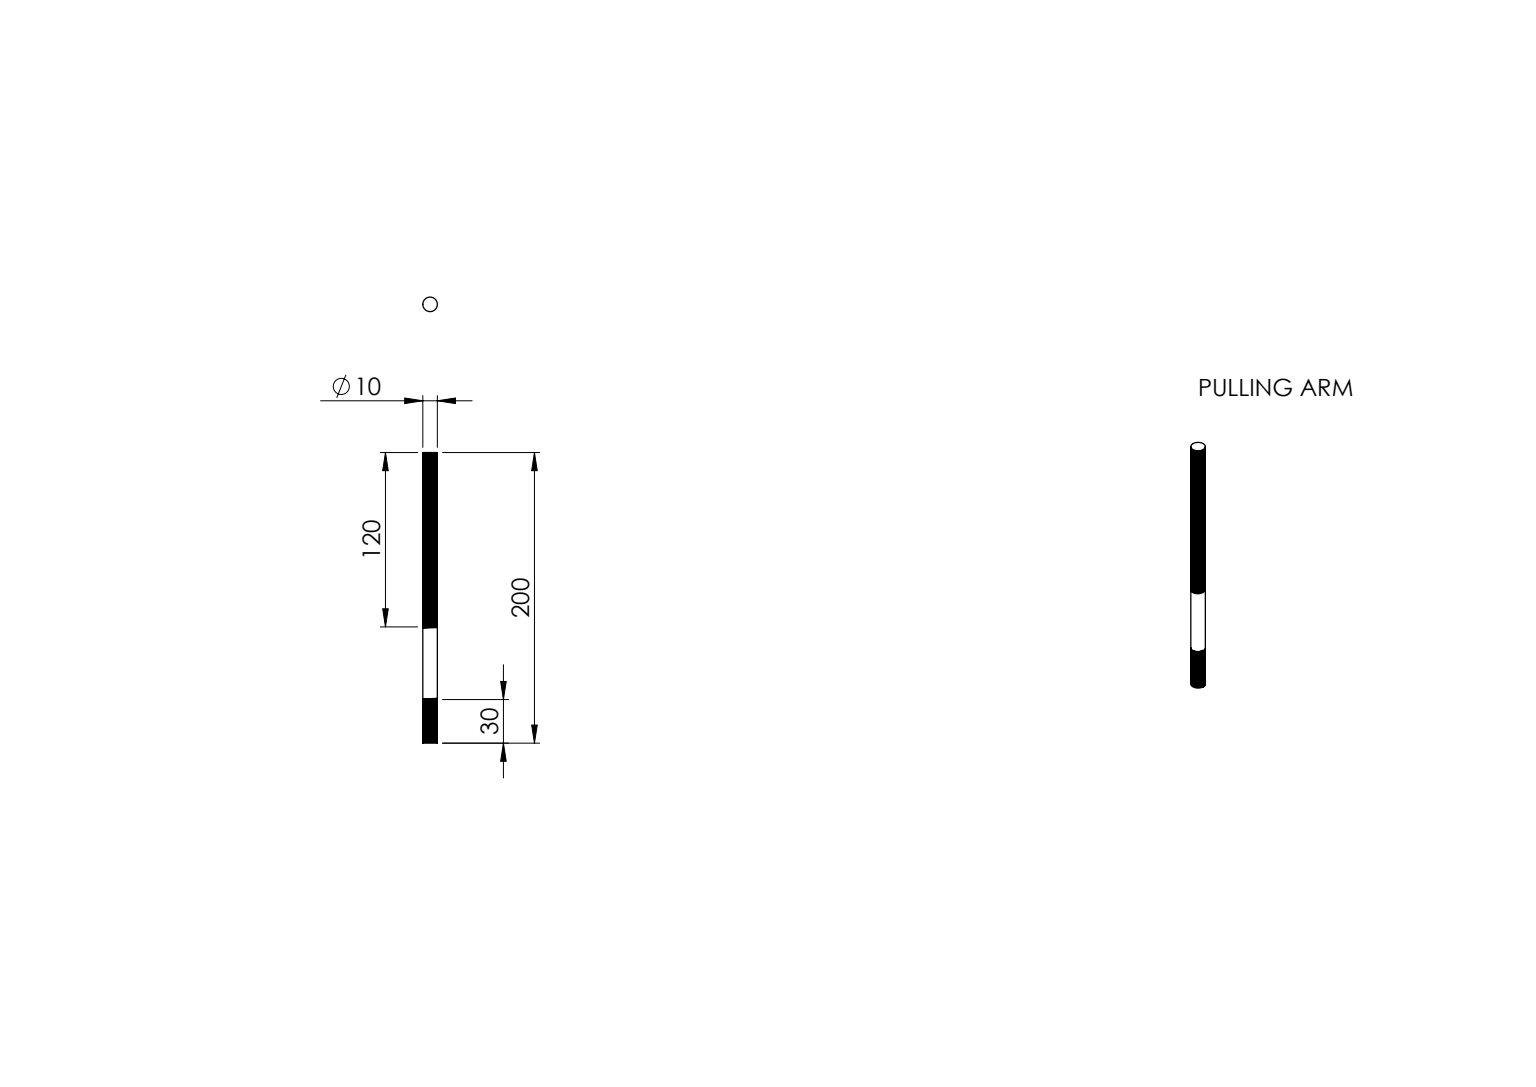
ISO-10303-21;
HEADER;
FILE_DESCRIPTION (('STEP AP214'),
    '1' );
FILE_NAME ('pulling arm.step',
    '2026-10-25T05:52:03',
    ( '' ),
    ( '' ),
    'SwSTEP 2.0',
    'SolidWorks 2026',
    '' );
FILE_SCHEMA (( 'AUTOMOTIVE_DESIGN' ));
ENDSEC;

DATA;
#1=CARTESIAN_POINT ( 'NONE',  ( -5.000000000000000888, -163.4375000000000284, 2.071067811865474617 ) ) ;
#4=ADVANCED_FACE ( 'NONE', ( #1643 ), #54385, .T. ) ;
#5=CARTESIAN_POINT ( 'NONE',  ( -4.458734124999998549, -12.47916666530107221, 2.574251347313722516 ) ) ;
#6=CARTESIAN_POINT ( 'NONE',  ( 2.229367062499998831, -45.89583333196774362, -3.861377020970580887 ) ) ;
#8=ADVANCED_FACE ( 'NONE', ( #45365 ), #55019, .T. ) ;
#9=CARTESIAN_POINT ( 'NONE',  ( -2.499999999999996447, -7.708333330602144429, 4.330127018922195425 ) ) ;
#10=CARTESIAN_POINT ( 'NONE',  ( -4.458734124999999437, -146.9375000013656063, -5.460374474430324690E-16 ) ) ;
#12=CARTESIAN_POINT ( 'NONE',  ( 3.061616997868383141E-16, -166.8750000027312126, -5.000000000000000000 ) ) ;
#15=CARTESIAN_POINT ( 'NONE',  ( -6.972266317189433020E-16, -69.12499999726880162, -5.000000000000000000 ) ) ;
#18=EDGE_LOOP ( 'NONE', ( #47508, #46479, #24387, #28082 ) ) ;
#23=CARTESIAN_POINT ( 'NONE',  ( -5.000000000000000000, -51.00000000000000711, 0.000000000000000000 ) ) ;
#24=CARTESIAN_POINT ( 'NONE',  ( -3.152548672688508926E-16, -0.5624999986344053626, -5.148502694627439702 ) ) ;
#26=CARTESIAN_POINT ( 'NONE',  ( -8.190561711645485556E-16, -153.6875000013656063, 4.458734124999999437 ) ) ;
#31=CARTESIAN_POINT ( 'NONE',  ( -2.499999999999996447, -74.83333333333332860, 4.330127018922195425 ) ) ;
#35=CARTESIAN_POINT ( 'NONE',  ( 2.499999999999998668, 29.66666666666666430, -4.330127018922193649 ) ) ;
#42=CARTESIAN_POINT ( 'NONE',  ( 4.458734124999999437, 16.18750000136559564, -5.460374474430324690E-16 ) ) ;
#45=CARTESIAN_POINT ( 'NONE',  ( -4.458734124999999437, -10.64583333196773829, -2.574251347313719407 ) ) ;
#48=CARTESIAN_POINT ( 'NONE',  ( 1.846868145590735200, -169.2500000013655779, -4.458734125000000326 ) ) ;
#49=CARTESIAN_POINT ( 'NONE',  ( 1.339745962155612702, -63.16965819600734022, -5.000000000000000000 ) ) ;
#50=AXIS2_PLACEMENT_3D ( 'NONE', #21966, #51867, #12316 ) ;
#55=CARTESIAN_POINT ( 'NONE',  ( 0.000000000000000000, -170.0000000000000000, 5.000000000000000000 ) ) ;
#57=CARTESIAN_POINT ( 'NONE',  ( -1.846868145590734756, -152.3750000013655779, -4.458734124999999437 ) ) ;
#59=CARTESIAN_POINT ( 'NONE',  ( 5.000000000000000000, -46.50000000000000000, -6.123233995736766282E-16 ) ) ;
#60=DIRECTION ( 'NONE',  ( -0.000000000000000000, 1.000000000000000000, -0.000000000000000000 ) ) ;
#64=DIRECTION ( 'NONE',  ( 0.000000000000000000, 0.000000000000000000, 1.000000000000000000 ) ) ;
#65=CARTESIAN_POINT ( 'NONE',  ( 5.000000000000000000, -2.500000000000002220, -6.123233995736766282E-16 ) ) ;
#66=CARTESIAN_POINT ( 'NONE',  ( 4.458734125000000326, -68.89583333196773651, 2.574251347313718519 ) ) ;
#67=CARTESIAN_POINT ( 'NONE',  ( -6.972266317189433020E-16, -49.24999999999999289, -5.000000000000000000 ) ) ;
#68=CARTESIAN_POINT ( 'NONE',  ( -2.499999999999996447, 0.2916666693978525737, 4.330127018922195425 ) ) ;
#69=CARTESIAN_POINT ( 'NONE',  ( -3.152548672688508926E-16, -36.56249999863441502, -5.148502694627439702 ) ) ;
#72=CARTESIAN_POINT ( 'NONE',  ( 1.975475456537005874E-15, 5.250000000000000000, 5.000000000000000000 ) ) ;
#73=CARTESIAN_POINT ( 'NONE',  ( 2.500000000000002220, -47.66666666666666430, 4.330127018922192761 ) ) ;
#74=CARTESIAN_POINT ( 'NONE',  ( 5.000000000000000000, -46.29166666393545881, -2.886751345948130876 ) ) ;
#77=CARTESIAN_POINT ( 'NONE',  ( -4.458734124999999437, -71.39583333196773651, -2.574251347313719407 ) ) ;
#78=( BOUNDED_CURVE ( )  B_SPLINE_CURVE ( 2, ( #57244, #32782, #8347, #47568, #3519, #57557, #53655, #9590, #43673 ),
 .UNSPECIFIED., .F., .F. ) 
 B_SPLINE_CURVE_WITH_KNOTS ( ( 3, 2, 2, 2, 3 ),
 ( 0.6562500000000000000, 0.6569444444444444420, 0.6583333333333333259, 0.6597222222222222099, 0.6604166666666666519 ),
 .UNSPECIFIED. ) 
 CURVE ( )  GEOMETRIC_REPRESENTATION_ITEM ( )  RATIONAL_B_SPLINE_CURVE ( ( 0.9330127018922194093, 0.9330127018922194093, 1.000000000000000000, 0.8660254037844387076, 1.000000000000000000, 0.8660254037844387076, 1.000000000000000000, 0.9330127018922194093, 0.9330127018922194093 ) ) 
 REPRESENTATION_ITEM ( '' )  );
#79=CARTESIAN_POINT ( 'NONE',  ( 4.458734124999999437, -144.7500000013656063, 1.846868145590737864 ) ) ;
#80=CARTESIAN_POINT ( 'NONE',  ( 2.229367062499998831, -80.64583333196773651, -3.861377020970580887 ) ) ;
#82=CARTESIAN_POINT ( 'NONE',  ( -2.229367062500000163, -28.72916666530107221, -3.861377020970580443 ) ) ;
#83=CARTESIAN_POINT ( 'NONE',  ( 5.000000000000000888, -73.45833333060214443, 2.886751345948126879 ) ) ;
#87=CARTESIAN_POINT ( 'NONE',  ( 0.000000000000000000, -170.0000000000000000, 0.000000000000000000 ) ) ;
#88=ORIENTED_EDGE ( 'NONE', *, *, #56635, .F. ) ;
#92=EDGE_LOOP ( 'NONE', ( #43267, #11517, #3797, #45500 ) ) ;
#95=EDGE_CURVE ( 'NONE', #8105, #59664, #19555, .T. ) ;
#96=CARTESIAN_POINT ( 'NONE',  ( -5.000000000000000000, -83.08333333333332860, -2.886751345948128211 ) ) ;
#97=CARTESIAN_POINT ( 'NONE',  ( -4.458734124999999437, -59.56249999863440081, 0.000000000000000000 ) ) ;
#98=EDGE_CURVE ( 'NONE', #46757, #28361, #15466, .T. ) ;
#105=CARTESIAN_POINT ( 'NONE',  ( 2.229367062500001939, 13.02083333469892779, 3.861377020970579999 ) ) ;
#107=CARTESIAN_POINT ( 'NONE',  ( 5.000000000000000888, -32.58333333333333570, 2.886751345948126879 ) ) ;
#108=CARTESIAN_POINT ( 'NONE',  ( -4.458734124999999437, -165.9375000013655779, -5.460374474430324690E-16 ) ) ;
#109=ORIENTED_EDGE ( 'NONE', *, *, #27518, .F. ) ;
#112=EDGE_CURVE ( 'NONE', #57087, #7190, #37304, .T. ) ;
#116=CARTESIAN_POINT ( 'NONE',  ( -4.999999999999998224, 2.083333333333333037, 2.886751345948131764 ) ) ;
#119=CARTESIAN_POINT ( 'NONE',  ( 3.061616997868383141E-16, -154.8750000027311842, -5.000000000000000000 ) ) ;
#122=CARTESIAN_POINT ( 'NONE',  ( -6.972266317189433020E-16, -58.24999999999999289, -5.000000000000000000 ) ) ;
#125=CARTESIAN_POINT ( 'NONE',  ( 4.458734124999998549, 8.020833334698926009, -2.574251347313721627 ) ) ;
#128=CARTESIAN_POINT ( 'NONE',  ( -9.184850993605147944E-16, -149.3750000027312126, 5.000000000000000000 ) ) ;
#133=CARTESIAN_POINT ( 'NONE',  ( -2.071067811865475061, -143.6875000000000284, -5.000000000000000888 ) ) ;
#135=CARTESIAN_POINT ( 'NONE',  ( 4.458734124999999437, -165.6250000013656063, -1.846868145590734978 ) ) ;
#136=CARTESIAN_POINT ( 'NONE',  ( 2.229367062499998831, -35.64583333196772941, -3.861377020970580887 ) ) ;
#137=CYLINDRICAL_SURFACE ( 'NONE', #42021, 5.000000000000000000 ) ;
#138=DIRECTION ( 'NONE',  ( 0.000000000000000000, 0.000000000000000000, 1.000000000000000000 ) ) ;
#140=CARTESIAN_POINT ( 'NONE',  ( 4.458734124999999437, -143.4375000013656063, 0.000000000000000000 ) ) ;
#141=VERTEX_POINT ( 'NONE', #56933 ) ;
#142=CARTESIAN_POINT ( 'NONE',  ( 4.458734125000001214, 28.85416666803225993, 2.574251347313718519 ) ) ;
#144=CARTESIAN_POINT ( 'NONE',  ( -2.229367062499996610, -62.39583333196774362, 3.861377020970582219 ) ) ;
#147=CARTESIAN_POINT ( 'NONE',  ( -5.000000000000000000, 17.91666666666666430, -2.886751345948128211 ) ) ;
#148=CARTESIAN_POINT ( 'NONE',  ( -3.152548672688508926E-16, -50.56249999863440792, -5.148502694627439702 ) ) ;
#149=CARTESIAN_POINT ( 'NONE',  ( -4.458734124999999437, -8.395833331967736513, -2.574251347313719407 ) ) ;
#153=CARTESIAN_POINT ( 'NONE',  ( 5.000000000000000000, -53.37499999726881583, -6.123233995736766282E-16 ) ) ;
#154=CARTESIAN_POINT ( 'NONE',  ( -6.972266317189433020E-16, 0.7499999999999996669, -5.000000000000000000 ) ) ;
#157=CARTESIAN_POINT ( 'NONE',  ( -3.152548672688508926E-16, -54.56249999863439371, -5.148502694627439702 ) ) ;
#158=CARTESIAN_POINT ( 'NONE',  ( -1.846868145590737420, -157.0000000013655779, 4.458734124999999437 ) ) ;
#160=CARTESIAN_POINT ( 'NONE',  ( -2.500000000000000444, -56.04166666393548013, -4.330127018922193649 ) ) ;
#161=EDGE_LOOP ( 'NONE', ( #40738, #29551, #10837, #16509 ) ) ;
#162=CARTESIAN_POINT ( 'NONE',  ( -3.152548672688508926E-16, 6.187500001365593860, -5.148502694627439702 ) ) ;
#165=FACE_OUTER_BOUND ( 'NONE', #54429, .T. ) ;
#166=CARTESIAN_POINT ( 'NONE',  ( 2.730187237215162345E-16, -156.1875000013655779, -4.458734124999999437 ) ) ;
#168=CARTESIAN_POINT ( 'NONE',  ( 5.000000000000000000, -87.29166666393547303, -2.886751345948130876 ) ) ;
#170=CARTESIAN_POINT ( 'NONE',  ( 0.000000000000000000, -170.0000000000000000, 0.000000000000000000 ) ) ;
#171=CARTESIAN_POINT ( 'NONE',  ( -4.458734124999999437, -45.56249999863440081, 0.000000000000000000 ) ) ;
#173=CARTESIAN_POINT ( 'NONE',  ( 1.339745962155615144, 9.419658201469706782, 4.999999999999999112 ) ) ;
#175=CARTESIAN_POINT ( 'NONE',  ( -5.000000000000000000, -156.6250000027311842, -6.123233995736766282E-16 ) ) ;
#176=VERTEX_POINT ( 'NONE', #46964 ) ;
#177=CARTESIAN_POINT ( 'NONE',  ( 9.457646018065525792E-16, -89.31249999863440792, 5.148502694627439702 ) ) ;
#179=CARTESIAN_POINT ( 'NONE',  ( -3.535533905932737309, -165.6250000000000284, -3.535533905932738197 ) ) ;
#181=CARTESIAN_POINT ( 'NONE',  ( 1.975475456537005874E-15, -52.62499999726880873, 5.000000000000000000 ) ) ;
#185=CARTESIAN_POINT ( 'NONE',  ( -5.000000000000000000, -78.95833333060213022, -2.886751345948128211 ) ) ;
#189=CARTESIAN_POINT ( 'NONE',  ( 2.500000000000002220, -42.54166666393548013, 4.330127018922192761 ) ) ;
#190=CARTESIAN_POINT ( 'NONE',  ( -1.339745962155613812, -46.08034179853028434, -5.000000000000000000 ) ) ;
#197=CARTESIAN_POINT ( 'NONE',  ( 5.000000000000000000, -162.1875000027311842, 2.071067811865478614 ) ) ;
#207=CARTESIAN_POINT ( 'NONE',  ( -6.972266317189433020E-16, -48.12499999726880873, -5.000000000000000000 ) ) ;
#208=CARTESIAN_POINT ( 'NONE',  ( 9.457646018065525792E-16, -14.06249999863440436, 5.148502694627439702 ) ) ;
#209=CARTESIAN_POINT ( 'NONE',  ( 2.499999999999998668, -71.33333333333332860, -4.330127018922193649 ) ) ;
#210=CARTESIAN_POINT ( 'NONE',  ( -9.184850993605147944E-16, -153.2500000000000000, 5.000000000000000000 ) ) ;
#213=CARTESIAN_POINT ( 'NONE',  ( -2.229367062499996610, -46.39583333196774362, 3.861377020970582219 ) ) ;
#219=CARTESIAN_POINT ( 'NONE',  ( -2.229367062499996610, 11.85416666803225993, 3.861377020970582219 ) ) ;
#222=CARTESIAN_POINT ( 'NONE',  ( -2.229367062500000163, -88.72916666530106511, -3.861377020970580443 ) ) ;
#223=CARTESIAN_POINT ( 'NONE',  ( -2.229367062500000163, 20.27083333469892779, -3.861377020970580443 ) ) ;
#225=CARTESIAN_POINT ( 'NONE',  ( 5.000000000000000000, 8.708333336064518093, -2.886751345948129988 ) ) ;
#226=ORIENTED_EDGE ( 'NONE', *, *, #26912, .F. ) ;
#229=( BOUNDED_CURVE ( )  B_SPLINE_CURVE ( 2, ( #7653, #61058, #50752, #27257, #26303, #46568, #45926, #60737, #46883 ),
 .UNSPECIFIED., .F., .F. ) 
 B_SPLINE_CURVE_WITH_KNOTS ( ( 3, 2, 2, 2, 3 ),
 ( 0.3562500000000000111, 0.3569444444444444531, 0.3583333333333333370, 0.3597222222222222210, 0.3604166666666666630 ),
 .UNSPECIFIED. ) 
 CURVE ( )  GEOMETRIC_REPRESENTATION_ITEM ( )  RATIONAL_B_SPLINE_CURVE ( ( 0.9330127018922194093, 0.9330127018922194093, 1.000000000000000000, 0.8660254037844387076, 1.000000000000000000, 0.8660254037844387076, 1.000000000000000000, 0.9330127018922194093, 0.9330127018922194093 ) ) 
 REPRESENTATION_ITEM ( '' )  );
#230=CARTESIAN_POINT ( 'NONE',  ( 1.060575238724906964E-15, -36.75000000000000711, 5.773502691896257311 ) ) ;
#231=CARTESIAN_POINT ( 'NONE',  ( 4.458734124999998549, -35.72916666530107221, -2.574251347313721627 ) ) ;
#232=CARTESIAN_POINT ( 'NONE',  ( -3.535250795749689387E-16, -35.12499999726881583, -5.773502691896257311 ) ) ;
#233=CARTESIAN_POINT ( 'NONE',  ( -4.458734124999998549, -68.22916666530107932, 2.574251347313722516 ) ) ;
#234=ORIENTED_EDGE ( 'NONE', *, *, #6265, .F. ) ;
#236=CARTESIAN_POINT ( 'NONE',  ( -3.152548672688508926E-16, -12.56249999863440081, -5.148502694627439702 ) ) ;
#237=CARTESIAN_POINT ( 'NONE',  ( -3.152548672688508926E-16, -15.81249999863440436, -5.148502694627439702 ) ) ;
#238=ORIENTED_EDGE ( 'NONE', *, *, #445, .F. ) ;
#239=CARTESIAN_POINT ( 'NONE',  ( 2.500000000000002220, -83.66666666666667140, 4.330127018922192761 ) ) ;
#240=CARTESIAN_POINT ( 'NONE',  ( -4.458734125000000326, -167.0000000013655779, -1.846868145590735644 ) ) ;
#243=CARTESIAN_POINT ( 'NONE',  ( 5.000000000000000000, -81.29166666393547303, -2.886751345948129988 ) ) ;
#244=LINE ( 'NONE', #10504, #18998 ) ;
#247=CARTESIAN_POINT ( 'NONE',  ( -4.458734124999998549, -29.47916666530106866, 2.574251347313722516 ) ) ;
#250=CARTESIAN_POINT ( 'NONE',  ( 1.846868145590736310, -167.8750000013656063, 4.458734124999999437 ) ) ;
#252=CYLINDRICAL_SURFACE ( 'NONE', #21504, 5.000000000000000000 ) ;
#257=CARTESIAN_POINT ( 'NONE',  ( -1.846868145590734756, -147.3750000013656063, -4.458734124999999437 ) ) ;
#259=CARTESIAN_POINT ( 'NONE',  ( 6.123233995736766282E-16, -170.0000000000000000, -5.000000000000000000 ) ) ;
#264=CARTESIAN_POINT ( 'NONE',  ( -4.458734125000001214, -141.1250000013655779, 1.846868145590734089 ) ) ;
#269=CARTESIAN_POINT ( 'NONE',  ( 4.458734125000001214, -75.14583333196775072, 2.574251347313718519 ) ) ;
#271=CARTESIAN_POINT ( 'NONE',  ( 1.975475456537005874E-15, -69.74999999999998579, 5.000000000000000000 ) ) ;
#272=CARTESIAN_POINT ( 'NONE',  ( -6.972266317189433020E-16, -58.12499999726880162, -5.000000000000000000 ) ) ;
#275=CARTESIAN_POINT ( 'NONE',  ( -6.972266317189433020E-16, 13.87500000273118594, -5.000000000000000000 ) ) ;
#281=CARTESIAN_POINT ( 'NONE',  ( -4.458734124999999437, 16.43750000136559564, 0.000000000000000000 ) ) ;
#288=CARTESIAN_POINT ( 'NONE',  ( -4.458734124999999437, 2.687500001365593860, 0.000000000000000000 ) ) ;
#289=ORIENTED_EDGE ( 'NONE', *, *, #15037, .T. ) ;
#290=CARTESIAN_POINT ( 'NONE',  ( 4.458734124999999437, -24.06249999863440436, -5.460374474430324690E-16 ) ) ;
#294=CARTESIAN_POINT ( 'NONE',  ( 4.458734125000001214, 25.10416666803225638, 2.574251347313718519 ) ) ;
#297=CARTESIAN_POINT ( 'NONE',  ( -4.458734124999997661, -71.47916666530107932, 2.574251347313722516 ) ) ;
#300=CARTESIAN_POINT ( 'NONE',  ( 2.499999999999998668, 27.79166666939785202, -4.330127018922193649 ) ) ;
#301=ORIENTED_EDGE ( 'NONE', *, *, #22893, .T. ) ;
#303=CARTESIAN_POINT ( 'NONE',  ( 5.000000000000000000, -18.50000000000000355, -6.123233995736766282E-16 ) ) ;
#304=CARTESIAN_POINT ( 'NONE',  ( -4.458734124999999437, -22.39583333196773651, -2.574251347313719407 ) ) ;
#305=CARTESIAN_POINT ( 'NONE',  ( -2.229367062500000163, -81.47916666530106511, -3.861377020970580443 ) ) ;
#306=CARTESIAN_POINT ( 'NONE',  ( 1.846868145590735200, -166.5000000013655779, -4.458734125000000326 ) ) ;
#307=CARTESIAN_POINT ( 'NONE',  ( 1.060575238724906964E-15, -19.62499999726881583, 5.773502691896257311 ) ) ;
#308=CARTESIAN_POINT ( 'NONE',  ( 4.458734124999999437, -48.81249999863440792, -5.460374474430324690E-16 ) ) ;
#312=CARTESIAN_POINT ( 'NONE',  ( -3.152548672688508926E-16, 3.187500001365594748, -5.148502694627439702 ) ) ;
#315=CARTESIAN_POINT ( 'NONE',  ( -2.500000000000000444, -64.16666666666665719, -4.330127018922193649 ) ) ;
#316=CARTESIAN_POINT ( 'NONE',  ( -1.846868145590737420, -152.0000000013655779, 4.458734124999999437 ) ) ;
#319=CARTESIAN_POINT ( 'NONE',  ( 5.000000000000000888, -161.9375000000000284, -2.071067811865475505 ) ) ;
#320=FACE_OUTER_BOUND ( 'NONE', #3833, .T. ) ;
#322=CARTESIAN_POINT ( 'NONE',  ( 2.229367062499998831, -10.89583333196773829, -3.861377020970580887 ) ) ;
#323=CARTESIAN_POINT ( 'NONE',  ( 4.458734124999998549, -45.97916666530106511, -2.574251347313721627 ) ) ;
#324=CARTESIAN_POINT ( 'NONE',  ( -6.972266317189433020E-16, -8.124999997268814056, -5.000000000000000000 ) ) ;
#325=CARTESIAN_POINT ( 'NONE',  ( -8.190561711645485556E-16, -149.6875000013656063, 4.458734124999999437 ) ) ;
#328=VERTEX_POINT ( 'NONE', #61131 ) ;
#332=CARTESIAN_POINT ( 'NONE',  ( 5.000000000000000888, -29.45833333060214443, 2.886751345948126879 ) ) ;
#338=CARTESIAN_POINT ( 'NONE',  ( -5.147856630858197489E-14, 2.375000002731183724, 5.000000000000000000 ) ) ;
#339=CARTESIAN_POINT ( 'NONE',  ( -4.458734124999999437, -4.395833331967740065, -2.574251347313719407 ) ) ;
#340=DIRECTION ( 'NONE',  ( -0.000000000000000000, -1.000000000000000000, -0.000000000000000000 ) ) ;
#341=CARTESIAN_POINT ( 'NONE',  ( 4.458734124999997661, -148.5000000013656347, 1.846868145590737864 ) ) ;
#348=CARTESIAN_POINT ( 'NONE',  ( 1.162044386198238837E-16, 28.37500000273118417, 5.000000000000000000 ) ) ;
#349=( BOUNDED_CURVE ( )  B_SPLINE_CURVE ( 2, ( #32871, #48595, #37379, #53427, #52500, #18392, #37690, #3921, #43452 ),
 .UNSPECIFIED., .F., .F. ) 
 B_SPLINE_CURVE_WITH_KNOTS ( ( 3, 2, 2, 2, 3 ),
 ( 0.5229166666666666963, 0.5236111111111111382, 0.5250000000000000222, 0.5263888888888889062, 0.5270833333333333481 ),
 .UNSPECIFIED. ) 
 CURVE ( )  GEOMETRIC_REPRESENTATION_ITEM ( )  RATIONAL_B_SPLINE_CURVE ( ( 0.9330127018922194093, 0.9330127018922194093, 1.000000000000000000, 0.8660254037844387076, 1.000000000000000000, 0.8660254037844387076, 1.000000000000000000, 0.9330127018922194093, 0.9330127018922194093 ) ) 
 REPRESENTATION_ITEM ( '' )  );
#355=DIRECTION ( 'NONE',  ( -0.000000000000000000, 1.000000000000000000, -0.000000000000000000 ) ) ;
#356=CARTESIAN_POINT ( 'NONE',  ( -2.229367062500000163, 18.52083333469892779, -3.861377020970580443 ) ) ;
#359=CARTESIAN_POINT ( 'NONE',  ( 4.458734125000000326, -8.145833331967736513, 2.574251347313718519 ) ) ;
#362=CARTESIAN_POINT ( 'NONE',  ( -4.458734125000000326, -169.0000000013655779, -1.846868145590735644 ) ) ;
#366=ADVANCED_FACE ( 'NONE', ( #2909 ), #32473, .T. ) ;
#369=CARTESIAN_POINT ( 'NONE',  ( 5.000000000000000000, -142.1875000027312126, 2.071067811865478614 ) ) ;
#371=CARTESIAN_POINT ( 'NONE',  ( 3.152801135295366208, -153.8125000013656063, 3.152801135295367985 ) ) ;
#373=CARTESIAN_POINT ( 'NONE',  ( 1.339745962155615144, -46.70534180126147561, 4.999999999999999112 ) ) ;
#379=CARTESIAN_POINT ( 'NONE',  ( -2.500000000000000444, -2.166666666666663854, -4.330127018922193649 ) ) ;
#380=EDGE_CURVE ( 'NONE', #47490, #35906, #55280, .T. ) ;
#381=CARTESIAN_POINT ( 'NONE',  ( -4.458734124999999437, -67.39583333196773651, -2.574251347313719407 ) ) ;
#384=CARTESIAN_POINT ( 'NONE',  ( 5.000000000000000000, -1.291666663935479908, -2.886751345948129988 ) ) ;
#385=CARTESIAN_POINT ( 'NONE',  ( -4.458734124999999437, -36.31249999863440792, 0.000000000000000000 ) ) ;
#386=ORIENTED_EDGE ( 'NONE', *, *, #25943, .F. ) ;
#390=ORIENTED_EDGE ( 'NONE', *, *, #14942, .T. ) ;
#391=CARTESIAN_POINT ( 'NONE',  ( -6.972266317189433020E-16, 5.749999999999999112, -5.000000000000000000 ) ) ;
#392=CARTESIAN_POINT ( 'NONE',  ( 2.500000000000002220, -50.66666666666666430, 4.330127018922192761 ) ) ;
#395=CARTESIAN_POINT ( 'NONE',  ( -5.000000000000000000, -4.083333333333334814, -2.886751345948128211 ) ) ;
#396=CARTESIAN_POINT ( 'NONE',  ( 4.458734124999998549, -72.72916666530106511, -2.574251347313721627 ) ) ;
#397=CARTESIAN_POINT ( 'NONE',  ( -3.152801135295367096, -143.3125000013655779, -3.152801135295367541 ) ) ;
#398=CARTESIAN_POINT ( 'NONE',  ( -2.229367062499996610, -81.14583333196773651, 3.861377020970582219 ) ) ;
#400=CARTESIAN_POINT ( 'NONE',  ( 9.457646018065525792E-16, -31.31249999863440436, 5.148502694627439702 ) ) ;
#401=CARTESIAN_POINT ( 'NONE',  ( -4.999999999999999112, -70.79166666393548724, 2.886751345948131764 ) ) ;
#406=CARTESIAN_POINT ( 'NONE',  ( 1.339745962155614256, 28.70534180126147561, -4.999999999999999112 ) ) ;
#407=ORIENTED_EDGE ( 'NONE', *, *, #54703, .T. ) ;
#409=( BOUNDED_CURVE ( )  B_SPLINE_CURVE ( 2, ( #59998, #10777, #6592, #50336, #36184, #21392, #31028, #50979, #30387 ),
 .UNSPECIFIED., .F., .F. ) 
 B_SPLINE_CURVE_WITH_KNOTS ( ( 3, 2, 2, 2, 3 ),
 ( 0.4083333333333336590, 0.4125000000000003109, 0.4166666666666670182, 0.4208333333333336701, 0.4250000000000003220 ),
 .UNSPECIFIED. ) 
 CURVE ( )  GEOMETRIC_REPRESENTATION_ITEM ( )  RATIONAL_B_SPLINE_CURVE ( ( 0.9999999999999938938, 0.9238795325112928447, 1.000000000000000000, 0.9238795325112867385, 1.000000000000000000, 0.9238795325112867385, 1.000000000000000000, 0.9238795325112806323, 1.000000000000005995 ) ) 
 REPRESENTATION_ITEM ( '' )  );
#411=EDGE_CURVE ( 'NONE', #51356, #16274, #33465, .T. ) ;
#412=CARTESIAN_POINT ( 'NONE',  ( 2.229367062499998831, -56.89583333196773651, -3.861377020970580887 ) ) ;
#414=ORIENTED_EDGE ( 'NONE', *, *, #41306, .F. ) ;
#415=CARTESIAN_POINT ( 'NONE',  ( -5.000000000000000888, -146.5625000000000000, -2.071067811865475949 ) ) ;
#417=CARTESIAN_POINT ( 'NONE',  ( -4.458734124999998549, 11.77083333469892601, 2.574251347313722516 ) ) ;
#419=CARTESIAN_POINT ( 'NONE',  ( -4.458734124999999437, -162.0000000013656063, -1.846868145590735644 ) ) ;
#422=CARTESIAN_POINT ( 'NONE',  ( -5.000000000000000000, -69.87499999726880162, 0.000000000000000000 ) ) ;
#425=CARTESIAN_POINT ( 'NONE',  ( -6.972266317189433020E-16, -40.12499999726880162, -5.000000000000000000 ) ) ;
#428=CARTESIAN_POINT ( 'NONE',  ( -6.972266317189433020E-16, 5.749999999999999112, -5.000000000000000000 ) ) ;
#429=CARTESIAN_POINT ( 'NONE',  ( 5.000000000000000888, -78.45833333060214443, 2.886751345948126879 ) ) ;
#434=CARTESIAN_POINT ( 'NONE',  ( -3.152548672688508926E-16, 6.187500001365593860, -5.148502694627439702 ) ) ;
#435=CARTESIAN_POINT ( 'NONE',  ( -4.999999999999998224, -9.791666663935476578, 2.886751345948131764 ) ) ;
#437=CARTESIAN_POINT ( 'NONE',  ( 2.071067811865475505, -147.9375000027312126, -5.000000000000000888 ) ) ;
#442=CYLINDRICAL_SURFACE ( 'NONE', #40067, 5.000000000000000000 ) ;
#443=EDGE_CURVE ( 'NONE', #39270, #17071, #61863, .T. ) ;
#445=EDGE_CURVE ( 'NONE', #14245, #8450, #57255, .T. ) ;
#447=CARTESIAN_POINT ( 'NONE',  ( -1.846868145590737420, -166.0000000013656063, 4.458734124999997661 ) ) ;
#448=CARTESIAN_POINT ( 'NONE',  ( -2.229367062500000163, -34.47916666530107221, -3.861377020970580443 ) ) ;
#449=EDGE_CURVE ( 'NONE', #23480, #42348, #53192, .T. ) ;
#453=CARTESIAN_POINT ( 'NONE',  ( 4.458734124999999437, -145.4375000013656063, 0.000000000000000000 ) ) ;
#455=CARTESIAN_POINT ( 'NONE',  ( 2.229367062499998831, 29.10416666803225993, -3.861377020970580887 ) ) ;
#457=CARTESIAN_POINT ( 'NONE',  ( -4.458734124999999437, -61.56249999863440081, 0.000000000000000000 ) ) ;
#461=CARTESIAN_POINT ( 'NONE',  ( 5.000000000000000000, 12.58333333333333215, -2.886751345948129988 ) ) ;
#463=CARTESIAN_POINT ( 'NONE',  ( -2.229367062500000163, -53.47916666530107221, -3.861377020970580443 ) ) ;
#464=CARTESIAN_POINT ( 'NONE',  ( 2.229367062500001939, -6.979166665301073103, 3.861377020970579999 ) ) ;
#465=CARTESIAN_POINT ( 'NONE',  ( -5.000000000000000000, 4.041666669397852019, -2.886751345948128211 ) ) ;
#466=CARTESIAN_POINT ( 'NONE',  ( -1.339745962155610925, -8.794658198738519062, 5.000000000000000000 ) ) ;
#472=CARTESIAN_POINT ( 'NONE',  ( 9.457646018065525792E-16, -52.06249999863440792, 5.148502694627439702 ) ) ;
#473=CARTESIAN_POINT ( 'NONE',  ( 3.152801135295366208, -154.8125000013656063, 3.152801135295367985 ) ) ;
#474=ADVANCED_FACE ( 'NONE', ( #38255 ), #24401, .T. ) ;
#475=AXIS2_PLACEMENT_3D ( 'NONE', #22306, #28376, #22629 ) ;
#476=CARTESIAN_POINT ( 'NONE',  ( 1.060575238724906964E-15, -53.62499999726880873, 5.773502691896257311 ) ) ;
#478=CARTESIAN_POINT ( 'NONE',  ( 4.458734125000001214, 2.854166668032259491, 2.574251347313718519 ) ) ;
#482=CARTESIAN_POINT ( 'NONE',  ( 1.846868145590735200, -156.2500000013656063, -4.458734125000000326 ) ) ;
#484=CARTESIAN_POINT ( 'NONE',  ( 2.499999999999998668, -83.33333333333332860, -4.330127018922193649 ) ) ;
#487=CARTESIAN_POINT ( 'NONE',  ( 2.229367062499998831, -40.89583333196773651, -3.861377020970580887 ) ) ;
#490=CARTESIAN_POINT ( 'NONE',  ( 1.339745962155612702, 3.830341803992665550, -5.000000000000000000 ) ) ;
#492=CARTESIAN_POINT ( 'NONE',  ( 4.458734124999999437, 28.18750000136559208, -5.460374474430324690E-16 ) ) ;
#495=CARTESIAN_POINT ( 'NONE',  ( -4.999999999999998224, 24.08333333333333215, 2.886751345948131764 ) ) ;
#497=CARTESIAN_POINT ( 'NONE',  ( -2.500000000000000444, -62.04166666393547303, -4.330127018922193649 ) ) ;
#499=CARTESIAN_POINT ( 'NONE',  ( 5.000000000000000000, -33.50000000000000000, -6.123233995736766282E-16 ) ) ;
#502=CARTESIAN_POINT ( 'NONE',  ( -2.500000000000000444, 4.833333333333332149, -4.330127018922193649 ) ) ;
#503=CARTESIAN_POINT ( 'NONE',  ( -5.147856630858197489E-14, 3.375000002731183280, 5.000000000000000000 ) ) ;
#504=CARTESIAN_POINT ( 'NONE',  ( 4.458734124999999437, -88.06249999863439371, -5.460374474430324690E-16 ) ) ;
#507=EDGE_LOOP ( 'NONE', ( #44935, #18884, #62333, #60547 ) ) ;
#510=CARTESIAN_POINT ( 'NONE',  ( 2.071067811865476394, -163.3125000027311842, 5.000000000000000000 ) ) ;
#514=CARTESIAN_POINT ( 'NONE',  ( -4.999999999999998224, -66.91666666666667140, 2.886751345948131764 ) ) ;
#522=CARTESIAN_POINT ( 'NONE',  ( -3.535533905932737309, -141.7500000027311842, -3.535533905932738197 ) ) ;
#523=CARTESIAN_POINT ( 'NONE',  ( -4.458734124999997661, -21.22916666530107221, 2.574251347313722516 ) ) ;
#524=CARTESIAN_POINT ( 'NONE',  ( -5.000000000000000000, -79.95833333060213022, -2.886751345948128211 ) ) ;
#525=CARTESIAN_POINT ( 'NONE',  ( 5.000000000000000000, -155.0625000000000284, 2.071067811865478614 ) ) ;
#528=CARTESIAN_POINT ( 'NONE',  ( 2.229367062499998831, -45.89583333196774362, -3.861377020970580887 ) ) ;
#529=CYLINDRICAL_SURFACE ( 'NONE', #46889, 5.000000000000000000 ) ;
#531=CARTESIAN_POINT ( 'NONE',  ( -4.999999999999999112, 28.08333333333333570, 2.886751345948131764 ) ) ;
#535=CARTESIAN_POINT ( 'NONE',  ( 4.458734125000001214, 8.104166668032261711, 2.574251347313718519 ) ) ;
#537=CARTESIAN_POINT ( 'NONE',  ( -5.000000000000000000, 12.00000000000000000, 0.000000000000000000 ) ) ;
#538=CARTESIAN_POINT ( 'NONE',  ( 1.339745962155615144, -82.70534180126146850, 4.999999999999999112 ) ) ;
#539=CARTESIAN_POINT ( 'NONE',  ( -4.458734124999999437, 19.35416666803225993, -2.574251347313719407 ) ) ;
#541=CARTESIAN_POINT ( 'NONE',  ( -3.535250795749689387E-16, 6.875000002731186832, -5.773502691896257311 ) ) ;
#547=CARTESIAN_POINT ( 'NONE',  ( 4.458734125000001214, -40.89583333196773651, 2.574251347313718519 ) ) ;
#548=EDGE_CURVE ( 'NONE', #7140, #8617, #11299, .T. ) ;
#549=ADVANCED_FACE ( 'NONE', ( #45611 ), #44645, .T. ) ;
#550=CARTESIAN_POINT ( 'NONE',  ( -2.500000000000000444, -39.04166666393548013, -4.330127018922193649 ) ) ;
#551=VERTEX_POINT ( 'NONE', #605 ) ;
#553=CARTESIAN_POINT ( 'NONE',  ( 2.229367062500001939, -11.97916666530107044, 3.861377020970579999 ) ) ;
#554=CARTESIAN_POINT ( 'NONE',  ( 4.458734124999999437, -13.06249999863440259, -5.460374474430324690E-16 ) ) ;
#556=CARTESIAN_POINT ( 'NONE',  ( -5.000000000000000000, -82.08333333333332860, -2.886751345948128211 ) ) ;
#557=CARTESIAN_POINT ( 'NONE',  ( 3.152801135295366208, -168.5625000013656063, 3.152801135295367985 ) ) ;
#559=CARTESIAN_POINT ( 'NONE',  ( 2.500000000000002220, -86.54166666393547303, 4.330127018922192761 ) ) ;
#560=CARTESIAN_POINT ( 'NONE',  ( -1.339745962155613812, -18.20534180126147916, -5.000000000000000000 ) ) ;
#561=ORIENTED_EDGE ( 'NONE', *, *, #9529, .F. ) ;
#563=CARTESIAN_POINT ( 'NONE',  ( -2.229367062500000163, -24.72916666530106866, -3.861377020970580443 ) ) ;
#564=CARTESIAN_POINT ( 'NONE',  ( 5.000000000000000000, -29.41666666666666785, -2.886751345948130876 ) ) ;
#565=EDGE_LOOP ( 'NONE', ( #55291, #23421, #60900, #47144 ) ) ;
#567=CARTESIAN_POINT ( 'NONE',  ( 4.458734124999999437, -163.7500000013655779, 1.846868145590737864 ) ) ;
#569=CARTESIAN_POINT ( 'NONE',  ( 1.339745962155612702, -23.29465819873851729, -5.000000000000000000 ) ) ;
#570=ORIENTED_EDGE ( 'NONE', *, *, #6344, .F. ) ;
#572=CARTESIAN_POINT ( 'NONE',  ( 2.229367062500001939, -75.22916666530106511, 3.861377020970579999 ) ) ;
#575=CARTESIAN_POINT ( 'NONE',  ( 1.846868145590735200, -145.5000000013656063, -4.458734124999999437 ) ) ;
#581=CARTESIAN_POINT ( 'NONE',  ( -3.152801135295367985, -140.0625000013655779, 3.152801135295367096 ) ) ;
#584=CARTESIAN_POINT ( 'NONE',  ( -1.339745962155613812, -40.08034179853028434, -5.000000000000000000 ) ) ;
#587=CARTESIAN_POINT ( 'NONE',  ( 9.457646018065525792E-16, -74.31249999863440792, 5.148502694627439702 ) ) ;
#589=CARTESIAN_POINT ( 'NONE',  ( 2.499999999999998668, -54.20833333060213732, -4.330127018922193649 ) ) ;
#590=LINE ( 'NONE', #44308, #43871 ) ;
#592=VERTEX_POINT ( 'NONE', #20542 ) ;
#593=DIRECTION ( 'NONE',  ( -0.000000000000000000, 1.000000000000000000, -0.000000000000000000 ) ) ;
#598=CARTESIAN_POINT ( 'NONE',  ( 4.458734124999998549, 19.02083333469892779, -2.574251347313721627 ) ) ;
#599=CARTESIAN_POINT ( 'NONE',  ( -2.498395430326213474E-14, 20.37500000273118062, 5.000000000000000000 ) ) ;
#605=CARTESIAN_POINT ( 'NONE',  ( 1.975475456537005874E-15, 19.37500000273118772, 5.000000000000000000 ) ) ;
#606=CARTESIAN_POINT ( 'NONE',  ( -2.229367062500000163, -1.479166665301071770, -3.861377020970580443 ) ) ;
#608=ORIENTED_EDGE ( 'NONE', *, *, #31528, .F. ) ;
#609=CARTESIAN_POINT ( 'NONE',  ( 4.458734124999998549, -29.97916666530107221, -2.574251347313721627 ) ) ;
#613=CARTESIAN_POINT ( 'NONE',  ( -4.458734124999999437, 23.68750000136559564, 0.000000000000000000 ) ) ;
#614=CARTESIAN_POINT ( 'NONE',  ( 2.499999999999998668, 26.79166666939785202, -4.330127018922193649 ) ) ;
#616=CARTESIAN_POINT ( 'NONE',  ( -2.229367062500000163, -73.72916666530106511, -3.861377020970580443 ) ) ;
#619=CARTESIAN_POINT ( 'NONE',  ( -5.000000000000000000, 24.12500000273118417, 0.000000000000000000 ) ) ;
#620=ORIENTED_EDGE ( 'NONE', *, *, #55792, .F. ) ;
#623=CARTESIAN_POINT ( 'NONE',  ( 2.499999999999998668, -19.33333333333333570, -4.330127018922193649 ) ) ;
#624=CARTESIAN_POINT ( 'NONE',  ( 2.229367062499998831, -20.64583333196774007, -3.861377020970580887 ) ) ;
#625=CARTESIAN_POINT ( 'NONE',  ( 4.458734124999998549, -82.72916666530106511, -2.574251347313721627 ) ) ;
#626=CARTESIAN_POINT ( 'NONE',  ( 5.000000000000000000, -22.29166666393548368, -2.886751345948129988 ) ) ;
#627=CARTESIAN_POINT ( 'NONE',  ( 4.458734125000001214, -50.89583333196772230, 2.574251347313718519 ) ) ;
#629=CARTESIAN_POINT ( 'NONE',  ( 2.500000000000002220, -70.54166666393547303, 4.330127018922192761 ) ) ;
#631=CARTESIAN_POINT ( 'NONE',  ( 4.458734124999999437, 3.937500001365595192, -5.460374474430324690E-16 ) ) ;
#634=CARTESIAN_POINT ( 'NONE',  ( 5.000000000000000888, -68.58333333333334281, 2.886751345948126879 ) ) ;
#635=CARTESIAN_POINT ( 'NONE',  ( 4.458734124999999437, -153.6875000013656063, 0.000000000000000000 ) ) ;
#638=( BOUNDED_CURVE ( )  B_SPLINE_CURVE ( 2, ( #48959, #44134, #22729, #58938, #61967, #33863, #48646, #56828, #22412 ),
 .UNSPECIFIED., .F., .F. ) 
 B_SPLINE_CURVE_WITH_KNOTS ( ( 3, 2, 2, 2, 3 ),
 ( 0.4312500000000000222, 0.4319444444444444642, 0.4333333333333333481, 0.4347222222222222321, 0.4354166666666666741 ),
 .UNSPECIFIED. ) 
 CURVE ( )  GEOMETRIC_REPRESENTATION_ITEM ( )  RATIONAL_B_SPLINE_CURVE ( ( 0.9330127018922194093, 0.9330127018922194093, 1.000000000000000000, 0.8660254037844387076, 1.000000000000000000, 0.8660254037844387076, 1.000000000000000000, 0.9330127018922194093, 0.9330127018922194093 ) ) 
 REPRESENTATION_ITEM ( '' )  );
#639=CARTESIAN_POINT ( 'NONE',  ( -3.535533905932737309, -161.6250000000000284, -3.535533905932738197 ) ) ;
#642=CARTESIAN_POINT ( 'NONE',  ( -2.229367062499996610, -12.39583333196774007, 3.861377020970582219 ) ) ;
#643=CARTESIAN_POINT ( 'NONE',  ( 2.229367062499998831, -46.89583333196774362, -3.861377020970580887 ) ) ;
#645=CARTESIAN_POINT ( 'NONE',  ( 4.458734125000000326, -145.3750000013656347, -1.846868145590734978 ) ) ;
#647=CARTESIAN_POINT ( 'NONE',  ( -2.498395430326213474E-14, 21.37500000273118062, 5.000000000000000000 ) ) ;
#650=CARTESIAN_POINT ( 'NONE',  ( -6.972266317189433020E-16, -12.12499999726881583, -5.000000000000000000 ) ) ;
#654=EDGE_CURVE ( 'NONE', #27389, #30981, #20215, .T. ) ;
#658=DIRECTION ( 'NONE',  ( 0.000000000000000000, 0.000000000000000000, 1.000000000000000000 ) ) ;
#660=CARTESIAN_POINT ( 'NONE',  ( -1.339745962155613812, 8.794658198738519062, -5.000000000000000000 ) ) ;
#661=CARTESIAN_POINT ( 'NONE',  ( -4.458734124999999437, -4.312499998634401699, 0.000000000000000000 ) ) ;
#662=CARTESIAN_POINT ( 'NONE',  ( 5.000000000000000000, -73.29166666393548724, -2.886751345948130876 ) ) ;
#663=CARTESIAN_POINT ( 'NONE',  ( -1.846868145590737420, -147.7500000013656063, 4.458734124999997661 ) ) ;
#665=ORIENTED_EDGE ( 'NONE', *, *, #42137, .T. ) ;
#667=CARTESIAN_POINT ( 'NONE',  ( -4.999999999999998224, -26.79166666393547658, 2.886751345948131764 ) ) ;
#671=CARTESIAN_POINT ( 'NONE',  ( 2.499999999999998668, 8.791666669397853795, -4.330127018922193649 ) ) ;
#676=CARTESIAN_POINT ( 'NONE',  ( -6.972266317189433020E-16, -90.12499999726880162, -5.000000000000000000 ) ) ;
#678=CARTESIAN_POINT ( 'NONE',  ( -4.458734124999999437, 16.60416666803225993, -2.574251347313719407 ) ) ;
#681=CARTESIAN_POINT ( 'NONE',  ( 2.229367062500001939, -16.22916666530107577, 3.861377020970579999 ) ) ;
#683=CARTESIAN_POINT ( 'NONE',  ( -4.458734124999999437, -162.9375000013655779, -5.460374474430324690E-16 ) ) ;
#684=CARTESIAN_POINT ( 'NONE',  ( -6.972266317189433020E-16, -88.25000000000000000, -5.000000000000000000 ) ) ;
#688=CARTESIAN_POINT ( 'NONE',  ( -5.000000000000000000, -77.00000000000000000, 0.000000000000000000 ) ) ;
#689=CARTESIAN_POINT ( 'NONE',  ( 5.000000000000000888, -142.0625000027312126, -2.071067811865475505 ) ) ;
#690=CARTESIAN_POINT ( 'NONE',  ( -3.152801135295367096, -152.3125000013655779, -3.152801135295367541 ) ) ;
#699=CARTESIAN_POINT ( 'NONE',  ( -3.535250795749689387E-16, -2.250000000000001776, -5.773502691896257311 ) ) ;
#701=CARTESIAN_POINT ( 'NONE',  ( -4.458734124999999437, -65.31249999863440792, 0.000000000000000000 ) ) ;
#702=CARTESIAN_POINT ( 'NONE',  ( -6.972266317189433020E-16, -31.12499999726880873, -5.000000000000000000 ) ) ;
#703=CARTESIAN_POINT ( 'NONE',  ( 5.000000000000000000, -4.374999997268816720, -6.123233995736766282E-16 ) ) ;
#704=CARTESIAN_POINT ( 'NONE',  ( 2.229367062499998831, -36.64583333196773651, -3.861377020970580887 ) ) ;
#705=ORIENTED_EDGE ( 'NONE', *, *, #8739, .F. ) ;
#707=CARTESIAN_POINT ( 'NONE',  ( -6.972266317189433020E-16, 12.75000000000000000, -5.000000000000000000 ) ) ;
#708=ORIENTED_EDGE ( 'NONE', *, *, #40165, .T. ) ;
#710=CARTESIAN_POINT ( 'NONE',  ( 1.060575238724906964E-15, -49.75000000000000000, 5.773502691896257311 ) ) ;
#711=CARTESIAN_POINT ( 'NONE',  ( 2.499999999999998668, -46.20833333060214443, -4.330127018922193649 ) ) ;
#713=CARTESIAN_POINT ( 'NONE',  ( -1.049326080737009628E-13, -4.750000000000003553, 5.000000000000000000 ) ) ;
#714=CARTESIAN_POINT ( 'NONE',  ( -2.229367062499996610, -76.14583333196773651, 3.861377020970582219 ) ) ;
#715=CARTESIAN_POINT ( 'NONE',  ( -4.458734125000000326, -142.2500000013656063, -1.846868145590735644 ) ) ;
#716=CARTESIAN_POINT ( 'NONE',  ( 2.229367062500001939, -82.97916666530106511, 3.861377020970579999 ) ) ;
#719=CARTESIAN_POINT ( 'NONE',  ( -4.458734124999999437, -30.56249999863440436, 0.000000000000000000 ) ) ;
#720=CARTESIAN_POINT ( 'NONE',  ( 2.500000000000002220, -69.54166666393547303, 4.330127018922192761 ) ) ;
#722=DIRECTION ( 'NONE',  ( -0.000000000000000000, 1.000000000000000000, -0.000000000000000000 ) ) ;
#723=ORIENTED_EDGE ( 'NONE', *, *, #22917, .T. ) ;
#725=CARTESIAN_POINT ( 'NONE',  ( 4.458734124999999437, -139.4375000013656063, 0.000000000000000000 ) ) ;
#730=CARTESIAN_POINT ( 'NONE',  ( -2.229367062499996610, -57.39583333196773651, 3.861377020970582219 ) ) ;
#733=VERTEX_POINT ( 'NONE', #1567 ) ;
#734=( BOUNDED_CURVE ( )  B_SPLINE_CURVE ( 2, ( #5253, #25183, #5897, #6215, #53814, #24875, #40300, #44476, #54130 ),
 .UNSPECIFIED., .F., .F. ) 
 B_SPLINE_CURVE_WITH_KNOTS ( ( 3, 2, 2, 2, 3 ),
 ( 0.6249999999999996669, 0.6291666666666663188, 0.6333333333333328596, 0.6374999999999995115, 0.6416666666666662744 ),
 .UNSPECIFIED. ) 
 CURVE ( )  GEOMETRIC_REPRESENTATION_ITEM ( )  RATIONAL_B_SPLINE_CURVE ( ( 1.000000000000005995, 0.9238795325112806323, 1.000000000000000000, 0.9238795325112867385, 1.000000000000000000, 0.9238795325112867385, 1.000000000000000000, 0.9238795325112948431, 0.9999999999999918954 ) ) 
 REPRESENTATION_ITEM ( '' )  );
#735=CARTESIAN_POINT ( 'NONE',  ( -3.535533905932737309, -146.6250000000000000, -3.535533905932738197 ) ) ;
#737=CARTESIAN_POINT ( 'NONE',  ( -4.458734124999999437, 13.68750000136559386, 0.000000000000000000 ) ) ;
#740=CARTESIAN_POINT ( 'NONE',  ( -3.152801135295367985, -162.8125000013656063, 3.152801135295367096 ) ) ;
#741=CARTESIAN_POINT ( 'NONE',  ( 0.000000000000000000, -170.0000000000000000, 5.000000000000000000 ) ) ;
#745=CARTESIAN_POINT ( 'NONE',  ( -6.972266317189433020E-16, -71.12499999726878741, -5.000000000000000000 ) ) ;
#748=EDGE_CURVE ( 'NONE', #5879, #5467, #50758, .T. ) ;
#751=VECTOR ( 'NONE', #62223, 1000.000000000000000 ) ;
#754=CARTESIAN_POINT ( 'NONE',  ( -5.000000000000000000, -21.08333333333333570, -2.886751345948128211 ) ) ;
#755=CARTESIAN_POINT ( 'NONE',  ( 5.000000000000000000, -78.37499999726881583, -6.123233995736766282E-16 ) ) ;
#760=CARTESIAN_POINT ( 'NONE',  ( -3.152548672688508926E-16, 5.187500001365592972, -5.148502694627439702 ) ) ;
#761=CARTESIAN_POINT ( 'NONE',  ( 3.061616997868383141E-16, -145.8750000027312126, -5.000000000000000000 ) ) ;
#763=CARTESIAN_POINT ( 'NONE',  ( 2.071067811865475505, -148.9375000027311842, -5.000000000000000888 ) ) ;
#772=CARTESIAN_POINT ( 'NONE',  ( 4.458734124999997661, -165.7500000013655779, 1.846868145590737864 ) ) ;
#773=LINE ( 'NONE', #20380, #16323 ) ;
#776=CARTESIAN_POINT ( 'NONE',  ( -8.190561711645485556E-16, -142.6875000013656063, 4.458734124999999437 ) ) ;
#777=ORIENTED_EDGE ( 'NONE', *, *, #29470, .F. ) ;
#778=CARTESIAN_POINT ( 'NONE',  ( -3.152548672688508926E-16, 27.18750000136559564, -5.148502694627439702 ) ) ;
#779=ORIENTED_EDGE ( 'NONE', *, *, #28315, .T. ) ;
#780=CARTESIAN_POINT ( 'NONE',  ( -4.458734124999999437, -63.56249999863440792, 0.000000000000000000 ) ) ;
#783=CARTESIAN_POINT ( 'NONE',  ( -2.499999999999996447, 11.16666666666666430, 4.330127018922195425 ) ) ;
#784=CARTESIAN_POINT ( 'NONE',  ( 2.229367062499998831, -48.64583333196772941, -3.861377020970580887 ) ) ;
#785=CARTESIAN_POINT ( 'NONE',  ( -2.229367062499996610, -13.14583333196774007, 3.861377020970582219 ) ) ;
#786=CARTESIAN_POINT ( 'NONE',  ( -5.000000000000000888, -168.5625000000000000, -2.071067811865475949 ) ) ;
#789=CYLINDRICAL_SURFACE ( 'NONE', #24783, 5.000000000000000000 ) ;
#790=FACE_OUTER_BOUND ( 'NONE', #10460, .T. ) ;
#791=( BOUNDED_CURVE ( )  B_SPLINE_CURVE ( 2, ( #30635, #1396, #6523, #20997, #32143, #60247, #35791, #26135, #30955 ),
 .UNSPECIFIED., .F., .F. ) 
 B_SPLINE_CURVE_WITH_KNOTS ( ( 3, 2, 2, 2, 3 ),
 ( 0.8145833333333333259, 0.8152777777777777679, 0.8166666666666666519, 0.8180555555555555358, 0.8187499999999999778 ),
 .UNSPECIFIED. ) 
 CURVE ( )  GEOMETRIC_REPRESENTATION_ITEM ( )  RATIONAL_B_SPLINE_CURVE ( ( 0.9330127018922194093, 0.9330127018922194093, 1.000000000000000000, 0.8660254037844387076, 1.000000000000000000, 0.8660254037844387076, 1.000000000000000000, 0.9330127018922194093, 0.9330127018922194093 ) ) 
 REPRESENTATION_ITEM ( '' )  );
#794=CARTESIAN_POINT ( 'NONE',  ( 3.061616997868383141E-16, -140.8750000027312126, -5.000000000000000000 ) ) ;
#795=CARTESIAN_POINT ( 'NONE',  ( -4.458734124999998549, -52.22916666530106511, 2.574251347313722516 ) ) ;
#796=CARTESIAN_POINT ( 'NONE',  ( -4.458734124999999437, -157.1875000013655779, -5.460374474430324690E-16 ) ) ;
#797=VECTOR ( 'NONE', #12996, 1000.000000000000000 ) ;
#799=CARTESIAN_POINT ( 'NONE',  ( -3.535250795749689387E-16, -56.12499999726880162, -5.773502691896257311 ) ) ;
#802=CARTESIAN_POINT ( 'NONE',  ( 9.457646018065525792E-16, 2.687500001365594304, 5.148502694627439702 ) ) ;
#806=CARTESIAN_POINT ( 'NONE',  ( -4.458734125000001214, -154.8750000013655779, 1.846868145590734089 ) ) ;
#807=ORIENTED_EDGE ( 'NONE', *, *, #51943, .T. ) ;
#808=CARTESIAN_POINT ( 'NONE',  ( 5.000000000000000888, -83.58333333333332860, 2.886751345948126879 ) ) ;
#811=CARTESIAN_POINT ( 'NONE',  ( -4.458734124999999437, -40.56249999863440081, 0.000000000000000000 ) ) ;
#812=EDGE_CURVE ( 'NONE', #28481, #7216, #43781, .T. ) ;
#814=EDGE_CURVE ( 'NONE', #10657, #17293, #229, .T. ) ;
#816=CARTESIAN_POINT ( 'NONE',  ( 1.975475456537005874E-15, 9.375000002731185944, 5.000000000000000000 ) ) ;
#818=CARTESIAN_POINT ( 'NONE',  ( -4.458734124999998549, -89.47916666530106511, 2.574251347313722516 ) ) ;
#820=CARTESIAN_POINT ( 'NONE',  ( -5.000000000000000888, -165.4375000000000284, 2.071067811865474617 ) ) ;
#821=DIRECTION ( 'NONE',  ( 0.000000000000000000, -0.000000000000000000, -1.000000000000000000 ) ) ;
#826=EDGE_CURVE ( 'NONE', #33613, #46845, #17878, .T. ) ;
#827=CARTESIAN_POINT ( 'NONE',  ( -1.339745962155613812, -79.08034179853028434, -5.000000000000000000 ) ) ;
#828=CARTESIAN_POINT ( 'NONE',  ( 3.061616997868383141E-16, -156.8750000027311842, -5.000000000000000000 ) ) ;
#831=CARTESIAN_POINT ( 'NONE',  ( 2.499999999999998668, -42.20833333060214443, -4.330127018922193649 ) ) ;
#833=CARTESIAN_POINT ( 'NONE',  ( 0.000000000000000000, -170.0000000000000000, 5.000000000000000000 ) ) ;
#834=CARTESIAN_POINT ( 'NONE',  ( -3.152548672688508926E-16, -88.81249999863439371, -5.148502694627439702 ) ) ;
#837=ORIENTED_EDGE ( 'NONE', *, *, #19159, .T. ) ;
#838=AXIS2_PLACEMENT_3D ( 'NONE', #60962, #8190, #7248 ) ;
#840=CARTESIAN_POINT ( 'NONE',  ( -2.071067811865470620, -169.3125000000000000, 5.000000000000007105 ) ) ;
#842=CARTESIAN_POINT ( 'NONE',  ( 3.535533905932736864, -162.2500000027312126, 3.535533905932738641 ) ) ;
#843=ORIENTED_EDGE ( 'NONE', *, *, #20028, .F. ) ;
#845=LINE ( 'NONE', #44235, #60304 ) ;
#854=CARTESIAN_POINT ( 'NONE',  ( 9.457646018065525792E-16, -22.06249999863440436, 5.148502694627439702 ) ) ;
#856=CARTESIAN_POINT ( 'NONE',  ( -2.071067811865475061, -156.6875000000000284, -5.000000000000000888 ) ) ;
#858=CARTESIAN_POINT ( 'NONE',  ( -4.458734125000001214, -154.8750000013655779, 1.846868145590734089 ) ) ;
#859=VERTEX_POINT ( 'NONE', #36915 ) ;
#860=CARTESIAN_POINT ( 'NONE',  ( -2.229367062500000163, -44.72916666530106511, -3.861377020970580443 ) ) ;
#861=CARTESIAN_POINT ( 'NONE',  ( -6.972266317189433020E-16, -2.250000000000000000, -5.000000000000000000 ) ) ;
#863=CARTESIAN_POINT ( 'NONE',  ( 4.458734124999998549, -89.72916666530106511, -2.574251347313721627 ) ) ;
#864=CARTESIAN_POINT ( 'NONE',  ( 4.458734124999999437, 12.18750000136559564, -5.460374474430324690E-16 ) ) ;
#868=CARTESIAN_POINT ( 'NONE',  ( 4.458734124999999437, 19.93750000136559208, -5.460374474430324690E-16 ) ) ;
#870=CARTESIAN_POINT ( 'NONE',  ( -5.000000000000000000, 8.041666669397852019, -2.886751345948128211 ) ) ;
#871=VERTEX_POINT ( 'NONE', #17616 ) ;
#872=DIRECTION ( 'NONE',  ( 0.000000000000000000, 0.000000000000000000, 1.000000000000000000 ) ) ;
#875=CARTESIAN_POINT ( 'NONE',  ( 2.229367062500001939, -37.97916666530107221, 3.861377020970579999 ) ) ;
#876=CARTESIAN_POINT ( 'NONE',  ( -2.499999999999996447, -37.70833333060213732, 4.330127018922195425 ) ) ;
#878=CARTESIAN_POINT ( 'NONE',  ( 4.458734124999999437, -12.81249999863440259, -5.460374474430324690E-16 ) ) ;
#879=CARTESIAN_POINT ( 'NONE',  ( -3.152548672688508926E-16, -20.81249999863440081, -5.148502694627439702 ) ) ;
#880=EDGE_LOOP ( 'NONE', ( #32343, #38666, #26508, #29732 ) ) ;
#881=CARTESIAN_POINT ( 'NONE',  ( -2.499999999999996447, -83.83333333333332860, 4.330127018922195425 ) ) ;
#882=CARTESIAN_POINT ( 'NONE',  ( 2.730187237215162345E-16, -167.1875000013655779, -4.458734124999999437 ) ) ;
#884=VECTOR ( 'NONE', #20351, 1000.000000000000000 ) ;
#885=CARTESIAN_POINT ( 'NONE',  ( -5.000000000000000000, -88.95833333060214443, -2.886751345948128211 ) ) ;
#886=CARTESIAN_POINT ( 'NONE',  ( -1.339745962155613812, -49.08034179853029144, -5.000000000000000000 ) ) ;
#887=ORIENTED_EDGE ( 'NONE', *, *, #35445, .T. ) ;
#889=VECTOR ( 'NONE', #11375, 1000.000000000000000 ) ;
#890=CARTESIAN_POINT ( 'NONE',  ( -4.458734124999999437, -25.64583333196773651, -2.574251347313719407 ) ) ;
#891=CARTESIAN_POINT ( 'NONE',  ( 5.000000000000000000, -5.374999997268811391, -6.123233995736766282E-16 ) ) ;
#893=EDGE_CURVE ( 'NONE', #33079, #5936, #31021, .T. ) ;
#894=CARTESIAN_POINT ( 'NONE',  ( 3.152801135295366208, -164.8125000013656063, 3.152801135295367985 ) ) ;
#896=CARTESIAN_POINT ( 'NONE',  ( 5.000000000000000000, -156.0625000000000284, 2.071067811865478614 ) ) ;
#897=VERTEX_POINT ( 'NONE', #11818 ) ;
#899=CARTESIAN_POINT ( 'NONE',  ( -4.458734124999999437, -74.64583333196773651, -2.574251347313719407 ) ) ;
#902=CARTESIAN_POINT ( 'NONE',  ( 2.730187237215162345E-16, -142.4375000013656063, -4.458734124999999437 ) ) ;
#904=DIRECTION ( 'NONE',  ( -0.000000000000000000, 1.000000000000000000, -0.000000000000000000 ) ) ;
#907=ADVANCED_FACE ( 'NONE', ( #28824 ), #9520, .T. ) ;
#912=CARTESIAN_POINT ( 'NONE',  ( 4.458734124999999437, -139.7500000013655779, 1.846868145590737864 ) ) ;
#915=CARTESIAN_POINT ( 'NONE',  ( -4.999999999999998224, -39.79166666393548013, 2.886751345948131764 ) ) ;
#917=CARTESIAN_POINT ( 'NONE',  ( 2.229367062500001939, -74.22916666530106511, 3.861377020970579999 ) ) ;
#919=CARTESIAN_POINT ( 'NONE',  ( -5.000000000000000888, -166.5625000000000000, -2.071067811865475949 ) ) ;
#920=CARTESIAN_POINT ( 'NONE',  ( -2.499999999999996447, -0.7083333306021483144, 4.330127018922195425 ) ) ;
#929=CARTESIAN_POINT ( 'NONE',  ( -1.339745962155660663, -4.794658198738521726, 4.999999999999972466 ) ) ;
#931=CARTESIAN_POINT ( 'NONE',  ( 2.229367062500001939, 18.77083333469892779, 3.861377020970579999 ) ) ;
#940=CARTESIAN_POINT ( 'NONE',  ( 2.229367062500001939, -84.97916666530107932, 3.861377020970579999 ) ) ;
#941=CARTESIAN_POINT ( 'NONE',  ( 4.458734125000000326, -2.895833331967738289, 2.574251347313718519 ) ) ;
#943=CARTESIAN_POINT ( 'NONE',  ( -2.229367062499996610, -30.39583333196773651, 3.861377020970582219 ) ) ;
#949=CARTESIAN_POINT ( 'NONE',  ( -4.458734124999998549, 25.77083333469892779, 2.574251347313722516 ) ) ;
#952=CARTESIAN_POINT ( 'NONE',  ( -3.152548672688508926E-16, -80.81249999863440792, -5.148502694627439702 ) ) ;
#955=CARTESIAN_POINT ( 'NONE',  ( -3.535250795749689387E-16, 21.87500000273118062, -5.773502691896257311 ) ) ;
#957=FACE_OUTER_BOUND ( 'NONE', #20802, .T. ) ;
#959=CARTESIAN_POINT ( 'NONE',  ( 5.000000000000000000, -170.0000000000000000, 0.000000000000000000 ) ) ;
#960=CARTESIAN_POINT ( 'NONE',  ( -2.499999999999996447, -20.83333333333333570, 4.330127018922195425 ) ) ;
#961=CARTESIAN_POINT ( 'NONE',  ( 4.458734124999999437, -20.81249999863440081, -5.460374474430324690E-16 ) ) ;
#962=CARTESIAN_POINT ( 'NONE',  ( -2.229367062499996610, -83.14583333196773651, 3.861377020970582219 ) ) ;
#963=CARTESIAN_POINT ( 'NONE',  ( 2.499999999999998668, -26.20833333060214798, -4.330127018922193649 ) ) ;
#964=CARTESIAN_POINT ( 'NONE',  ( 9.457646018065525792E-16, -52.06249999863440792, 5.148502694627439702 ) ) ;
#965=EDGE_LOOP ( 'NONE', ( #38732, #27924, #12630, #34159 ) ) ;
#966=CARTESIAN_POINT ( 'NONE',  ( 1.339745962155612702, -65.29465819873851729, -5.000000000000000000 ) ) ;
#967=LINE ( 'NONE', #11540, #51850 ) ;
#968=CARTESIAN_POINT ( 'NONE',  ( 9.457646018065525792E-16, -3.312499998634407472, 5.148502694627439702 ) ) ;
#971=CARTESIAN_POINT ( 'NONE',  ( -5.000000000000000000, -65.00000000000000000, 0.000000000000000000 ) ) ;
#972=CARTESIAN_POINT ( 'NONE',  ( 1.846868145590735200, -153.5000000013656063, -4.458734125000000326 ) ) ;
#975=CARTESIAN_POINT ( 'NONE',  ( 2.071067811865475505, -157.8125000000000284, -5.000000000000000888 ) ) ;
#976=CARTESIAN_POINT ( 'NONE',  ( -2.500000000000000444, 10.83333333333333393, -4.330127018922193649 ) ) ;
#978=CARTESIAN_POINT ( 'NONE',  ( 2.229367062499998831, -12.89583333196774007, -3.861377020970580887 ) ) ;
#979=CARTESIAN_POINT ( 'NONE',  ( -2.229367062500000163, -45.72916666530106511, -3.861377020970580443 ) ) ;
#981=CARTESIAN_POINT ( 'NONE',  ( -4.458734124999999437, -145.9375000013656063, -5.460374474430324690E-16 ) ) ;
#983=CARTESIAN_POINT ( 'NONE',  ( -5.000000000000000000, 21.12500000273118417, 0.000000000000000000 ) ) ;
#985=ORIENTED_EDGE ( 'NONE', *, *, #48987, .T. ) ;
#987=CARTESIAN_POINT ( 'NONE',  ( 2.229367062499998831, 28.10416666803225993, -3.861377020970580887 ) ) ;
#989=CARTESIAN_POINT ( 'NONE',  ( 1.975475456537005874E-15, -44.62499999726880162, 5.000000000000000000 ) ) ;
#990=VECTOR ( 'NONE', #31777, 1000.000000000000000 ) ;
#996=CARTESIAN_POINT ( 'NONE',  ( 4.458734124999999437, -7.812499998634405252, -5.460374474430324690E-16 ) ) ;
#998=CARTESIAN_POINT ( 'NONE',  ( 1.846868145590736310, -149.6250000013655779, 4.458734124999997661 ) ) ;
#1005=CARTESIAN_POINT ( 'NONE',  ( 1.339745962155614034, 29.29465819873852084, 5.000000000000000000 ) ) ;
#1012=CARTESIAN_POINT ( 'NONE',  ( -4.458734124999999437, 10.68750000136559386, 0.000000000000000000 ) ) ;
#1015=CARTESIAN_POINT ( 'NONE',  ( -4.458734124999999437, -16.56249999863440436, 0.000000000000000000 ) ) ;
#1017=CARTESIAN_POINT ( 'NONE',  ( 1.846868145590735200, -164.2500000013656063, -4.458734125000000326 ) ) ;
#1026=CARTESIAN_POINT ( 'NONE',  ( -1.846868145590734756, -151.3750000013656063, -4.458734124999999437 ) ) ;
#1028=CARTESIAN_POINT ( 'NONE',  ( -6.972266317189433020E-16, -14.24999999999999822, -5.000000000000000000 ) ) ;
#1029=CARTESIAN_POINT ( 'NONE',  ( 2.499999999999998668, -68.20833333060214443, -4.330127018922193649 ) ) ;
#1030=ORIENTED_EDGE ( 'NONE', *, *, #46844, .F. ) ;
#1035=CARTESIAN_POINT ( 'NONE',  ( -4.999999999999999112, -0.9166666666666664076, 2.886751345948131764 ) ) ;
#1036=CARTESIAN_POINT ( 'NONE',  ( 4.458734125000000326, -66.89583333196773651, 2.574251347313718519 ) ) ;
#1038=CARTESIAN_POINT ( 'NONE',  ( -3.535250795749689387E-16, -6.124999997268812280, -5.773502691896257311 ) ) ;
#1039=CARTESIAN_POINT ( 'NONE',  ( -4.458734124999999437, -33.31249999863440792, 0.000000000000000000 ) ) ;
#1040=VERTEX_POINT ( 'NONE', #58421 ) ;
#1041=DIRECTION ( 'NONE',  ( -0.000000000000000000, 1.000000000000000000, -0.000000000000000000 ) ) ;
#1043=VERTEX_POINT ( 'NONE', #3767 ) ;
#1045=CARTESIAN_POINT ( 'NONE',  ( 1.060575238724906964E-15, -50.75000000000000000, 5.773502691896257311 ) ) ;
#1046=CARTESIAN_POINT ( 'NONE',  ( 2.500000000000002220, -46.54166666393547303, 4.330127018922192761 ) ) ;
#1049=CARTESIAN_POINT ( 'NONE',  ( -3.152548672688508926E-16, -77.56249999863440792, -5.148502694627439702 ) ) ;
#1050=CARTESIAN_POINT ( 'NONE',  ( 3.061616997868383141E-16, -169.7500000000000000, -5.000000000000000000 ) ) ;
#1051=CARTESIAN_POINT ( 'NONE',  ( 4.458734124999998549, -81.72916666530106511, -2.574251347313721627 ) ) ;
#1053=CARTESIAN_POINT ( 'NONE',  ( 4.458734125000001214, -32.14583333196773651, 2.574251347313718519 ) ) ;
#1054=VERTEX_POINT ( 'NONE', #32716 ) ;
#1056=EDGE_LOOP ( 'NONE', ( #41680, #41288, #22154, #18984 ) ) ;
#1059=VERTEX_POINT ( 'NONE', #43302 ) ;
#1061=CARTESIAN_POINT ( 'NONE',  ( -1.339745962155613812, -76.08034179853028434, -5.000000000000000000 ) ) ;
#1062=CARTESIAN_POINT ( 'NONE',  ( -4.458734124999999437, -64.56249999863440792, 0.000000000000000000 ) ) ;
#1065=DIRECTION ( 'NONE',  ( -0.000000000000000000, 1.000000000000000000, -0.000000000000000000 ) ) ;
#1067=CARTESIAN_POINT ( 'NONE',  ( 4.458734124999999437, 8.187500001365595637, -5.460374474430324690E-16 ) ) ;
#1069=VECTOR ( 'NONE', #53193, 1000.000000000000000 ) ;
#1070=CARTESIAN_POINT ( 'NONE',  ( 5.000000000000000000, -32.50000000000000000, -6.123233995736766282E-16 ) ) ;
#1071=CARTESIAN_POINT ( 'NONE',  ( 4.458734124999997661, -162.5000000013655779, 1.846868145590737864 ) ) ;
#1072=DIRECTION ( 'NONE',  ( -0.000000000000000000, 1.000000000000000000, -0.000000000000000000 ) ) ;
#1077=AXIS2_PLACEMENT_3D ( 'NONE', #55433, #5576, #6538 ) ;
#1081=CARTESIAN_POINT ( 'NONE',  ( 6.123233995736766282E-16, -170.0000000000000000, -5.000000000000000000 ) ) ;
#1083=CARTESIAN_POINT ( 'NONE',  ( -3.152548672688508926E-16, 27.43750000136559564, -5.148502694627439702 ) ) ;
#1086=CARTESIAN_POINT ( 'NONE',  ( -2.229367062500000163, 1.270833334698927342, -3.861377020970580443 ) ) ;
#1089=CARTESIAN_POINT ( 'NONE',  ( -2.071067811865475061, -146.8125000027312126, -5.000000000000000888 ) ) ;
#1094=DIRECTION ( 'NONE',  ( -0.000000000000000000, 1.000000000000000000, -0.000000000000000000 ) ) ;
#1095=CARTESIAN_POINT ( 'NONE',  ( 3.535533905932736864, -141.2500000027311842, 3.535533905932738641 ) ) ;
#1097=CARTESIAN_POINT ( 'NONE',  ( -3.152801135295367096, -165.3125000013656063, -3.152801135295367541 ) ) ;
#1098=DIRECTION ( 'NONE',  ( 0.000000000000000000, 0.000000000000000000, 1.000000000000000000 ) ) ;
#1101=CARTESIAN_POINT ( 'NONE',  ( -4.458734125000000326, -140.0000000013655779, -1.846868145590735644 ) ) ;
#1102=EDGE_LOOP ( 'NONE', ( #4070, #49426, #36519, #36845 ) ) ;
#1103=CARTESIAN_POINT ( 'NONE',  ( -3.152548672688508926E-16, 22.18750000136559564, -5.148502694627439702 ) ) ;
#1104=EDGE_LOOP ( 'NONE', ( #30665, #13987, #44017, #23834 ) ) ;
#1105=CARTESIAN_POINT ( 'NONE',  ( -4.458734124999999437, -62.56249999863440792, 0.000000000000000000 ) ) ;
#1107=CARTESIAN_POINT ( 'NONE',  ( 0.000000000000000000, -170.0000000000000000, 5.000000000000000000 ) ) ;
#1108=CARTESIAN_POINT ( 'NONE',  ( -4.999999999999999112, 13.08333333333333037, 2.886751345948131764 ) ) ;
#1109=EDGE_CURVE ( 'NONE', #6571, #34317, #42104, .T. ) ;
#1111=CARTESIAN_POINT ( 'NONE',  ( -3.152548672688508926E-16, -52.56249999863440792, -5.148502694627439702 ) ) ;
#1112=CARTESIAN_POINT ( 'NONE',  ( -4.458734124999999437, -11.39583333196774007, -2.574251347313719407 ) ) ;
#1122=CARTESIAN_POINT ( 'NONE',  ( 2.229367062500001939, -57.97916666530107932, 3.861377020970579999 ) ) ;
#1123=CARTESIAN_POINT ( 'NONE',  ( 4.458734124999999437, -155.6875000013655779, 0.000000000000000000 ) ) ;
#1125=( BOUNDED_CURVE ( )  B_SPLINE_CURVE ( 2, ( #57789, #19152, #62622, #58087, #43595, #52639, #43907, #62303, #18225 ),
 .UNSPECIFIED., .F., .F. ) 
 B_SPLINE_CURVE_WITH_KNOTS ( ( 3, 2, 2, 2, 3 ),
 ( 0.08958333333333333426, 0.09027777777777777624, 0.09166666666666666019, 0.09305555555555555802, 0.09375000000000000000 ),
 .UNSPECIFIED. ) 
 CURVE ( )  GEOMETRIC_REPRESENTATION_ITEM ( )  RATIONAL_B_SPLINE_CURVE ( ( 0.9330127018922194093, 0.9330127018922194093, 1.000000000000000000, 0.8660254037844387076, 1.000000000000000000, 0.8660254037844387076, 1.000000000000000000, 0.9330127018922194093, 0.9330127018922194093 ) ) 
 REPRESENTATION_ITEM ( '' )  );
#1126=EDGE_CURVE ( 'NONE', #45557, #27450, #8856, .T. ) ;
#1127=CARTESIAN_POINT ( 'NONE',  ( 5.000000000000000888, -54.45833333060214443, 2.886751345948126879 ) ) ;
#1128=ORIENTED_EDGE ( 'NONE', *, *, #16124, .F. ) ;
#1129=CARTESIAN_POINT ( 'NONE',  ( 1.339745962155615144, -26.70534180126147561, 4.999999999999999112 ) ) ;
#1130=CARTESIAN_POINT ( 'NONE',  ( 9.457646018065525792E-16, 0.6875000013655957476, 5.148502694627439702 ) ) ;
#1132=VERTEX_POINT ( 'NONE', #57799 ) ;
#1135=CARTESIAN_POINT ( 'NONE',  ( -3.152801135295367096, -156.0625000013656063, -3.152801135295367541 ) ) ;
#1136=ORIENTED_EDGE ( 'NONE', *, *, #27471, .T. ) ;
#1139=CARTESIAN_POINT ( 'NONE',  ( 3.535533905932736864, -161.2500000027312126, 3.535533905932738641 ) ) ;
#1140=CARTESIAN_POINT ( 'NONE',  ( -3.152548672688508926E-16, -46.81249999863440081, -5.148502694627439702 ) ) ;
#1142=CARTESIAN_POINT ( 'NONE',  ( -6.972266317189433020E-16, 11.87500000273118594, -5.000000000000000000 ) ) ;
#1144=CARTESIAN_POINT ( 'NONE',  ( -2.229367062499996610, -89.39583333196773651, 3.861377020970582219 ) ) ;
#1147=CARTESIAN_POINT ( 'NONE',  ( 0.000000000000000000, -170.0000000000000000, 5.000000000000000000 ) ) ;
#1149=CARTESIAN_POINT ( 'NONE',  ( -1.339745962155610925, 1.205341801261479828, 5.000000000000000000 ) ) ;
#1152=CARTESIAN_POINT ( 'NONE',  ( 1.062108568985190270E-13, -27.25000000000000000, -4.999999999999999112 ) ) ;
#1156=CARTESIAN_POINT ( 'NONE',  ( -4.999999999999998224, 25.08333333333333215, 2.886751345948131764 ) ) ;
#1157=CARTESIAN_POINT ( 'NONE',  ( 0.000000000000000000, -170.0000000000000000, 0.000000000000000000 ) ) ;
#1158=CARTESIAN_POINT ( 'NONE',  ( 9.457646018065525792E-16, -89.31249999863440792, 5.148502694627439702 ) ) ;
#1164=CARTESIAN_POINT ( 'NONE',  ( 5.000000000000000000, -157.1875000027312126, 2.071067811865478614 ) ) ;
#1169=CARTESIAN_POINT ( 'NONE',  ( -6.972266317189433020E-16, -67.25000000000000000, -5.000000000000000000 ) ) ;
#1175=FACE_OUTER_BOUND ( 'NONE', #36826, .T. ) ;
#1176=CARTESIAN_POINT ( 'NONE',  ( 4.458734124999998549, -18.72916666530106866, -2.574251347313721627 ) ) ;
#1177=CARTESIAN_POINT ( 'NONE',  ( 3.061616997868383141E-16, -159.7500000000000000, -5.000000000000000000 ) ) ;
#1178=CARTESIAN_POINT ( 'NONE',  ( -9.184850993605147944E-16, -152.2500000000000000, 5.000000000000000000 ) ) ;
#1180=CARTESIAN_POINT ( 'NONE',  ( 4.458734124999999437, -154.4375000013655779, 0.000000000000000000 ) ) ;
#1182=CARTESIAN_POINT ( 'NONE',  ( 4.458734124999999437, -44.06249999863440081, -5.460374474430324690E-16 ) ) ;
#1186=CARTESIAN_POINT ( 'NONE',  ( -2.500000000000000444, 27.83333333333333215, -4.330127018922193649 ) ) ;
#1187=ADVANCED_FACE ( 'NONE', ( #1175 ), #59371, .T. ) ;
#1188=CARTESIAN_POINT ( 'NONE',  ( -4.458734124999999437, 4.687500001365595637, 0.000000000000000000 ) ) ;
#1189=LINE ( 'NONE', #15320, #62683 ) ;
#1192=CARTESIAN_POINT ( 'NONE',  ( -4.458734124999999437, 18.43750000136559564, 0.000000000000000000 ) ) ;
#1194=CARTESIAN_POINT ( 'NONE',  ( 2.500000000000002220, 10.45833333606451987, 4.330127018922192761 ) ) ;
#1198=FACE_OUTER_BOUND ( 'NONE', #16752, .T. ) ;
#1199=CARTESIAN_POINT ( 'NONE',  ( 9.457646018065525792E-16, -44.06249999863439371, 5.148502694627439702 ) ) ;
#1200=EDGE_CURVE ( 'NONE', #32427, #18888, #37599, .T. ) ;
#1201=CARTESIAN_POINT ( 'NONE',  ( 5.000000000000000000, -38.37499999726881583, -6.123233995736766282E-16 ) ) ;
#1203=CARTESIAN_POINT ( 'NONE',  ( 2.229367062500001939, -17.97916666530106866, 3.861377020970579999 ) ) ;
#1206=CARTESIAN_POINT ( 'NONE',  ( -5.000000000000000000, -84.99999999999998579, 0.000000000000000000 ) ) ;
#1207=CARTESIAN_POINT ( 'NONE',  ( -4.458734125000000326, -168.0000000013655779, -1.846868145590735644 ) ) ;
#1209=( BOUNDED_CURVE ( )  B_SPLINE_CURVE ( 2, ( #48764, #28837, #29455, #4709, #5674, #39745, #29142, #58433, #43935 ),
 .UNSPECIFIED., .F., .F. ) 
 B_SPLINE_CURVE_WITH_KNOTS ( ( 3, 2, 2, 2, 3 ),
 ( 0.8229166666666666297, 0.8236111111111110716, 0.8249999999999999556, 0.8263888888888888395, 0.8270833333333332815 ),
 .UNSPECIFIED. ) 
 CURVE ( )  GEOMETRIC_REPRESENTATION_ITEM ( )  RATIONAL_B_SPLINE_CURVE ( ( 0.9330127018922194093, 0.9330127018922194093, 1.000000000000000000, 0.8660254037844387076, 1.000000000000000000, 0.8660254037844387076, 1.000000000000000000, 0.9330127018922194093, 0.9330127018922194093 ) ) 
 REPRESENTATION_ITEM ( '' )  );
#1210=CARTESIAN_POINT ( 'NONE',  ( -5.000000000000000000, -87.87499999726880162, 0.000000000000000000 ) ) ;
#1211=ORIENTED_EDGE ( 'NONE', *, *, #16225, .F. ) ;
#1212=AXIS2_PLACEMENT_3D ( 'NONE', #22676, #47110, #1798 ) ;
#1214=CARTESIAN_POINT ( 'NONE',  ( -4.458734124999998549, -27.47916666530106866, 2.574251347313722516 ) ) ;
#1218=CARTESIAN_POINT ( 'NONE',  ( -1.846868145590737420, -164.0000000013656063, 4.458734124999999437 ) ) ;
#1220=CARTESIAN_POINT ( 'NONE',  ( 0.000000000000000000, -170.0000000000000000, 0.000000000000000000 ) ) ;
#1221=EDGE_LOOP ( 'NONE', ( #11382, #38108, #36799, #29871 ) ) ;
#1222=CARTESIAN_POINT ( 'NONE',  ( -3.535533905932738641, -166.5000000027312126, 3.535533905932737309 ) ) ;
#1224=CARTESIAN_POINT ( 'NONE',  ( 9.457646018065525792E-16, -74.31249999863440792, 5.148502694627439702 ) ) ;
#1227=CARTESIAN_POINT ( 'NONE',  ( 3.152801135295366208, -141.8125000013655779, 3.152801135295367985 ) ) ;
#1238=CARTESIAN_POINT ( 'NONE',  ( -2.229367062500000163, -73.72916666530106511, -3.861377020970580443 ) ) ;
#1239=CYLINDRICAL_SURFACE ( 'NONE', #24015, 5.000000000000000000 ) ;
#1243=CARTESIAN_POINT ( 'NONE',  ( 5.000000000000000000, -146.0625000000000000, 2.071067811865478614 ) ) ;
#1244=CARTESIAN_POINT ( 'NONE',  ( -6.972266317189433020E-16, -60.24999999999999289, -5.000000000000000000 ) ) ;
#1247=CARTESIAN_POINT ( 'NONE',  ( 3.061616997868383141E-16, -167.8750000027312126, -5.000000000000000000 ) ) ;
#1249=CARTESIAN_POINT ( 'NONE',  ( -4.458734124999999437, 16.35416666803225993, -2.574251347313719407 ) ) ;
#1250=CARTESIAN_POINT ( 'NONE',  ( 5.000000000000000888, -77.45833333060213022, 2.886751345948126879 ) ) ;
#1255=CARTESIAN_POINT ( 'NONE',  ( -5.000000000000000000, -50.95833333060213732, -2.886751345948128211 ) ) ;
#1256=CARTESIAN_POINT ( 'NONE',  ( 2.229367062499998831, -85.64583333196773651, -3.861377020970580887 ) ) ;
#1257=CARTESIAN_POINT ( 'NONE',  ( 4.458734124999999437, -1.812499998634406584, -5.460374474430324690E-16 ) ) ;
#1259=CARTESIAN_POINT ( 'NONE',  ( 4.458734124999999437, -32.06249999863440792, -5.460374474430324690E-16 ) ) ;
#1263=CARTESIAN_POINT ( 'NONE',  ( 4.458734124999999437, 19.18750000136559564, -5.460374474430324690E-16 ) ) ;
#1264=EDGE_CURVE ( 'NONE', #13616, #57087, #22019, .T. ) ;
#1267=CARTESIAN_POINT ( 'NONE',  ( 5.000000000000000888, -66.58333333333332860, 2.886751345948126879 ) ) ;
#1268=CARTESIAN_POINT ( 'NONE',  ( -3.152548672688508926E-16, -79.81249999863440792, -5.148502694627439702 ) ) ;
#1270=EDGE_CURVE ( 'NONE', #43575, #17248, #34927, .T. ) ;
#1272=CARTESIAN_POINT ( 'NONE',  ( -5.000000000000000000, 27.04166666939785202, -2.886751345948128211 ) ) ;
#1273=ORIENTED_EDGE ( 'NONE', *, *, #56758, .T. ) ;
#1276=CARTESIAN_POINT ( 'NONE',  ( -5.000000000000000000, -149.5000000000000284, -6.123233995736766282E-16 ) ) ;
#1277=CARTESIAN_POINT ( 'NONE',  ( 5.000000000000000000, -17.41666666666666430, -2.886751345948129988 ) ) ;
#1278=CARTESIAN_POINT ( 'NONE',  ( 4.458734124999998549, -20.72916666530106866, -2.574251347313721627 ) ) ;
#1279=CARTESIAN_POINT ( 'NONE',  ( 4.458734125000000326, -87.89583333196773651, 2.574251347313718519 ) ) ;
#1280=EDGE_CURVE ( 'NONE', #51312, #21022, #35166, .T. ) ;
#1281=CARTESIAN_POINT ( 'NONE',  ( 1.060575238724906964E-15, -22.62499999726881228, 5.773502691896257311 ) ) ;
#1282=CARTESIAN_POINT ( 'NONE',  ( -2.229367062500000163, -57.47916666530107932, -3.861377020970580443 ) ) ;
#1283=ORIENTED_EDGE ( 'NONE', *, *, #51078, .F. ) ;
#1284=CARTESIAN_POINT ( 'NONE',  ( 1.339745962155612702, -49.29465819873851018, -5.000000000000000000 ) ) ;
#1285=FACE_OUTER_BOUND ( 'NONE', #43628, .T. ) ;
#1287=CARTESIAN_POINT ( 'NONE',  ( -4.458734124999999437, -2.645833331967737845, -2.574251347313719407 ) ) ;
#1288=ORIENTED_EDGE ( 'NONE', *, *, #28159, .F. ) ;
#1290=CARTESIAN_POINT ( 'NONE',  ( 5.000000000000000000, -68.49999999999998579, -6.123233995736766282E-16 ) ) ;
#1292=CARTESIAN_POINT ( 'NONE',  ( 3.152801135295367541, -151.5625000013655779, -3.152801135295367541 ) ) ;
#1295=CARTESIAN_POINT ( 'NONE',  ( -9.184850993605147944E-16, -158.2500000000000000, 5.000000000000000000 ) ) ;
#1298=CARTESIAN_POINT ( 'NONE',  ( -6.972266317189433020E-16, 6.875000002731185944, -5.000000000000000000 ) ) ;
#1300=CARTESIAN_POINT ( 'NONE',  ( -4.458734124999999437, -12.64583333196774007, -2.574251347313719407 ) ) ;
#1301=CARTESIAN_POINT ( 'NONE',  ( -2.229367062499996610, -52.39583333196773651, 3.861377020970582219 ) ) ;
#1302=CARTESIAN_POINT ( 'NONE',  ( 1.975475456537005874E-15, 10.24999999999999822, 5.000000000000000000 ) ) ;
#1303=CARTESIAN_POINT ( 'NONE',  ( -4.458734124999999437, -143.9375000013656063, -5.460374474430324690E-16 ) ) ;
#1305=CARTESIAN_POINT ( 'NONE',  ( 2.626220312808019583E-14, 20.87500000273118062, -5.000000000000000000 ) ) ;
#1306=ORIENTED_EDGE ( 'NONE', *, *, #59063, .T. ) ;
#1308=CARTESIAN_POINT ( 'NONE',  ( 2.229367062499998831, 27.10416666803225993, -3.861377020970580887 ) ) ;
#1313=( BOUNDED_CURVE ( )  B_SPLINE_CURVE ( 2, ( #50711, #6343, #25950, #564, #5379, #44604, #21127, #6654, #26260 ),
 .UNSPECIFIED., .F., .F. ) 
 B_SPLINE_CURVE_WITH_KNOTS ( ( 3, 2, 2, 2, 3 ),
 ( 0.4937500000000000222, 0.4944444444444444642, 0.4958333333333333481, 0.4972222222222222321, 0.4979166666666666741 ),
 .UNSPECIFIED. ) 
 CURVE ( )  GEOMETRIC_REPRESENTATION_ITEM ( )  RATIONAL_B_SPLINE_CURVE ( ( 0.9330127018922194093, 0.9330127018922194093, 1.000000000000000000, 0.8660254037844387076, 1.000000000000000000, 0.8660254037844387076, 1.000000000000000000, 0.9330127018922194093, 0.9330127018922194093 ) ) 
 REPRESENTATION_ITEM ( '' )  );
#1316=CARTESIAN_POINT ( 'NONE',  ( -5.000000000000000000, 2.041666669397854239, -2.886751345948128211 ) ) ;
#1317=CARTESIAN_POINT ( 'NONE',  ( 2.229367062500001939, -7.979166665301073991, 3.861377020970579999 ) ) ;
#1319=CARTESIAN_POINT ( 'NONE',  ( -3.152801135295367096, -148.0625000013655779, -3.152801135295367541 ) ) ;
#1329=FACE_OUTER_BOUND ( 'NONE', #38194, .T. ) ;
#1333=CARTESIAN_POINT ( 'NONE',  ( -2.229367062499996610, 9.854166668032261711, 3.861377020970582219 ) ) ;
#1335=CARTESIAN_POINT ( 'NONE',  ( -3.152548672688508926E-16, -14.81249999863440436, -5.148502694627439702 ) ) ;
#1337=CARTESIAN_POINT ( 'NONE',  ( 4.458734124999999437, -165.5000000013655779, 1.846868145590737864 ) ) ;
#1342=CARTESIAN_POINT ( 'NONE',  ( -2.499999999999996447, -54.70833333060213732, 4.330127018922195425 ) ) ;
#1343=CARTESIAN_POINT ( 'NONE',  ( 5.000000000000000000, -69.41666666666667140, -2.886751345948130876 ) ) ;
#1345=CARTESIAN_POINT ( 'NONE',  ( 4.458734124999999437, -150.6250000013655779, -1.846868145590734978 ) ) ;
#1347=CARTESIAN_POINT ( 'NONE',  ( -1.339745962155613812, -58.08034179853029144, -5.000000000000000000 ) ) ;
#1352=DIRECTION ( 'NONE',  ( -0.000000000000000000, 1.000000000000000000, -0.000000000000000000 ) ) ;
#1353=CARTESIAN_POINT ( 'NONE',  ( 5.000000000000000000, -1.416666666666663188, -2.886751345948129988 ) ) ;
#1354=CARTESIAN_POINT ( 'NONE',  ( 2.229367062499998831, -66.64583333196773651, -3.861377020970580887 ) ) ;
#1355=CARTESIAN_POINT ( 'NONE',  ( 0.000000000000000000, -170.0000000000000000, 0.000000000000000000 ) ) ;
#1356=CARTESIAN_POINT ( 'NONE',  ( -3.535250795749689387E-16, -10.12499999726881583, -5.773502691896257311 ) ) ;
#1357=CARTESIAN_POINT ( 'NONE',  ( 4.458734125000001214, -41.89583333196773651, 2.574251347313718519 ) ) ;
#1361=CARTESIAN_POINT ( 'NONE',  ( 4.458734125000001214, 11.85416666803225993, 2.574251347313718519 ) ) ;
#1362=EDGE_LOOP ( 'NONE', ( #6334, #6963, #51446, #31577 ) ) ;
#1365=CARTESIAN_POINT ( 'NONE',  ( 2.499999999999998668, -51.33333333333332860, -4.330127018922193649 ) ) ;
#1366=EDGE_CURVE ( 'NONE', #4014, #25951, #44155, .T. ) ;
#1368=CARTESIAN_POINT ( 'NONE',  ( 4.458734124999999437, -77.81249999863440792, -5.460374474430324690E-16 ) ) ;
#1369=CARTESIAN_POINT ( 'NONE',  ( -4.458734125000000326, -140.2500000013656063, -1.846868145590735644 ) ) ;
#1371=CARTESIAN_POINT ( 'NONE',  ( 4.458734125000001214, -80.89583333196773651, 2.574251347313718519 ) ) ;
#1373=CARTESIAN_POINT ( 'NONE',  ( 9.457646018065525792E-16, -35.31249999863440792, 5.148502694627439702 ) ) ;
#1375=EDGE_LOOP ( 'NONE', ( #54448, #15901, #4722, #27782 ) ) ;
#1376=CARTESIAN_POINT ( 'NONE',  ( -6.972266317189433020E-16, -51.25000000000000000, -5.000000000000000000 ) ) ;
#1380=ORIENTED_EDGE ( 'NONE', *, *, #33927, .T. ) ;
#1382=CARTESIAN_POINT ( 'NONE',  ( 1.062108568985190270E-13, -12.25000000000000000, -4.999999999999999112 ) ) ;
#1383=CARTESIAN_POINT ( 'NONE',  ( 9.457646018065525792E-16, -64.31249999863440792, 5.148502694627439702 ) ) ;
#1387=CARTESIAN_POINT ( 'NONE',  ( 9.457646018065525792E-16, 8.937500001365597413, 5.148502694627439702 ) ) ;
#1390=CARTESIAN_POINT ( 'NONE',  ( 4.458734124999999437, -161.4375000013655779, 0.000000000000000000 ) ) ;
#1396=CARTESIAN_POINT ( 'NONE',  ( -1.339745962155610925, -67.79465819873851729, 5.000000000000000000 ) ) ;
#1399=CARTESIAN_POINT ( 'NONE',  ( 1.975475456537005874E-15, -84.74999999999998579, 5.000000000000000000 ) ) ;
#1401=CARTESIAN_POINT ( 'NONE',  ( -1.339745962155613812, -83.08034179853028434, -5.000000000000000000 ) ) ;
#1402=CARTESIAN_POINT ( 'NONE',  ( 4.458734124999998549, 27.27083333469892779, -2.574251347313721627 ) ) ;
#1405=CARTESIAN_POINT ( 'NONE',  ( -4.458734124999999437, 0.3541666680322609340, -2.574251347313719407 ) ) ;
#1406=( BOUNDED_CURVE ( )  B_SPLINE_CURVE ( 2, ( #52966, #58106, #14034, #52656, #24010, #3774, #23397, #57805, #57502 ),
 .UNSPECIFIED., .F., .F. ) 
 B_SPLINE_CURVE_WITH_KNOTS ( ( 3, 2, 2, 2, 3 ),
 ( 0.8937500000000000444, 0.8944444444444444864, 0.8958333333333333703, 0.8972222222222222543, 0.8979166666666666963 ),
 .UNSPECIFIED. ) 
 CURVE ( )  GEOMETRIC_REPRESENTATION_ITEM ( )  RATIONAL_B_SPLINE_CURVE ( ( 0.9330127018922194093, 0.9330127018922194093, 1.000000000000000000, 0.8660254037844387076, 1.000000000000000000, 0.8660254037844387076, 1.000000000000000000, 0.9330127018922194093, 0.9330127018922194093 ) ) 
 REPRESENTATION_ITEM ( '' )  );
#1409=CARTESIAN_POINT ( 'NONE',  ( 5.000000000000000000, -144.1250000027312126, 0.000000000000000000 ) ) ;
#1414=AXIS2_PLACEMENT_3D ( 'NONE', #47704, #53165, #3658 ) ;
#1415=DIRECTION ( 'NONE',  ( 0.000000000000000000, 0.000000000000000000, 1.000000000000000000 ) ) ;
#1419=CARTESIAN_POINT ( 'NONE',  ( 4.458734124999999437, -161.6875000013655779, 0.000000000000000000 ) ) ;
#1420=CARTESIAN_POINT ( 'NONE',  ( 5.000000000000000888, 7.416666666666665186, 2.886751345948126879 ) ) ;
#1424=CARTESIAN_POINT ( 'NONE',  ( -4.458734124999998549, 24.52083333469892779, 2.574251347313722516 ) ) ;
#1426=CARTESIAN_POINT ( 'NONE',  ( 9.457646018065525792E-16, -60.31249999863441502, 5.148502694627439702 ) ) ;
#1429=CARTESIAN_POINT ( 'NONE',  ( -5.000000000000000000, 13.00000000000000178, 0.000000000000000000 ) ) ;
#1430=CARTESIAN_POINT ( 'NONE',  ( 4.458734124999998549, -52.72916666530107221, -2.574251347313721627 ) ) ;
#1431=CARTESIAN_POINT ( 'NONE',  ( 4.458734125000001214, -11.89583333196774007, 2.574251347313718519 ) ) ;
#1433=CARTESIAN_POINT ( 'NONE',  ( -4.999999999999998224, 14.08333333333333393, 2.886751345948131764 ) ) ;
#1434=CARTESIAN_POINT ( 'NONE',  ( -1.339745962155613812, -64.20534180126146850, -5.000000000000000000 ) ) ;
#1435=CARTESIAN_POINT ( 'NONE',  ( -1.510657702057710340E-15, 27.37500000273118417, 5.000000000000000000 ) ) ;
#1436=CARTESIAN_POINT ( 'NONE',  ( -4.999999999999999112, -32.91666666666666430, 2.886751345948131764 ) ) ;
#1437=CARTESIAN_POINT ( 'NONE',  ( -1.339745962155613812, -34.20534180126147561, -5.000000000000000000 ) ) ;
#1439=CARTESIAN_POINT ( 'NONE',  ( -2.499999999999996447, -31.70833333060214798, 4.330127018922195425 ) ) ;
#1440=CARTESIAN_POINT ( 'NONE',  ( 2.229367062500001939, -60.97916666530106511, 3.861377020970579999 ) ) ;
#1441=CARTESIAN_POINT ( 'NONE',  ( 4.458734125000000326, -152.6250000013655495, -1.846868145590734978 ) ) ;
#1442=CARTESIAN_POINT ( 'NONE',  ( -4.458734124999999437, -65.39583333196773651, -2.574251347313719407 ) ) ;
#1443=CARTESIAN_POINT ( 'NONE',  ( -5.000000000000000000, -56.87499999726880162, 0.000000000000000000 ) ) ;
#1447=CARTESIAN_POINT ( 'NONE',  ( 4.458734124999998549, 1.020833334698927120, -2.574251347313721627 ) ) ;
#1448=VERTEX_POINT ( 'NONE', #61609 ) ;
#1450=CARTESIAN_POINT ( 'NONE',  ( -4.458734125000001214, -152.8750000013655779, 1.846868145590734089 ) ) ;
#1454=CARTESIAN_POINT ( 'NONE',  ( 5.000000000000000000, -161.1250000027311842, 0.000000000000000000 ) ) ;
#1455=CARTESIAN_POINT ( 'NONE',  ( -3.152548672688508926E-16, -47.81249999863440792, -5.148502694627439702 ) ) ;
#1460=CARTESIAN_POINT ( 'NONE',  ( 2.229367062500001939, 25.02083333469892779, 3.861377020970579999 ) ) ;
#1463=ORIENTED_EDGE ( 'NONE', *, *, #60243, .T. ) ;
#1465=CARTESIAN_POINT ( 'NONE',  ( 5.000000000000000000, -28.29166666393548013, -2.886751345948130876 ) ) ;
#1471=FACE_OUTER_BOUND ( 'NONE', #14492, .T. ) ;
#1473=CARTESIAN_POINT ( 'NONE',  ( 1.975475456537005874E-15, -87.75000000000001421, 5.000000000000000000 ) ) ;
#1474=CARTESIAN_POINT ( 'NONE',  ( -4.999999999999998224, 11.20833333606451809, 2.886751345948131764 ) ) ;
#1478=CARTESIAN_POINT ( 'NONE',  ( 3.535533905932738197, -156.0000000027312126, -3.535533905932738197 ) ) ;
#1479=ORIENTED_EDGE ( 'NONE', *, *, #11487, .T. ) ;
#1483=( BOUNDED_CURVE ( )  B_SPLINE_CURVE ( 2, ( #2069, #2377, #40642, #40955, #16522, #35830, #56083, #11368, #11053 ),
 .UNSPECIFIED., .F., .F. ) 
 B_SPLINE_CURVE_WITH_KNOTS ( ( 3, 2, 2, 2, 3 ),
 ( 0.5562500000000000222, 0.5569444444444444642, 0.5583333333333333481, 0.5597222222222222321, 0.5604166666666666741 ),
 .UNSPECIFIED. ) 
 CURVE ( )  GEOMETRIC_REPRESENTATION_ITEM ( )  RATIONAL_B_SPLINE_CURVE ( ( 0.9330127018922194093, 0.9330127018922194093, 1.000000000000000000, 0.8660254037844387076, 1.000000000000000000, 0.8660254037844387076, 1.000000000000000000, 0.9330127018922194093, 0.9330127018922194093 ) ) 
 REPRESENTATION_ITEM ( '' )  );
#1489=CARTESIAN_POINT ( 'NONE',  ( -2.229367062499996610, -19.14583333196774007, 3.861377020970582219 ) ) ;
#1490=CARTESIAN_POINT ( 'NONE',  ( -4.999999999999998224, -79.79166666393545881, 2.886751345948131764 ) ) ;
#1491=CARTESIAN_POINT ( 'NONE',  ( -2.071067811865475061, -150.6875000000000284, -5.000000000000000888 ) ) ;
#1493=CARTESIAN_POINT ( 'NONE',  ( -8.190561711645485556E-16, -153.6875000013656063, 4.458734124999999437 ) ) ;
#1495=CARTESIAN_POINT ( 'NONE',  ( 4.458734124999998549, -46.97916666530106511, -2.574251347313721627 ) ) ;
#1498=CARTESIAN_POINT ( 'NONE',  ( 4.458734125000001214, -88.89583333196773651, 2.574251347313718519 ) ) ;
#1500=CARTESIAN_POINT ( 'NONE',  ( 2.229367062500001939, 6.020833334698927786, 3.861377020970579999 ) ) ;
#1504=CARTESIAN_POINT ( 'NONE',  ( -4.458734124999999437, 13.35416666803225993, -2.574251347313719407 ) ) ;
#1506=CARTESIAN_POINT ( 'NONE',  ( -4.999999999999999112, 8.208333336064518093, 2.886751345948131764 ) ) ;
#1509=ORIENTED_EDGE ( 'NONE', *, *, #41308, .F. ) ;
#1510=CARTESIAN_POINT ( 'NONE',  ( 4.458734124999998549, -43.72916666530106511, -2.574251347313721627 ) ) ;
#1511=CARTESIAN_POINT ( 'NONE',  ( -8.190561711645485556E-16, -162.9375000013655779, 4.458734124999999437 ) ) ;
#1512=CARTESIAN_POINT ( 'NONE',  ( 2.499999999999998668, -39.20833333060214443, -4.330127018922193649 ) ) ;
#1513=VERTEX_POINT ( 'NONE', #57726 ) ;
#1514=CARTESIAN_POINT ( 'NONE',  ( 9.457646018065525792E-16, -16.06249999863440436, 5.148502694627439702 ) ) ;
#1515=ORIENTED_EDGE ( 'NONE', *, *, #26383, .T. ) ;
#1516=CARTESIAN_POINT ( 'NONE',  ( -4.999999999999999112, -89.91666666666665719, 2.886751345948131764 ) ) ;
#1517=CARTESIAN_POINT ( 'NONE',  ( 0.000000000000000000, -170.0000000000000000, 0.000000000000000000 ) ) ;
#1518=CARTESIAN_POINT ( 'NONE',  ( 5.000000000000000888, -87.45833333060214443, 2.886751345948126879 ) ) ;
#1519=CARTESIAN_POINT ( 'NONE',  ( -2.499999999999996447, -18.83333333333333215, 4.330127018922195425 ) ) ;
#1520=ORIENTED_EDGE ( 'NONE', *, *, #31152, .F. ) ;
#1522=CARTESIAN_POINT ( 'NONE',  ( 2.229367062499998831, -34.89583333196772941, -3.861377020970580887 ) ) ;
#1529=EDGE_LOOP ( 'NONE', ( #40093, #8346, #38892, #9831 ) ) ;
#1531=CARTESIAN_POINT ( 'NONE',  ( -4.458734124999999437, -81.56249999863440792, 0.000000000000000000 ) ) ;
#1534=CARTESIAN_POINT ( 'NONE',  ( -3.152801135295367096, -140.3125000013655779, -3.152801135295367541 ) ) ;
#1535=CARTESIAN_POINT ( 'NONE',  ( -5.000000000000000000, -57.99999999999999289, 0.000000000000000000 ) ) ;
#1537=CARTESIAN_POINT ( 'NONE',  ( 4.458734124999999437, -46.81249999863440792, -5.460374474430324690E-16 ) ) ;
#1538=CARTESIAN_POINT ( 'NONE',  ( -5.000000000000000000, 27.99999999999999645, 0.000000000000000000 ) ) ;
#1539=EDGE_CURVE ( 'NONE', #33853, #57375, #6812, .T. ) ;
#1543=CARTESIAN_POINT ( 'NONE',  ( -3.152801135295367985, -141.0625000013655779, 3.152801135295367096 ) ) ;
#1546=CARTESIAN_POINT ( 'NONE',  ( -1.339745962155610925, -39.66965819600733312, 5.000000000000000000 ) ) ;
#1548=CARTESIAN_POINT ( 'NONE',  ( 2.229367062500001939, -73.22916666530107932, 3.861377020970579999 ) ) ;
#1552=( BOUNDED_CURVE ( )  B_SPLINE_CURVE ( 2, ( #55304, #966, #2234, #25706, #40173, #6413, #15733, #59811, #26023 ),
 .UNSPECIFIED., .F., .F. ) 
 B_SPLINE_CURVE_WITH_KNOTS ( ( 3, 2, 2, 2, 3 ),
 ( 0.7937499999999999556, 0.7944444444444443976, 0.7958333333333332815, 0.7972222222222222765, 0.7979166666666667185 ),
 .UNSPECIFIED. ) 
 CURVE ( )  GEOMETRIC_REPRESENTATION_ITEM ( )  RATIONAL_B_SPLINE_CURVE ( ( 0.9330127018922194093, 0.9330127018922194093, 1.000000000000000000, 0.8660254037844387076, 1.000000000000000000, 0.8660254037844387076, 1.000000000000000000, 0.9330127018922194093, 0.9330127018922194093 ) ) 
 REPRESENTATION_ITEM ( '' )  );
#1558=CARTESIAN_POINT ( 'NONE',  ( -2.071067811865478170, -168.4375000027311842, 5.000000000000000000 ) ) ;
#1560=CARTESIAN_POINT ( 'NONE',  ( -2.229367062500000163, 15.27083333469892779, -3.861377020970580443 ) ) ;
#1565=EDGE_CURVE ( 'NONE', #60372, #41751, #41724, .T. ) ;
#1567=CARTESIAN_POINT ( 'NONE',  ( 1.975475456537005874E-15, -36.75000000000000000, 5.000000000000000000 ) ) ;
#1568=CARTESIAN_POINT ( 'NONE',  ( 4.458734124999998549, -83.72916666530107932, -2.574251347313721627 ) ) ;
#1569=CARTESIAN_POINT ( 'NONE',  ( -4.458734124999997661, -5.229166665301072214, 2.574251347313722516 ) ) ;
#1572=CARTESIAN_POINT ( 'NONE',  ( 2.229367062500001939, -28.22916666530107221, 3.861377020970579999 ) ) ;
#1576=EDGE_CURVE ( 'NONE', #45853, #42676, #57102, .T. ) ;
#1577=CARTESIAN_POINT ( 'NONE',  ( 4.458734125000001214, 22.10416666803225993, 2.574251347313718519 ) ) ;
#1578=CARTESIAN_POINT ( 'NONE',  ( -6.972266317189433020E-16, -53.24999999999999289, -5.000000000000000000 ) ) ;
#1579=CARTESIAN_POINT ( 'NONE',  ( 2.500000000000002220, -66.66666666666667140, 4.330127018922192761 ) ) ;
#1580=CARTESIAN_POINT ( 'NONE',  ( -2.229367062499996610, -77.39583333196773651, 3.861377020970582219 ) ) ;
#1583=CARTESIAN_POINT ( 'NONE',  ( 2.499999999999998668, 22.79166666939785202, -4.330127018922193649 ) ) ;
#1584=ORIENTED_EDGE ( 'NONE', *, *, #1635, .F. ) ;
#1585=CARTESIAN_POINT ( 'NONE',  ( -4.999999999999998224, -65.91666666666667140, 2.886751345948131764 ) ) ;
#1586=( BOUNDED_CURVE ( )  B_SPLINE_CURVE ( 2, ( #2293, #46016, #61144, #50530, #41813, #21580, #17392, #61460, #40862 ),
 .UNSPECIFIED., .F., .F. ) 
 B_SPLINE_CURVE_WITH_KNOTS ( ( 3, 2, 2, 2, 3 ),
 ( 0.7520833333333333259, 0.7527777777777777679, 0.7541666666666666519, 0.7555555555555555358, 0.7562499999999999778 ),
 .UNSPECIFIED. ) 
 CURVE ( )  GEOMETRIC_REPRESENTATION_ITEM ( )  RATIONAL_B_SPLINE_CURVE ( ( 0.9330127018922194093, 0.9330127018922194093, 1.000000000000000000, 0.8660254037844387076, 1.000000000000000000, 0.8660254037844387076, 1.000000000000000000, 0.9330127018922194093, 0.9330127018922194093 ) ) 
 REPRESENTATION_ITEM ( '' )  );
#1587=CARTESIAN_POINT ( 'NONE',  ( 0.000000000000000000, -170.0000000000000000, 5.000000000000000000 ) ) ;
#1589=CARTESIAN_POINT ( 'NONE',  ( 5.000000000000000000, -24.41666666666666430, -2.886751345948129988 ) ) ;
#1590=CARTESIAN_POINT ( 'NONE',  ( -4.458734124999999437, -25.31249999863440792, 0.000000000000000000 ) ) ;
#1593=CARTESIAN_POINT ( 'NONE',  ( 1.060575238724906964E-15, -21.62499999726881228, 5.773502691896257311 ) ) ;
#1594=EDGE_CURVE ( 'NONE', #1054, #5665, #13371, .T. ) ;
#1595=CARTESIAN_POINT ( 'NONE',  ( 4.458734124999999437, -53.81249999863439371, -5.460374474430324690E-16 ) ) ;
#1596=VERTEX_POINT ( 'NONE', #46851 ) ;
#1599=CARTESIAN_POINT ( 'NONE',  ( 4.458734124999998549, -1.979166665301068662, -2.574251347313721627 ) ) ;
#1600=ORIENTED_EDGE ( 'NONE', *, *, #34157, .F. ) ;
#1601=CARTESIAN_POINT ( 'NONE',  ( 5.000000000000000000, -70.50000000000000000, -6.123233995736766282E-16 ) ) ;
#1602=CARTESIAN_POINT ( 'NONE',  ( -3.152801135295367096, -151.3125000013655779, -3.152801135295367541 ) ) ;
#1604=CARTESIAN_POINT ( 'NONE',  ( -6.972266317189433020E-16, -78.12499999726881583, -5.000000000000000000 ) ) ;
#1605=CARTESIAN_POINT ( 'NONE',  ( -5.000000000000000000, -157.5000000000000000, -6.123233995736766282E-16 ) ) ;
#1608=CARTESIAN_POINT ( 'NONE',  ( -2.229367062499996610, -16.39583333196773651, 3.861377020970582219 ) ) ;
#1609=CARTESIAN_POINT ( 'NONE',  ( 4.458734125000001214, -52.14583333196772941, 2.574251347313718519 ) ) ;
#1611=CARTESIAN_POINT ( 'NONE',  ( -3.152801135295367096, -146.0625000013655779, -3.152801135295367541 ) ) ;
#1614=ORIENTED_EDGE ( 'NONE', *, *, #46136, .T. ) ;
#1615=CARTESIAN_POINT ( 'NONE',  ( -5.000000000000000000, -155.5000000000000000, -6.123233995736766282E-16 ) ) ;
#1616=CARTESIAN_POINT ( 'NONE',  ( -4.458734124999998549, 24.52083333469892779, 2.574251347313722516 ) ) ;
#1618=FACE_OUTER_BOUND ( 'NONE', #51809, .T. ) ;
#1621=ADVANCED_FACE ( 'NONE', ( #12750 ), #57773, .T. ) ;
#1623=CARTESIAN_POINT ( 'NONE',  ( 1.339745962155612702, -19.29465819873851729, -5.000000000000000000 ) ) ;
#1625=CARTESIAN_POINT ( 'NONE',  ( -1.339745962155610925, 9.205341801261479162, 5.000000000000000000 ) ) ;
#1626=CARTESIAN_POINT ( 'NONE',  ( 4.458734124999998549, -8.729166665301073991, -2.574251347313721627 ) ) ;
#1628=CARTESIAN_POINT ( 'NONE',  ( 1.846868145590735200, -148.2500000013656347, -4.458734124999999437 ) ) ;
#1631=CARTESIAN_POINT ( 'NONE',  ( -3.535533905932738641, -148.3750000000000000, 3.535533905932737309 ) ) ;
#1634=CARTESIAN_POINT ( 'NONE',  ( 2.499999999999998668, -85.20833333060214443, -4.330127018922193649 ) ) ;
#1635=EDGE_CURVE ( 'NONE', #41425, #23654, #2314, .T. ) ;
#1636=CARTESIAN_POINT ( 'NONE',  ( -1.127183054612291972E-14, 25.24999999999999645, 4.999999999999999112 ) ) ;
#1642=EDGE_CURVE ( 'NONE', #54415, #51386, #19932, .T. ) ;
#1643=FACE_OUTER_BOUND ( 'NONE', #58770, .T. ) ;
#1644=CARTESIAN_POINT ( 'NONE',  ( 4.458734125000000326, 12.10416666803226171, 2.574251347313718519 ) ) ;
#1646=CARTESIAN_POINT ( 'NONE',  ( -4.458734124999999437, -11.64583333196774184, -2.574251347313719407 ) ) ;
#1648=CARTESIAN_POINT ( 'NONE',  ( -3.152801135295367096, -165.0625000013656063, -3.152801135295367541 ) ) ;
#1649=CARTESIAN_POINT ( 'NONE',  ( 1.255007937094098239E-14, 23.75000000000000000, -4.999999999999999112 ) ) ;
#1652=CARTESIAN_POINT ( 'NONE',  ( -1.339745962155613812, -77.20534180126145429, -5.000000000000000000 ) ) ;
#1655=CARTESIAN_POINT ( 'NONE',  ( 4.458734124999999437, -33.81249999863440792, -5.460374474430324690E-16 ) ) ;
#1656=CARTESIAN_POINT ( 'NONE',  ( 1.339745962155612702, -51.16965819600732601, -5.000000000000000000 ) ) ;
#1658=CARTESIAN_POINT ( 'NONE',  ( -4.999999999999998224, -13.91666666666666785, 2.886751345948131764 ) ) ;
#1664=CARTESIAN_POINT ( 'NONE',  ( 2.499999999999998668, -9.333333333333332149, -4.330127018922193649 ) ) ;
#1665=CARTESIAN_POINT ( 'NONE',  ( -2.229367062499996610, -73.14583333196773651, 3.861377020970582219 ) ) ;
#1667=CARTESIAN_POINT ( 'NONE',  ( 2.499999999999998668, -5.208333330602148870, -4.330127018922193649 ) ) ;
#1668=CARTESIAN_POINT ( 'NONE',  ( -2.229367062499996610, -39.14583333196773651, 3.861377020970582219 ) ) ;
#1669=ORIENTED_EDGE ( 'NONE', *, *, #62930, .T. ) ;
#1671=CARTESIAN_POINT ( 'NONE',  ( -4.458734124999999437, 11.35416666803225993, -2.574251347313719407 ) ) ;
#1672=ORIENTED_EDGE ( 'NONE', *, *, #13075, .F. ) ;
#1674=CARTESIAN_POINT ( 'NONE',  ( -5.000000000000000000, -50.00000000000000000, 0.000000000000000000 ) ) ;
#1676=CARTESIAN_POINT ( 'NONE',  ( 3.061616997868383141E-16, -157.7500000000000000, -5.000000000000000000 ) ) ;
#1677=CARTESIAN_POINT ( 'NONE',  ( 4.458734124999999437, -76.81249999863440792, -5.460374474430324690E-16 ) ) ;
#1678=CARTESIAN_POINT ( 'NONE',  ( 3.535533905932736864, -169.1250000000000284, 3.535533905932738641 ) ) ;
#1679=CARTESIAN_POINT ( 'NONE',  ( 9.457646018065525792E-16, -85.06249999863440792, 5.148502694627439702 ) ) ;
#1682=AXIS2_PLACEMENT_3D ( 'NONE', #16414, #13167, #22837 ) ;
#1683=CARTESIAN_POINT ( 'NONE',  ( -4.458734124999999437, -37.64583333196773651, -2.574251347313719407 ) ) ;
#1684=( BOUNDED_CURVE ( )  B_SPLINE_CURVE ( 2, ( #47397, #62205, #11707, #36481, #17177, #18121, #7537, #56747, #12671 ),
 .UNSPECIFIED., .F., .F. ) 
 B_SPLINE_CURVE_WITH_KNOTS ( ( 3, 2, 2, 2, 3 ),
 ( 0.8645833333333333703, 0.8652777777777778123, 0.8666666666666666963, 0.8680555555555555802, 0.8687500000000000222 ),
 .UNSPECIFIED. ) 
 CURVE ( )  GEOMETRIC_REPRESENTATION_ITEM ( )  RATIONAL_B_SPLINE_CURVE ( ( 0.9330127018922194093, 0.9330127018922194093, 1.000000000000000000, 0.8660254037844387076, 1.000000000000000000, 0.8660254037844387076, 1.000000000000000000, 0.9330127018922194093, 0.9330127018922194093 ) ) 
 REPRESENTATION_ITEM ( '' )  );
#1692=CARTESIAN_POINT ( 'NONE',  ( 4.458734124999998549, -64.97916666530106511, -2.574251347313721627 ) ) ;
#1694=ORIENTED_EDGE ( 'NONE', *, *, #16924, .F. ) ;
#1695=CARTESIAN_POINT ( 'NONE',  ( -9.184850993605147944E-16, -156.3750000027311842, 5.000000000000000000 ) ) ;
#1697=CARTESIAN_POINT ( 'NONE',  ( 5.000000000000000000, -62.50000000000000000, -6.123233995736766282E-16 ) ) ;
#1700=CARTESIAN_POINT ( 'NONE',  ( -4.458734124999999437, 8.604166668032261711, -2.574251347313719407 ) ) ;
#1701=DIRECTION ( 'NONE',  ( -0.000000000000000000, 1.000000000000000000, -0.000000000000000000 ) ) ;
#1702=CARTESIAN_POINT ( 'NONE',  ( -3.152801135295367096, -160.0625000013656063, -3.152801135295367541 ) ) ;
#1703=CARTESIAN_POINT ( 'NONE',  ( -6.972266317189433020E-16, 18.87500000273119127, -5.000000000000000000 ) ) ;
#1704=ORIENTED_EDGE ( 'NONE', *, *, #34627, .F. ) ;
#1708=CARTESIAN_POINT ( 'NONE',  ( 6.042630808230842148E-15, 25.87500000273118062, -4.999999999999999112 ) ) ;
#1712=CARTESIAN_POINT ( 'NONE',  ( 4.458734124999999437, 26.18750000136559564, -5.460374474430324690E-16 ) ) ;
#1716=CARTESIAN_POINT ( 'NONE',  ( 4.458734124999998549, 1.020833334698927120, -2.574251347313721627 ) ) ;
#1720=EDGE_CURVE ( 'NONE', #13785, #44325, #15820, .T. ) ;
#1721=CARTESIAN_POINT ( 'NONE',  ( -2.071067811865475061, -145.8125000027311842, -5.000000000000000888 ) ) ;
#1727=CARTESIAN_POINT ( 'NONE',  ( 0.000000000000000000, -170.0000000000000000, 0.000000000000000000 ) ) ;
#1731=CARTESIAN_POINT ( 'NONE',  ( 4.458734124999999437, -160.6875000013655779, 0.000000000000000000 ) ) ;
#1732=( BOUNDED_CURVE ( )  B_SPLINE_CURVE ( 2, ( #30278, #59572, #25460, #54421, #10350, #15505, #30602, #35757, #49898 ),
 .UNSPECIFIED., .F., .F. ) 
 B_SPLINE_CURVE_WITH_KNOTS ( ( 3, 2, 2, 2, 3 ),
 ( 0.5895833333333333481, 0.5902777777777777901, 0.5916666666666666741, 0.5930555555555555580, 0.5937500000000000000 ),
 .UNSPECIFIED. ) 
 CURVE ( )  GEOMETRIC_REPRESENTATION_ITEM ( )  RATIONAL_B_SPLINE_CURVE ( ( 0.9330127018922194093, 0.9330127018922194093, 1.000000000000000000, 0.8660254037844387076, 1.000000000000000000, 0.8660254037844387076, 1.000000000000000000, 0.9330127018922194093, 0.9330127018922194093 ) ) 
 REPRESENTATION_ITEM ( '' )  );
#1735=CARTESIAN_POINT ( 'NONE',  ( 1.846868145590736310, -140.6250000013656063, 4.458734124999999437 ) ) ;
#1736=EDGE_LOOP ( 'NONE', ( #48858, #39056, #46762, #36556 ) ) ;
#1737=CARTESIAN_POINT ( 'NONE',  ( 9.457646018065525792E-16, 24.68750000136559208, 5.148502694627439702 ) ) ;
#1738=VERTEX_POINT ( 'NONE', #43272 ) ;
#1744=CARTESIAN_POINT ( 'NONE',  ( 2.500000000000002220, 15.33333333333333215, 4.330127018922192761 ) ) ;
#1745=CARTESIAN_POINT ( 'NONE',  ( -3.152548672688508926E-16, -56.56249999863439371, -5.148502694627439702 ) ) ;
#1746=CARTESIAN_POINT ( 'NONE',  ( -4.458734124999999437, -10.39583333196773829, -2.574251347313719407 ) ) ;
#1750=CARTESIAN_POINT ( 'NONE',  ( -2.500000000000000444, -0.04166666393548221214, -4.330127018922193649 ) ) ;
#1752=CARTESIAN_POINT ( 'NONE',  ( 2.500000000000002220, -33.66666666666666430, 4.330127018922192761 ) ) ;
#1754=LINE ( 'NONE', #49662, #29496 ) ;
#1756=CARTESIAN_POINT ( 'NONE',  ( -1.339745962155610925, -31.66965819600733312, 5.000000000000000000 ) ) ;
#1757=CARTESIAN_POINT ( 'NONE',  ( -4.458734124999999437, -61.31249999863440081, 0.000000000000000000 ) ) ;
#1758=CARTESIAN_POINT ( 'NONE',  ( -4.458734125000001214, -152.1250000013655779, 1.846868145590734089 ) ) ;
#1759=CARTESIAN_POINT ( 'NONE',  ( 2.229367062500001939, -63.97916666530106511, 3.861377020970579999 ) ) ;
#1761=CARTESIAN_POINT ( 'NONE',  ( 5.000000000000000888, -58.45833333060214443, 2.886751345948126879 ) ) ;
#1762=VERTEX_POINT ( 'NONE', #48102 ) ;
#1768=CARTESIAN_POINT ( 'NONE',  ( 2.730187237215162345E-16, -151.1875000013656063, -4.458734124999999437 ) ) ;
#1769=VERTEX_POINT ( 'NONE', #4357 ) ;
#1773=CARTESIAN_POINT ( 'NONE',  ( 2.229367062499998831, -46.89583333196774362, -3.861377020970580887 ) ) ;
#1775=VERTEX_POINT ( 'NONE', #23976 ) ;
#1776=VECTOR ( 'NONE', #54934, 1000.000000000000000 ) ;
#1777=CARTESIAN_POINT ( 'NONE',  ( -5.000000000000000888, -145.4375000000000000, 2.071067811865474617 ) ) ;
#1780=CARTESIAN_POINT ( 'NONE',  ( 9.457646018065525792E-16, 24.93750000136559564, 5.148502694627439702 ) ) ;
#1787=CARTESIAN_POINT ( 'NONE',  ( 1.975475456537005874E-15, -28.62499999726881583, 5.000000000000000000 ) ) ;
#1789=CARTESIAN_POINT ( 'NONE',  ( 5.000000000000000000, -63.50000000000000000, -6.123233995736766282E-16 ) ) ;
#1790=CARTESIAN_POINT ( 'NONE',  ( -1.339745962155613812, -2.080341798530293662, -5.000000000000000000 ) ) ;
#1793=CARTESIAN_POINT ( 'NONE',  ( -6.972266317189433020E-16, -77.25000000000000000, -5.000000000000000000 ) ) ;
#1797=ORIENTED_EDGE ( 'NONE', *, *, #35457, .F. ) ;
#1798=DIRECTION ( 'NONE',  ( 0.000000000000000000, 0.000000000000000000, 1.000000000000000000 ) ) ;
#1800=CARTESIAN_POINT ( 'NONE',  ( -2.071067811865478170, -159.4375000027312694, 5.000000000000000000 ) ) ;
#1810=CARTESIAN_POINT ( 'NONE',  ( 9.457646018065525792E-16, -19.06249999863440792, 5.148502694627439702 ) ) ;
#1811=CARTESIAN_POINT ( 'NONE',  ( 0.000000000000000000, -170.0000000000000000, 0.000000000000000000 ) ) ;
#1812=CARTESIAN_POINT ( 'NONE',  ( 2.071067811865476394, -149.1875000000000000, 5.000000000000000000 ) ) ;
#1814=CARTESIAN_POINT ( 'NONE',  ( 1.846868145590736310, -153.6250000013655779, 4.458734124999999437 ) ) ;
#1816=CARTESIAN_POINT ( 'NONE',  ( 4.458734124999999437, -51.06249999863440792, -5.460374474430324690E-16 ) ) ;
#1819=CARTESIAN_POINT ( 'NONE',  ( -4.458734124999999437, -89.31249999863440792, 0.000000000000000000 ) ) ;
#1822=CARTESIAN_POINT ( 'NONE',  ( -4.458734124999999437, 2.604166668032263043, -2.574251347313719407 ) ) ;
#1823=CARTESIAN_POINT ( 'NONE',  ( -4.729367062499999719, -90.15624999931721106, 0.000000000000000000 ) ) ;
#1824=AXIS2_PLACEMENT_3D ( 'NONE', #23045, #61972, #17893 ) ;
#1827=CARTESIAN_POINT ( 'NONE',  ( 4.458734124999999437, 12.93750000136559208, -5.460374474430324690E-16 ) ) ;
#1828=CARTESIAN_POINT ( 'NONE',  ( 2.499999999999998668, 3.791666669397852019, -4.330127018922193649 ) ) ;
#1831=ORIENTED_EDGE ( 'NONE', *, *, #12665, .F. ) ;
#1833=CARTESIAN_POINT ( 'NONE',  ( 4.458734124999999437, -43.81249999863440081, -5.460374474430324690E-16 ) ) ;
#1834=CARTESIAN_POINT ( 'NONE',  ( 1.846868145590736310, -164.8750000013655779, 4.458734124999999437 ) ) ;
#1835=CARTESIAN_POINT ( 'NONE',  ( 5.000000000000000000, -39.29166666393548724, -2.886751345948129988 ) ) ;
#1837=CARTESIAN_POINT ( 'NONE',  ( -2.229367062499996610, -16.14583333196773651, 3.861377020970582219 ) ) ;
#1838=ORIENTED_EDGE ( 'NONE', *, *, #53172, .T. ) ;
#1840=CARTESIAN_POINT ( 'NONE',  ( -3.152801135295367985, -162.8125000013656063, 3.152801135295367096 ) ) ;
#1841=CARTESIAN_POINT ( 'NONE',  ( -5.000000000000000000, -85.87499999726880162, 0.000000000000000000 ) ) ;
#1843=VERTEX_POINT ( 'NONE', #9800 ) ;
#1845=CARTESIAN_POINT ( 'NONE',  ( 4.458734124999999437, -32.06249999863440792, -5.460374474430324690E-16 ) ) ;
#1846=CARTESIAN_POINT ( 'NONE',  ( 3.061616997868383141E-16, -147.8750000027312126, -5.000000000000000000 ) ) ;
#1851=ORIENTED_EDGE ( 'NONE', *, *, #12605, .F. ) ;
#1852=CARTESIAN_POINT ( 'NONE',  ( -5.000000000000000888, -166.5625000027312126, 2.071067811865474617 ) ) ;
#1854=CARTESIAN_POINT ( 'NONE',  ( 2.229367062500001939, -81.22916666530106511, 3.861377020970579999 ) ) ;
#1857=CARTESIAN_POINT ( 'NONE',  ( -4.458734125000000326, -141.1250000013656063, 1.846868145590734089 ) ) ;
#1860=CARTESIAN_POINT ( 'NONE',  ( -4.458734124999999437, -43.31249999863440081, 0.000000000000000000 ) ) ;
#1863=( BOUNDED_CURVE ( )  B_SPLINE_CURVE ( 2, ( #28925, #43403, #33446, #9938, #18656, #38574, #49187, #5125, #34710 ),
 .UNSPECIFIED., .F., .F. ) 
 B_SPLINE_CURVE_WITH_KNOTS ( ( 3, 2, 2, 2, 3 ),
 ( 0.3687500000000000222, 0.3694444444444444642, 0.3708333333333333481, 0.3722222222222222321, 0.3729166666666666741 ),
 .UNSPECIFIED. ) 
 CURVE ( )  GEOMETRIC_REPRESENTATION_ITEM ( )  RATIONAL_B_SPLINE_CURVE ( ( 0.9330127018922194093, 0.9330127018922194093, 1.000000000000000000, 0.8660254037844387076, 1.000000000000000000, 0.8660254037844387076, 1.000000000000000000, 0.9330127018922194093, 0.9330127018922194093 ) ) 
 REPRESENTATION_ITEM ( '' )  );
#1865=DIRECTION ( 'NONE',  ( 0.000000000000000000, 0.000000000000000000, 1.000000000000000000 ) ) ;
#1870=CARTESIAN_POINT ( 'NONE',  ( 4.458734124999998549, -76.97916666530106511, -2.574251347313721627 ) ) ;
#1871=CARTESIAN_POINT ( 'NONE',  ( 1.975475456537005874E-15, -34.75000000000000000, 5.000000000000000000 ) ) ;
#1876=LINE ( 'NONE', #21481, #1776 ) ;
#1879=CARTESIAN_POINT ( 'NONE',  ( -2.071067811865475061, -167.8125000027311842, -5.000000000000000888 ) ) ;
#1881=CARTESIAN_POINT ( 'NONE',  ( -2.229367062500000163, 12.27083333469892601, -3.861377020970580443 ) ) ;
#1882=CARTESIAN_POINT ( 'NONE',  ( 5.000000000000000000, -77.29166666393547303, -2.886751345948130876 ) ) ;
#1885=( BOUNDED_CURVE ( )  B_SPLINE_CURVE ( 2, ( #3552, #23160, #24107, #63667, #58515, #8378, #8993, #44019, #34062 ),
 .UNSPECIFIED., .F., .F. ) 
 B_SPLINE_CURVE_WITH_KNOTS ( ( 3, 2, 2, 2, 3 ),
 ( 0.2937500000000000111, 0.2944444444444444531, 0.2958333333333333370, 0.2972222222222222210, 0.2979166666666666630 ),
 .UNSPECIFIED. ) 
 CURVE ( )  GEOMETRIC_REPRESENTATION_ITEM ( )  RATIONAL_B_SPLINE_CURVE ( ( 0.9330127018922194093, 0.9330127018922194093, 1.000000000000000000, 0.8660254037844387076, 1.000000000000000000, 0.8660254037844387076, 1.000000000000000000, 0.9330127018922194093, 0.9330127018922194093 ) ) 
 REPRESENTATION_ITEM ( '' )  );
#1889=CARTESIAN_POINT ( 'NONE',  ( 4.458734125000001214, -82.89583333196772230, 2.574251347313718519 ) ) ;
#1890=CARTESIAN_POINT ( 'NONE',  ( -4.458734124999999437, -5.395833331967740953, -2.574251347313719407 ) ) ;
#1893=CARTESIAN_POINT ( 'NONE',  ( -2.229367062500000163, -28.72916666530107221, -3.861377020970580443 ) ) ;
#1897=CARTESIAN_POINT ( 'NONE',  ( -2.229367062500000163, 18.52083333469892779, -3.861377020970580443 ) ) ;
#1898=CARTESIAN_POINT ( 'NONE',  ( -2.499999999999996447, -43.70833333060214443, 4.330127018922195425 ) ) ;
#1899=CARTESIAN_POINT ( 'NONE',  ( -2.500000000000000444, -26.04166666393547658, -4.330127018922193649 ) ) ;
#1900=CARTESIAN_POINT ( 'NONE',  ( 2.229367062499998831, -75.89583333196773651, -3.861377020970580887 ) ) ;
#1903=CARTESIAN_POINT ( 'NONE',  ( -2.500000000000000444, 23.95833333606451987, -4.330127018922193649 ) ) ;
#1904=ORIENTED_EDGE ( 'NONE', *, *, #54985, .T. ) ;
#1908=CARTESIAN_POINT ( 'NONE',  ( -6.972266317189433020E-16, -0.2500000000000001665, -5.000000000000000000 ) ) ;
#1909=CARTESIAN_POINT ( 'NONE',  ( -5.000000000000000000, -26.08333333333333215, -2.886751345948128211 ) ) ;
#1910=CARTESIAN_POINT ( 'NONE',  ( -4.458734124999999437, -29.39583333196773296, -2.574251347313719407 ) ) ;
#1912=CARTESIAN_POINT ( 'NONE',  ( 9.457646018065525792E-16, -87.06249999863439371, 5.148502694627439702 ) ) ;
#1913=CARTESIAN_POINT ( 'NONE',  ( -5.000000000000000000, -23.87499999726881228, 0.000000000000000000 ) ) ;
#1914=CARTESIAN_POINT ( 'NONE',  ( 2.229367062499998831, -53.64583333196773651, -3.861377020970580887 ) ) ;
#1916=CARTESIAN_POINT ( 'NONE',  ( 1.339745962155615144, -27.70534180126147561, 4.999999999999999112 ) ) ;
#1918=CARTESIAN_POINT ( 'NONE',  ( 4.458734124999998549, -2.979166665301069994, -2.574251347313721627 ) ) ;
#1920=CARTESIAN_POINT ( 'NONE',  ( 5.000000000000000000, -73.41666666666665719, -2.886751345948129988 ) ) ;
#1924=CARTESIAN_POINT ( 'NONE',  ( -3.535533905932738641, -160.3750000000000284, 3.535533905932737309 ) ) ;
#1925=CARTESIAN_POINT ( 'NONE',  ( 5.000000000000000888, -69.45833333060214443, 2.886751345948126879 ) ) ;
#1928=CARTESIAN_POINT ( 'NONE',  ( -4.458734124999999437, -14.64583333196773474, -2.574251347313719407 ) ) ;
#1929=AXIS2_PLACEMENT_3D ( 'NONE', #26212, #25893, #35870 ) ;
#1930=CARTESIAN_POINT ( 'NONE',  ( -4.458734124999999437, -50.56249999863440792, 0.000000000000000000 ) ) ;
#1934=CARTESIAN_POINT ( 'NONE',  ( 1.846868145590736310, -144.6250000013655779, 4.458734124999999437 ) ) ;
#1935=EDGE_CURVE ( 'NONE', #9299, #58694, #23674, .T. ) ;
#1937=CARTESIAN_POINT ( 'NONE',  ( 3.061616997868383141E-16, -157.7500000000000000, -5.000000000000000000 ) ) ;
#1938=EDGE_LOOP ( 'NONE', ( #30187, #28325, #36191, #40566 ) ) ;
#1940=CARTESIAN_POINT ( 'NONE',  ( 9.457646018065525792E-16, 24.68750000136559208, 5.148502694627439702 ) ) ;
#1946=CARTESIAN_POINT ( 'NONE',  ( 4.458734124999999437, -149.6875000013656063, 0.000000000000000000 ) ) ;
#1948=CARTESIAN_POINT ( 'NONE',  ( 4.458734124999998549, -61.97916666530106511, -2.574251347313721627 ) ) ;
#1949=CARTESIAN_POINT ( 'NONE',  ( -4.999999999999998224, -83.79166666393545881, 2.886751345948131764 ) ) ;
#1950=CARTESIAN_POINT ( 'NONE',  ( -2.229367062499996610, -9.145833331967736513, 3.861377020970582219 ) ) ;
#1952=CARTESIAN_POINT ( 'NONE',  ( -1.846868145590734756, -145.1250000013656063, -4.458734124999999437 ) ) ;
#1954=ORIENTED_EDGE ( 'NONE', *, *, #56312, .F. ) ;
#1960=CARTESIAN_POINT ( 'NONE',  ( 2.500000000000002220, 1.458333336064519203, 4.330127018922192761 ) ) ;
#1966=CARTESIAN_POINT ( 'NONE',  ( -2.499999999999996447, -14.83333333333333037, 4.330127018922195425 ) ) ;
#1967=CARTESIAN_POINT ( 'NONE',  ( 9.457646018065525792E-16, 12.93750000136559208, 5.148502694627439702 ) ) ;
#1969=CARTESIAN_POINT ( 'NONE',  ( 4.458734125000000326, -15.14583333196773474, 2.574251347313718519 ) ) ;
#1970=( BOUNDED_CURVE ( )  B_SPLINE_CURVE ( 2, ( #17741, #57310, #27074, #3587, #32207, #17106, #58472, #63300, #19219 ),
 .UNSPECIFIED., .F., .F. ) 
 B_SPLINE_CURVE_WITH_KNOTS ( ( 3, 2, 2, 2, 3 ),
 ( 0.7416666666666664742, 0.7458333333333331261, 0.7499999999999997780, 0.7541666666666664298, 0.7583333333333330817 ),
 .UNSPECIFIED. ) 
 CURVE ( )  GEOMETRIC_REPRESENTATION_ITEM ( )  RATIONAL_B_SPLINE_CURVE ( ( 1.000000000000003997, 0.9238795325112826307, 1.000000000000000000, 0.9238795325112867385, 1.000000000000000000, 0.9238795325112867385, 1.000000000000000000, 0.9238795325112908463, 0.9999999999999958922 ) ) 
 REPRESENTATION_ITEM ( '' )  );
#1972=CARTESIAN_POINT ( 'NONE',  ( -8.190561711645485556E-16, -162.6875000013655779, 4.458734124999999437 ) ) ;
#1973=CARTESIAN_POINT ( 'NONE',  ( -5.000000000000000000, -38.08333333333333570, -2.886751345948128211 ) ) ;
#1976=CARTESIAN_POINT ( 'NONE',  ( -2.500000000000000444, -28.16666666666666785, -4.330127018922193649 ) ) ;
#1978=CARTESIAN_POINT ( 'NONE',  ( 9.457646018065525792E-16, -33.06249999863440792, 5.148502694627439702 ) ) ;
#1980=LINE ( 'NONE', #21582, #16163 ) ;
#1982=ORIENTED_EDGE ( 'NONE', *, *, #32984, .F. ) ;
#1985=CARTESIAN_POINT ( 'NONE',  ( -5.000000000000000000, -67.87499999726881583, 0.000000000000000000 ) ) ;
#1986=CARTESIAN_POINT ( 'NONE',  ( -2.499999999999996447, -5.833333333333336590, 4.330127018922195425 ) ) ;
#1988=CARTESIAN_POINT ( 'NONE',  ( 4.458734125000000326, -73.89583333196773651, 2.574251347313718519 ) ) ;
#1989=CARTESIAN_POINT ( 'NONE',  ( 2.499999999999998668, -22.20833333060215153, -4.330127018922193649 ) ) ;
#1990=CARTESIAN_POINT ( 'NONE',  ( 5.000000000000000000, -9.374999997268814056, -6.123233995736766282E-16 ) ) ;
#1991=CARTESIAN_POINT ( 'NONE',  ( -4.458734124999999437, -40.39583333196773651, -2.574251347313719407 ) ) ;
#1992=VERTEX_POINT ( 'NONE', #55165 ) ;
#1994=CARTESIAN_POINT ( 'NONE',  ( 2.229367062500001939, 13.77083333469892779, 3.861377020970579999 ) ) ;
#1995=EDGE_LOOP ( 'NONE', ( #51913, #30074, #14352, #18115 ) ) ;
#1997=CARTESIAN_POINT ( 'NONE',  ( 5.000000000000000000, -54.41666666666666430, -2.886751345948129988 ) ) ;
#2000=CARTESIAN_POINT ( 'NONE',  ( 3.535533905932738197, -144.8750000000000000, -3.535533905932738197 ) ) ;
#2001=CARTESIAN_POINT ( 'NONE',  ( -2.229367062499996610, -77.14583333196773651, 3.861377020970582219 ) ) ;
#2002=CARTESIAN_POINT ( 'NONE',  ( 3.152801135295366208, -141.8125000013655779, 3.152801135295367985 ) ) ;
#2003=CARTESIAN_POINT ( 'NONE',  ( 2.229367062500001939, -87.97916666530107932, 3.861377020970579999 ) ) ;
#2004=VECTOR ( 'NONE', #7384, 1000.000000000000000 ) ;
#2006=CARTESIAN_POINT ( 'NONE',  ( 4.458734124999999437, -33.06249999863440792, -5.460374474430324690E-16 ) ) ;
#2008=ORIENTED_EDGE ( 'NONE', *, *, #60078, .F. ) ;
#2009=EDGE_CURVE ( 'NONE', #54337, #24836, #6435, .T. ) ;
#2012=VERTEX_POINT ( 'NONE', #6586 ) ;
#2014=CARTESIAN_POINT ( 'NONE',  ( 1.975475456537005874E-15, -11.62499999726881406, 5.000000000000000000 ) ) ;
#2015=CARTESIAN_POINT ( 'NONE',  ( -2.229367062499996610, -65.39583333196773651, 3.861377020970582219 ) ) ;
#2017=EDGE_LOOP ( 'NONE', ( #6645, #32915, #9936, #10300 ) ) ;
#2019=CARTESIAN_POINT ( 'NONE',  ( -6.972266317189433020E-16, -62.24999999999999289, -5.000000000000000000 ) ) ;
#2020=ORIENTED_EDGE ( 'NONE', *, *, #41778, .F. ) ;
#2022=CARTESIAN_POINT ( 'NONE',  ( -3.152548672688508926E-16, 8.437500001365595637, -5.148502694627439702 ) ) ;
#2023=CARTESIAN_POINT ( 'NONE',  ( -9.184850993605147944E-16, -154.2500000000000000, 5.000000000000000000 ) ) ;
#2024=CARTESIAN_POINT ( 'NONE',  ( -8.190561711645485556E-16, -157.6875000013655779, 4.458734124999999437 ) ) ;
#2025=DIRECTION ( 'NONE',  ( -0.000000000000000000, 1.000000000000000000, -0.000000000000000000 ) ) ;
#2028=CARTESIAN_POINT ( 'NONE',  ( 5.000000000000000000, -164.1875000027312126, 2.071067811865478614 ) ) ;
#2030=FACE_OUTER_BOUND ( 'NONE', #31095, .T. ) ;
#2032=CYLINDRICAL_SURFACE ( 'NONE', #39898, 5.000000000000000000 ) ;
#2035=CARTESIAN_POINT ( 'NONE',  ( 4.458734125000000326, 29.10416666803226349, 2.574251347313718519 ) ) ;
#2038=CARTESIAN_POINT ( 'NONE',  ( 4.458734125000000326, 3.854166668032260823, 2.574251347313718519 ) ) ;
#2040=CARTESIAN_POINT ( 'NONE',  ( 5.000000000000000000, -160.1250000027311842, 0.000000000000000000 ) ) ;
#2042=CARTESIAN_POINT ( 'NONE',  ( 2.071067811865476394, -144.3125000027312126, 5.000000000000000000 ) ) ;
#2050=CARTESIAN_POINT ( 'NONE',  ( 3.152801135295366208, -162.8125000013656063, 3.152801135295367985 ) ) ;
#2053=CARTESIAN_POINT ( 'NONE',  ( 1.846868145590735200, -140.2500000013656063, -4.458734125000000326 ) ) ;
#2055=CARTESIAN_POINT ( 'NONE',  ( -2.229367062499996610, 22.60416666803225993, 3.861377020970582219 ) ) ;
#2061=CARTESIAN_POINT ( 'NONE',  ( -5.000000000000000000, 8.916666666666666075, -2.886751345948128211 ) ) ;
#2062=CARTESIAN_POINT ( 'NONE',  ( -2.229367062499996610, -58.14583333196773651, 3.861377020970582219 ) ) ;
#2063=CARTESIAN_POINT ( 'NONE',  ( 9.457646018065525792E-16, -11.06249999863440969, 5.148502694627439702 ) ) ;
#2065=FACE_OUTER_BOUND ( 'NONE', #4715, .T. ) ;
#2066=EDGE_CURVE ( 'NONE', #55117, #44647, #33098, .T. ) ;
#2067=ADVANCED_FACE ( 'NONE', ( #50003 ), #60949, .T. ) ;
#2069=CARTESIAN_POINT ( 'NONE',  ( 1.975475456537005874E-15, -36.75000000000000000, 5.000000000000000000 ) ) ;
#2072=CARTESIAN_POINT ( 'NONE',  ( 2.500000000000002220, -39.66666666666667140, 4.330127018922192761 ) ) ;
#2077=FACE_OUTER_BOUND ( 'NONE', #22962, .T. ) ;
#2078=CARTESIAN_POINT ( 'NONE',  ( 9.457646018065525792E-16, -57.06249999863440081, 5.148502694627439702 ) ) ;
#2079=CARTESIAN_POINT ( 'NONE',  ( 4.458734124999999437, -151.7500000013655779, 1.846868145590737864 ) ) ;
#2080=CARTESIAN_POINT ( 'NONE',  ( 2.229367062500001939, -69.97916666530107932, 3.861377020970579999 ) ) ;
#2083=ADVANCED_FACE ( 'NONE', ( #40990 ), #34899, .T. ) ;
#2084=CARTESIAN_POINT ( 'NONE',  ( 2.229367062500001939, -22.22916666530107221, 3.861377020970579999 ) ) ;
#2085=CARTESIAN_POINT ( 'NONE',  ( -5.000000000000000000, -60.95833333060214443, -2.886751345948128211 ) ) ;
#2087=CARTESIAN_POINT ( 'NONE',  ( 5.000000000000000888, -31.45833333060214798, 2.886751345948126879 ) ) ;
#2088=ORIENTED_EDGE ( 'NONE', *, *, #51233, .T. ) ;
#2090=CARTESIAN_POINT ( 'NONE',  ( -3.535533905932737309, -157.7500000027312126, -3.535533905932738197 ) ) ;
#2092=CARTESIAN_POINT ( 'NONE',  ( 3.152801135295367541, -154.3125000013656063, -3.152801135295367541 ) ) ;
#2094=ORIENTED_EDGE ( 'NONE', *, *, #48422, .T. ) ;
#2095=EDGE_CURVE ( 'NONE', #34156, #19872, #30705, .T. ) ;
#2098=DIRECTION ( 'NONE',  ( -0.000000000000000000, 1.000000000000000000, -0.000000000000000000 ) ) ;
#2099=AXIS2_PLACEMENT_3D ( 'NONE', #63432, #44421, #34786 ) ;
#2100=CARTESIAN_POINT ( 'NONE',  ( 4.458734124999999437, -49.06249999863440792, -5.460374474430324690E-16 ) ) ;
#2101=ORIENTED_EDGE ( 'NONE', *, *, #34250, .F. ) ;
#2102=CARTESIAN_POINT ( 'NONE',  ( -5.000000000000000888, -145.5625000000000568, -2.071067811865475949 ) ) ;
#2104=CARTESIAN_POINT ( 'NONE',  ( -4.458734124999999437, 24.68750000136559208, 0.000000000000000000 ) ) ;
#2107=CARTESIAN_POINT ( 'NONE',  ( 0.000000000000000000, -170.0000000000000000, 0.000000000000000000 ) ) ;
#2108=ORIENTED_EDGE ( 'NONE', *, *, #38873, .F. ) ;
#2116=CARTESIAN_POINT ( 'NONE',  ( -5.000000000000000000, -139.6250000027312126, -6.123233995736766282E-16 ) ) ;
#2117=( BOUNDED_CURVE ( )  B_SPLINE_CURVE ( 2, ( #62044, #16709, #36324, #11866, #63613, #29175, #43653, #48492, #33082 ),
 .UNSPECIFIED., .F., .F. ) 
 B_SPLINE_CURVE_WITH_KNOTS ( ( 3, 2, 2, 2, 3 ),
 ( 0.3104166666666666741, 0.3111111111111111160, 0.3125000000000000000, 0.3138888888888888840, 0.3145833333333333259 ),
 .UNSPECIFIED. ) 
 CURVE ( )  GEOMETRIC_REPRESENTATION_ITEM ( )  RATIONAL_B_SPLINE_CURVE ( ( 0.9330127018922194093, 0.9330127018922194093, 1.000000000000000000, 0.8660254037844387076, 1.000000000000000000, 0.8660254037844387076, 1.000000000000000000, 0.9330127018922194093, 0.9330127018922194093 ) ) 
 REPRESENTATION_ITEM ( '' )  );
#2118=DIRECTION ( 'NONE',  ( -0.000000000000000000, 1.000000000000000000, -0.000000000000000000 ) ) ;
#2121=ORIENTED_EDGE ( 'NONE', *, *, #20497, .F. ) ;
#2123=CARTESIAN_POINT ( 'NONE',  ( 3.535533905932738197, -157.0000000027312126, -3.535533905932738197 ) ) ;
#2132=CARTESIAN_POINT ( 'NONE',  ( 4.458734124999999437, -23.81249999863440436, -5.460374474430324690E-16 ) ) ;
#2133=CARTESIAN_POINT ( 'NONE',  ( 2.071067811865392461, -147.1875000000000853, 5.000000000000084377 ) ) ;
#2134=CARTESIAN_POINT ( 'NONE',  ( 3.535533905932738197, -152.8750000000000000, -3.535533905932738197 ) ) ;
#2136=CARTESIAN_POINT ( 'NONE',  ( 4.458734124999999437, -151.4375000013655779, 0.000000000000000000 ) ) ;
#2137=ORIENTED_EDGE ( 'NONE', *, *, #32329, .T. ) ;
#2138=CARTESIAN_POINT ( 'NONE',  ( -2.229367062499996610, -49.39583333196772941, 3.861377020970582219 ) ) ;
#2140=CARTESIAN_POINT ( 'NONE',  ( -4.999999999999999112, 23.08333333333332860, 2.886751345948131764 ) ) ;
#2141=VECTOR ( 'NONE', #37387, 1000.000000000000000 ) ;
#2142=CARTESIAN_POINT ( 'NONE',  ( 1.975475456537005874E-15, 13.24999999999999822, 5.000000000000000000 ) ) ;
#2143=CARTESIAN_POINT ( 'NONE',  ( -2.229367062500000163, 3.520833334698929118, -3.861377020970580443 ) ) ;
#2145=CARTESIAN_POINT ( 'NONE',  ( -6.972266317189433020E-16, -41.12499999726880162, -5.000000000000000000 ) ) ;
#2147=CARTESIAN_POINT ( 'NONE',  ( -3.152548672688508926E-16, 14.18750000136559386, -5.148502694627439702 ) ) ;
#2148=CARTESIAN_POINT ( 'NONE',  ( 2.500000000000002220, 2.458333336064519870, 4.330127018922192761 ) ) ;
#2150=CARTESIAN_POINT ( 'NONE',  ( 2.500000000000002220, 26.33333333333333215, 4.330127018922192761 ) ) ;
#2151=VERTEX_POINT ( 'NONE', #8487 ) ;
#2153=CARTESIAN_POINT ( 'NONE',  ( -2.229367062500000163, -42.47916666530107932, -3.861377020970580443 ) ) ;
#2155=CARTESIAN_POINT ( 'NONE',  ( -8.190561711645485556E-16, -163.9375000013655779, 4.458734124999999437 ) ) ;
#2156=CARTESIAN_POINT ( 'NONE',  ( 2.500000000000002220, -45.54166666393547303, 4.330127018922192761 ) ) ;
#2158=CARTESIAN_POINT ( 'NONE',  ( -4.458734124999999437, -19.31249999863440081, 0.000000000000000000 ) ) ;
#2160=CARTESIAN_POINT ( 'NONE',  ( -5.000000000000000000, -87.08333333333331439, -2.886751345948128211 ) ) ;
#2161=CARTESIAN_POINT ( 'NONE',  ( 4.458734124999999437, -165.4375000013655779, 0.000000000000000000 ) ) ;
#2163=LINE ( 'NONE', #41362, #48744 ) ;
#2166=CARTESIAN_POINT ( 'NONE',  ( -4.458734124999999437, -33.56249999863440792, 0.000000000000000000 ) ) ;
#2167=CARTESIAN_POINT ( 'NONE',  ( -2.071067811865306307, -147.8125000027311842, -5.000000000000171418 ) ) ;
#2169=EDGE_CURVE ( 'NONE', #2464, #30447, #54888, .T. ) ;
#2177=CARTESIAN_POINT ( 'NONE',  ( 4.458734125000001214, -83.14583333196773651, 2.574251347313718519 ) ) ;
#2180=CARTESIAN_POINT ( 'NONE',  ( 2.730187237215162345E-16, -143.4375000013656063, -4.458734124999999437 ) ) ;
#2181=CARTESIAN_POINT ( 'NONE',  ( -2.499999999999996447, 6.291666669397851130, 4.330127018922195425 ) ) ;
#2183=CARTESIAN_POINT ( 'NONE',  ( 9.457646018065525792E-16, -47.06249999863440792, 5.148502694627439702 ) ) ;
#2186=CARTESIAN_POINT ( 'NONE',  ( 1.339745962155615144, -3.705341801261480494, 4.999999999999999112 ) ) ;
#2191=CARTESIAN_POINT ( 'NONE',  ( 4.458734125000001214, -77.14583333196775072, 2.574251347313718519 ) ) ;
#2201=CARTESIAN_POINT ( 'NONE',  ( -2.229367062500000163, 10.27083333469892779, -3.861377020970580443 ) ) ;
#2202=FACE_OUTER_BOUND ( 'NONE', #31709, .T. ) ;
#2207=CARTESIAN_POINT ( 'NONE',  ( -1.339745962155613812, -16.08034179853029499, -5.000000000000000000 ) ) ;
#2208=CARTESIAN_POINT ( 'NONE',  ( 4.458734125000001214, -86.89583333196773651, 2.574251347313718519 ) ) ;
#2209=CARTESIAN_POINT ( 'NONE',  ( 2.229367062500001939, -9.979166665301068662, 3.861377020970579999 ) ) ;
#2210=FACE_OUTER_BOUND ( 'NONE', #52909, .T. ) ;
#2212=CARTESIAN_POINT ( 'NONE',  ( 4.458734125000000326, -38.14583333196773651, 2.574251347313718519 ) ) ;
#2216=CARTESIAN_POINT ( 'NONE',  ( 2.229367062500001939, 18.02083333469892779, 3.861377020970579999 ) ) ;
#2217=CARTESIAN_POINT ( 'NONE',  ( 5.000000000000000000, -53.41666666666667140, -2.886751345948130876 ) ) ;
#2218=CARTESIAN_POINT ( 'NONE',  ( 5.000000000000000000, 1.583333333333332371, -2.886751345948130876 ) ) ;
#2219=CARTESIAN_POINT ( 'NONE',  ( 9.457646018065525792E-16, -81.31249999863440792, 5.148502694627439702 ) ) ;
#2222=CARTESIAN_POINT ( 'NONE',  ( 5.000000000000000000, 18.62500000273118772, -6.123233995736766282E-16 ) ) ;
#2224=CARTESIAN_POINT ( 'NONE',  ( -5.000000000000000000, -66.08333333333332860, -2.886751345948128211 ) ) ;
#2226=CARTESIAN_POINT ( 'NONE',  ( -2.071067811865604735, -149.3125000000000284, 4.999999999999872990 ) ) ;
#2227=CARTESIAN_POINT ( 'NONE',  ( 1.060575238724906964E-15, -24.75000000000000355, 5.773502691896257311 ) ) ;
#2228=CARTESIAN_POINT ( 'NONE',  ( 4.458734125000001214, -25.89583333196774007, 2.574251347313718519 ) ) ;
#2230=CARTESIAN_POINT ( 'NONE',  ( -4.458734124999999437, -87.39583333196773651, -2.574251347313719407 ) ) ;
#2231=CARTESIAN_POINT ( 'NONE',  ( 1.060575238724906964E-15, -28.62499999726881228, 5.773502691896257311 ) ) ;
#2232=CARTESIAN_POINT ( 'NONE',  ( -4.458734124999999437, -55.39583333196773651, -2.574251347313719407 ) ) ;
#2234=CARTESIAN_POINT ( 'NONE',  ( 2.499999999999998668, -65.33333333333332860, -4.330127018922193649 ) ) ;
#2236=CARTESIAN_POINT ( 'NONE',  ( -3.152548672688508926E-16, -1.812499998634406362, -5.148502694627439702 ) ) ;
#2237=ORIENTED_EDGE ( 'NONE', *, *, #6708, .F. ) ;
#2238=CARTESIAN_POINT ( 'NONE',  ( -5.000000000000000000, -73.08333333333334281, -2.886751345948128211 ) ) ;
#2241=DIRECTION ( 'NONE',  ( -0.000000000000000000, 1.000000000000000000, -0.000000000000000000 ) ) ;
#2242=CARTESIAN_POINT ( 'NONE',  ( 5.000000000000000000, -69.29166666393548724, -2.886751345948129988 ) ) ;
#2245=CARTESIAN_POINT ( 'NONE',  ( 4.458734124999999437, -14.06249999863440436, -5.460374474430324690E-16 ) ) ;
#2246=CARTESIAN_POINT ( 'NONE',  ( 4.458734124999999437, -49.06249999863440792, -5.460374474430324690E-16 ) ) ;
#2248=CARTESIAN_POINT ( 'NONE',  ( 1.339745962155637349, 10.70534180126147739, -4.999999999999985789 ) ) ;
#2249=CARTESIAN_POINT ( 'NONE',  ( 4.458734125000000326, -169.6250000013656063, -1.846868145590734978 ) ) ;
#2251=CARTESIAN_POINT ( 'NONE',  ( 5.000000000000000000, -158.0000000000000000, 0.000000000000000000 ) ) ;
#2254=CARTESIAN_POINT ( 'NONE',  ( -2.229367062499996610, 23.60416666803225993, 3.861377020970582219 ) ) ;
#2259=( BOUNDED_CURVE ( )  B_SPLINE_CURVE ( 2, ( #52182, #8127, #46720, #6858, #3306, #7493, #62158, #18077, #26472 ),
 .UNSPECIFIED., .F., .F. ) 
 B_SPLINE_CURVE_WITH_KNOTS ( ( 3, 2, 2, 2, 3 ),
 ( 0.9729166666666666519, 0.9736111111111110938, 0.9749999999999999778, 0.9763888888888888618, 0.9770833333333333037 ),
 .UNSPECIFIED. ) 
 CURVE ( )  GEOMETRIC_REPRESENTATION_ITEM ( )  RATIONAL_B_SPLINE_CURVE ( ( 0.9330127018922194093, 0.9330127018922194093, 1.000000000000000000, 0.8660254037844387076, 1.000000000000000000, 0.8660254037844387076, 1.000000000000000000, 0.9330127018922194093, 0.9330127018922194093 ) ) 
 REPRESENTATION_ITEM ( '' )  );
#2260=CARTESIAN_POINT ( 'NONE',  ( -3.152801135295367985, -148.0625000013655779, 3.152801135295367096 ) ) ;
#2263=CARTESIAN_POINT ( 'NONE',  ( -2.229367062500000163, -65.72916666530106511, -3.861377020970580443 ) ) ;
#2266=CARTESIAN_POINT ( 'NONE',  ( -1.846868145590737420, -143.7500000013655779, 4.458734124999997661 ) ) ;
#2270=CARTESIAN_POINT ( 'NONE',  ( 5.000000000000000888, 16.41666666666666785, 2.886751345948126879 ) ) ;
#2274=CARTESIAN_POINT ( 'NONE',  ( 4.458734125000000326, 26.85416666803225993, 2.574251347313718519 ) ) ;
#2277=CARTESIAN_POINT ( 'NONE',  ( 5.000000000000000888, -150.0625000027312126, -2.071067811865475505 ) ) ;
#2281=CARTESIAN_POINT ( 'NONE',  ( -2.229367062500000163, 12.52083333469892601, -3.861377020970580443 ) ) ;
#2284=CARTESIAN_POINT ( 'NONE',  ( -4.458734124999999437, -19.64583333196774362, -2.574251347313719407 ) ) ;
#2286=CARTESIAN_POINT ( 'NONE',  ( -3.152801135295367096, -161.0625000013656063, -3.152801135295367541 ) ) ;
#2287=DIRECTION ( 'NONE',  ( -0.000000000000000000, 1.000000000000000000, -0.000000000000000000 ) ) ;
#2290=CARTESIAN_POINT ( 'NONE',  ( 0.000000000000000000, -170.0000000000000000, 5.000000000000000000 ) ) ;
#2291=CARTESIAN_POINT ( 'NONE',  ( -5.000000000000000000, -88.87499999726880162, 0.000000000000000000 ) ) ;
#2292=CARTESIAN_POINT ( 'NONE',  ( -2.229367062500000163, -33.47916666530107221, -3.861377020970580443 ) ) ;
#2293=CARTESIAN_POINT ( 'NONE',  ( -6.972266317189433020E-16, -60.24999999999999289, -5.000000000000000000 ) ) ;
#2296=CARTESIAN_POINT ( 'NONE',  ( 1.975475456537005874E-15, -36.62499999726880873, 5.000000000000000000 ) ) ;
#2301=CARTESIAN_POINT ( 'NONE',  ( -5.000000000000000000, -10.08333333333333393, -2.886751345948128211 ) ) ;
#2302=CARTESIAN_POINT ( 'NONE',  ( 4.458734124999998549, -74.72916666530106511, -2.574251347313721627 ) ) ;
#2303=CARTESIAN_POINT ( 'NONE',  ( 0.000000000000000000, -170.0000000000000000, 0.000000000000000000 ) ) ;
#2304=CARTESIAN_POINT ( 'NONE',  ( 2.499999999999998668, -7.208333330602150646, -4.330127018922193649 ) ) ;
#2305=CARTESIAN_POINT ( 'NONE',  ( 2.229367062500001939, -37.97916666530107221, 3.861377020970579999 ) ) ;
#2307=CARTESIAN_POINT ( 'NONE',  ( -2.229367062499996610, 13.60416666803226171, 3.861377020970582219 ) ) ;
#2309=CARTESIAN_POINT ( 'NONE',  ( 2.499999999999998668, -81.33333333333332860, -4.330127018922193649 ) ) ;
#2310=CARTESIAN_POINT ( 'NONE',  ( 2.500000000000002220, -54.66666666666667140, 4.330127018922192761 ) ) ;
#2311=CARTESIAN_POINT ( 'NONE',  ( 3.152801135295367541, -159.5625000013656063, -3.152801135295367541 ) ) ;
#2313=CARTESIAN_POINT ( 'NONE',  ( 2.229367062499998831, -78.64583333196773651, -3.861377020970580887 ) ) ;
#2314=( BOUNDED_CURVE ( )  B_SPLINE_CURVE ( 2, ( #47785, #3742, #23363, #32049, #7626, #12437, #37513, #42962, #27854 ),
 .UNSPECIFIED., .F., .F. ) 
 B_SPLINE_CURVE_WITH_KNOTS ( ( 3, 2, 2, 2, 3 ),
 ( 0.3416666666666669516, 0.3458333333333336035, 0.3500000000000002554, 0.3541666666666669627, 0.3583333333333336146 ),
 .UNSPECIFIED. ) 
 CURVE ( )  GEOMETRIC_REPRESENTATION_ITEM ( )  RATIONAL_B_SPLINE_CURVE ( ( 0.9999999999999948930, 0.9238795325112918455, 1.000000000000000000, 0.9238795325112867385, 1.000000000000000000, 0.9238795325112867385, 1.000000000000000000, 0.9238795325112816315, 1.000000000000005107 ) ) 
 REPRESENTATION_ITEM ( '' )  );
#2315=CARTESIAN_POINT ( 'NONE',  ( 4.458734124999999437, -141.6875000013656063, 0.000000000000000000 ) ) ;
#2316=CARTESIAN_POINT ( 'NONE',  ( 4.458734124999998549, -85.72916666530106511, -2.574251347313721627 ) ) ;
#2318=CARTESIAN_POINT ( 'NONE',  ( 4.458734124999998549, -34.97916666530107221, -2.574251347313721627 ) ) ;
#2320=CARTESIAN_POINT ( 'NONE',  ( 2.499999999999998668, -86.33333333333332860, -4.330127018922193649 ) ) ;
#2323=CARTESIAN_POINT ( 'NONE',  ( -4.458734124999999437, -65.56249999863440792, 0.000000000000000000 ) ) ;
#2325=VERTEX_POINT ( 'NONE', #3356 ) ;
#2326=DIRECTION ( 'NONE',  ( 0.000000000000000000, 0.000000000000000000, 1.000000000000000000 ) ) ;
#2329=CARTESIAN_POINT ( 'NONE',  ( -6.972266317189433020E-16, 2.750000000000000000, -5.000000000000000000 ) ) ;
#2330=CARTESIAN_POINT ( 'NONE',  ( 4.458734124999999437, 9.187500001365592084, -5.460374474430324690E-16 ) ) ;
#2331=CARTESIAN_POINT ( 'NONE',  ( 2.071067811865645591, -154.1874999999999716, 4.999999999999830358 ) ) ;
#2332=CARTESIAN_POINT ( 'NONE',  ( -4.458734124999999437, -156.0000000013656063, -1.846868145590735644 ) ) ;
#2333=( BOUNDED_CURVE ( )  B_SPLINE_CURVE ( 2, ( #55407, #45107, #30628, #45749, #7157, #50250, #40911, #26767, #1703 ),
 .UNSPECIFIED., .F., .F. ) 
 B_SPLINE_CURVE_WITH_KNOTS ( ( 3, 2, 2, 2, 3 ),
 ( 0.08125000000000000278, 0.08194444444444444475, 0.08333333333333332871, 0.08472222222222222654, 0.08541666666666666852 ),
 .UNSPECIFIED. ) 
 CURVE ( )  GEOMETRIC_REPRESENTATION_ITEM ( )  RATIONAL_B_SPLINE_CURVE ( ( 0.9330127018922194093, 0.9330127018922194093, 1.000000000000000000, 0.8660254037844387076, 1.000000000000000000, 0.8660254037844387076, 1.000000000000000000, 0.9330127018922194093, 0.9330127018922194093 ) ) 
 REPRESENTATION_ITEM ( '' )  );
#2334=CYLINDRICAL_SURFACE ( 'NONE', #24456, 5.000000000000000000 ) ;
#2339=EDGE_CURVE ( 'NONE', #12432, #15117, #26524, .T. ) ;
#2342=CARTESIAN_POINT ( 'NONE',  ( 1.975475456537005874E-15, -78.74999999999998579, 5.000000000000000000 ) ) ;
#2344=CARTESIAN_POINT ( 'NONE',  ( 2.500000000000002220, -10.66666666666666430, 4.330127018922192761 ) ) ;
#2345=CARTESIAN_POINT ( 'NONE',  ( -2.229367062499996610, 27.85416666803225993, 3.861377020970582219 ) ) ;
#2348=CARTESIAN_POINT ( 'NONE',  ( -2.229367062500000163, -0.7291666653010709931, -3.861377020970580443 ) ) ;
#2351=CARTESIAN_POINT ( 'NONE',  ( -2.071067811865478170, -141.4375000027312410, 5.000000000000000000 ) ) ;
#2352=DIRECTION ( 'NONE',  ( -0.000000000000000000, 1.000000000000000000, -0.000000000000000000 ) ) ;
#2353=EDGE_CURVE ( 'NONE', #27072, #23020, #12987, .T. ) ;
#2361=CARTESIAN_POINT ( 'NONE',  ( 2.730187237215162345E-16, -161.4375000013655779, -4.458734124999999437 ) ) ;
#2364=CARTESIAN_POINT ( 'NONE',  ( 1.846868145590735200, -141.2500000013656063, -4.458734125000000326 ) ) ;
#2365=ORIENTED_EDGE ( 'NONE', *, *, #42129, .T. ) ;
#2366=CARTESIAN_POINT ( 'NONE',  ( 4.458734124999998549, 21.02083333469892779, -2.574251347313721627 ) ) ;
#2367=VERTEX_POINT ( 'NONE', #20840 ) ;
#2372=CARTESIAN_POINT ( 'NONE',  ( 2.500000000000002220, 6.333333333333333037, 4.330127018922192761 ) ) ;
#2373=CARTESIAN_POINT ( 'NONE',  ( 4.458734125000000326, -56.89583333196774362, 2.574251347313718519 ) ) ;
#2374=CARTESIAN_POINT ( 'NONE',  ( -6.972266317189433020E-16, -89.24999999999998579, -5.000000000000000000 ) ) ;
#2377=CARTESIAN_POINT ( 'NONE',  ( -1.339745962155610925, -36.79465819873852439, 5.000000000000000000 ) ) ;
#2379=CARTESIAN_POINT ( 'NONE',  ( -3.535250795749689387E-16, -39.24999999999999289, -5.773502691896257311 ) ) ;
#2380=CARTESIAN_POINT ( 'NONE',  ( -9.184850993605147944E-16, -163.2500000000000000, 5.000000000000000000 ) ) ;
#2383=CARTESIAN_POINT ( 'NONE',  ( -6.972266317189433020E-16, 12.75000000000000178, -5.000000000000000000 ) ) ;
#2384=CARTESIAN_POINT ( 'NONE',  ( 2.229367062499998831, -57.64583333196773651, -3.861377020970580887 ) ) ;
#2385=CARTESIAN_POINT ( 'NONE',  ( -3.152801135295367985, -152.0625000013655779, 3.152801135295367096 ) ) ;
#2386=CARTESIAN_POINT ( 'NONE',  ( -4.458734124999999437, -73.39583333196773651, -2.574251347313719407 ) ) ;
#2388=CARTESIAN_POINT ( 'NONE',  ( 4.458734124999999437, -19.06249999863440792, -5.460374474430324690E-16 ) ) ;
#2389=CARTESIAN_POINT ( 'NONE',  ( 1.060575238724906964E-15, -59.62499999726880873, 5.773502691896257311 ) ) ;
#2391=CARTESIAN_POINT ( 'NONE',  ( -9.184850993605147944E-16, -150.2500000000000284, 5.000000000000000000 ) ) ;
#2395=CARTESIAN_POINT ( 'NONE',  ( 4.458734125000000326, -151.3750000013656063, -1.846868145590734978 ) ) ;
#2396=ORIENTED_EDGE ( 'NONE', *, *, #23242, .T. ) ;
#2397=CARTESIAN_POINT ( 'NONE',  ( 5.000000000000000888, 25.41666666666666430, 2.886751345948126879 ) ) ;
#2399=CARTESIAN_POINT ( 'NONE',  ( -1.339745962155610925, -77.66965819600730470, 5.000000000000000000 ) ) ;
#2400=CARTESIAN_POINT ( 'NONE',  ( 4.458734124999998549, -46.97916666530106511, -2.574251347313721627 ) ) ;
#2403=CARTESIAN_POINT ( 'NONE',  ( -4.458734124999998549, 23.77083333469892423, 2.574251347313722516 ) ) ;
#2405=CARTESIAN_POINT ( 'NONE',  ( -1.846868145590734756, -167.1250000013656063, -4.458734124999999437 ) ) ;
#2406=ORIENTED_EDGE ( 'NONE', *, *, #12488, .F. ) ;
#2417=CARTESIAN_POINT ( 'NONE',  ( 1.339745962155612702, -45.29465819873851729, -5.000000000000000000 ) ) ;
#2421=ORIENTED_EDGE ( 'NONE', *, *, #48347, .F. ) ;
#2424=CARTESIAN_POINT ( 'NONE',  ( -5.000000000000000888, -157.5625000027311842, 2.071067811865474617 ) ) ;
#2429=EDGE_CURVE ( 'NONE', #8193, #59584, #22402, .T. ) ;
#2432=CARTESIAN_POINT ( 'NONE',  ( 3.535533905932736864, -147.1250000000000000, 3.535533905932738641 ) ) ;
#2434=EDGE_CURVE ( 'NONE', #16392, #5665, #590, .T. ) ;
#2436=CARTESIAN_POINT ( 'NONE',  ( -2.499999999999996447, -89.83333333333332860, 4.330127018922195425 ) ) ;
#2437=CARTESIAN_POINT ( 'NONE',  ( -2.229367062500000163, -23.47916666530107221, -3.861377020970580443 ) ) ;
#2439=CARTESIAN_POINT ( 'NONE',  ( -5.000000000000000888, -152.4375000000000284, 2.071067811865474617 ) ) ;
#2441=CARTESIAN_POINT ( 'NONE',  ( 4.458734124999999437, -153.4375000013655779, 0.000000000000000000 ) ) ;
#2442=VERTEX_POINT ( 'NONE', #272 ) ;
#2443=CARTESIAN_POINT ( 'NONE',  ( 3.061616997868383141E-16, -149.7500000000000284, -5.000000000000000000 ) ) ;
#2444=CARTESIAN_POINT ( 'NONE',  ( 4.458734125000000326, -51.14583333196772941, 2.574251347313718519 ) ) ;
#2448=CARTESIAN_POINT ( 'NONE',  ( 2.500000000000002220, 26.33333333333333215, 4.330127018922192761 ) ) ;
#2450=CARTESIAN_POINT ( 'NONE',  ( -2.229367062499996610, 4.854166668032261711, 3.861377020970582219 ) ) ;
#2452=CARTESIAN_POINT ( 'NONE',  ( 5.000000000000000888, -11.45833333060214976, 2.886751345948126879 ) ) ;
#2453=CARTESIAN_POINT ( 'NONE',  ( 9.457646018065525792E-16, 17.68750000136559564, 5.148502694627439702 ) ) ;
#2454=CARTESIAN_POINT ( 'NONE',  ( -4.999999999999999112, 1.208333336064518759, 2.886751345948131764 ) ) ;
#2456=CARTESIAN_POINT ( 'NONE',  ( 5.000000000000000000, -42.41666666666667140, -2.886751345948130876 ) ) ;
#2457=ORIENTED_EDGE ( 'NONE', *, *, #26383, .F. ) ;
#2459=CARTESIAN_POINT ( 'NONE',  ( 9.457646018065525792E-16, -41.06249999863440792, 5.148502694627439702 ) ) ;
#2460=CARTESIAN_POINT ( 'NONE',  ( 4.458734124999999437, -165.7500000013655495, 1.846868145590737864 ) ) ;
#2461=CARTESIAN_POINT ( 'NONE',  ( -4.999999999999999112, -45.79166666393547303, 2.886751345948131764 ) ) ;
#2463=CARTESIAN_POINT ( 'NONE',  ( 4.458734124999998549, -19.72916666530107221, -2.574251347313721627 ) ) ;
#2464=VERTEX_POINT ( 'NONE', #59765 ) ;
#2465=CARTESIAN_POINT ( 'NONE',  ( -5.000000000000000000, -86.08333333333334281, -2.886751345948128211 ) ) ;
#2466=CARTESIAN_POINT ( 'NONE',  ( 4.458734124999999437, -166.4375000013655779, 0.000000000000000000 ) ) ;
#2467=CARTESIAN_POINT ( 'NONE',  ( 2.500000000000002220, -20.54166666393548013, 4.330127018922192761 ) ) ;
#2468=ORIENTED_EDGE ( 'NONE', *, *, #14861, .T. ) ;
#2470=CARTESIAN_POINT ( 'NONE',  ( -4.458734124999998549, -30.47916666530107221, 2.574251347313722516 ) ) ;
#2471=ORIENTED_EDGE ( 'NONE', *, *, #25040, .T. ) ;
#2474=CARTESIAN_POINT ( 'NONE',  ( 5.000000000000000000, 24.62500000273118417, -6.123233995736766282E-16 ) ) ;
#2475=ORIENTED_EDGE ( 'NONE', *, *, #50260, .T. ) ;
#2478=CARTESIAN_POINT ( 'NONE',  ( 4.458734124999998549, -77.97916666530106511, -2.574251347313721627 ) ) ;
#2483=CARTESIAN_POINT ( 'NONE',  ( 6.123233995736766282E-16, -170.0000000000000000, -5.000000000000000000 ) ) ;
#2485=CARTESIAN_POINT ( 'NONE',  ( 2.229367062500001939, -42.97916666530107932, 3.861377020970579999 ) ) ;
#2488=CARTESIAN_POINT ( 'NONE',  ( -6.972266317189433020E-16, 20.74999999999999645, -5.000000000000000000 ) ) ;
#2489=ADVANCED_FACE ( 'NONE', ( #10225 ), #15050, .T. ) ;
#2492=CARTESIAN_POINT ( 'NONE',  ( -3.535533905932737309, -153.7500000027312126, -3.535533905932738197 ) ) ;
#2494=CARTESIAN_POINT ( 'NONE',  ( -2.229367062500000163, -78.72916666530106511, -3.861377020970580443 ) ) ;
#2498=ORIENTED_EDGE ( 'NONE', *, *, #33570, .T. ) ;
#2500=CYLINDRICAL_SURFACE ( 'NONE', #20251, 5.000000000000000000 ) ;
#2502=CARTESIAN_POINT ( 'NONE',  ( -4.458734124999999437, 11.43750000136559564, 0.000000000000000000 ) ) ;
#2509=FACE_OUTER_BOUND ( 'NONE', #36769, .T. ) ;
#2510=CARTESIAN_POINT ( 'NONE',  ( -2.229367062500000163, -11.47916666530107044, -3.861377020970580443 ) ) ;
#2512=EDGE_CURVE ( 'NONE', #22662, #34612, #29831, .T. ) ;
#2514=CARTESIAN_POINT ( 'NONE',  ( 4.458734125000000326, -34.14583333196772941, 2.574251347313718519 ) ) ;
#2519=CARTESIAN_POINT ( 'NONE',  ( 2.730187237215162345E-16, -149.4375000013656063, -4.458734124999999437 ) ) ;
#2520=CARTESIAN_POINT ( 'NONE',  ( -4.458734124999998549, 22.77083333469892423, 2.574251347313722516 ) ) ;
#2524=CARTESIAN_POINT ( 'NONE',  ( -3.152548672688508926E-16, -82.81249999863442213, -5.148502694627439702 ) ) ;
#2527=CARTESIAN_POINT ( 'NONE',  ( 2.499999999999998668, 16.79166666939785202, -4.330127018922193649 ) ) ;
#2529=CARTESIAN_POINT ( 'NONE',  ( 1.975475456537005874E-15, -25.75000000000000355, 5.000000000000000000 ) ) ;
#2531=( BOUNDED_CURVE ( )  B_SPLINE_CURVE ( 2, ( #32216, #12913, #12603, #36739, #8107, #51537, #61827, #28338, #3597 ),
 .UNSPECIFIED., .F., .F. ) 
 B_SPLINE_CURVE_WITH_KNOTS ( ( 3, 2, 2, 2, 3 ),
 ( 0.4562499999999999889, 0.4569444444444444309, 0.4583333333333333148, 0.4597222222222221988, 0.4604166666666666963 ),
 .UNSPECIFIED. ) 
 CURVE ( )  GEOMETRIC_REPRESENTATION_ITEM ( )  RATIONAL_B_SPLINE_CURVE ( ( 0.9330127018922194093, 0.9330127018922194093, 1.000000000000000000, 0.8660254037844387076, 1.000000000000000000, 0.8660254037844387076, 1.000000000000000000, 0.9330127018922167448, 0.9330127018922194093 ) ) 
 REPRESENTATION_ITEM ( '' )  );
#2532=CARTESIAN_POINT ( 'NONE',  ( 2.500000000000002220, -52.66666666666666430, 4.330127018922192761 ) ) ;
#2533=CARTESIAN_POINT ( 'NONE',  ( -5.000000000000000000, -24.00000000000000000, 0.000000000000000000 ) ) ;
#2534=CARTESIAN_POINT ( 'NONE',  ( -2.229367062500000163, -26.47916666530106866, -3.861377020970580443 ) ) ;
#2535=CARTESIAN_POINT ( 'NONE',  ( 9.457646018065525792E-16, -86.06249999863439371, 5.148502694627439702 ) ) ;
#2536=CARTESIAN_POINT ( 'NONE',  ( 2.499999999999998668, -31.20833333060214443, -4.330127018922193649 ) ) ;
#2537=CARTESIAN_POINT ( 'NONE',  ( -2.229367062499996610, -56.14583333196773651, 3.861377020970582219 ) ) ;
#2540=CARTESIAN_POINT ( 'NONE',  ( -3.152548672688508926E-16, -9.812499998634406140, -5.148502694627439702 ) ) ;
#2541=ORIENTED_EDGE ( 'NONE', *, *, #4646, .T. ) ;
#2542=CARTESIAN_POINT ( 'NONE',  ( 5.000000000000000000, -73.50000000000000000, -6.123233995736766282E-16 ) ) ;
#2545=CARTESIAN_POINT ( 'NONE',  ( 0.000000000000000000, -170.0000000000000000, 0.000000000000000000 ) ) ;
#2546=CARTESIAN_POINT ( 'NONE',  ( 2.500000000000002220, -77.54166666393547303, 4.330127018922192761 ) ) ;
#2548=ORIENTED_EDGE ( 'NONE', *, *, #10235, .T. ) ;
#2550=CARTESIAN_POINT ( 'NONE',  ( 4.458734124999998549, -15.97916666530107221, -2.574251347313721627 ) ) ;
#2551=CARTESIAN_POINT ( 'NONE',  ( -2.229367062499996610, -51.39583333196773651, 3.861377020970582219 ) ) ;
#2553=PRESENTATION_STYLE_ASSIGNMENT (( #31807 ) ) ;
#2554=CARTESIAN_POINT ( 'NONE',  ( -4.458734125000001214, -139.8750000013656063, 1.846868145590734089 ) ) ;
#2557=VERTEX_POINT ( 'NONE', #32302 ) ;
#2563=CARTESIAN_POINT ( 'NONE',  ( 4.458734125000000326, -148.6250000013655779, -1.846868145590734978 ) ) ;
#2567=CARTESIAN_POINT ( 'NONE',  ( 9.457646018065525792E-16, -61.31249999863440792, 5.148502694627439702 ) ) ;
#2568=CARTESIAN_POINT ( 'NONE',  ( -5.000000000000000888, -154.6875000027312126, -2.071067811865475949 ) ) ;
#2570=CARTESIAN_POINT ( 'NONE',  ( 4.458734124999997661, -146.5000000013656347, 1.846868145590737864 ) ) ;
#2577=CARTESIAN_POINT ( 'NONE',  ( 0.000000000000000000, -170.0000000000000000, 0.000000000000000000 ) ) ;
#2579=CARTESIAN_POINT ( 'NONE',  ( 4.458734124999998549, 28.02083333469893134, -2.574251347313721627 ) ) ;
#2580=DIRECTION ( 'NONE',  ( -0.000000000000000000, 1.000000000000000000, -0.000000000000000000 ) ) ;
#2586=CARTESIAN_POINT ( 'NONE',  ( 4.458734124999998549, 9.270833334698927786, -2.574251347313721627 ) ) ;
#2588=CARTESIAN_POINT ( 'NONE',  ( -3.152548672688508926E-16, -19.81249999863440081, -5.148502694627439702 ) ) ;
#2590=CARTESIAN_POINT ( 'NONE',  ( -3.152801135295367985, -160.8125000013656063, 3.152801135295367096 ) ) ;
#2591=CARTESIAN_POINT ( 'NONE',  ( 5.000000000000000888, 15.54166666939785202, 2.886751345948126879 ) ) ;
#2595=CARTESIAN_POINT ( 'NONE',  ( -2.500000000000000444, -36.16666666666666430, -4.330127018922193649 ) ) ;
#2596=CARTESIAN_POINT ( 'NONE',  ( 4.458734125000000326, -39.89583333196772941, 2.574251347313718519 ) ) ;
#2597=CARTESIAN_POINT ( 'NONE',  ( -2.229367062499996610, -68.39583333196773651, 3.861377020970582219 ) ) ;
#2602=CARTESIAN_POINT ( 'NONE',  ( -2.500000000000000444, -85.16666666666667140, -4.330127018922193649 ) ) ;
#2604=CARTESIAN_POINT ( 'NONE',  ( -2.500000000000000444, -68.04166666393547303, -4.330127018922193649 ) ) ;
#2605=CARTESIAN_POINT ( 'NONE',  ( -4.999999999999999112, -6.916666666666667851, 2.886751345948131764 ) ) ;
#2606=CARTESIAN_POINT ( 'NONE',  ( 4.458734124999998549, -71.72916666530107932, -2.574251347313721627 ) ) ;
#2609=CARTESIAN_POINT ( 'NONE',  ( 1.060575238724906964E-15, -13.62499999726881050, 5.773502691896257311 ) ) ;
#2610=CARTESIAN_POINT ( 'NONE',  ( -4.458734124999999437, -41.31249999863440081, 0.000000000000000000 ) ) ;
#2611=VERTEX_POINT ( 'NONE', #13635 ) ;
#2613=CARTESIAN_POINT ( 'NONE',  ( 4.458734124999999437, 9.937500001365593860, -5.460374474430324690E-16 ) ) ;
#2614=ORIENTED_EDGE ( 'NONE', *, *, #24363, .T. ) ;
#2615=CARTESIAN_POINT ( 'NONE',  ( -6.972266317189433020E-16, -53.24999999999999289, -5.000000000000000000 ) ) ;
#2616=CARTESIAN_POINT ( 'NONE',  ( 2.499999999999998668, -53.33333333333332860, -4.330127018922193649 ) ) ;
#2617=CARTESIAN_POINT ( 'NONE',  ( 1.846868145590735200, -160.5000000013656347, -4.458734125000000326 ) ) ;
#2619=CARTESIAN_POINT ( 'NONE',  ( 0.000000000000000000, -170.0000000000000000, 5.000000000000000000 ) ) ;
#2620=CARTESIAN_POINT ( 'NONE',  ( 4.458734124999999437, -80.81249999863440792, -5.460374474430324690E-16 ) ) ;
#2621=CARTESIAN_POINT ( 'NONE',  ( -5.000000000000000888, -165.4375000000000000, 2.071067811865474617 ) ) ;
#2622=CARTESIAN_POINT ( 'NONE',  ( -4.458734124999998549, -88.22916666530107932, 2.574251347313722516 ) ) ;
#2623=ADVANCED_FACE ( 'NONE', ( #52248 ), #45910, .T. ) ;
#2625=CARTESIAN_POINT ( 'NONE',  ( 4.458734125000001214, -1.145833331967740509, 2.574251347313718519 ) ) ;
#2626=CARTESIAN_POINT ( 'NONE',  ( 4.458734124999998549, -36.97916666530107221, -2.574251347313721627 ) ) ;
#2629=CARTESIAN_POINT ( 'NONE',  ( -5.000000000000000000, 16.12500000273118417, 0.000000000000000000 ) ) ;
#2630=ORIENTED_EDGE ( 'NONE', *, *, #56762, .F. ) ;
#2631=LINE ( 'NONE', #27695, #20357 ) ;
#2633=CARTESIAN_POINT ( 'NONE',  ( 4.458734124999998549, -71.97916666530107932, -2.574251347313721627 ) ) ;
#2636=VECTOR ( 'NONE', #36962, 1000.000000000000000 ) ;
#2637=CARTESIAN_POINT ( 'NONE',  ( 2.500000000000002220, -5.666666666666666963, 4.330127018922192761 ) ) ;
#2641=CARTESIAN_POINT ( 'NONE',  ( 2.229367062500001939, 5.020833334698926897, 3.861377020970579999 ) ) ;
#2642=CARTESIAN_POINT ( 'NONE',  ( -2.499999999999996447, -32.70833333060215153, 4.330127018922195425 ) ) ;
#2643=CARTESIAN_POINT ( 'NONE',  ( 1.846868145590735200, -155.2500000013656063, -4.458734124999999437 ) ) ;
#2655=CARTESIAN_POINT ( 'NONE',  ( 4.458734125000000326, 22.10416666803225993, 2.574251347313718519 ) ) ;
#2657=CARTESIAN_POINT ( 'NONE',  ( -2.229367062499996610, -5.395833331967740953, 3.861377020970582219 ) ) ;
#2660=CARTESIAN_POINT ( 'NONE',  ( 2.071067811865476394, -143.3125000027312126, 5.000000000000000000 ) ) ;
#2661=CARTESIAN_POINT ( 'NONE',  ( 5.000000000000000000, -159.0625000000000284, 2.071067811865478614 ) ) ;
#2666=CARTESIAN_POINT ( 'NONE',  ( -4.999999999999998224, -87.91666666666667140, 2.886751345948131764 ) ) ;
#2668=CARTESIAN_POINT ( 'NONE',  ( -3.152801135295367096, -163.3125000013656063, -3.152801135295367541 ) ) ;
#2672=CARTESIAN_POINT ( 'NONE',  ( 9.457646018065525792E-16, 15.68750000136559386, 5.148502694627439702 ) ) ;
#2679=CARTESIAN_POINT ( 'NONE',  ( 1.060575238724906964E-15, 10.24999999999999822, 5.773502691896257311 ) ) ;
#2680=CARTESIAN_POINT ( 'NONE',  ( -2.229367062499996610, -56.14583333196773651, 3.861377020970582219 ) ) ;
#2686=FACE_OUTER_BOUND ( 'NONE', #1104, .T. ) ;
#2687=CYLINDRICAL_SURFACE ( 'NONE', #7363, 5.000000000000000000 ) ;
#2688=CARTESIAN_POINT ( 'NONE',  ( 2.500000000000002220, -40.66666666666667140, 4.330127018922192761 ) ) ;
#2689=CARTESIAN_POINT ( 'NONE',  ( 3.535533905932736864, -149.1250000000000000, 3.535533905932738641 ) ) ;
#2690=CARTESIAN_POINT ( 'NONE',  ( -4.999999999999998224, -47.91666666666667140, 2.886751345948131764 ) ) ;
#2692=CARTESIAN_POINT ( 'NONE',  ( -5.000000000000000888, -143.5625000000000568, -2.071067811865475949 ) ) ;
#2693=CARTESIAN_POINT ( 'NONE',  ( 4.458734125000001214, -62.89583333196775072, 2.574251347313718519 ) ) ;
#2694=CARTESIAN_POINT ( 'NONE',  ( 4.458734124999999437, -150.6875000013656063, 0.000000000000000000 ) ) ;
#2695=CARTESIAN_POINT ( 'NONE',  ( -4.458734124999998549, -71.22916666530106511, 2.574251347313722516 ) ) ;
#2698=CARTESIAN_POINT ( 'NONE',  ( -2.229367062499996610, -20.39583333196774007, 3.861377020970582219 ) ) ;
#2699=CARTESIAN_POINT ( 'NONE',  ( -2.500000000000000444, -62.04166666393547303, -4.330127018922193649 ) ) ;
#2706=CARTESIAN_POINT ( 'NONE',  ( 4.458734124999999437, -151.5000000013655779, 1.846868145590737864 ) ) ;
#2707=VERTEX_POINT ( 'NONE', #13002 ) ;
#2711=CARTESIAN_POINT ( 'NONE',  ( 2.229367062499998831, -54.89583333196773651, -3.861377020970580887 ) ) ;
#2713=EDGE_CURVE ( 'NONE', #51834, #61074, #13321, .T. ) ;
#2715=EDGE_CURVE ( 'NONE', #21692, #17887, #31115, .T. ) ;
#2717=CARTESIAN_POINT ( 'NONE',  ( -2.229367062499996610, 23.85416666803225993, 3.861377020970582219 ) ) ;
#2719=CARTESIAN_POINT ( 'NONE',  ( -4.458734124999999437, -169.0000000013655779, -1.846868145590735644 ) ) ;
#2728=CARTESIAN_POINT ( 'NONE',  ( 5.000000000000000000, -69.29166666393547303, -2.886751345948130876 ) ) ;
#2731=CARTESIAN_POINT ( 'NONE',  ( -6.972266317189433020E-16, -77.12499999726881583, -5.000000000000000000 ) ) ;
#2735=ORIENTED_EDGE ( 'NONE', *, *, #20076, .F. ) ;
#2736=CARTESIAN_POINT ( 'NONE',  ( -5.000000000000000000, -4.874999997268810503, 0.000000000000000000 ) ) ;
#2738=CARTESIAN_POINT ( 'NONE',  ( -5.000000000000000000, -153.6250000027312126, -6.123233995736766282E-16 ) ) ;
#2744=CARTESIAN_POINT ( 'NONE',  ( 2.071067811865476394, -146.1875000000000284, 5.000000000000000000 ) ) ;
#2745=EDGE_CURVE ( 'NONE', #1059, #23096, #39273, .T. ) ;
#2749=CARTESIAN_POINT ( 'NONE',  ( 4.458734125000000326, -24.89583333196773651, 2.574251347313718519 ) ) ;
#2753=CARTESIAN_POINT ( 'NONE',  ( 1.846868145590735200, -151.2500000013656063, -4.458734125000000326 ) ) ;
#2755=CARTESIAN_POINT ( 'NONE',  ( -4.458734124999999437, -49.64583333196772941, -2.574251347313719407 ) ) ;
#2756=CYLINDRICAL_SURFACE ( 'NONE', #57184, 5.000000000000000000 ) ;
#2758=CARTESIAN_POINT ( 'NONE',  ( 2.500000000000002220, 25.33333333333333215, 4.330127018922192761 ) ) ;
#2759=CARTESIAN_POINT ( 'NONE',  ( -6.972266317189433020E-16, 7.750000000000000000, -5.000000000000000000 ) ) ;
#2760=CARTESIAN_POINT ( 'NONE',  ( -4.458734124999998549, -0.2291666653010705768, 2.574251347313722516 ) ) ;
#2764=CARTESIAN_POINT ( 'NONE',  ( 4.458734124999998549, 15.02083333469892601, -2.574251347313721627 ) ) ;
#2765=CARTESIAN_POINT ( 'NONE',  ( -4.999999999999999112, 5.208333336064518981, 2.886751345948131764 ) ) ;
#2768=ORIENTED_EDGE ( 'NONE', *, *, #17370, .T. ) ;
#2770=CARTESIAN_POINT ( 'NONE',  ( -2.499999999999996447, -23.70833333060214443, 4.330127018922195425 ) ) ;
#2771=CARTESIAN_POINT ( 'NONE',  ( -3.152548672688508926E-16, -50.56249999863440792, -5.148502694627439702 ) ) ;
#2772=CARTESIAN_POINT ( 'NONE',  ( 4.458734124999999437, -163.6875000013655779, 0.000000000000000000 ) ) ;
#2773=ADVANCED_FACE ( 'NONE', ( #21478 ), #57710, .T. ) ;
#2775=CARTESIAN_POINT ( 'NONE',  ( -3.535250795749689387E-16, -46.12499999726881583, -5.773502691896257311 ) ) ;
#2777=ORIENTED_EDGE ( 'NONE', *, *, #27801, .T. ) ;
#2778=CARTESIAN_POINT ( 'NONE',  ( -4.458734124999999437, -22.31249999863440436, 0.000000000000000000 ) ) ;
#2779=ORIENTED_EDGE ( 'NONE', *, *, #35022, .F. ) ;
#2780=CARTESIAN_POINT ( 'NONE',  ( 5.000000000000000888, -85.58333333333332860, 2.886751345948126879 ) ) ;
#2781=CARTESIAN_POINT ( 'NONE',  ( -8.190561711645485556E-16, -162.6875000013655779, 4.458734124999999437 ) ) ;
#2784=CARTESIAN_POINT ( 'NONE',  ( -4.458734124999999437, -34.64583333196773651, -2.574251347313719407 ) ) ;
#2785=CARTESIAN_POINT ( 'NONE',  ( -2.498395430326213474E-14, 20.37500000273118062, 5.000000000000000000 ) ) ;
#2786=VERTEX_POINT ( 'NONE', #4602 ) ;
#2787=( BOUNDED_CURVE ( )  B_SPLINE_CURVE ( 2, ( #37216, #12125, #52328, #56842, #41071, #47485, #2808, #51056, #7000 ),
 .UNSPECIFIED., .F., .F. ) 
 B_SPLINE_CURVE_WITH_KNOTS ( ( 3, 2, 2, 2, 3 ),
 ( 0.8562499999999999556, 0.8569444444444443976, 0.8583333333333332815, 0.8597222222222222765, 0.8604166666666667185 ),
 .UNSPECIFIED. ) 
 CURVE ( )  GEOMETRIC_REPRESENTATION_ITEM ( )  RATIONAL_B_SPLINE_CURVE ( ( 0.9330127018922194093, 0.9330127018922194093, 1.000000000000000000, 0.8660254037844387076, 1.000000000000000000, 0.8660254037844387076, 1.000000000000000000, 0.9330127018922194093, 0.9330127018922194093 ) ) 
 REPRESENTATION_ITEM ( '' )  );
#2792=VERTEX_POINT ( 'NONE', #19715 ) ;
#2793=DIRECTION ( 'NONE',  ( -0.000000000000000000, 1.000000000000000000, -0.000000000000000000 ) ) ;
#2795=CARTESIAN_POINT ( 'NONE',  ( -4.458734124999999437, -78.64583333196773651, -2.574251347313719407 ) ) ;
#2798=CARTESIAN_POINT ( 'NONE',  ( -6.972266317189433020E-16, -9.250000000000000000, -5.000000000000000000 ) ) ;
#2799=CARTESIAN_POINT ( 'NONE',  ( 2.071067811865560326, -144.9375000027311842, -4.999999999999914735 ) ) ;
#2801=CARTESIAN_POINT ( 'NONE',  ( -1.339745962155613812, -85.08034179853028434, -5.000000000000000000 ) ) ;
#2808=CARTESIAN_POINT ( 'NONE',  ( -2.500000000000000444, -73.16666666666665719, -4.330127018922193649 ) ) ;
#2810=CARTESIAN_POINT ( 'NONE',  ( 2.229367062500001939, -80.22916666530106511, 3.861377020970579999 ) ) ;
#2813=ORIENTED_EDGE ( 'NONE', *, *, #32159, .F. ) ;
#2815=CARTESIAN_POINT ( 'NONE',  ( 0.000000000000000000, -170.0000000000000000, 5.000000000000000000 ) ) ;
#2817=CARTESIAN_POINT ( 'NONE',  ( 3.535533905932736864, -164.2500000027312126, 3.535533905932738641 ) ) ;
#2819=STYLED_ITEM('',(#63698),#7586);
#2820=CARTESIAN_POINT ( 'NONE',  ( 9.457646018065525792E-16, 12.68750000136559208, 5.148502694627439702 ) ) ;
#2829=CARTESIAN_POINT ( 'NONE',  ( 9.457646018065525792E-16, -8.062499998634404363, 5.148502694627439702 ) ) ;
#2832=CARTESIAN_POINT ( 'NONE',  ( -2.229367062499996610, -34.39583333196772941, 3.861377020970582219 ) ) ;
#2837=CARTESIAN_POINT ( 'NONE',  ( -4.458734124999999437, -149.1875000013656063, -5.460374474430324690E-16 ) ) ;
#2838=CARTESIAN_POINT ( 'NONE',  ( -2.229367062500000163, 17.52083333469892779, -3.861377020970580443 ) ) ;
#2841=CARTESIAN_POINT ( 'NONE',  ( -4.458734124999997661, -82.47916666530106511, 2.574251347313722516 ) ) ;
#2844=CARTESIAN_POINT ( 'NONE',  ( 5.000000000000000888, 16.54166666939785202, 2.886751345948126879 ) ) ;
#2849=CARTESIAN_POINT ( 'NONE',  ( 2.500000000000002220, -21.66666666666666785, 4.330127018922192761 ) ) ;
#2850=CARTESIAN_POINT ( 'NONE',  ( -3.152548672688508926E-16, -25.56249999863440436, -5.148502694627439702 ) ) ;
#2852=ADVANCED_FACE ( 'NONE', ( #39324 ), #58956, .T. ) ;
#2853=CARTESIAN_POINT ( 'NONE',  ( -4.999999999999999112, -28.79166666393548013, 2.886751345948131764 ) ) ;
#2854=CARTESIAN_POINT ( 'NONE',  ( 4.458734124999998549, -61.72916666530106511, -2.574251347313721627 ) ) ;
#2857=CARTESIAN_POINT ( 'NONE',  ( -3.152548672688508926E-16, -10.81249999863440792, -5.148502694627439702 ) ) ;
#2858=EDGE_LOOP ( 'NONE', ( #51614, #47847, #21108, #28499 ) ) ;
#2859=CARTESIAN_POINT ( 'NONE',  ( 5.000000000000000888, -69.58333333333332860, 2.886751345948126879 ) ) ;
#2862=( BOUNDED_CURVE ( )  B_SPLINE_CURVE ( 2, ( #8989, #13814, #33746, #53363, #39511, #63346, #14749, #23478, #43081 ),
 .UNSPECIFIED., .F., .F. ) 
 B_SPLINE_CURVE_WITH_KNOTS ( ( 3, 2, 2, 2, 3 ),
 ( 0.8604166666666667185, 0.8611111111111111605, 0.8625000000000000444, 0.8638888888888889284, 0.8645833333333333703 ),
 .UNSPECIFIED. ) 
 CURVE ( )  GEOMETRIC_REPRESENTATION_ITEM ( )  RATIONAL_B_SPLINE_CURVE ( ( 0.9330127018922194093, 0.9330127018922194093, 1.000000000000000000, 0.8660254037844387076, 1.000000000000000000, 0.8660254037844387076, 1.000000000000000000, 0.9330127018922194093, 0.9330127018922194093 ) ) 
 REPRESENTATION_ITEM ( '' )  );
#2865=CARTESIAN_POINT ( 'NONE',  ( -5.000000000000000000, -74.95833333060214443, -2.886751345948128211 ) ) ;
#2866=CARTESIAN_POINT ( 'NONE',  ( -6.972266317189433020E-16, -86.25000000000001421, -5.000000000000000000 ) ) ;
#2867=VERTEX_POINT ( 'NONE', #53808 ) ;
#2869=VECTOR ( 'NONE', #6150, 1000.000000000000000 ) ;
#2870=EDGE_CURVE ( 'NONE', #45174, #20081, #52824, .T. ) ;
#2871=CARTESIAN_POINT ( 'NONE',  ( 2.229367062499998831, -13.89583333196774184, -3.861377020970580887 ) ) ;
#2872=ADVANCED_FACE ( 'NONE', ( #4299 ), #23612, .T. ) ;
#2873=CARTESIAN_POINT ( 'NONE',  ( 9.457646018065525792E-16, -58.31249999863440792, 5.148502694627439702 ) ) ;
#2874=CARTESIAN_POINT ( 'NONE',  ( 1.975475456537005874E-15, -23.75000000000000000, 5.000000000000000000 ) ) ;
#2876=CARTESIAN_POINT ( 'NONE',  ( -3.152801135295367985, -169.0625000013656063, 3.152801135295367096 ) ) ;
#2878=CARTESIAN_POINT ( 'NONE',  ( 5.000000000000000000, -148.1875000027312126, 2.071067811865478614 ) ) ;
#2879=ORIENTED_EDGE ( 'NONE', *, *, #15258, .F. ) ;
#2883=EDGE_CURVE ( 'NONE', #30981, #63093, #28573, .T. ) ;
#2888=CARTESIAN_POINT ( 'NONE',  ( 3.152801135295367541, -146.5625000013655779, -3.152801135295367541 ) ) ;
#2892=CARTESIAN_POINT ( 'NONE',  ( 4.458734125000001214, -61.14583333196773651, 2.574251347313718519 ) ) ;
#2894=CYLINDRICAL_SURFACE ( 'NONE', #47020, 5.000000000000000000 ) ;
#2895=CARTESIAN_POINT ( 'NONE',  ( 4.458734124999999437, -145.3750000013656063, -1.846868145590734978 ) ) ;
#2902=FACE_OUTER_BOUND ( 'NONE', #19370, .T. ) ;
#2904=CARTESIAN_POINT ( 'NONE',  ( 2.229367062500001939, 27.77083333469892779, 3.861377020970579999 ) ) ;
#2905=CARTESIAN_POINT ( 'NONE',  ( 0.000000000000000000, -170.0000000000000000, 0.000000000000000000 ) ) ;
#2909=FACE_OUTER_BOUND ( 'NONE', #15655, .T. ) ;
#2910=CARTESIAN_POINT ( 'NONE',  ( -4.458734124999997661, 8.770833334698927786, 2.574251347313722516 ) ) ;
#2912=CARTESIAN_POINT ( 'NONE',  ( 9.457646018065525792E-16, -17.31249999863440792, 5.148502694627439702 ) ) ;
#2916=CARTESIAN_POINT ( 'NONE',  ( 1.846868145590736310, -158.6250000013655779, 4.458734124999999437 ) ) ;
#2917=CARTESIAN_POINT ( 'NONE',  ( -9.184850993605147944E-16, -158.2500000000000000, 5.000000000000000000 ) ) ;
#2921=CARTESIAN_POINT ( 'NONE',  ( 2.229367062499998831, -41.64583333196773651, -3.861377020970580887 ) ) ;
#2922=CARTESIAN_POINT ( 'NONE',  ( 1.339745962155612702, 19.83034180399266688, -5.000000000000000000 ) ) ;
#2923=CARTESIAN_POINT ( 'NONE',  ( -4.458734124999999437, -69.64583333196773651, -2.574251347313719407 ) ) ;
#2929=CARTESIAN_POINT ( 'NONE',  ( 6.123233995736766282E-16, -170.0000000000000000, -5.000000000000000000 ) ) ;
#2930=CARTESIAN_POINT ( 'NONE',  ( 1.060575238724906964E-15, -5.749999999999998224, 5.773502691896257311 ) ) ;
#2931=CARTESIAN_POINT ( 'NONE',  ( 2.229367062500001939, -70.97916666530107932, 3.861377020970579999 ) ) ;
#2934=CARTESIAN_POINT ( 'NONE',  ( -3.535250795749689387E-16, -14.12499999726881050, -5.773502691896257311 ) ) ;
#2935=CARTESIAN_POINT ( 'NONE',  ( 2.229367062500001939, -46.97916666530106511, 3.861377020970579999 ) ) ;
#2936=ORIENTED_EDGE ( 'NONE', *, *, #22841, .T. ) ;
#2937=CARTESIAN_POINT ( 'NONE',  ( 5.000000000000000000, -41.49999999999999289, -6.123233995736766282E-16 ) ) ;
#2938=CARTESIAN_POINT ( 'NONE',  ( -3.152548672688508926E-16, 5.187500001365592972, -5.148502694627439702 ) ) ;
#2939=ORIENTED_EDGE ( 'NONE', *, *, #37679, .T. ) ;
#2940=CARTESIAN_POINT ( 'NONE',  ( 3.061616997868383141E-16, -151.7500000000000284, -5.000000000000000000 ) ) ;
#2941=CARTESIAN_POINT ( 'NONE',  ( -5.000000000000000000, -55.08333333333332860, -2.886751345948128211 ) ) ;
#2942=CARTESIAN_POINT ( 'NONE',  ( -4.458734125000000326, -161.2500000013655779, -1.846868145590735644 ) ) ;
#2945=CARTESIAN_POINT ( 'NONE',  ( -2.229367062500000163, -80.47916666530106511, -3.861377020970580443 ) ) ;
#2946=CARTESIAN_POINT ( 'NONE',  ( -5.000000000000000888, -167.4375000000000284, 2.071067811865474617 ) ) ;
#2947=CARTESIAN_POINT ( 'NONE',  ( -3.152548672688508926E-16, -87.56249999863440792, -5.148502694627439702 ) ) ;
#2949=CARTESIAN_POINT ( 'NONE',  ( 4.458734125000001214, 0.8541666680322613781, 2.574251347313718519 ) ) ;
#2950=CARTESIAN_POINT ( 'NONE',  ( 4.458734124999999437, -39.06249999863440081, -5.460374474430324690E-16 ) ) ;
#2951=CARTESIAN_POINT ( 'NONE',  ( -2.500000000000000444, 23.95833333606451987, -4.330127018922193649 ) ) ;
#2953=CARTESIAN_POINT ( 'NONE',  ( -1.339745962155610925, 16.33034180399266333, 5.000000000000000000 ) ) ;
#2958=CARTESIAN_POINT ( 'NONE',  ( -2.229367062499996610, -72.39583333196773651, 3.861377020970582219 ) ) ;
#2967=CARTESIAN_POINT ( 'NONE',  ( 9.457646018065525792E-16, 0.9375000013655959696, 5.148502694627439702 ) ) ;
#2968=CARTESIAN_POINT ( 'NONE',  ( -4.999999999999998224, -75.91666666666665719, 2.886751345948131764 ) ) ;
#2969=CARTESIAN_POINT ( 'NONE',  ( 2.730187237215162345E-16, -155.1875000013655779, -4.458734124999999437 ) ) ;
#2971=ORIENTED_EDGE ( 'NONE', *, *, #32783, .T. ) ;
#2973=CARTESIAN_POINT ( 'NONE',  ( -2.499999999999996447, -46.83333333333333570, 4.330127018922195425 ) ) ;
#2975=FACE_OUTER_BOUND ( 'NONE', #41973, .T. ) ;
#2977=CARTESIAN_POINT ( 'NONE',  ( 5.000000000000000000, -67.50000000000000000, -6.123233995736766282E-16 ) ) ;
#2982=CARTESIAN_POINT ( 'NONE',  ( -2.229367062499996610, 22.85416666803225993, 3.861377020970582219 ) ) ;
#2984=CARTESIAN_POINT ( 'NONE',  ( 2.229367062499998831, -4.895833331967740065, -3.861377020970580887 ) ) ;
#2985=CARTESIAN_POINT ( 'NONE',  ( 2.500000000000002220, -0.5416666639354792423, 4.330127018922192761 ) ) ;
#2987=CARTESIAN_POINT ( 'NONE',  ( -5.000000000000000888, -141.5625000027312126, 2.071067811865474617 ) ) ;
#2992=( BOUNDED_CURVE ( )  B_SPLINE_CURVE ( 2, ( #61025, #56194, #7312, #27231, #25962, #11791, #15993, #31740, #46541 ),
 .UNSPECIFIED., .F., .F. ) 
 B_SPLINE_CURVE_WITH_KNOTS ( ( 3, 2, 2, 2, 3 ),
 ( 0.9437499999999999778, 0.9444444444444444198, 0.9458333333333333037, 0.9472222222222221877, 0.9479166666666666297 ),
 .UNSPECIFIED. ) 
 CURVE ( )  GEOMETRIC_REPRESENTATION_ITEM ( )  RATIONAL_B_SPLINE_CURVE ( ( 0.9330127018922194093, 0.9330127018922194093, 1.000000000000000000, 0.8660254037844387076, 1.000000000000000000, 0.8660254037844387076, 1.000000000000000000, 0.9330127018922194093, 0.9330127018922194093 ) ) 
 REPRESENTATION_ITEM ( '' )  );
#2996=CARTESIAN_POINT ( 'NONE',  ( 3.152801135295366208, -156.8125000013656063, 3.152801135295367985 ) ) ;
#3000=CARTESIAN_POINT ( 'NONE',  ( 2.229367062500001939, 18.77083333469892779, 3.861377020970579999 ) ) ;
#3001=EDGE_LOOP ( 'NONE', ( #31996, #50141, #52598, #35426 ) ) ;
#3005=CARTESIAN_POINT ( 'NONE',  ( 1.339745962155612702, -16.29465819873851729, -5.000000000000000000 ) ) ;
#3006=CARTESIAN_POINT ( 'NONE',  ( 2.500000000000002220, 10.33333333333333393, 4.330127018922192761 ) ) ;
#3008=CARTESIAN_POINT ( 'NONE',  ( 9.457646018065525792E-16, -58.06249999863440081, 5.148502694627439702 ) ) ;
#3009=CARTESIAN_POINT ( 'NONE',  ( -5.000000000000000000, -52.87499999726881583, 0.000000000000000000 ) ) ;
#3011=CARTESIAN_POINT ( 'NONE',  ( 0.000000000000000000, -170.0000000000000000, 0.000000000000000000 ) ) ;
#3015=CARTESIAN_POINT ( 'NONE',  ( -2.499999999999996447, -41.83333333333333570, 4.330127018922195425 ) ) ;
#3016=CARTESIAN_POINT ( 'NONE',  ( 0.000000000000000000, -170.0000000000000000, 0.000000000000000000 ) ) ;
#3020=CARTESIAN_POINT ( 'NONE',  ( 4.458734125000001214, -66.89583333196773651, 2.574251347313718519 ) ) ;
#3021=CARTESIAN_POINT ( 'NONE',  ( 4.458734124999999437, -146.7500000013656063, 1.846868145590737864 ) ) ;
#3022=CARTESIAN_POINT ( 'NONE',  ( -3.152548672688508926E-16, -70.56249999863439371, -5.148502694627439702 ) ) ;
#3024=CARTESIAN_POINT ( 'NONE',  ( 4.458734124999999437, -21.06249999863440436, -5.460374474430324690E-16 ) ) ;
#3025=CARTESIAN_POINT ( 'NONE',  ( -3.535250795749689387E-16, -61.12499999726880873, -5.773502691896257311 ) ) ;
#3026=EDGE_LOOP ( 'NONE', ( #61086, #11746, #10990, #62857 ) ) ;
#3027=CARTESIAN_POINT ( 'NONE',  ( -5.000000000000000000, -150.5000000000000284, -6.123233995736766282E-16 ) ) ;
#3032=CARTESIAN_POINT ( 'NONE',  ( 2.071067811865645591, -155.3125000027311557, 4.999999999999830358 ) ) ;
#3035=CARTESIAN_POINT ( 'NONE',  ( 4.458734124999998549, -52.97916666530107932, -2.574251347313721627 ) ) ;
#3039=( BOUNDED_CURVE ( )  B_SPLINE_CURVE ( 2, ( #29731, #490, #20093, #40587, #60232, #35777, #55399, #11316, #18043 ),
 .UNSPECIFIED., .F., .F. ) 
 B_SPLINE_CURVE_WITH_KNOTS ( ( 3, 2, 2, 2, 3 ),
 ( 0.2104166666666666685, 0.2111111111111111105, 0.2124999999999999944, 0.2138888888888888784, 0.2145833333333333481 ),
 .UNSPECIFIED. ) 
 CURVE ( )  GEOMETRIC_REPRESENTATION_ITEM ( )  RATIONAL_B_SPLINE_CURVE ( ( 0.9330127018922194093, 0.9330127018922194093, 1.000000000000000000, 0.8660254037844387076, 1.000000000000000000, 0.8660254037844387076, 1.000000000000000000, 0.9330127018922180770, 0.9330127018922194093 ) ) 
 REPRESENTATION_ITEM ( '' )  );
#3040=CARTESIAN_POINT ( 'NONE',  ( 2.229367062499998831, 19.35416666803225993, -3.861377020970580887 ) ) ;
#3046=CARTESIAN_POINT ( 'NONE',  ( -1.339745962155610925, -39.79465819873851729, 5.000000000000000000 ) ) ;
#3053=CARTESIAN_POINT ( 'NONE',  ( -5.000000000000000888, -139.6875000027311842, -2.071067811865475949 ) ) ;
#3058=CARTESIAN_POINT ( 'NONE',  ( -1.339745962155610925, -4.669658196007337558, 5.000000000000000000 ) ) ;
#3060=CARTESIAN_POINT ( 'NONE',  ( 3.535533905932736864, -154.2500000027312126, 3.535533905932738641 ) ) ;
#3067=CARTESIAN_POINT ( 'NONE',  ( -5.000000000000000888, -145.4375000000000000, 2.071067811865474617 ) ) ;
#3070=CARTESIAN_POINT ( 'NONE',  ( 2.499999999999998668, 22.79166666939785202, -4.330127018922193649 ) ) ;
#3071=CARTESIAN_POINT ( 'NONE',  ( 4.458734125000000326, -22.89583333196773651, 2.574251347313718519 ) ) ;
#3075=CARTESIAN_POINT ( 'NONE',  ( 4.458734124999999437, -147.4375000013656063, 0.000000000000000000 ) ) ;
#3076=ORIENTED_EDGE ( 'NONE', *, *, #62096, .F. ) ;
#3078=CARTESIAN_POINT ( 'NONE',  ( 4.458734125000000326, -50.14583333196772230, 2.574251347313718519 ) ) ;
#3080=DIRECTION ( 'NONE',  ( -0.000000000000000000, 1.000000000000000000, -0.000000000000000000 ) ) ;
#3081=CARTESIAN_POINT ( 'NONE',  ( -3.535250795749689387E-16, 24.75000000000000355, -5.773502691896257311 ) ) ;
#3083=CARTESIAN_POINT ( 'NONE',  ( -4.458734124999999437, -0.3124999986344051406, 0.000000000000000000 ) ) ;
#3085=CARTESIAN_POINT ( 'NONE',  ( 1.339745962155615144, 19.29465819873852439, 4.999999999999999112 ) ) ;
#3087=CARTESIAN_POINT ( 'NONE',  ( -6.972266317189433020E-16, -74.25000000000000000, -5.000000000000000000 ) ) ;
#3088=CARTESIAN_POINT ( 'NONE',  ( 9.457646018065525792E-16, 7.687500001365596525, 5.148502694627439702 ) ) ;
#3091=ORIENTED_EDGE ( 'NONE', *, *, #41313, .T. ) ;
#3092=( BOUNDED_CURVE ( )  B_SPLINE_CURVE ( 2, ( #13625, #47713, #12985, #33243, #9109, #33866, #32610, #52236, #13929 ),
 .UNSPECIFIED., .F., .F. ) 
 B_SPLINE_CURVE_WITH_KNOTS ( ( 3, 2, 2, 2, 3 ),
 ( 0.06875000000000000555, 0.06944444444444444753, 0.07083333333333333148, 0.07222222222222221544, 0.07291666666666667129 ),
 .UNSPECIFIED. ) 
 CURVE ( )  GEOMETRIC_REPRESENTATION_ITEM ( )  RATIONAL_B_SPLINE_CURVE ( ( 0.9330127018922194093, 0.9330127018922200755, 1.000000000000000000, 0.8660254037844387076, 1.000000000000000000, 0.8660254037844387076, 1.000000000000000000, 0.9330127018922187432, 0.9330127018922194093 ) ) 
 REPRESENTATION_ITEM ( '' )  );
#3094=CARTESIAN_POINT ( 'NONE',  ( -3.152548672688508926E-16, -46.56249999863440792, -5.148502694627439702 ) ) ;
#3095=CARTESIAN_POINT ( 'NONE',  ( 4.458734125000000326, -159.6250000013656063, -1.846868145590734978 ) ) ;
#3097=CARTESIAN_POINT ( 'NONE',  ( 2.500000000000002220, -43.54166666393548013, 4.330127018922192761 ) ) ;
#3098=ORIENTED_EDGE ( 'NONE', *, *, #19331, .F. ) ;
#3099=CARTESIAN_POINT ( 'NONE',  ( -4.458734124999999437, -24.39583333196773651, -2.574251347313719407 ) ) ;
#3100=ORIENTED_EDGE ( 'NONE', *, *, #5883, .T. ) ;
#3102=CARTESIAN_POINT ( 'NONE',  ( -4.458734124999999437, -164.9375000013655779, -5.460374474430324690E-16 ) ) ;
#3103=CARTESIAN_POINT ( 'NONE',  ( 1.975475456537005874E-15, -12.74999999999999822, 5.000000000000000000 ) ) ;
#3105=CARTESIAN_POINT ( 'NONE',  ( 4.458734125000001214, -40.14583333196772941, 2.574251347313718519 ) ) ;
#3107=VERTEX_POINT ( 'NONE', #21320 ) ;
#3110=CARTESIAN_POINT ( 'NONE',  ( -2.499999999999996447, -28.70833333060214798, 4.330127018922195425 ) ) ;
#3113=CARTESIAN_POINT ( 'NONE',  ( 9.457646018065525792E-16, -84.31249999863437949, 5.148502694627439702 ) ) ;
#3115=CARTESIAN_POINT ( 'NONE',  ( 0.000000000000000000, -170.0000000000000000, 0.000000000000000000 ) ) ;
#3118=CARTESIAN_POINT ( 'NONE',  ( -4.999999999999998224, -71.79166666393547303, 2.886751345948131764 ) ) ;
#3121=CARTESIAN_POINT ( 'NONE',  ( 3.061616997868383141E-16, -158.8750000027311842, -5.000000000000000000 ) ) ;
#3124=DIRECTION ( 'NONE',  ( -0.000000000000000000, 1.000000000000000000, -0.000000000000000000 ) ) ;
#3126=CARTESIAN_POINT ( 'NONE',  ( -4.458734124999999437, -81.64583333196773651, -2.574251347313719407 ) ) ;
#3130=VERTEX_POINT ( 'NONE', #11648 ) ;
#3133=CARTESIAN_POINT ( 'NONE',  ( -9.184850993605147944E-16, -167.3750000027312126, 5.000000000000000000 ) ) ;
#3136=CARTESIAN_POINT ( 'NONE',  ( -3.152548672688508926E-16, 10.18750000136559208, -5.148502694627439702 ) ) ;
#3144=CARTESIAN_POINT ( 'NONE',  ( -5.000000000000000888, -152.5625000000000284, -2.071067811865475949 ) ) ;
#3145=CARTESIAN_POINT ( 'NONE',  ( 4.458734125000000326, -9.895833331967738289, 2.574251347313718519 ) ) ;
#3147=ORIENTED_EDGE ( 'NONE', *, *, #61347, .F. ) ;
#3148=CARTESIAN_POINT ( 'NONE',  ( 4.458734124999999437, -35.06249999863440792, -5.460374474430324690E-16 ) ) ;
#3154=CARTESIAN_POINT ( 'NONE',  ( 9.457646018065525792E-16, 13.93750000136559564, 5.148502694627439702 ) ) ;
#3158=CARTESIAN_POINT ( 'NONE',  ( -2.229367062500000163, -81.72916666530106511, -3.861377020970580443 ) ) ;
#3160=LINE ( 'NONE', #37555, #39787 ) ;
#3161=CARTESIAN_POINT ( 'NONE',  ( -5.000000000000000000, 19.04166666939785202, -2.886751345948128211 ) ) ;
#3166=CARTESIAN_POINT ( 'NONE',  ( -2.500000000000000444, -27.16666666666666430, -4.330127018922193649 ) ) ;
#3167=CARTESIAN_POINT ( 'NONE',  ( 4.458734125000001214, -30.89583333196773296, 2.574251347313718519 ) ) ;
#3170=CARTESIAN_POINT ( 'NONE',  ( -4.999999999999999112, -29.79166666393548368, 2.886751345948131764 ) ) ;
#3171=CARTESIAN_POINT ( 'NONE',  ( -4.458734124999999437, -61.31249999863440081, 0.000000000000000000 ) ) ;
#3174=CARTESIAN_POINT ( 'NONE',  ( 2.229367062499998831, -9.895833331967738289, -3.861377020970580887 ) ) ;
#3176=CARTESIAN_POINT ( 'NONE',  ( -2.500000000000000444, -76.16666666666665719, -4.330127018922193649 ) ) ;
#3178=VECTOR ( 'NONE', #16349, 1000.000000000000000 ) ;
#3180=CARTESIAN_POINT ( 'NONE',  ( 1.060575238724906964E-15, -74.62499999726880162, 5.773502691896257311 ) ) ;
#3181=CYLINDRICAL_SURFACE ( 'NONE', #41592, 5.000000000000000000 ) ;
#3182=ORIENTED_EDGE ( 'NONE', *, *, #38985, .T. ) ;
#3186=CARTESIAN_POINT ( 'NONE',  ( -4.458734124999999437, -19.64583333196774362, -2.574251347313719407 ) ) ;
#3187=CARTESIAN_POINT ( 'NONE',  ( -3.152548672688508926E-16, -58.81249999863440081, -5.148502694627439702 ) ) ;
#3188=ORIENTED_EDGE ( 'NONE', *, *, #35006, .T. ) ;
#3189=( BOUNDED_CURVE ( )  B_SPLINE_CURVE ( 2, ( #4670, #33948, #14009, #23050, #53256, #33013, #3435, #63229, #23680 ),
 .UNSPECIFIED., .F., .F. ) 
 B_SPLINE_CURVE_WITH_KNOTS ( ( 3, 2, 2, 2, 3 ),
 ( 0.9312500000000000222, 0.9319444444444444642, 0.9333333333333333481, 0.9347222222222222321, 0.9354166666666666741 ),
 .UNSPECIFIED. ) 
 CURVE ( )  GEOMETRIC_REPRESENTATION_ITEM ( )  RATIONAL_B_SPLINE_CURVE ( ( 0.9330127018922194093, 0.9330127018922194093, 1.000000000000000000, 0.8660254037844387076, 1.000000000000000000, 0.8660254037844387076, 1.000000000000000000, 0.9330127018922194093, 0.9330127018922194093 ) ) 
 REPRESENTATION_ITEM ( '' )  );
#3191=CARTESIAN_POINT ( 'NONE',  ( 4.458734124999999437, -139.5000000013655779, 1.846868145590737864 ) ) ;
#3197=CYLINDRICAL_SURFACE ( 'NONE', #58905, 5.000000000000000000 ) ;
#3200=CARTESIAN_POINT ( 'NONE',  ( 4.458734125000000326, -149.6250000013655779, -1.846868145590734978 ) ) ;
#3204=CARTESIAN_POINT ( 'NONE',  ( -4.458734124999998549, -64.47916666530106511, 2.574251347313722516 ) ) ;
#3205=CARTESIAN_POINT ( 'NONE',  ( 0.000000000000000000, -170.0000000000000000, 0.000000000000000000 ) ) ;
#3206=CARTESIAN_POINT ( 'NONE',  ( -6.972266317189433020E-16, -43.12499999726880873, -5.000000000000000000 ) ) ;
#3207=CARTESIAN_POINT ( 'NONE',  ( 3.152801135295366208, -146.5625000013655779, 3.152801135295367985 ) ) ;
#3209=ORIENTED_EDGE ( 'NONE', *, *, #53820, .F. ) ;
#3220=EDGE_CURVE ( 'NONE', #61158, #22662, #34388, .T. ) ;
#3222=CARTESIAN_POINT ( 'NONE',  ( 0.000000000000000000, -170.0000000000000000, 0.000000000000000000 ) ) ;
#3223=CARTESIAN_POINT ( 'NONE',  ( -5.000000000000000000, -15.00000000000000000, 0.000000000000000000 ) ) ;
#3225=CARTESIAN_POINT ( 'NONE',  ( 2.229367062500001939, 6.020833334698927786, 3.861377020970579999 ) ) ;
#3227=CARTESIAN_POINT ( 'NONE',  ( 4.458734125000000326, -19.14583333196774007, 2.574251347313718519 ) ) ;
#3229=CARTESIAN_POINT ( 'NONE',  ( -3.152801135295367096, -158.0625000013656063, -3.152801135295367541 ) ) ;
#3230=CARTESIAN_POINT ( 'NONE',  ( 1.339745962155609149, 23.29465819873852084, 5.000000000000003553 ) ) ;
#3235=CARTESIAN_POINT ( 'NONE',  ( 4.458734124999999437, -39.81249999863440081, -5.460374474430324690E-16 ) ) ;
#3238=CARTESIAN_POINT ( 'NONE',  ( 4.458734125000000326, -65.14583333196773651, 2.574251347313718519 ) ) ;
#3240=CARTESIAN_POINT ( 'NONE',  ( -1.339745962155610925, -40.79465819873852439, 5.000000000000000000 ) ) ;
#3241=EDGE_CURVE ( 'NONE', #14051, #10657, #38007, .T. ) ;
#3242=CARTESIAN_POINT ( 'NONE',  ( 2.071067811865645591, -152.3125000027312126, 4.999999999999830358 ) ) ;
#3244=CARTESIAN_POINT ( 'NONE',  ( -1.339745962155623360, 15.33034180399266333, 4.999999999999991118 ) ) ;
#3247=CARTESIAN_POINT ( 'NONE',  ( -3.535250795749689387E-16, -13.24999999999999822, -5.773502691896257311 ) ) ;
#3248=CARTESIAN_POINT ( 'NONE',  ( 2.229367062499998831, -18.64583333196774007, -3.861377020970580887 ) ) ;
#3250=CARTESIAN_POINT ( 'NONE',  ( 4.458734125000000326, -74.89583333196773651, 2.574251347313718519 ) ) ;
#3252=CARTESIAN_POINT ( 'NONE',  ( -2.499999999999996447, -11.70833333060214798, 4.330127018922195425 ) ) ;
#3253=CARTESIAN_POINT ( 'NONE',  ( 4.458734125000001214, -44.89583333196774362, 2.574251347313718519 ) ) ;
#3255=CARTESIAN_POINT ( 'NONE',  ( 5.000000000000000000, -144.0625000000000000, 2.071067811865478614 ) ) ;
#3256=CARTESIAN_POINT ( 'NONE',  ( -4.458734124999999437, 4.354166668032260823, -2.574251347313719407 ) ) ;
#3258=CARTESIAN_POINT ( 'NONE',  ( -2.071067811865604735, -151.3125000000000284, 4.999999999999872990 ) ) ;
#3259=CARTESIAN_POINT ( 'NONE',  ( 2.500000000000002220, -55.66666666666667140, 4.330127018922192761 ) ) ;
#3260=CARTESIAN_POINT ( 'NONE',  ( 3.152801135295367541, -158.5625000013656063, -3.152801135295367541 ) ) ;
#3262=CARTESIAN_POINT ( 'NONE',  ( 3.535533905932736864, -145.1250000000000000, 3.535533905932738641 ) ) ;
#3263=CARTESIAN_POINT ( 'NONE',  ( -4.458734124999999437, -79.31249999863440792, 0.000000000000000000 ) ) ;
#3264=CARTESIAN_POINT ( 'NONE',  ( -2.071067811865478170, -165.3125000000000284, 5.000000000000000000 ) ) ;
#3265=CARTESIAN_POINT ( 'NONE',  ( 1.339745962155612702, -11.29465819873852261, -5.000000000000000000 ) ) ;
#3267=CARTESIAN_POINT ( 'NONE',  ( 2.229367062499998831, -2.895833331967738289, -3.861377020970580887 ) ) ;
#3268=CARTESIAN_POINT ( 'NONE',  ( -2.229367062500000163, -41.72916666530107932, -3.861377020970580443 ) ) ;
#3269=CARTESIAN_POINT ( 'NONE',  ( -9.184850993605147944E-16, -151.3750000027311842, 5.000000000000000000 ) ) ;
#3271=CARTESIAN_POINT ( 'NONE',  ( -4.999999999999998224, 16.20833333606451987, 2.886751345948131764 ) ) ;
#3276=CARTESIAN_POINT ( 'NONE',  ( 4.458734125000001214, -71.14583333196773651, 2.574251347313718519 ) ) ;
#3278=EDGE_LOOP ( 'NONE', ( #3963, #17331, #27113 ) ) ;
#3279=CARTESIAN_POINT ( 'NONE',  ( 1.975475456537005874E-15, -5.750000000000000000, 5.000000000000000000 ) ) ;
#3282=CARTESIAN_POINT ( 'NONE',  ( -2.229367062500000163, 3.520833334698929118, -3.861377020970580443 ) ) ;
#3283=CARTESIAN_POINT ( 'NONE',  ( -1.339745962155613812, -43.20534180126148271, -5.000000000000000000 ) ) ;
#3284=CARTESIAN_POINT ( 'NONE',  ( -1.846868145590734756, -157.1250000013656063, -4.458734124999999437 ) ) ;
#3286=ORIENTED_EDGE ( 'NONE', *, *, #61844, .F. ) ;
#3288=CARTESIAN_POINT ( 'NONE',  ( -5.000000000000000000, -47.00000000000000000, 0.000000000000000000 ) ) ;
#3290=CARTESIAN_POINT ( 'NONE',  ( 5.000000000000000000, -140.0000000000000000, 0.000000000000000000 ) ) ;
#3294=CARTESIAN_POINT ( 'NONE',  ( 1.339745962155612702, -78.29465819873851729, -5.000000000000000000 ) ) ;
#3296=CARTESIAN_POINT ( 'NONE',  ( -2.229367062500000163, 20.52083333469892779, -3.861377020970580443 ) ) ;
#3298=CARTESIAN_POINT ( 'NONE',  ( 2.229367062499998831, -5.895833331967740953, -3.861377020970580887 ) ) ;
#3301=CARTESIAN_POINT ( 'NONE',  ( 2.071067811865475505, -140.9375000027311842, -5.000000000000000888 ) ) ;
#3306=CARTESIAN_POINT ( 'NONE',  ( -5.000000000000000000, -87.00000000000000000, 0.000000000000000000 ) ) ;
#3309=CARTESIAN_POINT ( 'NONE',  ( 4.458734124999997661, -157.7500000013656063, 1.846868145590737864 ) ) ;
#3311=DIRECTION ( 'NONE',  ( -0.000000000000000000, 1.000000000000000000, -0.000000000000000000 ) ) ;
#3312=ORIENTED_EDGE ( 'NONE', *, *, #48802, .F. ) ;
#3313=EDGE_CURVE ( 'NONE', #44876, #44350, #45106, .T. ) ;
#3314=CARTESIAN_POINT ( 'NONE',  ( 4.458734124999998549, 15.02083333469892601, -2.574251347313721627 ) ) ;
#3320=EDGE_CURVE ( 'NONE', #51834, #16219, #36862, .T. ) ;
#3321=CARTESIAN_POINT ( 'NONE',  ( 5.000000000000000000, 8.583333333333330373, -2.886751345948129988 ) ) ;
#3322=CARTESIAN_POINT ( 'NONE',  ( 4.458734124999999437, -59.81249999863440081, -5.460374474430324690E-16 ) ) ;
#3326=CARTESIAN_POINT ( 'NONE',  ( -2.229367062500000163, -26.47916666530106866, -3.861377020970580443 ) ) ;
#3327=CARTESIAN_POINT ( 'NONE',  ( -6.972266317189433020E-16, 7.875000002731185056, -5.000000000000000000 ) ) ;
#3330=CARTESIAN_POINT ( 'NONE',  ( 2.500000000000002220, -37.66666666666666430, 4.330127018922192761 ) ) ;
#3331=CARTESIAN_POINT ( 'NONE',  ( 5.000000000000000000, -149.0000000000000284, 0.000000000000000000 ) ) ;
#3332=CARTESIAN_POINT ( 'NONE',  ( -6.972266317189433020E-16, -48.24999999999999289, -5.000000000000000000 ) ) ;
#3334=CARTESIAN_POINT ( 'NONE',  ( 3.061616997868383141E-16, -143.7500000000000284, -5.000000000000000000 ) ) ;
#3335=CARTESIAN_POINT ( 'NONE',  ( -4.458734124999998549, -66.22916666530107932, 2.574251347313722516 ) ) ;
#3336=CARTESIAN_POINT ( 'NONE',  ( 4.458734125000000326, -147.6250000013655779, -1.846868145590734978 ) ) ;
#3337=CARTESIAN_POINT ( 'NONE',  ( 2.229367062499998831, -76.64583333196773651, -3.861377020970580887 ) ) ;
#3339=CARTESIAN_POINT ( 'NONE',  ( 2.229367062500001939, -26.22916666530106866, 3.861377020970579999 ) ) ;
#3340=CARTESIAN_POINT ( 'NONE',  ( 5.000000000000000888, -64.45833333060213022, 2.886751345948126879 ) ) ;
#3342=CARTESIAN_POINT ( 'NONE',  ( -5.000000000000000000, -22.08333333333333215, -2.886751345948128211 ) ) ;
#3346=ORIENTED_EDGE ( 'NONE', *, *, #38919, .T. ) ;
#3348=CARTESIAN_POINT ( 'NONE',  ( -5.000000000000000000, -55.95833333060214443, -2.886751345948128211 ) ) ;
#3349=CARTESIAN_POINT ( 'NONE',  ( -2.229367062499996610, -52.39583333196773651, 3.861377020970582219 ) ) ;
#3350=ORIENTED_EDGE ( 'NONE', *, *, #9525, .T. ) ;
#3353=CARTESIAN_POINT ( 'NONE',  ( -4.458734124999999437, 20.60416666803225993, -2.574251347313719407 ) ) ;
#3356=CARTESIAN_POINT ( 'NONE',  ( 1.975475456537005874E-15, -8.750000000000000000, 5.000000000000000000 ) ) ;
#3361=( BOUNDED_CURVE ( )  B_SPLINE_CURVE ( 2, ( #35283, #15978, #15021, #54904, #15347, #39769, #55229, #31088, #45247 ),
 .UNSPECIFIED., .F., .F. ) 
 B_SPLINE_CURVE_WITH_KNOTS ( ( 3, 2, 2, 2, 3 ),
 ( 0.6645833333333333037, 0.6652777777777777457, 0.6666666666666666297, 0.6680555555555555136, 0.6687499999999999556 ),
 .UNSPECIFIED. ) 
 CURVE ( )  GEOMETRIC_REPRESENTATION_ITEM ( )  RATIONAL_B_SPLINE_CURVE ( ( 0.9330127018922194093, 0.9330127018922194093, 1.000000000000000000, 0.8660254037844387076, 1.000000000000000000, 0.8660254037844387076, 1.000000000000000000, 0.9330127018922194093, 0.9330127018922194093 ) ) 
 REPRESENTATION_ITEM ( '' )  );
#3365=CARTESIAN_POINT ( 'NONE',  ( 5.000000000000000888, 4.416666666666666075, 2.886751345948126879 ) ) ;
#3368=DIRECTION ( 'NONE',  ( -0.000000000000000000, 1.000000000000000000, -0.000000000000000000 ) ) ;
#3375=CARTESIAN_POINT ( 'NONE',  ( -3.535533905932737309, -152.7500000027312126, -3.535533905932738197 ) ) ;
#3376=EDGE_LOOP ( 'NONE', ( #43952, #19473, #42253, #25414 ) ) ;
#3381=CARTESIAN_POINT ( 'NONE',  ( -2.071067811865475061, -148.6875000000000568, -5.000000000000000888 ) ) ;
#3382=ADVANCED_BREP_SHAPE_REPRESENTATION ( '', ( #7586, #43054 ), #38957 ) ;
#3386=CARTESIAN_POINT ( 'NONE',  ( 4.458734125000000326, -26.89583333196774007, 2.574251347313718519 ) ) ;
#3390=CARTESIAN_POINT ( 'NONE',  ( 1.846868145590736310, -147.6250000013655779, 4.458734124999999437 ) ) ;
#3393=CARTESIAN_POINT ( 'NONE',  ( -2.229367062499996610, -55.39583333196773651, 3.861377020970582219 ) ) ;
#3396=CARTESIAN_POINT ( 'NONE',  ( 2.499999999999998668, 21.66666666666666785, -4.330127018922193649 ) ) ;
#3398=CARTESIAN_POINT ( 'NONE',  ( 4.458734124999999437, 0.1875000013655953035, -5.460374474430324690E-16 ) ) ;
#3399=CARTESIAN_POINT ( 'NONE',  ( 1.975475456537005874E-15, -48.74999999999999289, 5.000000000000000000 ) ) ;
#3400=CARTESIAN_POINT ( 'NONE',  ( -5.000000000000000000, -164.5000000000000000, -6.123233995736766282E-16 ) ) ;
#3401=CARTESIAN_POINT ( 'NONE',  ( -2.229367062499996610, 11.60416666803225993, 3.861377020970582219 ) ) ;
#3402=ORIENTED_EDGE ( 'NONE', *, *, #2883, .F. ) ;
#3403=CARTESIAN_POINT ( 'NONE',  ( 1.975475456537005874E-15, -32.74999999999999289, 5.000000000000000000 ) ) ;
#3405=CARTESIAN_POINT ( 'NONE',  ( 5.000000000000000000, -168.1250000027312126, 0.000000000000000000 ) ) ;
#3406=CARTESIAN_POINT ( 'NONE',  ( 9.457646018065525792E-16, -51.06249999863440792, 5.148502694627439702 ) ) ;
#3407=CARTESIAN_POINT ( 'NONE',  ( 3.152801135295366208, -159.8125000013656063, 3.152801135295367985 ) ) ;
#3408=CARTESIAN_POINT ( 'NONE',  ( -5.000000000000000000, -46.87499999726880873, 0.000000000000000000 ) ) ;
#3409=ORIENTED_EDGE ( 'NONE', *, *, #31803, .T. ) ;
#3410=CARTESIAN_POINT ( 'NONE',  ( 4.458734124999998549, -21.72916666530107221, -2.574251347313721627 ) ) ;
#3414=CARTESIAN_POINT ( 'NONE',  ( -4.458734124999999437, -159.9375000013655779, -5.460374474430324690E-16 ) ) ;
#3417=CARTESIAN_POINT ( 'NONE',  ( 2.229367062500001939, -38.22916666530107221, 3.861377020970579999 ) ) ;
#3426=CARTESIAN_POINT ( 'NONE',  ( 4.458734125000001214, -84.14583333196772230, 2.574251347313718519 ) ) ;
#3428=DIRECTION ( 'NONE',  ( -0.000000000000000000, 1.000000000000000000, -0.000000000000000000 ) ) ;
#3429=CARTESIAN_POINT ( 'NONE',  ( 3.152801135295366208, -139.8125000013655779, 3.152801135295367985 ) ) ;
#3432=CARTESIAN_POINT ( 'NONE',  ( -6.972266317189433020E-16, -72.12499999726878741, -5.000000000000000000 ) ) ;
#3435=CARTESIAN_POINT ( 'NONE',  ( -2.500000000000000444, -82.16666666666667140, -4.330127018922193649 ) ) ;
#3438=CARTESIAN_POINT ( 'NONE',  ( 0.000000000000000000, -170.0000000000000000, 5.000000000000000000 ) ) ;
#3439=CARTESIAN_POINT ( 'NONE',  ( -4.999999999999998224, -45.79166666393547303, 2.886751345948131764 ) ) ;
#3440=CARTESIAN_POINT ( 'NONE',  ( 2.229367062499998831, -86.89583333196773651, -3.861377020970580887 ) ) ;
#3444=CARTESIAN_POINT ( 'NONE',  ( 1.339745962155615144, -9.580341798530296771, 4.999999999999999112 ) ) ;
#3446=CARTESIAN_POINT ( 'NONE',  ( -3.535533905932737309, -163.7500000027312126, -3.535533905932738197 ) ) ;
#3448=CARTESIAN_POINT ( 'NONE',  ( 9.457646018065525792E-16, 6.687500001365594748, 5.148502694627439702 ) ) ;
#3449=CARTESIAN_POINT ( 'NONE',  ( -5.000000000000000000, -16.00000000000000000, 0.000000000000000000 ) ) ;
#3455=DIRECTION ( 'NONE',  ( 0.000000000000000000, 0.000000000000000000, 1.000000000000000000 ) ) ;
#3456=CARTESIAN_POINT ( 'NONE',  ( 2.229367062499998831, -10.64583333196773829, -3.861377020970580887 ) ) ;
#3459=CARTESIAN_POINT ( 'NONE',  ( -4.458734124999999437, -37.64583333196774362, -2.574251347313719407 ) ) ;
#3460=( BOUNDED_CURVE ( )  B_SPLINE_CURVE ( 2, ( #45855, #29770, #14987, #34597, #54227, #49404, #30417, #25604, #5348 ),
 .UNSPECIFIED., .F., .F. ) 
 B_SPLINE_CURVE_WITH_KNOTS ( ( 3, 2, 2, 2, 3 ),
 ( 0.03125000000000000000, 0.03194444444444444198, 0.03333333333333333287, 0.03472222222222222376, 0.03541666666666666574 ),
 .UNSPECIFIED. ) 
 CURVE ( )  GEOMETRIC_REPRESENTATION_ITEM ( )  RATIONAL_B_SPLINE_CURVE ( ( 0.9330127018922194093, 0.9330127018922195203, 1.000000000000000000, 0.8660254037844387076, 1.000000000000000000, 0.8660254037844387076, 1.000000000000000000, 0.9330127018922194093, 0.9330127018922194093 ) ) 
 REPRESENTATION_ITEM ( '' )  );
#3463=DIRECTION ( 'NONE',  ( -0.000000000000000000, 1.000000000000000000, -0.000000000000000000 ) ) ;
#3466=AXIS2_PLACEMENT_3D ( 'NONE', #63142, #28087, #43187 ) ;
#3467=CARTESIAN_POINT ( 'NONE',  ( 4.458734124999999437, 14.18750000136559386, -5.460374474430324690E-16 ) ) ;
#3468=CYLINDRICAL_SURFACE ( 'NONE', #13361, 5.000000000000000000 ) ;
#3469=CARTESIAN_POINT ( 'NONE',  ( -6.972266317189433020E-16, -55.24999999999999289, -5.000000000000000000 ) ) ;
#3470=CARTESIAN_POINT ( 'NONE',  ( -4.458734124999999437, -81.64583333196773651, -2.574251347313719407 ) ) ;
#3472=CARTESIAN_POINT ( 'NONE',  ( 5.000000000000000888, 18.54166666939785202, 2.886751345948126879 ) ) ;
#3473=ORIENTED_EDGE ( 'NONE', *, *, #45337, .F. ) ;
#3474=CARTESIAN_POINT ( 'NONE',  ( 1.062108568985190270E-13, -25.25000000000000355, -4.999999999999999112 ) ) ;
#3477=CARTESIAN_POINT ( 'NONE',  ( 2.500000000000002220, -26.66666666666666430, 4.330127018922192761 ) ) ;
#3478=CARTESIAN_POINT ( 'NONE',  ( 2.229367062500001939, -30.97916666530107221, 3.861377020970579999 ) ) ;
#3479=LINE ( 'NONE', #12803, #11933 ) ;
#3480=CARTESIAN_POINT ( 'NONE',  ( -2.499999999999996447, -30.70833333060214443, 4.330127018922195425 ) ) ;
#3481=CARTESIAN_POINT ( 'NONE',  ( 9.457646018065525792E-16, -59.06249999863439371, 5.148502694627439702 ) ) ;
#3483=FACE_OUTER_BOUND ( 'NONE', #3376, .T. ) ;
#3484=CARTESIAN_POINT ( 'NONE',  ( 2.229367062499998831, -6.895833331967741842, -3.861377020970580887 ) ) ;
#3486=CARTESIAN_POINT ( 'NONE',  ( 1.060575238724906964E-15, -75.75000000000000000, 5.773502691896257311 ) ) ;
#3487=CARTESIAN_POINT ( 'NONE',  ( -2.499999999999996447, 1.291666669397853351, 4.330127018922195425 ) ) ;
#3489=CARTESIAN_POINT ( 'NONE',  ( -2.499999999999996447, -77.70833333060214443, 4.330127018922195425 ) ) ;
#3490=CARTESIAN_POINT ( 'NONE',  ( 2.500000000000002220, -65.54166666393547303, 4.330127018922192761 ) ) ;
#3491=VERTEX_POINT ( 'NONE', #6771 ) ;
#3493=EDGE_CURVE ( 'NONE', #57905, #6259, #7745, .T. ) ;
#3494=CARTESIAN_POINT ( 'NONE',  ( -4.458734124999999437, -22.56249999863440436, 0.000000000000000000 ) ) ;
#3495=CARTESIAN_POINT ( 'NONE',  ( -2.229367062499996610, -59.39583333196773651, 3.861377020970582219 ) ) ;
#3497=CARTESIAN_POINT ( 'NONE',  ( -4.458734125000000326, -140.0000000013655779, -1.846868145590735644 ) ) ;
#3499=CARTESIAN_POINT ( 'NONE',  ( -1.339745962155613812, 17.79465819873852439, -5.000000000000000000 ) ) ;
#3500=ORIENTED_EDGE ( 'NONE', *, *, #62930, .F. ) ;
#3508=CARTESIAN_POINT ( 'NONE',  ( 1.846868145590736310, -143.8750000013656063, 4.458734124999999437 ) ) ;
#3510=ADVANCED_FACE ( 'NONE', ( #1329 ), #16096, .T. ) ;
#3513=CARTESIAN_POINT ( 'NONE',  ( 4.458734124999999437, -67.06249999863440792, -5.460374474430324690E-16 ) ) ;
#3514=CARTESIAN_POINT ( 'NONE',  ( 5.000000000000000000, -43.50000000000000000, -6.123233995736766282E-16 ) ) ;
#3516=CARTESIAN_POINT ( 'NONE',  ( -4.458734124999999437, -140.0000000013655779, -1.846868145590735644 ) ) ;
#3518=ORIENTED_EDGE ( 'NONE', *, *, #54318, .F. ) ;
#3519=CARTESIAN_POINT ( 'NONE',  ( -5.000000000000000000, -49.87499999726881583, 0.000000000000000000 ) ) ;
#3520=CARTESIAN_POINT ( 'NONE',  ( 0.000000000000000000, -170.0000000000000000, 0.000000000000000000 ) ) ;
#3525=CARTESIAN_POINT ( 'NONE',  ( 2.229367062499998831, 27.10416666803225993, -3.861377020970580887 ) ) ;
#3533=CARTESIAN_POINT ( 'NONE',  ( 4.458734124999998549, 7.270833334698930450, -2.574251347313721627 ) ) ;
#3535=CARTESIAN_POINT ( 'NONE',  ( -3.152548672688508926E-16, -21.81249999863440436, -5.148502694627439702 ) ) ;
#3537=CARTESIAN_POINT ( 'NONE',  ( -8.190561711645485556E-16, -161.6875000013655779, 4.458734124999999437 ) ) ;
#3538=CARTESIAN_POINT ( 'NONE',  ( -3.535533905932738641, -158.3750000000000284, 3.535533905932737309 ) ) ;
#3542=CARTESIAN_POINT ( 'NONE',  ( 2.500000000000002220, 15.33333333333333215, 4.330127018922192761 ) ) ;
#3543=CARTESIAN_POINT ( 'NONE',  ( 2.229367062500001939, -41.97916666530107932, 3.861377020970579999 ) ) ;
#3546=CARTESIAN_POINT ( 'NONE',  ( 9.457646018065525792E-16, -66.31249999863440792, 5.148502694627439702 ) ) ;
#3549=CARTESIAN_POINT ( 'NONE',  ( 2.499999999999998668, -89.33333333333332860, -4.330127018922193649 ) ) ;
#3552=CARTESIAN_POINT ( 'NONE',  ( -6.972266317189433020E-16, -6.124999997268813168, -5.000000000000000000 ) ) ;
#3553=CARTESIAN_POINT ( 'NONE',  ( 5.000000000000000000, -13.41666666666666607, -2.886751345948129988 ) ) ;
#3554=CARTESIAN_POINT ( 'NONE',  ( -4.458734124999999437, -17.39583333196773651, -2.574251347313719407 ) ) ;
#3555=CARTESIAN_POINT ( 'NONE',  ( 9.457646018065525792E-16, -75.06249999863440792, 5.148502694627439702 ) ) ;
#3556=AXIS2_PLACEMENT_3D ( 'NONE', #37023, #17408, #27355 ) ;
#3558=CARTESIAN_POINT ( 'NONE',  ( 2.500000000000002220, -10.54166666393547835, 4.330127018922192761 ) ) ;
#3559=CARTESIAN_POINT ( 'NONE',  ( -2.229367062499996610, -46.14583333196774362, 3.861377020970582219 ) ) ;
#3560=VERTEX_POINT ( 'NONE', #46000 ) ;
#3561=CARTESIAN_POINT ( 'NONE',  ( -9.184850993605147944E-16, -144.2500000000000284, 5.000000000000000000 ) ) ;
#3562=CARTESIAN_POINT ( 'NONE',  ( 4.458734124999999437, 4.937500001365595637, -5.460374474430324690E-16 ) ) ;
#3564=LINE ( 'NONE', #42782, #39141 ) ;
#3565=CARTESIAN_POINT ( 'NONE',  ( 2.500000000000002220, -62.66666666666666430, 4.330127018922192761 ) ) ;
#3566=CARTESIAN_POINT ( 'NONE',  ( 2.730187237215162345E-16, -159.4375000013655779, -4.458734124999999437 ) ) ;
#3568=CARTESIAN_POINT ( 'NONE',  ( 1.975475456537005874E-15, -14.74999999999999822, 5.000000000000000000 ) ) ;
#3569=CARTESIAN_POINT ( 'NONE',  ( 3.061616997868383141E-16, -167.7500000000000000, -5.000000000000000000 ) ) ;
#3570=CARTESIAN_POINT ( 'NONE',  ( 5.000000000000000888, -11.58333333333333393, 2.886751345948126879 ) ) ;
#3572=EDGE_CURVE ( 'NONE', #48999, #18747, #6817, .T. ) ;
#3573=CARTESIAN_POINT ( 'NONE',  ( 4.458734124999998549, -3.979166665301070438, -2.574251347313721627 ) ) ;
#3574=CARTESIAN_POINT ( 'NONE',  ( -4.458734124999999437, -41.56249999863440081, 0.000000000000000000 ) ) ;
#3575=ADVANCED_FACE ( 'NONE', ( #59207 ), #26067, .T. ) ;
#3577=CARTESIAN_POINT ( 'NONE',  ( 2.499999999999998668, -67.20833333060214443, -4.330127018922193649 ) ) ;
#3579=CARTESIAN_POINT ( 'NONE',  ( 2.500000000000002220, -84.66666666666667140, 4.330127018922192761 ) ) ;
#3582=CARTESIAN_POINT ( 'NONE',  ( -2.500000000000000444, -12.04166666393547835, -4.330127018922193649 ) ) ;
#3583=CARTESIAN_POINT ( 'NONE',  ( -4.458734124999999437, -67.64583333196773651, -2.574251347313719407 ) ) ;
#3584=CARTESIAN_POINT ( 'NONE',  ( -8.190561711645485556E-16, -146.9375000013656063, 4.458734124999999437 ) ) ;
#3586=ADVANCED_FACE ( 'NONE', ( #34758 ), #29922, .T. ) ;
#3587=CARTESIAN_POINT ( 'NONE',  ( -5.000000000000000888, -146.6875000027312126, -2.071067811865475949 ) ) ;
#3591=CARTESIAN_POINT ( 'NONE',  ( -4.458734124999999437, 0.6041666680322611560, -2.574251347313719407 ) ) ;
#3592=CARTESIAN_POINT ( 'NONE',  ( 5.000000000000000000, -30.37499999726881228, -6.123233995736766282E-16 ) ) ;
#3593=CARTESIAN_POINT ( 'NONE',  ( -4.458734124999999437, -153.0000000013656063, -1.846868145590735644 ) ) ;
#3595=ORIENTED_EDGE ( 'NONE', *, *, #20124, .T. ) ;
#3597=CARTESIAN_POINT ( 'NONE',  ( 1.062108568985190270E-13, -25.25000000000000355, -4.999999999999999112 ) ) ;
#3601=CARTESIAN_POINT ( 'NONE',  ( 1.339745962155612702, -87.29465819873851729, -5.000000000000000000 ) ) ;
#3603=CARTESIAN_POINT ( 'NONE',  ( 5.000000000000000000, -64.37499999726881583, -6.123233995736766282E-16 ) ) ;
#3606=CARTESIAN_POINT ( 'NONE',  ( 4.458734124999998549, 24.27083333469892779, -2.574251347313721627 ) ) ;
#3608=CARTESIAN_POINT ( 'NONE',  ( 2.229367062500001939, -3.229166665301069550, 3.861377020970579999 ) ) ;
#3609=( BOUNDED_CURVE ( )  B_SPLINE_CURVE ( 2, ( #25379, #18102, #57358, #58524, #13279, #44669, #629, #49502, #53693 ),
 .UNSPECIFIED., .F., .F. ) 
 B_SPLINE_CURVE_WITH_KNOTS ( ( 3, 2, 2, 2, 3 ),
 ( 0.8270833333333332815, 0.8277777777777777235, 0.8291666666666667185, 0.8305555555555556024, 0.8312500000000000444 ),
 .UNSPECIFIED. ) 
 CURVE ( )  GEOMETRIC_REPRESENTATION_ITEM ( )  RATIONAL_B_SPLINE_CURVE ( ( 0.9330127018922194093, 0.9330127018922194093, 1.000000000000000000, 0.8660254037844387076, 1.000000000000000000, 0.8660254037844387076, 1.000000000000000000, 0.9330127018922194093, 0.9330127018922194093 ) ) 
 REPRESENTATION_ITEM ( '' )  );
#3610=CYLINDRICAL_SURFACE ( 'NONE', #49380, 5.000000000000000000 ) ;
#3612=CARTESIAN_POINT ( 'NONE',  ( -3.535533905932737309, -139.7500000027311842, -3.535533905932738197 ) ) ;
#3613=CARTESIAN_POINT ( 'NONE',  ( -6.972266317189433020E-16, -52.25000000000000711, -5.000000000000000000 ) ) ;
#3620=CARTESIAN_POINT ( 'NONE',  ( -4.458734124999999437, -159.1875000013655779, -5.460374474430324690E-16 ) ) ;
#3624=CARTESIAN_POINT ( 'NONE',  ( -4.458734124999998549, 17.52083333469892779, 2.574251347313722516 ) ) ;
#3625=ORIENTED_EDGE ( 'NONE', *, *, #53182, .F. ) ;
#3629=LINE ( 'NONE', #22939, #55570 ) ;
#3630=CARTESIAN_POINT ( 'NONE',  ( 2.500000000000002220, 1.333333333333332149, 4.330127018922192761 ) ) ;
#3631=CARTESIAN_POINT ( 'NONE',  ( -3.152548672688508926E-16, -63.56249999863440792, -5.148502694627439702 ) ) ;
#3632=DIRECTION ( 'NONE',  ( -0.000000000000000000, 1.000000000000000000, -0.000000000000000000 ) ) ;
#3633=CARTESIAN_POINT ( 'NONE',  ( 2.229367062500001939, -28.97916666530107221, 3.861377020970579999 ) ) ;
#3634=CARTESIAN_POINT ( 'NONE',  ( 1.975475456537005874E-15, 5.249999999999999112, 5.000000000000000000 ) ) ;
#3635=LINE ( 'NONE', #27749, #37437 ) ;
#3637=CARTESIAN_POINT ( 'NONE',  ( 1.060575238724906964E-15, -43.75000000000000000, 5.773502691896257311 ) ) ;
#3643=CARTESIAN_POINT ( 'NONE',  ( -2.229367062500000163, -62.47916666530106511, -3.861377020970580443 ) ) ;
#3644=CARTESIAN_POINT ( 'NONE',  ( -1.846868145590737420, -147.0000000013655779, 4.458734124999999437 ) ) ;
#3645=CARTESIAN_POINT ( 'NONE',  ( 9.457646018065525792E-16, -77.06249999863440792, 5.148502694627439702 ) ) ;
#3647=AXIS2_PLACEMENT_3D ( 'NONE', #57760, #4043, #23031 ) ;
#3648=CARTESIAN_POINT ( 'NONE',  ( -4.458734124999999437, -24.64583333196773651, -2.574251347313719407 ) ) ;
#3649=CARTESIAN_POINT ( 'NONE',  ( -4.999999999999999112, -63.79166666393547303, 2.886751345948131764 ) ) ;
#3651=ORIENTED_EDGE ( 'NONE', *, *, #41308, .T. ) ;
#3652=CARTESIAN_POINT ( 'NONE',  ( -1.339745962155613812, -22.20534180126147561, -5.000000000000000000 ) ) ;
#3655=CARTESIAN_POINT ( 'NONE',  ( -9.184850993605147944E-16, -149.3750000027312126, 5.000000000000000000 ) ) ;
#3656=ORIENTED_EDGE ( 'NONE', *, *, #55776, .F. ) ;
#3658=DIRECTION ( 'NONE',  ( 0.000000000000000000, 0.000000000000000000, 1.000000000000000000 ) ) ;
#3659=CARTESIAN_POINT ( 'NONE',  ( 4.458734124999998549, -51.97916666530107221, -2.574251347313721627 ) ) ;
#3660=EDGE_CURVE ( 'NONE', #11945, #53004, #27021, .T. ) ;
#3665=ADVANCED_FACE ( 'NONE', ( #60808 ), #27647, .T. ) ;
#3666=CARTESIAN_POINT ( 'NONE',  ( -4.458734124999999437, 20.68750000136559208, 0.000000000000000000 ) ) ;
#3669=CARTESIAN_POINT ( 'NONE',  ( 4.458734124999997661, -167.5000000013655779, 1.846868145590737864 ) ) ;
#3670=VERTEX_POINT ( 'NONE', #17374 ) ;
#3675=ADVANCED_FACE ( 'NONE', ( #17688 ), #16735, .T. ) ;
#3676=CARTESIAN_POINT ( 'NONE',  ( 5.000000000000000000, -140.1875000027311842, 2.071067811865478614 ) ) ;
#3681=CARTESIAN_POINT ( 'NONE',  ( 5.000000000000000000, -76.50000000000000000, -6.123233995736766282E-16 ) ) ;
#3688=CARTESIAN_POINT ( 'NONE',  ( -5.000000000000000888, -153.6875000027312126, -2.071067811865475949 ) ) ;
#3689=ORIENTED_EDGE ( 'NONE', *, *, #18863, .F. ) ;
#3695=CARTESIAN_POINT ( 'NONE',  ( -3.535533905932737309, -148.6250000000000000, -3.535533905932738197 ) ) ;
#3698=CARTESIAN_POINT ( 'NONE',  ( -4.999999999999998224, -54.91666666666667140, 2.886751345948131764 ) ) ;
#3699=CARTESIAN_POINT ( 'NONE',  ( 9.457646018065525792E-16, -30.06249999863440436, 5.148502694627439702 ) ) ;
#3703=CARTESIAN_POINT ( 'NONE',  ( 3.152801135295367541, -148.3125000013655779, -3.152801135295367541 ) ) ;
#3704=ORIENTED_EDGE ( 'NONE', *, *, #49603, .T. ) ;
#3705=LINE ( 'NONE', #27815, #46142 ) ;
#3706=CARTESIAN_POINT ( 'NONE',  ( -2.229367062499996610, -58.39583333196773651, 3.861377020970582219 ) ) ;
#3708=DIRECTION ( 'NONE',  ( 0.000000000000000000, 0.000000000000000000, 1.000000000000000000 ) ) ;
#3709=CARTESIAN_POINT ( 'NONE',  ( -5.000000000000000000, 19.99999999999999645, 0.000000000000000000 ) ) ;
#3710=FACE_OUTER_BOUND ( 'NONE', #8135, .T. ) ;
#3711=CARTESIAN_POINT ( 'NONE',  ( -2.229367062500000163, -1.479166665301071770, -3.861377020970580443 ) ) ;
#3712=CARTESIAN_POINT ( 'NONE',  ( 5.000000000000000000, -48.50000000000000000, -6.123233995736766282E-16 ) ) ;
#3714=CARTESIAN_POINT ( 'NONE',  ( -4.458734124999999437, 9.354166668032261711, -2.574251347313719407 ) ) ;
#3716=ORIENTED_EDGE ( 'NONE', *, *, #34943, .F. ) ;
#3717=CARTESIAN_POINT ( 'NONE',  ( 4.458734124999999437, -169.4375000013656063, 0.000000000000000000 ) ) ;
#3718=CARTESIAN_POINT ( 'NONE',  ( 2.229367062500001939, -47.97916666530106511, 3.861377020970579999 ) ) ;
#3719=CARTESIAN_POINT ( 'NONE',  ( -1.846868145590737420, -162.0000000013655779, 4.458734124999999437 ) ) ;
#3720=CARTESIAN_POINT ( 'NONE',  ( -5.000000000000000000, -48.87499999726880873, 0.000000000000000000 ) ) ;
#3722=CARTESIAN_POINT ( 'NONE',  ( 9.457646018065525792E-16, -24.06249999863440436, 5.148502694627439702 ) ) ;
#3723=ORIENTED_EDGE ( 'NONE', *, *, #46043, .F. ) ;
#3726=CARTESIAN_POINT ( 'NONE',  ( -4.458734125000001214, -160.8750000013655779, 1.846868145590734089 ) ) ;
#3730=CARTESIAN_POINT ( 'NONE',  ( 4.458734124999998549, -38.97916666530107221, -2.574251347313721627 ) ) ;
#3732=VECTOR ( 'NONE', #38002, 1000.000000000000000 ) ;
#3733=( BOUNDED_CURVE ( )  B_SPLINE_CURVE ( 2, ( #10042, #45096, #29974, #49601, #16147, #26118, #5543, #1061, #20667 ),
 .UNSPECIFIED., .F., .F. ) 
 B_SPLINE_CURVE_WITH_KNOTS ( ( 3, 2, 2, 2, 3 ),
 ( 0.8729166666666666741, 0.8736111111111111160, 0.8750000000000000000, 0.8763888888888888840, 0.8770833333333333259 ),
 .UNSPECIFIED. ) 
 CURVE ( )  GEOMETRIC_REPRESENTATION_ITEM ( )  RATIONAL_B_SPLINE_CURVE ( ( 0.9330127018922194093, 0.9330127018922194093, 1.000000000000000000, 0.8660254037844387076, 1.000000000000000000, 0.8660254037844387076, 1.000000000000000000, 0.9330127018922194093, 0.9330127018922194093 ) ) 
 REPRESENTATION_ITEM ( '' )  );
#3739=CARTESIAN_POINT ( 'NONE',  ( -4.458734124999998549, -84.47916666530107932, 2.574251347313722516 ) ) ;
#3741=CARTESIAN_POINT ( 'NONE',  ( -6.972266317189433020E-16, -35.12499999726880873, -5.000000000000000000 ) ) ;
#3742=CARTESIAN_POINT ( 'NONE',  ( -2.071067811865580754, -158.8125000027312126, -4.999999999999894307 ) ) ;
#3743=CARTESIAN_POINT ( 'NONE',  ( 2.500000000000002220, -57.66666666666667140, 4.330127018922192761 ) ) ;
#3745=CARTESIAN_POINT ( 'NONE',  ( 5.000000000000000888, -37.58333333333332860, 2.886751345948126879 ) ) ;
#3751=DIRECTION ( 'NONE',  ( -0.000000000000000000, 1.000000000000000000, -0.000000000000000000 ) ) ;
#3753=CARTESIAN_POINT ( 'NONE',  ( 9.457646018065525792E-16, -87.31249999863440792, 5.148502694627439702 ) ) ;
#3759=CARTESIAN_POINT ( 'NONE',  ( 3.061616997868383141E-16, -165.8750000027312126, -5.000000000000000000 ) ) ;
#3762=CARTESIAN_POINT ( 'NONE',  ( -6.972266317189433020E-16, -23.24999999999999645, -5.000000000000000000 ) ) ;
#3767=CARTESIAN_POINT ( 'NONE',  ( -6.972266317189433020E-16, -46.24999999999999289, -5.000000000000000000 ) ) ;
#3768=CARTESIAN_POINT ( 'NONE',  ( 3.061616997868383141E-16, -152.7500000000000000, -5.000000000000000000 ) ) ;
#3769=CARTESIAN_POINT ( 'NONE',  ( 2.229367062499998831, -12.64583333196774007, -3.861377020970580887 ) ) ;
#3772=CARTESIAN_POINT ( 'NONE',  ( 4.458734124999998549, -39.97916666530107221, -2.574251347313721627 ) ) ;
#3773=VECTOR ( 'NONE', #60, 1000.000000000000000 ) ;
#3774=CARTESIAN_POINT ( 'NONE',  ( 5.000000000000000888, -77.58333333333334281, 2.886751345948126879 ) ) ;
#3775=CARTESIAN_POINT ( 'NONE',  ( -2.500000000000000444, 26.95833333606451632, -4.330127018922193649 ) ) ;
#3779=AXIS2_PLACEMENT_3D ( 'NONE', #35008, #30158, #5733 ) ;
#3780=CARTESIAN_POINT ( 'NONE',  ( 4.458734124999998549, 15.27083333469893134, -2.574251347313721627 ) ) ;
#3783=CARTESIAN_POINT ( 'NONE',  ( 9.457646018065525792E-16, -88.31249999863439371, 5.148502694627439702 ) ) ;
#3785=( BOUNDED_CURVE ( )  B_SPLINE_CURVE ( 2, ( #4565, #34149, #24511, #19040, #23253, #43796, #38972, #38044, #28383 ),
 .UNSPECIFIED., .F., .F. ) 
 B_SPLINE_CURVE_WITH_KNOTS ( ( 3, 2, 2, 2, 3 ),
 ( 0.2770833333333333481, 0.2777777777777777901, 0.2791666666666666741, 0.2805555555555555580, 0.2812500000000000000 ),
 .UNSPECIFIED. ) 
 CURVE ( )  GEOMETRIC_REPRESENTATION_ITEM ( )  RATIONAL_B_SPLINE_CURVE ( ( 0.9330127018922194093, 0.9330127018922194093, 1.000000000000000000, 0.8660254037844387076, 1.000000000000000000, 0.8660254037844387076, 1.000000000000000000, 0.9330127018922194093, 0.9330127018922194093 ) ) 
 REPRESENTATION_ITEM ( '' )  );
#3786=CARTESIAN_POINT ( 'NONE',  ( -4.999999999999999112, 12.20833333606451632, 2.886751345948131764 ) ) ;
#3790=CARTESIAN_POINT ( 'NONE',  ( -5.000000000000000000, 15.91666666666666430, -2.886751345948128211 ) ) ;
#3792=CARTESIAN_POINT ( 'NONE',  ( -3.535250795749689387E-16, -29.25000000000000000, -5.773502691896257311 ) ) ;
#3793=CARTESIAN_POINT ( 'NONE',  ( 4.458734125000001214, -32.89583333196774362, 2.574251347313718519 ) ) ;
#3795=CARTESIAN_POINT ( 'NONE',  ( -2.499999999999996447, -31.70833333060214798, 4.330127018922195425 ) ) ;
#3796=CARTESIAN_POINT ( 'NONE',  ( -4.458734124999999437, -62.39583333196774362, -2.574251347313719407 ) ) ;
#3797=ORIENTED_EDGE ( 'NONE', *, *, #28405, .T. ) ;
#3799=CARTESIAN_POINT ( 'NONE',  ( -4.458734124999998549, -8.479166665301073991, 2.574251347313722516 ) ) ;
#3801=CARTESIAN_POINT ( 'NONE',  ( -2.500000000000000444, -77.16666666666665719, -4.330127018922193649 ) ) ;
#3803=CARTESIAN_POINT ( 'NONE',  ( -3.535250795749689387E-16, -76.12499999726881583, -5.773502691896257311 ) ) ;
#3804=CARTESIAN_POINT ( 'NONE',  ( 2.500000000000002220, -13.66666666666666785, 4.330127018922192761 ) ) ;
#3807=CARTESIAN_POINT ( 'NONE',  ( -2.229367062500000163, -19.72916666530107221, -3.861377020970580443 ) ) ;
#3808=CARTESIAN_POINT ( 'NONE',  ( -4.458734124999998549, -55.47916666530107221, 2.574251347313722516 ) ) ;
#3811=CARTESIAN_POINT ( 'NONE',  ( -4.458734125000001214, -168.1250000013656063, 1.846868145590734089 ) ) ;
#3813=CARTESIAN_POINT ( 'NONE',  ( -6.972266317189433020E-16, -50.12499999726881583, -5.000000000000000000 ) ) ;
#3815=EDGE_LOOP ( 'NONE', ( #61954, #23823, #32039, #46530 ) ) ;
#3823=CARTESIAN_POINT ( 'NONE',  ( -3.152801135295367096, -145.3125000013655779, -3.152801135295367541 ) ) ;
#3825=LINE ( 'NONE', #57857, #26262 ) ;
#3827=CARTESIAN_POINT ( 'NONE',  ( 4.458734124999999437, -71.06249999863439371, -5.460374474430324690E-16 ) ) ;
#3829=FACE_OUTER_BOUND ( 'NONE', #54106, .T. ) ;
#3830=CARTESIAN_POINT ( 'NONE',  ( 3.152801135295366208, -140.5625000013655779, 3.152801135295367985 ) ) ;
#3833=EDGE_LOOP ( 'NONE', ( #26978, #17584, #61966, #11244 ) ) ;
#3834=CARTESIAN_POINT ( 'NONE',  ( 1.975475456537005874E-15, -7.624999997268812280, 5.000000000000000000 ) ) ;
#3835=FACE_OUTER_BOUND ( 'NONE', #45418, .T. ) ;
#3840=CARTESIAN_POINT ( 'NONE',  ( 4.458734124999999437, 21.93750000136559208, -5.460374474430324690E-16 ) ) ;
#3846=CARTESIAN_POINT ( 'NONE',  ( -2.229367062500000163, 4.520833334698926897, -3.861377020970580443 ) ) ;
#3847=CARTESIAN_POINT ( 'NONE',  ( -4.458734124999999437, -26.56249999863440792, 0.000000000000000000 ) ) ;
#3848=CARTESIAN_POINT ( 'NONE',  ( -8.190561711645485556E-16, -155.6875000013655779, 4.458734124999999437 ) ) ;
#3851=EDGE_CURVE ( 'NONE', #63425, #7768, #63152, .T. ) ;
#3855=CARTESIAN_POINT ( 'NONE',  ( 2.229367062499998831, -67.89583333196773651, -3.861377020970580887 ) ) ;
#3858=CARTESIAN_POINT ( 'NONE',  ( 5.000000000000000000, 27.62500000273118417, -6.123233995736766282E-16 ) ) ;
#3859=VERTEX_POINT ( 'NONE', #36670 ) ;
#3862=CARTESIAN_POINT ( 'NONE',  ( -5.000000000000000000, -13.99999999999999822, 0.000000000000000000 ) ) ;
#3863=CARTESIAN_POINT ( 'NONE',  ( -4.458734124999998549, -19.22916666530106866, 2.574251347313722516 ) ) ;
#3864=CARTESIAN_POINT ( 'NONE',  ( 2.229367062499998831, -79.64583333196773651, -3.861377020970580887 ) ) ;
#3867=EDGE_CURVE ( 'NONE', #42419, #44127, #7727, .T. ) ;
#3868=CARTESIAN_POINT ( 'NONE',  ( 5.000000000000000000, -15.37499999726881228, -6.123233995736766282E-16 ) ) ;
#3869=CARTESIAN_POINT ( 'NONE',  ( -2.229367062500000163, -44.47916666530106511, -3.861377020970580443 ) ) ;
#3872=EDGE_CURVE ( 'NONE', #35072, #29621, #51785, .T. ) ;
#3873=CARTESIAN_POINT ( 'NONE',  ( -3.152548672688508926E-16, 6.187500001365593860, -5.148502694627439702 ) ) ;
#3876=CARTESIAN_POINT ( 'NONE',  ( 2.499999999999998668, -60.33333333333333570, -4.330127018922193649 ) ) ;
#3877=CARTESIAN_POINT ( 'NONE',  ( -4.458734125000000326, -157.2500000013656063, -1.846868145590735644 ) ) ;
#3880=CARTESIAN_POINT ( 'NONE',  ( -2.071067811865475061, -165.6875000000000284, -5.000000000000000888 ) ) ;
#3881=DIRECTION ( 'NONE',  ( -0.000000000000000000, 1.000000000000000000, -0.000000000000000000 ) ) ;
#3883=CARTESIAN_POINT ( 'NONE',  ( 2.229367062500001939, -8.229166665301073991, 3.861377020970579999 ) ) ;
#3885=CARTESIAN_POINT ( 'NONE',  ( -4.458734124999999437, -38.64583333196772941, -2.574251347313719407 ) ) ;
#3887=CARTESIAN_POINT ( 'NONE',  ( 3.152801135295367541, -150.3125000013655779, -3.152801135295367541 ) ) ;
#3889=CARTESIAN_POINT ( 'NONE',  ( 2.071067811865455077, -166.9375000027312126, -5.000000000000022204 ) ) ;
#3891=CARTESIAN_POINT ( 'NONE',  ( -3.535533905932738641, -148.5000000027311842, 3.535533905932737309 ) ) ;
#3893=CARTESIAN_POINT ( 'NONE',  ( 9.457646018065525792E-16, -70.31249999863439371, 5.148502694627439702 ) ) ;
#3894=CARTESIAN_POINT ( 'NONE',  ( 3.152801135295366208, -144.8125000013655779, 3.152801135295367985 ) ) ;
#3900=CARTESIAN_POINT ( 'NONE',  ( -2.229367062499996610, 4.854166668032261711, 3.861377020970582219 ) ) ;
#3902=CARTESIAN_POINT ( 'NONE',  ( -1.846868145590734756, -153.1250000013656063, -4.458734124999999437 ) ) ;
#3906=CARTESIAN_POINT ( 'NONE',  ( -6.972266317189433020E-16, -75.25000000000000000, -5.000000000000000000 ) ) ;
#3910=DIRECTION ( 'NONE',  ( 0.000000000000000000, 0.000000000000000000, 1.000000000000000000 ) ) ;
#3912=( BOUNDED_CURVE ( )  B_SPLINE_CURVE ( 2, ( #6243, #25853, #21987, #45469, #17155, #21351, #56411, #1434, #60603 ),
 .UNSPECIFIED., .F., .F. ) 
 B_SPLINE_CURVE_WITH_KNOTS ( ( 3, 2, 2, 2, 3 ),
 ( 0.7812500000000000000, 0.7819444444444444420, 0.7833333333333333259, 0.7847222222222222099, 0.7854166666666666519 ),
 .UNSPECIFIED. ) 
 CURVE ( )  GEOMETRIC_REPRESENTATION_ITEM ( )  RATIONAL_B_SPLINE_CURVE ( ( 0.9330127018922194093, 0.9330127018922194093, 1.000000000000000000, 0.8660254037844387076, 1.000000000000000000, 0.8660254037844387076, 1.000000000000000000, 0.9330127018922194093, 0.9330127018922194093 ) ) 
 REPRESENTATION_ITEM ( '' )  );
#3917=CARTESIAN_POINT ( 'NONE',  ( -2.499999999999996447, -71.83333333333332860, 4.330127018922195425 ) ) ;
#3918=CARTESIAN_POINT ( 'NONE',  ( -2.229367062500000163, 25.52083333469892779, -3.861377020970580443 ) ) ;
#3920=CARTESIAN_POINT ( 'NONE',  ( 4.458734124999999437, -5.062499998634402587, -5.460374474430324690E-16 ) ) ;
#3921=CARTESIAN_POINT ( 'NONE',  ( -1.339745962155613812, -34.08034179853029144, -5.000000000000000000 ) ) ;
#3923=CARTESIAN_POINT ( 'NONE',  ( 1.846868145590736310, -168.6250000013655779, 4.458734124999999437 ) ) ;
#3933=CARTESIAN_POINT ( 'NONE',  ( -4.458734124999999437, -157.1875000013655779, -5.460374474430324690E-16 ) ) ;
#3936=ORIENTED_EDGE ( 'NONE', *, *, #8369, .T. ) ;
#3942=CARTESIAN_POINT ( 'NONE',  ( 5.000000000000000888, 12.41666666666666607, 2.886751345948126879 ) ) ;
#3943=CARTESIAN_POINT ( 'NONE',  ( 5.000000000000000000, 2.499999999999998668, -6.123233995736766282E-16 ) ) ;
#3944=CARTESIAN_POINT ( 'NONE',  ( 4.458734125000000326, -63.89583333196772941, 2.574251347313718519 ) ) ;
#3946=CARTESIAN_POINT ( 'NONE',  ( 2.499999999999998668, 1.791666669397853795, -4.330127018922193649 ) ) ;
#3947=CARTESIAN_POINT ( 'NONE',  ( 4.458734124999999437, -26.81249999863440081, -5.460374474430324690E-16 ) ) ;
#3949=CARTESIAN_POINT ( 'NONE',  ( -1.339745962155611370, 25.91965820146970856, -5.000000000000000888 ) ) ;
#3952=CARTESIAN_POINT ( 'NONE',  ( 2.499999999999998668, -44.33333333333333570, -4.330127018922193649 ) ) ;
#3956=CARTESIAN_POINT ( 'NONE',  ( 4.458734124999999437, -63.81249999863440792, -5.460374474430324690E-16 ) ) ;
#3957=CARTESIAN_POINT ( 'NONE',  ( -3.152801135295367985, -146.0625000013655779, 3.152801135295367096 ) ) ;
#3958=CARTESIAN_POINT ( 'NONE',  ( -4.458734124999998549, -75.22916666530106511, 2.574251347313722516 ) ) ;
#3959=VECTOR ( 'NONE', #9156, 1000.000000000000000 ) ;
#3961=CARTESIAN_POINT ( 'NONE',  ( -4.458734124999998549, -27.47916666530106866, 2.574251347313722516 ) ) ;
#3962=CARTESIAN_POINT ( 'NONE',  ( -5.000000000000000000, -65.95833333060213022, -2.886751345948128211 ) ) ;
#3963=ORIENTED_EDGE ( 'NONE', *, *, #10765, .T. ) ;
#3964=CARTESIAN_POINT ( 'NONE',  ( 1.975475456537005874E-15, -51.75000000000000711, 5.000000000000000000 ) ) ;
#3965=ORIENTED_EDGE ( 'NONE', *, *, #22115, .F. ) ;
#3967=CARTESIAN_POINT ( 'NONE',  ( 2.788906526875773208E-15, 28.75000000000000000, -5.000000000000000000 ) ) ;
#3972=CARTESIAN_POINT ( 'NONE',  ( 2.229367062500001939, -52.22916666530107221, 3.861377020970579999 ) ) ;
#3974=ORIENTED_EDGE ( 'NONE', *, *, #52664, .F. ) ;
#3976=CARTESIAN_POINT ( 'NONE',  ( -4.458734124999999437, 17.68750000136559208, 0.000000000000000000 ) ) ;
#3979=CARTESIAN_POINT ( 'NONE',  ( -1.846868145590737420, -165.7500000013655779, 4.458734124999997661 ) ) ;
#3981=ORIENTED_EDGE ( 'NONE', *, *, #60913, .F. ) ;
#3985=CARTESIAN_POINT ( 'NONE',  ( 5.000000000000000000, -19.37499999726881583, -6.123233995736766282E-16 ) ) ;
#3990=CARTESIAN_POINT ( 'NONE',  ( -4.458734124999999437, 29.68750000136559208, 0.000000000000000000 ) ) ;
#3994=AXIS2_PLACEMENT_3D ( 'NONE', #44911, #63582, #30098 ) ;
#3997=CARTESIAN_POINT ( 'NONE',  ( -5.000000000000000888, -151.5625000027311842, 2.071067811865474617 ) ) ;
#3998=ORIENTED_EDGE ( 'NONE', *, *, #41247, .T. ) ;
#4000=AXIS2_PLACEMENT_3D ( 'NONE', #37123, #42246, #17171 ) ;
#4004=CARTESIAN_POINT ( 'NONE',  ( 3.535533905932738197, -141.8750000000000000, -3.535533905932738197 ) ) ;
#4006=EDGE_CURVE ( 'NONE', #37366, #29442, #57589, .T. ) ;
#4008=CARTESIAN_POINT ( 'NONE',  ( -1.339745962155610925, -54.79465819873851018, 5.000000000000000000 ) ) ;
#4009=CARTESIAN_POINT ( 'NONE',  ( 4.458734125000000326, -32.89583333196774362, 2.574251347313718519 ) ) ;
#4013=CARTESIAN_POINT ( 'NONE',  ( 4.458734124999999437, -146.4375000013656063, 0.000000000000000000 ) ) ;
#4014=VERTEX_POINT ( 'NONE', #61779 ) ;
#4015=CARTESIAN_POINT ( 'NONE',  ( 2.229367062499998831, -58.89583333196773651, -3.861377020970580887 ) ) ;
#4016=( BOUNDED_CURVE ( )  B_SPLINE_CURVE ( 2, ( #2019, #35455, #45100, #56036, #1697, #31253, #20986, #54760, #46058 ),
 .UNSPECIFIED., .F., .F. ) 
 B_SPLINE_CURVE_WITH_KNOTS ( ( 3, 2, 2, 2, 3 ),
 ( 0.7687500000000000444, 0.7694444444444444864, 0.7708333333333333703, 0.7722222222222222543, 0.7729166666666666963 ),
 .UNSPECIFIED. ) 
 CURVE ( )  GEOMETRIC_REPRESENTATION_ITEM ( )  RATIONAL_B_SPLINE_CURVE ( ( 0.9330127018922194093, 0.9330127018922194093, 1.000000000000000000, 0.8660254037844387076, 1.000000000000000000, 0.8660254037844387076, 1.000000000000000000, 0.9330127018922194093, 0.9330127018922194093 ) ) 
 REPRESENTATION_ITEM ( '' )  );
#4020=CARTESIAN_POINT ( 'NONE',  ( -3.535250795749689387E-16, 17.75000000000000355, -5.773502691896257311 ) ) ;
#4021=ADVANCED_FACE ( 'NONE', ( #41819 ), #33436, .T. ) ;
#4023=CARTESIAN_POINT ( 'NONE',  ( -2.229367062499996610, -8.145833331967736513, 3.861377020970582219 ) ) ;
#4026=CARTESIAN_POINT ( 'NONE',  ( 4.458734125000001214, 9.854166668032263487, 2.574251347313718519 ) ) ;
#4027=EDGE_CURVE ( 'NONE', #31959, #12417, #29881, .T. ) ;
#4030=CARTESIAN_POINT ( 'NONE',  ( -4.458734124999999437, -47.31249999863440792, 0.000000000000000000 ) ) ;
#4032=CARTESIAN_POINT ( 'NONE',  ( -1.846868145590734756, -160.3750000013656063, -4.458734125000000326 ) ) ;
#4033=EDGE_CURVE ( 'NONE', #13136, #8193, #38898, .T. ) ;
#4034=CARTESIAN_POINT ( 'NONE',  ( 2.500000000000002220, -48.54166666393547303, 4.330127018922192761 ) ) ;
#4036=CARTESIAN_POINT ( 'NONE',  ( -4.458734124999999437, -21.39583333196774007, -2.574251347313719407 ) ) ;
#4040=CARTESIAN_POINT ( 'NONE',  ( 1.846868145590736310, -161.6250000013656063, 4.458734124999999437 ) ) ;
#4041=ORIENTED_EDGE ( 'NONE', *, *, #59246, .F. ) ;
#4042=AXIS2_PLACEMENT_3D ( 'NONE', #23320, #42921, #28447 ) ;
#4043=DIRECTION ( 'NONE',  ( -0.000000000000000000, 1.000000000000000000, -0.000000000000000000 ) ) ;
#4046=CARTESIAN_POINT ( 'NONE',  ( 9.457646018065525792E-16, -37.31249999863440792, 5.148502694627439702 ) ) ;
#4053=CARTESIAN_POINT ( 'NONE',  ( 9.457646018065525792E-16, -86.31249999863440792, 5.148502694627439702 ) ) ;
#4056=CARTESIAN_POINT ( 'NONE',  ( -5.000000000000000000, -6.999999999999999112, 0.000000000000000000 ) ) ;
#4057=CARTESIAN_POINT ( 'NONE',  ( -1.339745962155610925, -44.66965819600733312, 5.000000000000000000 ) ) ;
#4065=CARTESIAN_POINT ( 'NONE',  ( 0.000000000000000000, -170.0000000000000000, 5.000000000000000000 ) ) ;
#4066=CARTESIAN_POINT ( 'NONE',  ( -1.339745962155613812, -61.20534180126147561, -5.000000000000000000 ) ) ;
#4067=CARTESIAN_POINT ( 'NONE',  ( 2.229367062500001939, -85.22916666530107932, 3.861377020970579999 ) ) ;
#4070=ORIENTED_EDGE ( 'NONE', *, *, #3320, .F. ) ;
#4073=CARTESIAN_POINT ( 'NONE',  ( 3.061616997868383141E-16, -166.8750000027312126, -5.000000000000000000 ) ) ;
#4084=CARTESIAN_POINT ( 'NONE',  ( 2.229367062499998831, -13.64583333196774184, -3.861377020970580887 ) ) ;
#4085=DIRECTION ( 'NONE',  ( -0.000000000000000000, 1.000000000000000000, -0.000000000000000000 ) ) ;
#4087=CARTESIAN_POINT ( 'NONE',  ( 9.457646018065525792E-16, -40.31249999863440081, 5.148502694627439702 ) ) ;
#4094=AXIS2_PLACEMENT_3D ( 'NONE', #55763, #7197, #55125 ) ;
#4095=CARTESIAN_POINT ( 'NONE',  ( 2.229367062500001939, 14.02083333469892779, 3.861377020970579999 ) ) ;
#4096=CARTESIAN_POINT ( 'NONE',  ( -5.000000000000000000, -81.87499999726881583, 0.000000000000000000 ) ) ;
#4098=CARTESIAN_POINT ( 'NONE',  ( -4.458734124999997661, -88.47916666530107932, 2.574251347313722516 ) ) ;
#4100=CARTESIAN_POINT ( 'NONE',  ( 5.000000000000000000, 13.70833333606451987, -2.886751345948129988 ) ) ;
#4106=CARTESIAN_POINT ( 'NONE',  ( -2.499999999999996447, -28.83333333333333570, 4.330127018922195425 ) ) ;
#4107=CARTESIAN_POINT ( 'NONE',  ( -4.458734124999998549, -31.22916666530107221, 2.574251347313722516 ) ) ;
#4110=CARTESIAN_POINT ( 'NONE',  ( 2.499999999999998668, -36.20833333060213732, -4.330127018922193649 ) ) ;
#4111=CARTESIAN_POINT ( 'NONE',  ( 9.457646018065525792E-16, -63.06249999863440081, 5.148502694627439702 ) ) ;
#4114=CARTESIAN_POINT ( 'NONE',  ( -3.152548672688508926E-16, -13.81249999863440436, -5.148502694627439702 ) ) ;
#4116=CARTESIAN_POINT ( 'NONE',  ( -4.999999999999999112, -78.91666666666665719, 2.886751345948131764 ) ) ;
#4119=CARTESIAN_POINT ( 'NONE',  ( 5.000000000000000888, -83.45833333060213022, 2.886751345948126879 ) ) ;
#4120=LINE ( 'NONE', #8622, #6672 ) ;
#4123=CARTESIAN_POINT ( 'NONE',  ( -4.458734124999998549, -22.47916666530107577, 2.574251347313722516 ) ) ;
#4124=CARTESIAN_POINT ( 'NONE',  ( -4.458734124999999437, -55.56249999863440081, 0.000000000000000000 ) ) ;
#4127=CARTESIAN_POINT ( 'NONE',  ( -8.190561711645485556E-16, -167.9375000013655779, 4.458734124999999437 ) ) ;
#4129=CARTESIAN_POINT ( 'NONE',  ( -2.499999999999996447, 18.16666666666666430, 4.330127018922195425 ) ) ;
#4130=ORIENTED_EDGE ( 'NONE', *, *, #42035, .F. ) ;
#4138=CARTESIAN_POINT ( 'NONE',  ( 4.458734124999999437, -142.7500000013656063, 1.846868145590737864 ) ) ;
#4140=CARTESIAN_POINT ( 'NONE',  ( 1.339745962155615144, -70.70534180126148271, 4.999999999999999112 ) ) ;
#4142=CARTESIAN_POINT ( 'NONE',  ( -2.229367062500000163, -69.72916666530107932, -3.861377020970580443 ) ) ;
#4144=CARTESIAN_POINT ( 'NONE',  ( -1.339745962155610925, -42.66965819600731891, 5.000000000000000000 ) ) ;
#4145=CARTESIAN_POINT ( 'NONE',  ( -4.458734125000000326, -141.8750000013656063, 1.846868145590734089 ) ) ;
#4148=FACE_OUTER_BOUND ( 'NONE', #35499, .T. ) ;
#4153=CARTESIAN_POINT ( 'NONE',  ( 5.000000000000000000, -14.37499999726881228, -6.123233995736766282E-16 ) ) ;
#4155=CARTESIAN_POINT ( 'NONE',  ( 9.457646018065525792E-16, 22.68750000136559564, 5.148502694627439702 ) ) ;
#4156=CARTESIAN_POINT ( 'NONE',  ( 0.000000000000000000, -170.0000000000000000, 0.000000000000000000 ) ) ;
#4161=( BOUNDED_CURVE ( )  B_SPLINE_CURVE ( 2, ( #3655, #12351, #13294, #7532, #42558, #27144, #42872, #37429, #18435 ),
 .UNSPECIFIED., .F., .F. ) 
 B_SPLINE_CURVE_WITH_KNOTS ( ( 3, 2, 2, 2, 3 ),
 ( 0.6583333333333329929, 0.6624999999999996447, 0.6666666666666662966, 0.6708333333333328374, 0.6749999999999996003 ),
 .UNSPECIFIED. ) 
 CURVE ( )  GEOMETRIC_REPRESENTATION_ITEM ( )  RATIONAL_B_SPLINE_CURVE ( ( 1.000000000000005995, 0.9238795325112806323, 1.000000000000000000, 0.9238795325112867385, 1.000000000000000000, 0.9238795325112867385, 1.000000000000000000, 0.9238795325112948431, 0.9999999999999918954 ) ) 
 REPRESENTATION_ITEM ( '' )  );
#4162=CARTESIAN_POINT ( 'NONE',  ( 1.975475456537005874E-15, -60.62499999726880162, 5.000000000000000000 ) ) ;
#4163=CARTESIAN_POINT ( 'NONE',  ( 4.458734124999998549, 0.2708333346989263979, -2.574251347313721627 ) ) ;
#4164=CARTESIAN_POINT ( 'NONE',  ( 2.229367062499998831, -24.89583333196773651, -3.861377020970580887 ) ) ;
#4165=( BOUNDED_CURVE ( )  B_SPLINE_CURVE ( 2, ( #57438, #37183, #17238, #56808, #3405, #41661, #62580, #42624, #47762 ),
 .UNSPECIFIED., .F., .F. ) 
 B_SPLINE_CURVE_WITH_KNOTS ( ( 3, 2, 2, 2, 3 ),
 ( 0.02500000000000002220, 0.02916666666666669488, 0.03333333333333336757, 0.03750000000000003331, 0.04166666666666670599 ),
 .UNSPECIFIED. ) 
 CURVE ( )  GEOMETRIC_REPRESENTATION_ITEM ( )  RATIONAL_B_SPLINE_CURVE ( ( 0.9999999999999996669, 0.9238795325112870716, 1.000000000000000000, 0.9238795325112867385, 1.000000000000000000, 0.9238795325112867385, 1.000000000000000000, 0.9238795325112859613, 1.000000000000000666 ) ) 
 REPRESENTATION_ITEM ( '' )  );
#4166=CARTESIAN_POINT ( 'NONE',  ( 2.730187237215162345E-16, -155.1875000013655779, -4.458734124999999437 ) ) ;
#4169=FACE_OUTER_BOUND ( 'NONE', #6587, .T. ) ;
#4172=CARTESIAN_POINT ( 'NONE',  ( 4.458734125000000326, -74.14583333196773651, 2.574251347313718519 ) ) ;
#4174=CARTESIAN_POINT ( 'NONE',  ( -6.972266317189433020E-16, -66.12499999726881583, -5.000000000000000000 ) ) ;
#4175=CARTESIAN_POINT ( 'NONE',  ( -5.000000000000000000, 27.12500000273118772, 0.000000000000000000 ) ) ;
#4176=ORIENTED_EDGE ( 'NONE', *, *, #46858, .F. ) ;
#4177=CARTESIAN_POINT ( 'NONE',  ( 5.000000000000000000, 6.583333333333333037, -2.886751345948130876 ) ) ;
#4179=CARTESIAN_POINT ( 'NONE',  ( 5.000000000000000888, -11.58333333333333570, 2.886751345948126879 ) ) ;
#4180=CARTESIAN_POINT ( 'NONE',  ( 2.229367062500001939, -14.97916666530107399, 3.861377020970579999 ) ) ;
#4181=VECTOR ( 'NONE', #37085, 1000.000000000000000 ) ;
#4182=CARTESIAN_POINT ( 'NONE',  ( 2.229367062499998831, -76.64583333196773651, -3.861377020970580887 ) ) ;
#4183=CARTESIAN_POINT ( 'NONE',  ( 2.730187237215162345E-16, -166.4375000013655779, -4.458734124999999437 ) ) ;
#4184=CARTESIAN_POINT ( 'NONE',  ( -5.000000000000000000, -17.95833333060214798, -2.886751345948128211 ) ) ;
#4185=CARTESIAN_POINT ( 'NONE',  ( 4.458734124999998549, -44.72916666530106511, -2.574251347313721627 ) ) ;
#4188=CARTESIAN_POINT ( 'NONE',  ( 4.458734124999999437, 7.937500001365595637, -5.460374474430324690E-16 ) ) ;
#4189=ORIENTED_EDGE ( 'NONE', *, *, #46406, .F. ) ;
#4190=( BOUNDED_CURVE ( )  B_SPLINE_CURVE ( 2, ( #42932, #33286, #52905, #27508, #13972, #48069, #53219, #9151, #28763 ),
 .UNSPECIFIED., .F., .F. ) 
 B_SPLINE_CURVE_WITH_KNOTS ( ( 3, 2, 2, 2, 3 ),
 ( 0.5083333333333337478, 0.5125000000000003997, 0.5166666666666671626, 0.5208333333333338144, 0.5250000000000004663 ),
 .UNSPECIFIED. ) 
 CURVE ( )  GEOMETRIC_REPRESENTATION_ITEM ( )  RATIONAL_B_SPLINE_CURVE ( ( 0.9999999999999918954, 0.9238795325112948431, 1.000000000000000000, 0.9238795325112867385, 1.000000000000000000, 0.9238795325112867385, 1.000000000000000000, 0.9238795325112786339, 1.000000000000008216 ) ) 
 REPRESENTATION_ITEM ( '' )  );
#4192=CARTESIAN_POINT ( 'NONE',  ( -5.000000000000000000, -62.08333333333332860, -2.886751345948128211 ) ) ;
#4193=CARTESIAN_POINT ( 'NONE',  ( 1.846868145590736310, -154.8750000013655779, 4.458734124999999437 ) ) ;
#4195=CARTESIAN_POINT ( 'NONE',  ( -4.999999999999998224, -78.91666666666665719, 2.886751345948131764 ) ) ;
#4196=CARTESIAN_POINT ( 'NONE',  ( -5.000000000000000000, -163.5000000000000000, -6.123233995736766282E-16 ) ) ;
#4197=CARTESIAN_POINT ( 'NONE',  ( 1.975475456537005874E-15, 5.375000002731185944, 5.000000000000000000 ) ) ;
#4199=CARTESIAN_POINT ( 'NONE',  ( -4.458734124999998549, -8.479166665301073991, 2.574251347313722516 ) ) ;
#4200=CARTESIAN_POINT ( 'NONE',  ( -2.229367062499996610, -41.39583333196773651, 3.861377020970582219 ) ) ;
#4202=CARTESIAN_POINT ( 'NONE',  ( -4.458734124999999437, -148.9375000013656063, -5.460374474430324690E-16 ) ) ;
#4208=( BOUNDED_CURVE ( )  B_SPLINE_CURVE ( 2, ( #32220, #57004, #37682, #42504, #2977, #22594, #56691, #61833, #42191 ),
 .UNSPECIFIED., .F., .F. ) 
 B_SPLINE_CURVE_WITH_KNOTS ( ( 3, 2, 2, 2, 3 ),
 ( 0.8104166666666666741, 0.8111111111111111160, 0.8125000000000000000, 0.8138888888888888840, 0.8145833333333333259 ),
 .UNSPECIFIED. ) 
 CURVE ( )  GEOMETRIC_REPRESENTATION_ITEM ( )  RATIONAL_B_SPLINE_CURVE ( ( 0.9330127018922194093, 0.9330127018922194093, 1.000000000000000000, 0.8660254037844387076, 1.000000000000000000, 0.8660254037844387076, 1.000000000000000000, 0.9330127018922194093, 0.9330127018922194093 ) ) 
 REPRESENTATION_ITEM ( '' )  );
#4210=CARTESIAN_POINT ( 'NONE',  ( -2.229367062499996610, -76.39583333196773651, 3.861377020970582219 ) ) ;
#4211=EDGE_CURVE ( 'NONE', #8687, #17322, #47553, .T. ) ;
#4215=CARTESIAN_POINT ( 'NONE',  ( 2.500000000000002220, -79.54166666393547303, 4.330127018922192761 ) ) ;
#4216=CARTESIAN_POINT ( 'NONE',  ( 4.458734125000001214, -2.895833331967738289, 2.574251347313718519 ) ) ;
#4217=CARTESIAN_POINT ( 'NONE',  ( -5.000000000000000000, -43.00000000000000000, 0.000000000000000000 ) ) ;
#4218=CARTESIAN_POINT ( 'NONE',  ( -8.190561711645485556E-16, -152.6875000013656063, 4.458734124999999437 ) ) ;
#4220=EDGE_LOOP ( 'NONE', ( #33309, #40510, #36918, #37503 ) ) ;
#4222=DIRECTION ( 'NONE',  ( -0.000000000000000000, 1.000000000000000000, -0.000000000000000000 ) ) ;
#4231=CARTESIAN_POINT ( 'NONE',  ( 2.229367062500001939, 17.02083333469892779, 3.861377020970579999 ) ) ;
#4233=CARTESIAN_POINT ( 'NONE',  ( -4.458734124999999437, -6.562499998634403475, 0.000000000000000000 ) ) ;
#4236=CARTESIAN_POINT ( 'NONE',  ( 5.000000000000000000, -139.1875000027312126, 2.071067811865478614 ) ) ;
#4241=CARTESIAN_POINT ( 'NONE',  ( -6.972266317189433020E-16, -87.25000000000001421, -5.000000000000000000 ) ) ;
#4242=CARTESIAN_POINT ( 'NONE',  ( 6.123233995736766282E-16, -170.0000000000000000, -5.000000000000000000 ) ) ;
#4244=CARTESIAN_POINT ( 'NONE',  ( 4.458734124999999437, -153.6875000013656063, 0.000000000000000000 ) ) ;
#4247=LINE ( 'NONE', #34777, #3773 ) ;
#4253=CARTESIAN_POINT ( 'NONE',  ( 2.499999999999998668, 0.6666666666666660745, -4.330127018922193649 ) ) ;
#4254=CARTESIAN_POINT ( 'NONE',  ( -2.229367062500000163, -59.47916666530106511, -3.861377020970580443 ) ) ;
#4256=CARTESIAN_POINT ( 'NONE',  ( 1.060575238724906964E-15, 0.3750000027311871098, 5.773502691896257311 ) ) ;
#4257=CARTESIAN_POINT ( 'NONE',  ( -3.152548672688508926E-16, -26.56249999863440792, -5.148502694627439702 ) ) ;
#4258=CARTESIAN_POINT ( 'NONE',  ( 5.000000000000000888, -153.0625000027311842, -2.071067811865475505 ) ) ;
#4260=CARTESIAN_POINT ( 'NONE',  ( 5.000000000000000888, -45.58333333333333570, 2.886751345948126879 ) ) ;
#4264=CARTESIAN_POINT ( 'NONE',  ( 4.458734124999999437, -70.81249999863439371, -5.460374474430324690E-16 ) ) ;
#4265=CARTESIAN_POINT ( 'NONE',  ( -4.458734125000000326, -146.2500000013656063, -1.846868145590735644 ) ) ;
#4266=AXIS2_PLACEMENT_3D ( 'NONE', #61233, #17156, #22307 ) ;
#4267=CARTESIAN_POINT ( 'NONE',  ( 2.229367062499998831, -74.64583333196773651, -3.861377020970580887 ) ) ;
#4269=CARTESIAN_POINT ( 'NONE',  ( -4.458734124999998549, -24.47916666530107577, 2.574251347313722516 ) ) ;
#4270=CARTESIAN_POINT ( 'NONE',  ( -4.999999999999999112, -64.79166666393547303, 2.886751345948131764 ) ) ;
#4272=CARTESIAN_POINT ( 'NONE',  ( -5.000000000000000000, -22.00000000000000000, 0.000000000000000000 ) ) ;
#4273=EDGE_LOOP ( 'NONE', ( #27067, #46203, #5073, #44052 ) ) ;
#4278=CARTESIAN_POINT ( 'NONE',  ( -2.229367062500000163, -60.72916666530106511, -3.861377020970580443 ) ) ;
#4283=LINE ( 'NONE', #9725, #17313 ) ;
#4284=CARTESIAN_POINT ( 'NONE',  ( -4.458734124999999437, 16.68750000136559564, 0.000000000000000000 ) ) ;
#4287=CARTESIAN_POINT ( 'NONE',  ( -3.152801135295367096, -164.0625000013656063, -3.152801135295367541 ) ) ;
#4290=ADVANCED_FACE ( 'NONE', ( #24734 ), #34369, .T. ) ;
#4293=DIRECTION ( 'NONE',  ( -0.000000000000000000, 1.000000000000000000, -0.000000000000000000 ) ) ;
#4296=EDGE_CURVE ( 'NONE', #61790, #9668, #31966, .T. ) ;
#4299=FACE_OUTER_BOUND ( 'NONE', #41758, .T. ) ;
#4300=CARTESIAN_POINT ( 'NONE',  ( -2.071067811865622943, -156.6875000000000000, -4.999999999999850786 ) ) ;
#4303=CYLINDRICAL_SURFACE ( 'NONE', #56576, 5.000000000000000000 ) ;
#4305=CARTESIAN_POINT ( 'NONE',  ( -5.000000000000000000, -150.6250000027312126, -6.123233995736766282E-16 ) ) ;
#4310=CARTESIAN_POINT ( 'NONE',  ( -3.535533905932737309, -141.6250000000000000, -3.535533905932738197 ) ) ;
#4312=CARTESIAN_POINT ( 'NONE',  ( 3.152801135295366208, -168.8125000013656063, 3.152801135295367985 ) ) ;
#4313=CARTESIAN_POINT ( 'NONE',  ( -4.458734124999999437, -29.39583333196773296, -2.574251347313719407 ) ) ;
#4314=CARTESIAN_POINT ( 'NONE',  ( 6.123233995736766282E-16, -170.0000000000000000, -5.000000000000000000 ) ) ;
#4315=CARTESIAN_POINT ( 'NONE',  ( 5.000000000000000000, -45.29166666393547303, -2.886751345948130876 ) ) ;
#4317=CARTESIAN_POINT ( 'NONE',  ( -4.458734124999999437, -144.9375000013656063, -5.460374474430324690E-16 ) ) ;
#4318=EDGE_LOOP ( 'NONE', ( #52133, #40142, #37149, #20318 ) ) ;
#4319=CARTESIAN_POINT ( 'NONE',  ( 4.458734124999999437, 28.93750000136559208, -5.460374474430324690E-16 ) ) ;
#4321=CARTESIAN_POINT ( 'NONE',  ( -4.458734124999999437, -58.56249999863440081, 0.000000000000000000 ) ) ;
#4324=CARTESIAN_POINT ( 'NONE',  ( -4.999999999999999112, 18.08333333333333570, 2.886751345948131764 ) ) ;
#4326=CARTESIAN_POINT ( 'NONE',  ( -3.152548672688508926E-16, -6.562499998634404363, -5.148502694627439702 ) ) ;
#4327=CARTESIAN_POINT ( 'NONE',  ( -6.972266317189433020E-16, 3.875000002731185500, -5.000000000000000000 ) ) ;
#4329=CARTESIAN_POINT ( 'NONE',  ( -2.499999999999996447, -8.833333333333332149, 4.330127018922195425 ) ) ;
#4330=CARTESIAN_POINT ( 'NONE',  ( 2.229367062500001939, 12.77083333469892779, 3.861377020970579999 ) ) ;
#4333=CARTESIAN_POINT ( 'NONE',  ( -2.229367062499996610, -55.14583333196773651, 3.861377020970582219 ) ) ;
#4334=CARTESIAN_POINT ( 'NONE',  ( -8.190561711645485556E-16, -158.9375000013655779, 4.458734124999999437 ) ) ;
#4335=CARTESIAN_POINT ( 'NONE',  ( -2.499999999999996447, -52.70833333060213732, 4.330127018922195425 ) ) ;
#4337=CARTESIAN_POINT ( 'NONE',  ( 4.458734125000001214, 4.854166668032262599, 2.574251347313718519 ) ) ;
#4341=CARTESIAN_POINT ( 'NONE',  ( -4.458734124999999437, -158.9375000013655779, -5.460374474430324690E-16 ) ) ;
#4342=ORIENTED_EDGE ( 'NONE', *, *, #36617, .T. ) ;
#4345=CARTESIAN_POINT ( 'NONE',  ( 1.339745962155615144, -47.58034179853029144, 4.999999999999999112 ) ) ;
#4346=CARTESIAN_POINT ( 'NONE',  ( 4.458734125000001214, -38.14583333196773651, 2.574251347313718519 ) ) ;
#4349=EDGE_CURVE ( 'NONE', #40158, #8193, #15408, .T. ) ;
#4350=FACE_OUTER_BOUND ( 'NONE', #34825, .T. ) ;
#4352=CARTESIAN_POINT ( 'NONE',  ( 5.000000000000000000, -59.41666666666665719, -2.886751345948130876 ) ) ;
#4354=CARTESIAN_POINT ( 'NONE',  ( -4.458734124999999437, -85.56249999863439371, 0.000000000000000000 ) ) ;
#4357=CARTESIAN_POINT ( 'NONE',  ( -6.972266317189433020E-16, -26.25000000000000355, -5.000000000000000000 ) ) ;
#4358=CARTESIAN_POINT ( 'NONE',  ( 5.000000000000000000, -52.37499999726881583, -6.123233995736766282E-16 ) ) ;
#4360=CARTESIAN_POINT ( 'NONE',  ( 5.275681513340003914E-14, 9.875000002731184168, -5.000000000000000000 ) ) ;
#4362=EDGE_CURVE ( 'NONE', #12432, #1054, #9300, .T. ) ;
#4367=CARTESIAN_POINT ( 'NONE',  ( -1.339745962155617365, 25.20534180126147916, 4.999999999999998224 ) ) ;
#4369=DIRECTION ( 'NONE',  ( -0.000000000000000000, 1.000000000000000000, -0.000000000000000000 ) ) ;
#4370=CARTESIAN_POINT ( 'NONE',  ( 4.458734124999999437, -85.06249999863439371, -5.460374474430324690E-16 ) ) ;
#4376=CARTESIAN_POINT ( 'NONE',  ( -5.000000000000000000, -162.6250000027311842, -6.123233995736766282E-16 ) ) ;
#4385=CARTESIAN_POINT ( 'NONE',  ( -6.972266317189433020E-16, -20.24999999999999289, -5.000000000000000000 ) ) ;
#4386=CARTESIAN_POINT ( 'NONE',  ( -4.458734124999999437, -14.31249999863440436, 0.000000000000000000 ) ) ;
#4387=CARTESIAN_POINT ( 'NONE',  ( -6.972266317189433020E-16, -71.25000000000000000, -5.000000000000000000 ) ) ;
#4388=CARTESIAN_POINT ( 'NONE',  ( 3.535533905932738197, -153.8750000000000000, -3.535533905932738197 ) ) ;
#4390=CARTESIAN_POINT ( 'NONE',  ( -2.229367062499996610, -38.39583333196773651, 3.861377020970582219 ) ) ;
#4393=CARTESIAN_POINT ( 'NONE',  ( -4.999999999999998224, 27.20833333606451276, 2.886751345948131764 ) ) ;
#4396=CARTESIAN_POINT ( 'NONE',  ( -2.229367062499996610, 9.854166668032261711, 3.861377020970582219 ) ) ;
#4397=DIRECTION ( 'NONE',  ( -0.000000000000000000, 1.000000000000000000, -0.000000000000000000 ) ) ;
#4398=CARTESIAN_POINT ( 'NONE',  ( -2.499999999999996447, 12.16666666666666607, 4.330127018922195425 ) ) ;
#4399=CARTESIAN_POINT ( 'NONE',  ( -4.458734124999999437, -87.56249999863439371, 0.000000000000000000 ) ) ;
#4401=CARTESIAN_POINT ( 'NONE',  ( 5.000000000000000888, 12.54166666939785202, 2.886751345948126879 ) ) ;
#4403=ORIENTED_EDGE ( 'NONE', *, *, #35438, .F. ) ;
#4405=CARTESIAN_POINT ( 'NONE',  ( 1.339745962155612702, -85.29465819873851729, -5.000000000000000000 ) ) ;
#4406=CARTESIAN_POINT ( 'NONE',  ( 2.500000000000002220, -30.66666666666666785, 4.330127018922192761 ) ) ;
#4407=CARTESIAN_POINT ( 'NONE',  ( 2.229367062500001939, -33.97916666530107221, 3.861377020970579999 ) ) ;
#4408=CARTESIAN_POINT ( 'NONE',  ( 5.000000000000000000, -35.37499999726881583, -6.123233995736766282E-16 ) ) ;
#4409=CARTESIAN_POINT ( 'NONE',  ( -2.229367062500000163, -66.47916666530106511, -3.861377020970580443 ) ) ;
#4412=CARTESIAN_POINT ( 'NONE',  ( -3.152548672688508926E-16, -11.56249999863440792, -5.148502694627439702 ) ) ;
#4413=CARTESIAN_POINT ( 'NONE',  ( 2.229367062499998831, -15.89583333196773651, -3.861377020970580887 ) ) ;
#4415=CARTESIAN_POINT ( 'NONE',  ( -4.999999999999999112, -77.91666666666665719, 2.886751345948131764 ) ) ;
#4418=CARTESIAN_POINT ( 'NONE',  ( -5.000000000000000000, -83.87499999726880162, 0.000000000000000000 ) ) ;
#4420=ORIENTED_EDGE ( 'NONE', *, *, #6002, .F. ) ;
#4422=CARTESIAN_POINT ( 'NONE',  ( 4.458734124999998549, -23.97916666530107221, -2.574251347313721627 ) ) ;
#4423=CARTESIAN_POINT ( 'NONE',  ( -4.458734124999998549, -60.47916666530105800, 2.574251347313722516 ) ) ;
#4427=CARTESIAN_POINT ( 'NONE',  ( 4.458734124999999437, -167.6875000013655779, 0.000000000000000000 ) ) ;
#4437=CARTESIAN_POINT ( 'NONE',  ( 4.458734124999999437, -145.6875000013656063, 0.000000000000000000 ) ) ;
#4441=CARTESIAN_POINT ( 'NONE',  ( 4.458734124999998549, -68.97916666530106511, -2.574251347313721627 ) ) ;
#4442=ADVANCED_FACE ( 'NONE', ( #957 ), #31457, .T. ) ;
#4444=CARTESIAN_POINT ( 'NONE',  ( -1.339745962155610925, -0.6696581960073348938, 5.000000000000000000 ) ) ;
#4445=CARTESIAN_POINT ( 'NONE',  ( 4.458734124999997661, -140.5000000013655779, 1.846868145590737864 ) ) ;
#4447=EDGE_LOOP ( 'NONE', ( #60557, #30535, #51293, #60827 ) ) ;
#4448=CARTESIAN_POINT ( 'NONE',  ( -2.499999999999996447, -70.70833333060214443, 4.330127018922195425 ) ) ;
#4455=CARTESIAN_POINT ( 'NONE',  ( 4.458734124999999437, 23.93750000136559564, -5.460374474430324690E-16 ) ) ;
#4463=DIRECTION ( 'NONE',  ( -0.000000000000000000, 1.000000000000000000, -0.000000000000000000 ) ) ;
#4464=CARTESIAN_POINT ( 'NONE',  ( 4.458734125000000326, -0.8958333319677401763, 2.574251347313718519 ) ) ;
#4466=CARTESIAN_POINT ( 'NONE',  ( 9.457646018065525792E-16, -27.31249999863440081, 5.148502694627439702 ) ) ;
#4467=CARTESIAN_POINT ( 'NONE',  ( 1.846868145590736310, -157.6250000013655779, 4.458734124999999437 ) ) ;
#4471=CARTESIAN_POINT ( 'NONE',  ( 2.229367062499998831, 24.35416666803225993, -3.861377020970580887 ) ) ;
#4472=CARTESIAN_POINT ( 'NONE',  ( 0.000000000000000000, -170.0000000000000000, 0.000000000000000000 ) ) ;
#4473=CARTESIAN_POINT ( 'NONE',  ( 2.229367062500001939, -74.22916666530106511, 3.861377020970579999 ) ) ;
#4475=DIRECTION ( 'NONE',  ( -0.000000000000000000, 1.000000000000000000, -0.000000000000000000 ) ) ;
#4476=CARTESIAN_POINT ( 'NONE',  ( 0.000000000000000000, -170.0000000000000000, 0.000000000000000000 ) ) ;
#4478=CARTESIAN_POINT ( 'NONE',  ( 5.000000000000000888, 6.416666666666667851, 2.886751345948126879 ) ) ;
#4479=CARTESIAN_POINT ( 'NONE',  ( 1.339745962155615144, -89.58034179853028434, 4.999999999999999112 ) ) ;
#4480=CARTESIAN_POINT ( 'NONE',  ( -2.500000000000000444, -15.16666666666666785, -4.330127018922193649 ) ) ;
#4481=CARTESIAN_POINT ( 'NONE',  ( -4.458734124999999437, -15.39583333196773474, -2.574251347313719407 ) ) ;
#4482=CARTESIAN_POINT ( 'NONE',  ( 2.229367062499998831, -78.64583333196773651, -3.861377020970580887 ) ) ;
#4483=CARTESIAN_POINT ( 'NONE',  ( -1.846868145590734756, -168.3750000013655779, -4.458734125000000326 ) ) ;
#4484=CARTESIAN_POINT ( 'NONE',  ( 1.060575238724906964E-15, -15.62499999726881406, 5.773502691896257311 ) ) ;
#4485=CARTESIAN_POINT ( 'NONE',  ( 2.229367062499998831, -47.64583333196774362, -3.861377020970580887 ) ) ;
#4486=ORIENTED_EDGE ( 'NONE', *, *, #55946, .T. ) ;
#4488=CARTESIAN_POINT ( 'NONE',  ( -4.458734124999998549, -0.4791666653010707710, 2.574251347313722516 ) ) ;
#4489=ORIENTED_EDGE ( 'NONE', *, *, #23699, .T. ) ;
#4491=CARTESIAN_POINT ( 'NONE',  ( 5.000000000000000888, -59.58333333333334281, 2.886751345948126879 ) ) ;
#4492=CARTESIAN_POINT ( 'NONE',  ( -1.846868145590734756, -154.3750000013655779, -4.458734125000000326 ) ) ;
#4494=CARTESIAN_POINT ( 'NONE',  ( -2.500000000000000444, -65.16666666666667140, -4.330127018922193649 ) ) ;
#4495=CARTESIAN_POINT ( 'NONE',  ( -5.000000000000000000, -162.5000000000000000, -6.123233995736766282E-16 ) ) ;
#4498=CARTESIAN_POINT ( 'NONE',  ( 2.229367062499998831, -3.895833331967739177, -3.861377020970580887 ) ) ;
#4499=CARTESIAN_POINT ( 'NONE',  ( -2.229367062499996610, -45.39583333196774362, 3.861377020970582219 ) ) ;
#4502=CARTESIAN_POINT ( 'NONE',  ( 0.000000000000000000, -170.0000000000000000, 5.000000000000000000 ) ) ;
#4503=CARTESIAN_POINT ( 'NONE',  ( 4.458734124999999437, -149.5000000013655779, 1.846868145590737864 ) ) ;
#4506=ORIENTED_EDGE ( 'NONE', *, *, #59887, .F. ) ;
#4507=CARTESIAN_POINT ( 'NONE',  ( 2.071067811865306751, -154.9375000027311842, -5.000000000000171418 ) ) ;
#4508=CARTESIAN_POINT ( 'NONE',  ( -5.000000000000000000, -68.95833333060214443, -2.886751345948128211 ) ) ;
#4510=CARTESIAN_POINT ( 'NONE',  ( -6.972266317189433020E-16, -12.12499999726881406, -5.000000000000000000 ) ) ;
#4515=CARTESIAN_POINT ( 'NONE',  ( 9.457646018065525792E-16, -3.062499998634407472, 5.148502694627439702 ) ) ;
#4517=CARTESIAN_POINT ( 'NONE',  ( -4.458734124999999437, -152.9375000013655779, -5.460374474430324690E-16 ) ) ;
#4522=CARTESIAN_POINT ( 'NONE',  ( -5.000000000000000000, -47.08333333333333570, -2.886751345948128211 ) ) ;
#4523=CARTESIAN_POINT ( 'NONE',  ( 5.000000000000000000, -40.41666666666667140, -2.886751345948130876 ) ) ;
#4532=ORIENTED_EDGE ( 'NONE', *, *, #9074, .T. ) ;
#4533=CARTESIAN_POINT ( 'NONE',  ( 2.229367062499998831, 18.35416666803225993, -3.861377020970580887 ) ) ;
#4535=CARTESIAN_POINT ( 'NONE',  ( 2.229367062500001939, -7.229166665301073103, 3.861377020970579999 ) ) ;
#4537=CARTESIAN_POINT ( 'NONE',  ( -4.458734125000001214, -165.8750000013656063, 1.846868145590734089 ) ) ;
#4538=CARTESIAN_POINT ( 'NONE',  ( 1.975475456537005874E-15, -35.62499999726880162, 5.000000000000000000 ) ) ;
#4542=AXIS2_PLACEMENT_3D ( 'NONE', #54084, #58911, #24822 ) ;
#4545=CARTESIAN_POINT ( 'NONE',  ( -4.458734124999999437, -152.2500000013656063, -1.846868145590735644 ) ) ;
#4548=CARTESIAN_POINT ( 'NONE',  ( 0.000000000000000000, -170.0000000000000000, 5.000000000000000000 ) ) ;
#4549=ORIENTED_EDGE ( 'NONE', *, *, #748, .T. ) ;
#4553=CARTESIAN_POINT ( 'NONE',  ( -4.999999999999999112, 1.083333333333331927, 2.886751345948131764 ) ) ;
#4554=CARTESIAN_POINT ( 'NONE',  ( -3.152548672688508926E-16, -62.56249999863440792, -5.148502694627439702 ) ) ;
#4555=CARTESIAN_POINT ( 'NONE',  ( -5.000000000000000000, 19.99999999999999645, 0.000000000000000000 ) ) ;
#4556=CARTESIAN_POINT ( 'NONE',  ( 5.000000000000000000, -3.374999997268816276, -6.123233995736766282E-16 ) ) ;
#4557=CARTESIAN_POINT ( 'NONE',  ( -3.152548672688508926E-16, -30.56249999863440436, -5.148502694627439702 ) ) ;
#4560=CARTESIAN_POINT ( 'NONE',  ( 5.000000000000000000, -157.0000000000000000, 0.000000000000000000 ) ) ;
#4561=CARTESIAN_POINT ( 'NONE',  ( 0.000000000000000000, -170.0000000000000000, 0.000000000000000000 ) ) ;
#4562=CARTESIAN_POINT ( 'NONE',  ( 2.499999999999998668, -46.33333333333333570, -4.330127018922193649 ) ) ;
#4565=CARTESIAN_POINT ( 'NONE',  ( -6.972266317189433020E-16, -4.124999997268814056, -5.000000000000000000 ) ) ;
#4566=CARTESIAN_POINT ( 'NONE',  ( 4.458734125000001214, -67.89583333196773651, 2.574251347313718519 ) ) ;
#4568=CARTESIAN_POINT ( 'NONE',  ( 3.152801135295367541, -143.5625000013655779, -3.152801135295367541 ) ) ;
#4569=CARTESIAN_POINT ( 'NONE',  ( -2.229367062499996610, -75.14583333196773651, 3.861377020970582219 ) ) ;
#4571=CARTESIAN_POINT ( 'NONE',  ( 4.458734124999998549, -24.97916666530106511, -2.574251347313721627 ) ) ;
#4572=CARTESIAN_POINT ( 'NONE',  ( -2.499999999999996447, -67.70833333060214443, 4.330127018922195425 ) ) ;
#4574=CARTESIAN_POINT ( 'NONE',  ( -2.071067811865308972, -152.4375000027312126, 5.000000000000169642 ) ) ;
#4577=CARTESIAN_POINT ( 'NONE',  ( 3.061616997868383141E-16, -147.8750000027312126, -5.000000000000000000 ) ) ;
#4579=VERTEX_POINT ( 'NONE', #61075 ) ;
#4580=EDGE_CURVE ( 'NONE', #35184, #13144, #21644, .T. ) ;
#4581=CARTESIAN_POINT ( 'NONE',  ( -5.000000000000000000, -39.08333333333332860, -2.886751345948128211 ) ) ;
#4582=CYLINDRICAL_SURFACE ( 'NONE', #14733, 5.000000000000000000 ) ;
#4583=CARTESIAN_POINT ( 'NONE',  ( 4.458734125000001214, -59.14583333196773651, 2.574251347313718519 ) ) ;
#4585=ORIENTED_EDGE ( 'NONE', *, *, #50779, .F. ) ;
#4587=CARTESIAN_POINT ( 'NONE',  ( -2.071067811865562991, -146.3124999999999716, 4.999999999999913847 ) ) ;
#4589=CARTESIAN_POINT ( 'NONE',  ( -4.458734124999998549, 10.77083333469892956, 2.574251347313722516 ) ) ;
#4592=CARTESIAN_POINT ( 'NONE',  ( -1.846868145590737420, -164.7500000013655779, 4.458734124999997661 ) ) ;
#4595=DIRECTION ( 'NONE',  ( -0.000000000000000000, 1.000000000000000000, -0.000000000000000000 ) ) ;
#4597=CARTESIAN_POINT ( 'NONE',  ( -3.535533905932737309, -162.7500000027312126, -3.535533905932738197 ) ) ;
#4600=CARTESIAN_POINT ( 'NONE',  ( -5.000000000000000000, 5.999999999999998224, 0.000000000000000000 ) ) ;
#4602=CARTESIAN_POINT ( 'NONE',  ( -6.972266317189433020E-16, -31.24999999999999645, -5.000000000000000000 ) ) ;
#4603=CARTESIAN_POINT ( 'NONE',  ( 2.499999999999998668, -58.33333333333333570, -4.330127018922193649 ) ) ;
#4606=CARTESIAN_POINT ( 'NONE',  ( 2.229367062499998831, 8.104166668032261711, -3.861377020970580887 ) ) ;
#4607=CYLINDRICAL_SURFACE ( 'NONE', #25713, 5.000000000000000000 ) ;
#4609=CARTESIAN_POINT ( 'NONE',  ( -3.535533905932738641, -150.5000000027312126, 3.535533905932737309 ) ) ;
#4614=CARTESIAN_POINT ( 'NONE',  ( 3.535533905932738197, -143.8750000000000000, -3.535533905932738197 ) ) ;
#4616=CARTESIAN_POINT ( 'NONE',  ( 1.846868145590736310, -164.8750000013656063, 4.458734124999997661 ) ) ;
#4617=CARTESIAN_POINT ( 'NONE',  ( -4.458734124999999437, -31.31249999863440436, 0.000000000000000000 ) ) ;
#4621=CARTESIAN_POINT ( 'NONE',  ( 4.458734124999999437, -144.4375000013656063, 0.000000000000000000 ) ) ;
#4623=CARTESIAN_POINT ( 'NONE',  ( 4.458734124999998549, 27.02083333469892423, -2.574251347313721627 ) ) ;
#4625=CARTESIAN_POINT ( 'NONE',  ( 4.458734124999998549, -54.97916666530107221, -2.574251347313721627 ) ) ;
#4627=CARTESIAN_POINT ( 'NONE',  ( 1.339745962155612702, -90.16965819600733312, -5.000000000000000000 ) ) ;
#4628=CARTESIAN_POINT ( 'NONE',  ( 2.499999999999998668, 19.66666666666666430, -4.330127018922193649 ) ) ;
#4629=EDGE_CURVE ( 'NONE', #51386, #30756, #25696, .T. ) ;
#4631=AXIS2_PLACEMENT_3D ( 'NONE', #62462, #13238, #51848 ) ;
#4632=CARTESIAN_POINT ( 'NONE',  ( -2.229367062500000163, -4.479166665301070438, -3.861377020970580443 ) ) ;
#4633=CARTESIAN_POINT ( 'NONE',  ( 5.000000000000000000, -166.1875000027311842, 2.071067811865478614 ) ) ;
#4636=CARTESIAN_POINT ( 'NONE',  ( -6.972266317189433020E-16, -51.12499999726880873, -5.000000000000000000 ) ) ;
#4639=CARTESIAN_POINT ( 'NONE',  ( 4.458734124999999437, -52.81249999863440792, -5.460374474430324690E-16 ) ) ;
#4640=CARTESIAN_POINT ( 'NONE',  ( 3.152801135295366208, -156.8125000013656063, 3.152801135295367985 ) ) ;
#4642=EDGE_CURVE ( 'NONE', #5304, #16689, #28201, .T. ) ;
#4643=CARTESIAN_POINT ( 'NONE',  ( 2.500000000000002220, -49.54166666393547303, 4.330127018922192761 ) ) ;
#4645=CARTESIAN_POINT ( 'NONE',  ( -4.458734124999999437, 6.437500001365593860, 0.000000000000000000 ) ) ;
#4646=EDGE_CURVE ( 'NONE', #26438, #46520, #27830, .T. ) ;
#4650=CARTESIAN_POINT ( 'NONE',  ( 4.458734125000000326, -159.3750000013656347, -1.846868145590734978 ) ) ;
#4655=CARTESIAN_POINT ( 'NONE',  ( 4.458734125000001214, -43.14583333196773651, 2.574251347313718519 ) ) ;
#4658=CARTESIAN_POINT ( 'NONE',  ( 5.000000000000000000, -143.1250000027312126, 0.000000000000000000 ) ) ;
#4662=CARTESIAN_POINT ( 'NONE',  ( -4.458734124999999437, -90.56249999863440792, 0.000000000000000000 ) ) ;
#4665=CARTESIAN_POINT ( 'NONE',  ( 2.071067811865484387, -169.1875000000000284, 4.999999999999991118 ) ) ;
#4667=CARTESIAN_POINT ( 'NONE',  ( -4.999999999999998224, -61.79166666393547303, 2.886751345948131764 ) ) ;
#4669=AXIS2_PLACEMENT_3D ( 'NONE', #35470, #40289, #55413 ) ;
#4670=CARTESIAN_POINT ( 'NONE',  ( 1.975475456537005874E-15, -81.74999999999998579, 5.000000000000000000 ) ) ;
#4672=EDGE_CURVE ( 'NONE', #33371, #35072, #62779, .T. ) ;
#4674=LINE ( 'NONE', #9194, #23240 ) ;
#4675=CARTESIAN_POINT ( 'NONE',  ( 1.975475456537005874E-15, -19.62499999726881228, 5.000000000000000000 ) ) ;
#4676=CARTESIAN_POINT ( 'NONE',  ( -4.458734124999999437, -82.56249999863440792, 0.000000000000000000 ) ) ;
#4680=CARTESIAN_POINT ( 'NONE',  ( 5.000000000000000000, -9.374999997268814056, -6.123233995736766282E-16 ) ) ;
#4682=CARTESIAN_POINT ( 'NONE',  ( 2.071067811865475505, -161.9375000027311842, -5.000000000000000888 ) ) ;
#4684=CARTESIAN_POINT ( 'NONE',  ( 5.000000000000000888, -163.0625000027312410, -2.071067811865475505 ) ) ;
#4692=CARTESIAN_POINT ( 'NONE',  ( -2.499999999999996447, -53.83333333333332860, 4.330127018922195425 ) ) ;
#4693=CARTESIAN_POINT ( 'NONE',  ( -4.458734124999997661, -14.22916666530107221, 2.574251347313722516 ) ) ;
#4694=CARTESIAN_POINT ( 'NONE',  ( -9.184850993605147944E-16, -146.2500000000000284, 5.000000000000000000 ) ) ;
#4695=CARTESIAN_POINT ( 'NONE',  ( -2.071067811865478170, -155.3125000000000284, 5.000000000000000000 ) ) ;
#4698=CARTESIAN_POINT ( 'NONE',  ( -4.458734124999999437, -40.56249999863440081, 0.000000000000000000 ) ) ;
#4699=CARTESIAN_POINT ( 'NONE',  ( 2.500000000000002220, -83.54166666393547303, 4.330127018922192761 ) ) ;
#4704=EDGE_CURVE ( 'NONE', #42419, #7188, #6055, .T. ) ;
#4705=CARTESIAN_POINT ( 'NONE',  ( -4.458734124999999437, 11.60416666803225993, -2.574251347313719407 ) ) ;
#4708=CARTESIAN_POINT ( 'NONE',  ( -5.000000000000000000, -44.08333333333333570, -2.886751345948128211 ) ) ;
#4709=CARTESIAN_POINT ( 'NONE',  ( -4.999999999999998224, -68.91666666666667140, 2.886751345948131764 ) ) ;
#4710=CARTESIAN_POINT ( 'NONE',  ( 2.229367062500001939, -89.22916666530106511, 3.861377020970579999 ) ) ;
#4711=CARTESIAN_POINT ( 'NONE',  ( 9.457646018065525792E-16, 21.68750000136559208, 5.148502694627439702 ) ) ;
#4713=CARTESIAN_POINT ( 'NONE',  ( 1.060575238724906964E-15, 12.37500000273118417, 5.773502691896257311 ) ) ;
#4715=EDGE_LOOP ( 'NONE', ( #9155, #47606, #55221, #837 ) ) ;
#4717=CARTESIAN_POINT ( 'NONE',  ( -6.972266317189433020E-16, -82.24999999999998579, -5.000000000000000000 ) ) ;
#4718=CARTESIAN_POINT ( 'NONE',  ( 5.000000000000000000, -32.41666666666665719, -2.886751345948129988 ) ) ;
#4719=CARTESIAN_POINT ( 'NONE',  ( 4.458734125000001214, -37.89583333196772941, 2.574251347313718519 ) ) ;
#4720=CARTESIAN_POINT ( 'NONE',  ( 5.000000000000000000, -32.37499999726880873, -6.123233995736766282E-16 ) ) ;
#4721=CARTESIAN_POINT ( 'NONE',  ( 2.229367062499998831, -67.64583333196773651, -3.861377020970580887 ) ) ;
#4722=ORIENTED_EDGE ( 'NONE', *, *, #40871, .T. ) ;
#4724=CARTESIAN_POINT ( 'NONE',  ( 4.458734124999999437, -10.81249999863440792, -5.460374474430324690E-16 ) ) ;
#4725=EDGE_CURVE ( 'NONE', #3130, #12680, #47922, .T. ) ;
#4726=CARTESIAN_POINT ( 'NONE',  ( 4.458734124999999437, -14.06249999863440436, -5.460374474430324690E-16 ) ) ;
#4728=CARTESIAN_POINT ( 'NONE',  ( 1.060575238724906964E-15, -80.75000000000000000, 5.773502691896257311 ) ) ;
#4731=APPLICATION_CONTEXT ( 'automotive_design' ) ;
#4732=CARTESIAN_POINT ( 'NONE',  ( -5.000000000000000000, -80.95833333060214443, -2.886751345948128211 ) ) ;
#4735=CARTESIAN_POINT ( 'NONE',  ( -2.229367062499996610, -27.39583333196774007, 3.861377020970582219 ) ) ;
#4736=ORIENTED_EDGE ( 'NONE', *, *, #23349, .F. ) ;
#4738=CARTESIAN_POINT ( 'NONE',  ( 4.458734124999999437, -165.6875000013655779, 0.000000000000000000 ) ) ;
#4741=EDGE_LOOP ( 'NONE', ( #40553, #39140, #17407, #11318, #17810, #18038, #21123, #14304, #38965, #6332, #38364, #22396, #29462, #54225, #15827, #36407, #47450, #1288, #39597, #40912, #28006, #36483, #19441, #10313, #7657, #33022, #5219, #41022, #16609, #56847, #45706, #8481, #54766, #25915, #21213, #23735, #9959, #31393, #30071, #7284, #52065, #32630, #1584, #42554, #10046, #50286, #44747, #30436, #18795, #45138, #5370, #17571, #33589, #14298, #17359, #3076, #15012, #38277, #20556, #62956, #1128, #25257, #40097, #6743 ) ) ;
#4745=( BOUNDED_CURVE ( )  B_SPLINE_CURVE ( 2, ( #21784, #37206, #7938, #17892, #31407, #17262, #32370, #41376, #51684 ),
 .UNSPECIFIED., .F., .F. ) 
 B_SPLINE_CURVE_WITH_KNOTS ( ( 3, 2, 2, 2, 3 ),
 ( 0.8916666666666664964, 0.8958333333333331483, 0.8999999999999999112, 0.9041666666666665630, 0.9083333333333332149 ),
 .UNSPECIFIED. ) 
 CURVE ( )  GEOMETRIC_REPRESENTATION_ITEM ( )  RATIONAL_B_SPLINE_CURVE ( ( 1.000000000000003997, 0.9238795325112826307, 1.000000000000000000, 0.9238795325112867385, 1.000000000000000000, 0.9238795325112867385, 1.000000000000000000, 0.9238795325112887369, 0.9999999999999980016 ) ) 
 REPRESENTATION_ITEM ( '' )  );
#4750=CARTESIAN_POINT ( 'NONE',  ( 3.152801135295367541, -145.5625000013655779, -3.152801135295367541 ) ) ;
#4754=CARTESIAN_POINT ( 'NONE',  ( -2.229367062500000163, -68.72916666530107932, -3.861377020970580443 ) ) ;
#4755=CARTESIAN_POINT ( 'NONE',  ( -9.184850993605147944E-16, -154.2500000000000000, 5.000000000000000000 ) ) ;
#4756=CARTESIAN_POINT ( 'NONE',  ( 5.000000000000000000, -54.37499999726880162, -6.123233995736766282E-16 ) ) ;
#4758=ORIENTED_EDGE ( 'NONE', *, *, #48798, .T. ) ;
#4759=VECTOR ( 'NONE', #48137, 1000.000000000000000 ) ;
#4764=CARTESIAN_POINT ( 'NONE',  ( -1.127183054612291972E-14, 23.37500000273118772, 4.999999999999999112 ) ) ;
#4767=CARTESIAN_POINT ( 'NONE',  ( 9.457646018065525792E-16, 21.68750000136559208, 5.148502694627439702 ) ) ;
#4768=CARTESIAN_POINT ( 'NONE',  ( -4.999999999999998224, 27.08333333333333215, 2.886751345948131764 ) ) ;
#4775=CARTESIAN_POINT ( 'NONE',  ( 4.458734124999999437, 1.187500001365596081, -5.460374474430324690E-16 ) ) ;
#4777=CARTESIAN_POINT ( 'NONE',  ( 2.229367062499998831, -22.89583333196773651, -3.861377020970580887 ) ) ;
#4780=CARTESIAN_POINT ( 'NONE',  ( -2.229367062500000163, 26.52083333469892779, -3.861377020970580443 ) ) ;
#4781=ADVANCED_FACE ( 'NONE', ( #34298 ), #62655, .T. ) ;
#4785=CARTESIAN_POINT ( 'NONE',  ( 2.229367062499998831, -73.89583333196773651, -3.861377020970580887 ) ) ;
#4789=CARTESIAN_POINT ( 'NONE',  ( -4.999999999999998224, -10.79166666393547835, 2.886751345948131764 ) ) ;
#4793=CARTESIAN_POINT ( 'NONE',  ( -2.500000000000000444, -16.16666666666666785, -4.330127018922193649 ) ) ;
#4794=CARTESIAN_POINT ( 'NONE',  ( 2.229367062500001939, -21.97916666530107221, 3.861377020970579999 ) ) ;
#4796=CARTESIAN_POINT ( 'NONE',  ( -4.458734124999999437, -82.39583333196773651, -2.574251347313719407 ) ) ;
#4797=EDGE_CURVE ( 'NONE', #26724, #14472, #25387, .T. ) ;
#4798=CARTESIAN_POINT ( 'NONE',  ( 3.152801135295367541, -167.5625000013656063, -3.152801135295367541 ) ) ;
#4799=CARTESIAN_POINT ( 'NONE',  ( -4.999999999999999112, -16.79166666393548368, 2.886751345948131764 ) ) ;
#4800=CARTESIAN_POINT ( 'NONE',  ( 2.229367062499998831, -49.64583333196772941, -3.861377020970580887 ) ) ;
#4803=CARTESIAN_POINT ( 'NONE',  ( -4.999999999999998224, -27.79166666393548013, 2.886751345948131764 ) ) ;
#4804=CARTESIAN_POINT ( 'NONE',  ( 4.458734124999999437, -0.06249999863440491854, -5.460374474430324690E-16 ) ) ;
#4807=CARTESIAN_POINT ( 'NONE',  ( -2.499999999999996447, -60.83333333333333570, 4.330127018922195425 ) ) ;
#4809=CARTESIAN_POINT ( 'NONE',  ( -4.458734125000000326, -155.2500000013656063, -1.846868145590735644 ) ) ;
#4812=CARTESIAN_POINT ( 'NONE',  ( 5.000000000000000000, -161.0000000000000000, 0.000000000000000000 ) ) ;
#4817=CARTESIAN_POINT ( 'NONE',  ( 2.229367062500001939, -5.229166665301071326, 3.861377020970579999 ) ) ;
#4818=CARTESIAN_POINT ( 'NONE',  ( -3.152548672688508926E-16, -48.81249999863440792, -5.148502694627439702 ) ) ;
#4821=CARTESIAN_POINT ( 'NONE',  ( -4.458734125000000326, -147.0000000013655779, -1.846868145590735644 ) ) ;
#4824=EDGE_LOOP ( 'NONE', ( #234, #18241, #24008, #34143 ) ) ;
#4825=CARTESIAN_POINT ( 'NONE',  ( -2.500000000000000444, -69.04166666393547303, -4.330127018922193649 ) ) ;
#4827=DIRECTION ( 'NONE',  ( -0.000000000000000000, 1.000000000000000000, -0.000000000000000000 ) ) ;
#4828=ORIENTED_EDGE ( 'NONE', *, *, #39442, .T. ) ;
#4829=( BOUNDED_CURVE ( )  B_SPLINE_CURVE ( 2, ( #15131, #20280, #59203, #33488, #38931, #53107, #9982, #33799, #48585 ),
 .UNSPECIFIED., .F., .F. ) 
 B_SPLINE_CURVE_WITH_KNOTS ( ( 3, 2, 2, 2, 3 ),
 ( 0.3562500000000000111, 0.3569444444444444531, 0.3583333333333333370, 0.3597222222222222210, 0.3604166666666666630 ),
 .UNSPECIFIED. ) 
 CURVE ( )  GEOMETRIC_REPRESENTATION_ITEM ( )  RATIONAL_B_SPLINE_CURVE ( ( 0.9330127018922194093, 0.9330127018922194093, 1.000000000000000000, 0.8660254037844387076, 1.000000000000000000, 0.8660254037844387076, 1.000000000000000000, 0.9330127018922194093, 0.9330127018922194093 ) ) 
 REPRESENTATION_ITEM ( '' )  );
#4834=CARTESIAN_POINT ( 'NONE',  ( 9.457646018065525792E-16, -4.062499998634408804, 5.148502694627439702 ) ) ;
#4836=CARTESIAN_POINT ( 'NONE',  ( -3.152801135295367985, -153.8125000013656063, 3.152801135295367096 ) ) ;
#4838=EDGE_LOOP ( 'NONE', ( #46377, #17472, #45316, #21399 ) ) ;
#4841=DIRECTION ( 'NONE',  ( -0.000000000000000000, 1.000000000000000000, -0.000000000000000000 ) ) ;
#4844=CARTESIAN_POINT ( 'NONE',  ( 5.000000000000000888, 8.541666669397853795, 2.886751345948126879 ) ) ;
#4845=( BOUNDED_CURVE ( )  B_SPLINE_CURVE ( 2, ( #53265, #24302, #38166, #62926, #38770, #29115, #53889, #63556, #13402 ),
 .UNSPECIFIED., .F., .F. ) 
 B_SPLINE_CURVE_WITH_KNOTS ( ( 3, 2, 2, 2, 3 ),
 ( 0.9229166666666667185, 0.9236111111111111605, 0.9250000000000000444, 0.9263888888888889284, 0.9270833333333333703 ),
 .UNSPECIFIED. ) 
 CURVE ( )  GEOMETRIC_REPRESENTATION_ITEM ( )  RATIONAL_B_SPLINE_CURVE ( ( 0.9330127018922194093, 0.9330127018922194093, 1.000000000000000000, 0.8660254037844387076, 1.000000000000000000, 0.8660254037844387076, 1.000000000000000000, 0.9330127018922194093, 0.9330127018922194093 ) ) 
 REPRESENTATION_ITEM ( '' )  );
#4848=CARTESIAN_POINT ( 'NONE',  ( 1.339745962155612702, -64.16965819600731891, -5.000000000000000000 ) ) ;
#4850=CARTESIAN_POINT ( 'NONE',  ( 2.499999999999998668, -44.33333333333333570, -4.330127018922193649 ) ) ;
#4852=CARTESIAN_POINT ( 'NONE',  ( 9.457646018065525792E-16, 18.93750000136559564, 5.148502694627439702 ) ) ;
#4854=CARTESIAN_POINT ( 'NONE',  ( 4.458734124999998549, -8.979166665301075767, -2.574251347313721627 ) ) ;
#4855=VECTOR ( 'NONE', #17110, 1000.000000000000000 ) ;
#4858=CARTESIAN_POINT ( 'NONE',  ( 2.730187237215162345E-16, -167.1875000013655779, -4.458734124999999437 ) ) ;
#4865=CARTESIAN_POINT ( 'NONE',  ( -5.000000000000000000, -54.87499999726880162, 0.000000000000000000 ) ) ;
#4867=VECTOR ( 'NONE', #28108, 1000.000000000000000 ) ;
#4868=CARTESIAN_POINT ( 'NONE',  ( 3.152801135295366208, -154.8125000013656063, 3.152801135295367985 ) ) ;
#4870=CARTESIAN_POINT ( 'NONE',  ( 2.499999999999998668, -46.33333333333333570, -4.330127018922193649 ) ) ;
#4871=DIRECTION ( 'NONE',  ( -0.000000000000000000, 1.000000000000000000, -0.000000000000000000 ) ) ;
#4875=CARTESIAN_POINT ( 'NONE',  ( 1.975475456537005874E-15, -87.62499999726880162, 5.000000000000000000 ) ) ;
#4876=CARTESIAN_POINT ( 'NONE',  ( 2.499999999999998668, -4.333333333333334814, -4.330127018922193649 ) ) ;
#4877=CARTESIAN_POINT ( 'NONE',  ( -4.458734124999997661, -65.22916666530106511, 2.574251347313722516 ) ) ;
#4878=CARTESIAN_POINT ( 'NONE',  ( -4.999999999999998224, -30.79166666393548013, 2.886751345948131764 ) ) ;
#4879=CARTESIAN_POINT ( 'NONE',  ( 2.499999999999998668, -0.2083333306021478704, -4.330127018922193649 ) ) ;
#4880=CARTESIAN_POINT ( 'NONE',  ( -4.458734124999999437, -36.39583333196772941, -2.574251347313719407 ) ) ;
#4884=CARTESIAN_POINT ( 'NONE',  ( 2.499999999999998668, 5.666666666666666963, -4.330127018922193649 ) ) ;
#4885=CARTESIAN_POINT ( 'NONE',  ( -4.999999999999999112, -44.91666666666666430, 2.886751345948131764 ) ) ;
#4889=CARTESIAN_POINT ( 'NONE',  ( 2.229367062500001939, -69.97916666530107932, 3.861377020970579999 ) ) ;
#4890=CARTESIAN_POINT ( 'NONE',  ( 1.846868145590736310, -144.8750000013655779, 4.458734124999999437 ) ) ;
#4891=CARTESIAN_POINT ( 'NONE',  ( -3.152548672688508926E-16, -84.56249999863439371, -5.148502694627439702 ) ) ;
#4893=CARTESIAN_POINT ( 'NONE',  ( -4.458734124999999437, -32.64583333196774362, -2.574251347313719407 ) ) ;
#4894=CARTESIAN_POINT ( 'NONE',  ( 2.499999999999998668, -73.20833333060214443, -4.330127018922193649 ) ) ;
#4897=CARTESIAN_POINT ( 'NONE',  ( 1.975475456537005874E-15, -51.75000000000000000, 5.000000000000000000 ) ) ;
#4901=( LENGTH_UNIT ( ) NAMED_UNIT ( * ) SI_UNIT ( .MILLI., .METRE. ) );
#4902=VERTEX_POINT ( 'NONE', #50377 ) ;
#4906=CARTESIAN_POINT ( 'NONE',  ( -5.000000000000000000, -3.083333333333333925, -2.886751345948128211 ) ) ;
#4907=CARTESIAN_POINT ( 'NONE',  ( -4.458734124999998549, -60.47916666530105800, 2.574251347313722516 ) ) ;
#4912=CARTESIAN_POINT ( 'NONE',  ( 9.457646018065525792E-16, 13.93750000136559564, 5.148502694627439702 ) ) ;
#4914=CARTESIAN_POINT ( 'NONE',  ( 2.500000000000002220, -24.66666666666666430, 4.330127018922192761 ) ) ;
#4915=CARTESIAN_POINT ( 'NONE',  ( 4.458734124999999437, -164.3750000013656063, -1.846868145590734978 ) ) ;
#4916=VECTOR ( 'NONE', #24128, 1000.000000000000000 ) ;
#4919=CARTESIAN_POINT ( 'NONE',  ( -5.000000000000000888, -153.4375000000000000, 2.071067811865474617 ) ) ;
#4927=CARTESIAN_POINT ( 'NONE',  ( 2.500000000000002220, -61.66666666666666430, 4.330127018922192761 ) ) ;
#4931=CARTESIAN_POINT ( 'NONE',  ( 2.229367062500001939, 8.770833334698927786, 3.861377020970579999 ) ) ;
#4934=CARTESIAN_POINT ( 'NONE',  ( 2.071067811865476394, -151.3125000027311842, 5.000000000000000000 ) ) ;
#4938=CARTESIAN_POINT ( 'NONE',  ( -2.071067811865475061, -141.6875000000000000, -5.000000000000000888 ) ) ;
#4940=CARTESIAN_POINT ( 'NONE',  ( -3.152801135295367985, -167.0625000013656063, 3.152801135295367096 ) ) ;
#4941=CARTESIAN_POINT ( 'NONE',  ( 4.458734125000000326, -30.89583333196773651, 2.574251347313718519 ) ) ;
#4942=CYLINDRICAL_SURFACE ( 'NONE', #62573, 5.000000000000000000 ) ;
#4943=DIRECTION ( 'NONE',  ( -0.000000000000000000, 1.000000000000000000, -0.000000000000000000 ) ) ;
#4945=CARTESIAN_POINT ( 'NONE',  ( -3.152801135295367985, -143.8125000013655779, 3.152801135295367096 ) ) ;
#4947=CARTESIAN_POINT ( 'NONE',  ( 9.457646018065525792E-16, 25.68750000136559208, 5.148502694627439702 ) ) ;
#4948=VERTEX_POINT ( 'NONE', #45229 ) ;
#4949=CARTESIAN_POINT ( 'NONE',  ( 4.458734124999999437, -60.06249999863440081, -5.460374474430324690E-16 ) ) ;
#4951=( BOUNDED_CURVE ( )  B_SPLINE_CURVE ( 2, ( #23525, #15127, #31, #24781, #58867, #5161, #34748, #14169, #3906 ),
 .UNSPECIFIED., .F., .F. ) 
 B_SPLINE_CURVE_WITH_KNOTS ( ( 3, 2, 2, 2, 3 ),
 ( 0.8729166666666666741, 0.8736111111111111160, 0.8750000000000000000, 0.8763888888888888840, 0.8770833333333333259 ),
 .UNSPECIFIED. ) 
 CURVE ( )  GEOMETRIC_REPRESENTATION_ITEM ( )  RATIONAL_B_SPLINE_CURVE ( ( 0.9330127018922194093, 0.9330127018922194093, 1.000000000000000000, 0.8660254037844387076, 1.000000000000000000, 0.8660254037844387076, 1.000000000000000000, 0.9330127018922194093, 0.9330127018922194093 ) ) 
 REPRESENTATION_ITEM ( '' )  );
#4952=CARTESIAN_POINT ( 'NONE',  ( 5.000000000000000000, -90.29166666393547303, -2.886751345948130876 ) ) ;
#4953=CARTESIAN_POINT ( 'NONE',  ( 2.500000000000002220, 19.33333333333333570, 4.330127018922192761 ) ) ;
#4955=CYLINDRICAL_SURFACE ( 'NONE', #56267, 5.000000000000000000 ) ;
#4956=CARTESIAN_POINT ( 'NONE',  ( 2.229367062499998831, -3.645833331967739177, -3.861377020970580887 ) ) ;
#4957=CYLINDRICAL_SURFACE ( 'NONE', #7226, 5.000000000000000000 ) ;
#4958=CYLINDRICAL_SURFACE ( 'NONE', #33783, 5.000000000000000000 ) ;
#4960=DIRECTION ( 'NONE',  ( -0.000000000000000000, 1.000000000000000000, -0.000000000000000000 ) ) ;
#4961=CARTESIAN_POINT ( 'NONE',  ( 2.500000000000002220, 0.3333333333333348136, 4.330127018922192761 ) ) ;
#4964=CARTESIAN_POINT ( 'NONE',  ( 4.458734124999999437, -53.81249999863439371, -5.460374474430324690E-16 ) ) ;
#4965=CARTESIAN_POINT ( 'NONE',  ( -3.152801135295367096, -157.3125000013656063, -3.152801135295367541 ) ) ;
#4966=CARTESIAN_POINT ( 'NONE',  ( -5.000000000000000000, -50.95833333060213732, -2.886751345948128211 ) ) ;
#4967=ORIENTED_EDGE ( 'NONE', *, *, #23606, .F. ) ;
#4968=CARTESIAN_POINT ( 'NONE',  ( 2.229367062500001939, 6.770833334698928674, 3.861377020970579999 ) ) ;
#4972=CARTESIAN_POINT ( 'NONE',  ( 1.846868145590736310, -157.6250000013655779, 4.458734124999999437 ) ) ;
#4976=CARTESIAN_POINT ( 'NONE',  ( 5.000000000000000888, -47.45833333060215153, 2.886751345948126879 ) ) ;
#4977=CARTESIAN_POINT ( 'NONE',  ( -3.152548672688508926E-16, -41.81249999863440081, -5.148502694627439702 ) ) ;
#4979=CARTESIAN_POINT ( 'NONE',  ( -5.000000000000000000, -46.08333333333333570, -2.886751345948128211 ) ) ;
#4981=CARTESIAN_POINT ( 'NONE',  ( -3.535533905932738641, -156.5000000027312126, 3.535533905932737309 ) ) ;
#4982=ORIENTED_EDGE ( 'NONE', *, *, #60733, .T. ) ;
#4983=CARTESIAN_POINT ( 'NONE',  ( 4.458734124999998549, -89.97916666530105090, -2.574251347313721627 ) ) ;
#4987=VECTOR ( 'NONE', #27748, 1000.000000000000000 ) ;
#4990=CARTESIAN_POINT ( 'NONE',  ( -5.000000000000000000, 10.12500000273118594, 0.000000000000000000 ) ) ;
#4992=EDGE_CURVE ( 'NONE', #46250, #43716, #54886, .T. ) ;
#4993=VECTOR ( 'NONE', #2241, 1000.000000000000000 ) ;
#5003=ORIENTED_EDGE ( 'NONE', *, *, #14955, .T. ) ;
#5006=CARTESIAN_POINT ( 'NONE',  ( -5.000000000000000888, -159.6875000027312126, -2.071067811865475949 ) ) ;
#5008=CARTESIAN_POINT ( 'NONE',  ( 5.000000000000000000, -163.1250000027311842, 0.000000000000000000 ) ) ;
#5018=CARTESIAN_POINT ( 'NONE',  ( -2.229367062499996610, -13.14583333196774007, 3.861377020970582219 ) ) ;
#5020=CARTESIAN_POINT ( 'NONE',  ( 2.071067811865475505, -154.8125000000000000, -5.000000000000000888 ) ) ;
#5022=VERTEX_POINT ( 'NONE', #11450 ) ;
#5023=CARTESIAN_POINT ( 'NONE',  ( -4.458734124999999437, -38.64583333196773651, -2.574251347313719407 ) ) ;
#5030=CARTESIAN_POINT ( 'NONE',  ( -4.458734124999998549, 10.77083333469892956, 2.574251347313722516 ) ) ;
#5031=CARTESIAN_POINT ( 'NONE',  ( 1.975475456537005874E-15, -48.62499999726880162, 5.000000000000000000 ) ) ;
#5032=CARTESIAN_POINT ( 'NONE',  ( -2.071067811865507036, -165.8125000027312126, -4.999999999999968914 ) ) ;
#5033=CARTESIAN_POINT ( 'NONE',  ( 2.229367062499998831, -89.89583333196773651, -3.861377020970580887 ) ) ;
#5034=CARTESIAN_POINT ( 'NONE',  ( -4.458734124999998549, 21.52083333469893134, 2.574251347313722516 ) ) ;
#5036=CARTESIAN_POINT ( 'NONE',  ( -5.000000000000000000, 8.125000002731187720, 0.000000000000000000 ) ) ;
#5037=VERTEX_POINT ( 'NONE', #30104 ) ;
#5040=ORIENTED_EDGE ( 'NONE', *, *, #13898, .F. ) ;
#5041=CARTESIAN_POINT ( 'NONE',  ( 3.061616997868383141E-16, -160.8750000027311842, -5.000000000000000000 ) ) ;
#5042=CARTESIAN_POINT ( 'NONE',  ( 5.000000000000000000, -36.50000000000000711, -6.123233995736766282E-16 ) ) ;
#5043=CARTESIAN_POINT ( 'NONE',  ( -4.458734124999998549, -39.22916666530107221, 2.574251347313722516 ) ) ;
#5044=CARTESIAN_POINT ( 'NONE',  ( -5.000000000000000000, -33.95833333060213732, -2.886751345948128211 ) ) ;
#5045=CARTESIAN_POINT ( 'NONE',  ( 2.229367062500001939, -65.97916666530106511, 3.861377020970579999 ) ) ;
#5048=CARTESIAN_POINT ( 'NONE',  ( -2.229367062499996610, -11.14583333196773829, 3.861377020970582219 ) ) ;
#5049=CARTESIAN_POINT ( 'NONE',  ( -3.152548672688508926E-16, -14.81249999863440436, -5.148502694627439702 ) ) ;
#5051=CARTESIAN_POINT ( 'NONE',  ( -2.499999999999996447, -81.83333333333332860, 4.330127018922195425 ) ) ;
#5052=CARTESIAN_POINT ( 'NONE',  ( -8.190561711645485556E-16, -167.6875000013655779, 4.458734124999999437 ) ) ;
#5054=CARTESIAN_POINT ( 'NONE',  ( -2.500000000000000444, -83.04166666393547303, -4.330127018922193649 ) ) ;
#5055=CARTESIAN_POINT ( 'NONE',  ( 0.000000000000000000, -170.0000000000000000, 0.000000000000000000 ) ) ;
#5056=ORIENTED_EDGE ( 'NONE', *, *, #8243, .T. ) ;
#5058=CARTESIAN_POINT ( 'NONE',  ( -2.229367062499996610, -25.39583333196773651, 3.861377020970582219 ) ) ;
#5059=ORIENTED_EDGE ( 'NONE', *, *, #55068, .F. ) ;
#5060=CARTESIAN_POINT ( 'NONE',  ( 1.846868145590735200, -167.5000000013655779, -4.458734125000000326 ) ) ;
#5062=CARTESIAN_POINT ( 'NONE',  ( 5.000000000000000000, -55.29166666393548013, -2.886751345948130876 ) ) ;
#5063=ORIENTED_EDGE ( 'NONE', *, *, #11108, .T. ) ;
#5067=CARTESIAN_POINT ( 'NONE',  ( -4.458734124999999437, -145.2500000013656347, -1.846868145590735644 ) ) ;
#5073=ORIENTED_EDGE ( 'NONE', *, *, #45977, .T. ) ;
#5074=CARTESIAN_POINT ( 'NONE',  ( 4.458734124999999437, -141.6875000013656063, 0.000000000000000000 ) ) ;
#5080=CARTESIAN_POINT ( 'NONE',  ( -4.458734124999999437, -74.56249999863440792, 0.000000000000000000 ) ) ;
#5081=CARTESIAN_POINT ( 'NONE',  ( 1.339745962155615144, -54.58034179853029144, 4.999999999999999112 ) ) ;
#5082=CARTESIAN_POINT ( 'NONE',  ( 5.000000000000000000, 14.70833333606451809, -2.886751345948130876 ) ) ;
#5085=EDGE_LOOP ( 'NONE', ( #50063, #46655, #12453, #6831 ) ) ;
#5086=CARTESIAN_POINT ( 'NONE',  ( -5.000000000000000000, -70.95833333060214443, -2.886751345948128211 ) ) ;
#5090=EDGE_CURVE ( 'NONE', #34156, #11358, #12615, .T. ) ;
#5093=AXIS2_PLACEMENT_3D ( 'NONE', #29055, #58348, #19091 ) ;
#5094=CARTESIAN_POINT ( 'NONE',  ( -2.229367062499996610, 20.60416666803225993, 3.861377020970582219 ) ) ;
#5102=CARTESIAN_POINT ( 'NONE',  ( -3.152548672688508926E-16, 0.4375000013655955255, -5.148502694627439702 ) ) ;
#5104=CARTESIAN_POINT ( 'NONE',  ( -4.458734124999999437, -24.64583333196773651, -2.574251347313719407 ) ) ;
#5107=CARTESIAN_POINT ( 'NONE',  ( 2.229367062500001939, 24.02083333469892779, 3.861377020970579999 ) ) ;
#5110=CARTESIAN_POINT ( 'NONE',  ( 4.458734124999999437, -71.06249999863439371, -5.460374474430324690E-16 ) ) ;
#5113=CARTESIAN_POINT ( 'NONE',  ( -5.000000000000000000, -10.87499999726881583, 0.000000000000000000 ) ) ;
#5116=CARTESIAN_POINT ( 'NONE',  ( -1.339745962155610925, -56.66965819600733312, 5.000000000000000000 ) ) ;
#5117=CARTESIAN_POINT ( 'NONE',  ( -2.499999999999996447, -17.83333333333333215, 4.330127018922195425 ) ) ;
#5118=CARTESIAN_POINT ( 'NONE',  ( 2.229367062499998831, -23.64583333196773651, -3.861377020970580887 ) ) ;
#5119=EDGE_CURVE ( 'NONE', #32095, #51645, #58259, .T. ) ;
#5120=CARTESIAN_POINT ( 'NONE',  ( -4.458734124999999437, -81.31249999863440792, 0.000000000000000000 ) ) ;
#5121=CARTESIAN_POINT ( 'NONE',  ( -5.000000000000000000, -19.87499999726880873, 0.000000000000000000 ) ) ;
#5122=CARTESIAN_POINT ( 'NONE',  ( 4.458734124999998549, -47.72916666530106511, -2.574251347313721627 ) ) ;
#5123=ORIENTED_EDGE ( 'NONE', *, *, #19159, .F. ) ;
#5125=CARTESIAN_POINT ( 'NONE',  ( 1.339745962155615144, -15.58034179853029499, 4.999999999999999112 ) ) ;
#5126=CARTESIAN_POINT ( 'NONE',  ( -4.458734124999999437, 1.354166668032261933, -2.574251347313719407 ) ) ;
#5129=CARTESIAN_POINT ( 'NONE',  ( -2.499999999999996447, -67.83333333333332860, 4.330127018922195425 ) ) ;
#5130=CARTESIAN_POINT ( 'NONE',  ( 4.458734125000000326, -156.6250000013655779, -1.846868145590734978 ) ) ;
#5134=CARTESIAN_POINT ( 'NONE',  ( 5.000000000000000000, -163.0000000000000000, 0.000000000000000000 ) ) ;
#5136=VECTOR ( 'NONE', #40247, 1000.000000000000000 ) ;
#5138=CARTESIAN_POINT ( 'NONE',  ( 4.458734124999998549, -11.97916666530107044, -2.574251347313721627 ) ) ;
#5139=CARTESIAN_POINT ( 'NONE',  ( 2.229367062500001939, -45.22916666530106511, 3.861377020970579999 ) ) ;
#5140=CARTESIAN_POINT ( 'NONE',  ( 2.071067811865602959, -150.9375000027312126, -4.999999999999874767 ) ) ;
#5141=CARTESIAN_POINT ( 'NONE',  ( 4.458734124999999437, -150.4375000013656063, 0.000000000000000000 ) ) ;
#5144=ORIENTED_EDGE ( 'NONE', *, *, #11330, .T. ) ;
#5150=ADVANCED_FACE ( 'NONE', ( #55845 ), #11761, .T. ) ;
#5154=CARTESIAN_POINT ( 'NONE',  ( -2.499999999999996447, 2.291666669397850686, 4.330127018922195425 ) ) ;
#5155=CARTESIAN_POINT ( 'NONE',  ( -3.152548672688508926E-16, -3.562499998634408360, -5.148502694627439702 ) ) ;
#5157=CARTESIAN_POINT ( 'NONE',  ( -3.152801135295367096, -151.0625000013655779, -3.152801135295367541 ) ) ;
#5161=CARTESIAN_POINT ( 'NONE',  ( -5.000000000000000000, -75.08333333333332860, -2.886751345948128211 ) ) ;
#5162=CARTESIAN_POINT ( 'NONE',  ( 1.975475456537005874E-15, -12.62499999726881050, 5.000000000000000000 ) ) ;
#5165=EDGE_CURVE ( 'NONE', #10357, #48933, #56594, .T. ) ;
#5166=CARTESIAN_POINT ( 'NONE',  ( 0.000000000000000000, -170.0000000000000000, 0.000000000000000000 ) ) ;
#5169=DIRECTION ( 'NONE',  ( -0.000000000000000000, 1.000000000000000000, -0.000000000000000000 ) ) ;
#5173=CARTESIAN_POINT ( 'NONE',  ( 5.000000000000000000, 9.583333333333332149, -2.886751345948130876 ) ) ;
#5174=CARTESIAN_POINT ( 'NONE',  ( 2.229367062499998831, 17.35416666803225993, -3.861377020970580887 ) ) ;
#5177=VECTOR ( 'NONE', #6927, 1000.000000000000000 ) ;
#5178=CARTESIAN_POINT ( 'NONE',  ( -2.229367062499996610, -6.395833331967741842, 3.861377020970582219 ) ) ;
#5180=CARTESIAN_POINT ( 'NONE',  ( -4.458734125000000326, -167.0000000013655779, -1.846868145590735644 ) ) ;
#5187=CARTESIAN_POINT ( 'NONE',  ( 5.000000000000000000, -38.49999999999999289, -6.123233995736766282E-16 ) ) ;
#5189=CARTESIAN_POINT ( 'NONE',  ( 2.499999999999998668, -69.33333333333332860, -4.330127018922193649 ) ) ;
#5190=CARTESIAN_POINT ( 'NONE',  ( -4.458734125000000326, -154.1250000013655779, 1.846868145590734089 ) ) ;
#5196=CARTESIAN_POINT ( 'NONE',  ( 0.000000000000000000, -170.0000000000000000, 0.000000000000000000 ) ) ;
#5197=CARTESIAN_POINT ( 'NONE',  ( 2.500000000000002220, -1.666666666666663410, 4.330127018922192761 ) ) ;
#5198=CARTESIAN_POINT ( 'NONE',  ( 4.458734124999999437, -68.81249999863439371, -5.460374474430324690E-16 ) ) ;
#5199=CARTESIAN_POINT ( 'NONE',  ( -6.972266317189433020E-16, 19.75000000000000000, -5.000000000000000000 ) ) ;
#5200=CARTESIAN_POINT ( 'NONE',  ( 1.060575238724906964E-15, -0.6249999972688138339, 5.773502691896257311 ) ) ;
#5201=CARTESIAN_POINT ( 'NONE',  ( 2.229367062499998831, -34.64583333196772941, -3.861377020970580887 ) ) ;
#5203=CYLINDRICAL_SURFACE ( 'NONE', #18360, 5.000000000000000000 ) ;
#5206=CARTESIAN_POINT ( 'NONE',  ( 5.000000000000000888, -51.58333333333332149, 2.886751345948126879 ) ) ;
#5210=CARTESIAN_POINT ( 'NONE',  ( -4.458734124999999437, -72.39583333196775072, -2.574251347313719407 ) ) ;
#5211=CARTESIAN_POINT ( 'NONE',  ( 4.458734124999999437, -142.7500000013656063, 1.846868145590737864 ) ) ;
#5212=CARTESIAN_POINT ( 'NONE',  ( 9.457646018065525792E-16, -83.06249999863439371, 5.148502694627439702 ) ) ;
#5215=CARTESIAN_POINT ( 'NONE',  ( -2.229367062499996610, -29.39583333196774007, 3.861377020970582219 ) ) ;
#5216=CARTESIAN_POINT ( 'NONE',  ( -4.999999999999999112, -73.79166666393547303, 2.886751345948131764 ) ) ;
#5217=ORIENTED_EDGE ( 'NONE', *, *, #31984, .F. ) ;
#5219=ORIENTED_EDGE ( 'NONE', *, *, #16937, .F. ) ;
#5226=CARTESIAN_POINT ( 'NONE',  ( -3.152548672688508926E-16, -58.81249999863440081, -5.148502694627439702 ) ) ;
#5228=ORIENTED_EDGE ( 'NONE', *, *, #42909, .F. ) ;
#5231=DIRECTION ( 'NONE',  ( -0.000000000000000000, 1.000000000000000000, -0.000000000000000000 ) ) ;
#5232=CYLINDRICAL_SURFACE ( 'NONE', #55149, 5.000000000000000000 ) ;
#5233=CARTESIAN_POINT ( 'NONE',  ( 4.458734124999999437, 12.18750000136559564, -5.460374474430324690E-16 ) ) ;
#5235=CARTESIAN_POINT ( 'NONE',  ( 5.000000000000000000, -24.50000000000000000, -6.123233995736766282E-16 ) ) ;
#5236=CARTESIAN_POINT ( 'NONE',  ( -1.846868145590734756, -166.1250000013656063, -4.458734124999999437 ) ) ;
#5239=CARTESIAN_POINT ( 'NONE',  ( -3.535533905932737309, -153.6250000000000000, -3.535533905932738197 ) ) ;
#5244=CARTESIAN_POINT ( 'NONE',  ( -2.500000000000000444, -29.16666666666666785, -4.330127018922193649 ) ) ;
#5250=EDGE_CURVE ( 'NONE', #39875, #21118, #5667, .T. ) ;
#5252=CARTESIAN_POINT ( 'NONE',  ( 4.458734124999998549, 5.020833334698926897, -2.574251347313721627 ) ) ;
#5253=CARTESIAN_POINT ( 'NONE',  ( -9.184850993605147944E-16, -151.2500000000000284, 5.000000000000000000 ) ) ;
#5256=CARTESIAN_POINT ( 'NONE',  ( 3.535533905932738197, -149.0000000027311842, -3.535533905932738197 ) ) ;
#5261=CARTESIAN_POINT ( 'NONE',  ( 0.000000000000000000, -170.0000000000000000, 0.000000000000000000 ) ) ;
#5265=CARTESIAN_POINT ( 'NONE',  ( -3.152801135295367096, -164.3125000013656063, -3.152801135295367541 ) ) ;
#5266=CARTESIAN_POINT ( 'NONE',  ( 4.458734125000000326, -36.89583333196773651, 2.574251347313718519 ) ) ;
#5267=DIRECTION ( 'NONE',  ( 0.000000000000000000, 0.000000000000000000, 1.000000000000000000 ) ) ;
#5269=CARTESIAN_POINT ( 'NONE',  ( 4.458734125000000326, -142.3750000013656063, -1.846868145590734978 ) ) ;
#5270=VERTEX_POINT ( 'NONE', #3403 ) ;
#5271=CARTESIAN_POINT ( 'NONE',  ( 4.458734124999998549, 28.02083333469892779, -2.574251347313721627 ) ) ;
#5272=ORIENTED_EDGE ( 'NONE', *, *, #34846, .F. ) ;
#5273=CARTESIAN_POINT ( 'NONE',  ( -2.229367062499996610, -61.39583333196774362, 3.861377020970582219 ) ) ;
#5276=CARTESIAN_POINT ( 'NONE',  ( -2.500000000000000444, 15.83333333333333037, -4.330127018922193649 ) ) ;
#5278=CARTESIAN_POINT ( 'NONE',  ( -4.458734124999999437, -52.31249999863440792, 0.000000000000000000 ) ) ;
#5279=CARTESIAN_POINT ( 'NONE',  ( -2.229367062499996610, -7.145833331967735624, 3.861377020970582219 ) ) ;
#5281=CARTESIAN_POINT ( 'NONE',  ( -2.500000000000000444, -9.166666666666662522, -4.330127018922193649 ) ) ;
#5282=DIRECTION ( 'NONE',  ( -0.000000000000000000, 1.000000000000000000, -0.000000000000000000 ) ) ;
#5283=CARTESIAN_POINT ( 'NONE',  ( -4.999999999999998224, -9.916666666666662522, 2.886751345948131764 ) ) ;
#5286=( BOUNDED_CURVE ( )  B_SPLINE_CURVE ( 2, ( #30713, #59675, #45186, #54845, #40675, #36493, #20435, #15922, #1152 ),
 .UNSPECIFIED., .F., .F. ) 
 B_SPLINE_CURVE_WITH_KNOTS ( ( 3, 2, 2, 2, 3 ),
 ( 0.4729166666666666519, 0.4736111111111110938, 0.4749999999999999778, 0.4763888888888888618, 0.4770833333333333592 ),
 .UNSPECIFIED. ) 
 CURVE ( )  GEOMETRIC_REPRESENTATION_ITEM ( )  RATIONAL_B_SPLINE_CURVE ( ( 0.9330127018922194093, 0.9330127018922194093, 1.000000000000000000, 0.8660254037844387076, 1.000000000000000000, 0.8660254037844387076, 1.000000000000000000, 0.9330127018922167448, 0.9330127018922194093 ) ) 
 REPRESENTATION_ITEM ( '' )  );
#5289=CARTESIAN_POINT ( 'NONE',  ( -4.458734124999999437, -54.39583333196773651, -2.574251347313719407 ) ) ;
#5290=CARTESIAN_POINT ( 'NONE',  ( -8.190561711645485556E-16, -154.9375000013655779, 4.458734124999999437 ) ) ;
#5291=CARTESIAN_POINT ( 'NONE',  ( -5.000000000000000000, -54.95833333060213732, -2.886751345948128211 ) ) ;
#5292=VERTEX_POINT ( 'NONE', #23019 ) ;
#5293=CARTESIAN_POINT ( 'NONE',  ( 1.975475456537005874E-15, -48.74999999999999289, 5.000000000000000000 ) ) ;
#5294=CARTESIAN_POINT ( 'NONE',  ( 9.457646018065525792E-16, 3.687500001365594748, 5.148502694627439702 ) ) ;
#5296=CARTESIAN_POINT ( 'NONE',  ( 2.499999999999998668, -56.33333333333333570, -4.330127018922193649 ) ) ;
#5298=CARTESIAN_POINT ( 'NONE',  ( 3.152801135295367541, -156.3125000013656063, -3.152801135295367541 ) ) ;
#5299=EDGE_LOOP ( 'NONE', ( #56424, #10490, #36132, #61597 ) ) ;
#5303=CARTESIAN_POINT ( 'NONE',  ( -4.458734124999999437, -41.64583333196773651, -2.574251347313719407 ) ) ;
#5304=VERTEX_POINT ( 'NONE', #42622 ) ;
#5305=DIRECTION ( 'NONE',  ( 0.000000000000000000, 0.000000000000000000, 1.000000000000000000 ) ) ;
#5307=CARTESIAN_POINT ( 'NONE',  ( 6.123233995736766282E-16, -170.0000000000000000, -5.000000000000000000 ) ) ;
#5309=CARTESIAN_POINT ( 'NONE',  ( 4.458734125000001214, 29.10416666803225993, 2.574251347313718519 ) ) ;
#5312=DIRECTION ( 'NONE',  ( -0.000000000000000000, 1.000000000000000000, -0.000000000000000000 ) ) ;
#5314=CARTESIAN_POINT ( 'NONE',  ( 5.000000000000000000, -169.0000000000000000, 0.000000000000000000 ) ) ;
#5318=CARTESIAN_POINT ( 'NONE',  ( 1.339745962155612702, -33.29465819873851729, -5.000000000000000000 ) ) ;
#5321=CARTESIAN_POINT ( 'NONE',  ( -5.000000000000000000, 5.000000000000000888, 0.000000000000000000 ) ) ;
#5322=CARTESIAN_POINT ( 'NONE',  ( -6.972266317189433020E-16, -67.12499999726881583, -5.000000000000000000 ) ) ;
#5323=CARTESIAN_POINT ( 'NONE',  ( -2.229367062500000163, -89.72916666530106511, -3.861377020970580443 ) ) ;
#5325=VECTOR ( 'NONE', #49906, 1000.000000000000000 ) ;
#5327=ORIENTED_EDGE ( 'NONE', *, *, #61815, .T. ) ;
#5331=CARTESIAN_POINT ( 'NONE',  ( -5.000000000000000888, -160.6875000027311842, -2.071067811865475949 ) ) ;
#5333=CARTESIAN_POINT ( 'NONE',  ( 1.975475456537005874E-15, -49.62499999726880873, 5.000000000000000000 ) ) ;
#5341=DIRECTION ( 'NONE',  ( -0.000000000000000000, 1.000000000000000000, -0.000000000000000000 ) ) ;
#5342=CARTESIAN_POINT ( 'NONE',  ( -3.152548672688508926E-16, -18.56249999863440792, -5.148502694627439702 ) ) ;
#5343=CARTESIAN_POINT ( 'NONE',  ( -1.127183054612291972E-14, 23.25000000000000000, 4.999999999999999112 ) ) ;
#5344=CARTESIAN_POINT ( 'NONE',  ( -5.000000000000000000, -155.5000000000000000, -6.123233995736766282E-16 ) ) ;
#5347=CARTESIAN_POINT ( 'NONE',  ( -2.229367062500000163, -46.72916666530106511, -3.861377020970580443 ) ) ;
#5348=CARTESIAN_POINT ( 'NONE',  ( -6.972266317189433020E-16, 25.74999999999999645, -5.000000000000000000 ) ) ;
#5350=CARTESIAN_POINT ( 'NONE',  ( 9.457646018065525792E-16, -89.06249999863439371, 5.148502694627439702 ) ) ;
#5353=CARTESIAN_POINT ( 'NONE',  ( -4.458734124999998549, 7.770833334698925121, 2.574251347313722516 ) ) ;
#5355=CARTESIAN_POINT ( 'NONE',  ( -9.184850993605147944E-16, -165.3750000027312126, 5.000000000000000000 ) ) ;
#5356=CARTESIAN_POINT ( 'NONE',  ( -2.229367062499996610, 21.60416666803226349, 3.861377020970582219 ) ) ;
#5358=CARTESIAN_POINT ( 'NONE',  ( -2.499999999999996447, 9.291666669397853795, 4.330127018922195425 ) ) ;
#5359=ORIENTED_EDGE ( 'NONE', *, *, #46706, .T. ) ;
#5362=CARTESIAN_POINT ( 'NONE',  ( 5.000000000000000000, -85.49999999999998579, -6.123233995736766282E-16 ) ) ;
#5363=CARTESIAN_POINT ( 'NONE',  ( 2.229367062499998831, -40.64583333196773651, -3.861377020970580887 ) ) ;
#5365=CARTESIAN_POINT ( 'NONE',  ( -5.000000000000000000, -39.95833333060213732, -2.886751345948128211 ) ) ;
#5368=CARTESIAN_POINT ( 'NONE',  ( -4.458734124999999437, -11.31249999863440792, 0.000000000000000000 ) ) ;
#5369=CARTESIAN_POINT ( 'NONE',  ( -4.458734124999999437, -12.56249999863440259, 0.000000000000000000 ) ) ;
#5370=ORIENTED_EDGE ( 'NONE', *, *, #6689, .F. ) ;
#5371=CARTESIAN_POINT ( 'NONE',  ( 1.060575238724906964E-15, -82.75000000000001421, 5.773502691896257311 ) ) ;
#5372=CARTESIAN_POINT ( 'NONE',  ( -3.152801135295367985, -168.8125000013656063, 3.152801135295367096 ) ) ;
#5374=CARTESIAN_POINT ( 'NONE',  ( -2.499999999999996447, -83.70833333060214443, 4.330127018922195425 ) ) ;
#5375=CARTESIAN_POINT ( 'NONE',  ( -2.500000000000000444, -32.16666666666666430, -4.330127018922193649 ) ) ;
#5376=ORIENTED_EDGE ( 'NONE', *, *, #35458, .F. ) ;
#5378=CARTESIAN_POINT ( 'NONE',  ( -3.152548672688508926E-16, -26.81249999863440436, -5.148502694627439702 ) ) ;
#5379=CARTESIAN_POINT ( 'NONE',  ( 5.000000000000000000, -29.50000000000000000, -6.123233995736766282E-16 ) ) ;
#5382=CARTESIAN_POINT ( 'NONE',  ( 4.458734125000000326, -164.6250000013655779, -1.846868145590734978 ) ) ;
#5385=ORIENTED_EDGE ( 'NONE', *, *, #27823, .F. ) ;
#5387=CARTESIAN_POINT ( 'NONE',  ( 4.458734124999998549, -72.97916666530107932, -2.574251347313721627 ) ) ;
#5390=CARTESIAN_POINT ( 'NONE',  ( -4.458734124999999437, -147.1875000013656063, -5.460374474430324690E-16 ) ) ;
#5392=CARTESIAN_POINT ( 'NONE',  ( -2.499999999999996447, 28.16666666666666785, 4.330127018922195425 ) ) ;
#5396=CARTESIAN_POINT ( 'NONE',  ( -4.458734125000001214, -142.1250000013656063, 1.846868145590734089 ) ) ;
#5399=CARTESIAN_POINT ( 'NONE',  ( -5.000000000000000000, -53.08333333333332860, -2.886751345948128211 ) ) ;
#5401=CARTESIAN_POINT ( 'NONE',  ( -2.229367062500000163, -71.72916666530107932, -3.861377020970580443 ) ) ;
#5402=CARTESIAN_POINT ( 'NONE',  ( -2.071067811865562991, -144.4375000027311842, 4.999999999999913847 ) ) ;
#5403=CARTESIAN_POINT ( 'NONE',  ( -2.500000000000000444, -70.16666666666667140, -4.330127018922193649 ) ) ;
#5405=ORIENTED_EDGE ( 'NONE', *, *, #46516, .T. ) ;
#5411=CARTESIAN_POINT ( 'NONE',  ( -4.458734124999997661, 19.52083333469893134, 2.574251347313722516 ) ) ;
#5419=CARTESIAN_POINT ( 'NONE',  ( -4.458734124999999437, 1.687500001365593194, 0.000000000000000000 ) ) ;
#5420=ORIENTED_EDGE ( 'NONE', *, *, #35544, .T. ) ;
#5421=CARTESIAN_POINT ( 'NONE',  ( 4.458734124999998549, -31.97916666530107577, -2.574251347313721627 ) ) ;
#5424=CARTESIAN_POINT ( 'NONE',  ( -2.229367062499996610, 27.85416666803225993, 3.861377020970582219 ) ) ;
#5427=CARTESIAN_POINT ( 'NONE',  ( -2.229367062499996610, -74.39583333196773651, 3.861377020970582219 ) ) ;
#5430=CARTESIAN_POINT ( 'NONE',  ( -3.535250795749689387E-16, 25.87500000273118772, -5.773502691896257311 ) ) ;
#5434=CARTESIAN_POINT ( 'NONE',  ( -2.500000000000000444, -18.16666666666666430, -4.330127018922193649 ) ) ;
#5435=CARTESIAN_POINT ( 'NONE',  ( 4.458734125000001214, -21.89583333196773296, 2.574251347313718519 ) ) ;
#5437=CARTESIAN_POINT ( 'NONE',  ( -4.458734124999997661, -81.22916666530106511, 2.574251347313722516 ) ) ;
#5438=CARTESIAN_POINT ( 'NONE',  ( -2.500000000000000444, -19.04166666393547658, -4.330127018922193649 ) ) ;
#5439=CARTESIAN_POINT ( 'NONE',  ( -4.458734124999999437, -51.31249999863440792, 0.000000000000000000 ) ) ;
#5442=CARTESIAN_POINT ( 'NONE',  ( -2.500000000000000444, -28.04166666393548013, -4.330127018922193649 ) ) ;
#5443=CARTESIAN_POINT ( 'NONE',  ( 4.458734124999998549, 0.02083333469892617584, -2.574251347313721627 ) ) ;
#5444=ORIENTED_EDGE ( 'NONE', *, *, #33469, .F. ) ;
#5446=CARTESIAN_POINT ( 'NONE',  ( 2.500000000000002220, -64.66666666666665719, 4.330127018922192761 ) ) ;
#5447=CARTESIAN_POINT ( 'NONE',  ( -4.458734124999999437, -153.1875000013656063, -5.460374474430324690E-16 ) ) ;
#5450=CARTESIAN_POINT ( 'NONE',  ( 3.535533905932736864, -161.1250000000000284, 3.535533905932738641 ) ) ;
#5451=CARTESIAN_POINT ( 'NONE',  ( -1.339745962155610925, 7.330341803992665994, 5.000000000000000000 ) ) ;
#5453=CARTESIAN_POINT ( 'NONE',  ( 4.458734124999999437, -9.062499998634406140, -5.460374474430324690E-16 ) ) ;
#5454=CARTESIAN_POINT ( 'NONE',  ( -4.458734124999999437, -46.64583333196774362, -2.574251347313719407 ) ) ;
#5456=FACE_OUTER_BOUND ( 'NONE', #61812, .T. ) ;
#5457=CARTESIAN_POINT ( 'NONE',  ( -4.458734125000000326, -145.0000000013656063, -1.846868145590735644 ) ) ;
#5461=( BOUNDED_CURVE ( )  B_SPLINE_CURVE ( 2, ( #62403, #8671, #38557, #28284, #37949, #47897, #47592, #37625, #43694 ),
 .UNSPECIFIED., .F., .F. ) 
 B_SPLINE_CURVE_WITH_KNOTS ( ( 3, 2, 2, 2, 3 ),
 ( 0.9479166666666666297, 0.9486111111111110716, 0.9499999999999999556, 0.9513888888888888395, 0.9520833333333332815 ),
 .UNSPECIFIED. ) 
 CURVE ( )  GEOMETRIC_REPRESENTATION_ITEM ( )  RATIONAL_B_SPLINE_CURVE ( ( 0.9330127018922194093, 0.9330127018922194093, 1.000000000000000000, 0.8660254037844387076, 1.000000000000000000, 0.8660254037844387076, 1.000000000000000000, 0.9330127018922194093, 0.9330127018922194093 ) ) 
 REPRESENTATION_ITEM ( '' )  );
#5464=CARTESIAN_POINT ( 'NONE',  ( -2.229367062499996610, 28.60416666803226349, 3.861377020970582219 ) ) ;
#5466=CARTESIAN_POINT ( 'NONE',  ( 1.339745962155612702, -30.29465819873851729, -5.000000000000000000 ) ) ;
#5467=VERTEX_POINT ( 'NONE', #4636 ) ;
#5473=CARTESIAN_POINT ( 'NONE',  ( 2.229367062499998831, -4.645833331967740065, -3.861377020970580887 ) ) ;
#5474=DIRECTION ( 'NONE',  ( -0.000000000000000000, 1.000000000000000000, -0.000000000000000000 ) ) ;
#5475=CARTESIAN_POINT ( 'NONE',  ( 2.730187237215162345E-16, -148.1875000013656063, -4.458734124999999437 ) ) ;
#5482=CARTESIAN_POINT ( 'NONE',  ( 1.339745962155615144, -85.58034179853028434, 4.999999999999999112 ) ) ;
#5487=CARTESIAN_POINT ( 'NONE',  ( 1.975475456537005874E-15, -22.74999999999999645, 5.000000000000000000 ) ) ;
#5489=CARTESIAN_POINT ( 'NONE',  ( -2.499999999999996447, -89.70833333060214443, 4.330127018922195425 ) ) ;
#5490=DIRECTION ( 'NONE',  ( -0.000000000000000000, 1.000000000000000000, -0.000000000000000000 ) ) ;
#5491=CARTESIAN_POINT ( 'NONE',  ( 2.229367062499998831, 16.35416666803225993, -3.861377020970580887 ) ) ;
#5493=VERTEX_POINT ( 'NONE', #38419 ) ;
#5494=CARTESIAN_POINT ( 'NONE',  ( 2.229367062499998831, -10.89583333196773829, -3.861377020970580887 ) ) ;
#5496=CARTESIAN_POINT ( 'NONE',  ( -4.458734124999999437, -164.9375000013655779, -5.460374474430324690E-16 ) ) ;
#5497=CARTESIAN_POINT ( 'NONE',  ( 3.061616997868383141E-16, -166.8750000027312126, -5.000000000000000000 ) ) ;
#5502=CARTESIAN_POINT ( 'NONE',  ( -4.458734124999999437, -154.2500000013656063, -1.846868145590735644 ) ) ;
#5505=DIRECTION ( 'NONE',  ( 0.000000000000000000, 0.000000000000000000, 1.000000000000000000 ) ) ;
#5506=ORIENTED_EDGE ( 'NONE', *, *, #4027, .T. ) ;
#5509=( BOUNDED_CURVE ( )  B_SPLINE_CURVE ( 2, ( #12049, #41622, #10856, #3053, #2116, #59764, #22030, #30471, #32301 ),
 .UNSPECIFIED., .F., .F. ) 
 B_SPLINE_CURVE_WITH_KNOTS ( ( 3, 2, 2, 2, 3 ),
 ( 0.9749999999999998668, 0.9791666666666665186, 0.9833333333333331705, 0.9874999999999999334, 0.9916666666666665853 ),
 .UNSPECIFIED. ) 
 CURVE ( )  GEOMETRIC_REPRESENTATION_ITEM ( )  RATIONAL_B_SPLINE_CURVE ( ( 1.000000000000001998, 0.9238795325112847401, 1.000000000000000000, 0.9238795325112867385, 1.000000000000000000, 0.9238795325112867385, 1.000000000000000000, 0.9238795325112887369, 0.9999999999999980016 ) ) 
 REPRESENTATION_ITEM ( '' )  );
#5511=CARTESIAN_POINT ( 'NONE',  ( 5.000000000000000888, -4.583333333333334814, 2.886751345948126879 ) ) ;
#5513=CARTESIAN_POINT ( 'NONE',  ( 4.458734124999998549, -65.72916666530106511, -2.574251347313721627 ) ) ;
#5515=EDGE_CURVE ( 'NONE', #8855, #5467, #9154, .T. ) ;
#5516=EDGE_CURVE ( 'NONE', #27844, #32427, #58675, .T. ) ;
#5517=CARTESIAN_POINT ( 'NONE',  ( -3.535250795749689387E-16, -4.124999997268816720, -5.773502691896257311 ) ) ;
#5518=CARTESIAN_POINT ( 'NONE',  ( -4.458734124999999437, -35.39583333196773651, -2.574251347313719407 ) ) ;
#5520=DIRECTION ( 'NONE',  ( 0.000000000000000000, 0.000000000000000000, 1.000000000000000000 ) ) ;
#5521=CARTESIAN_POINT ( 'NONE',  ( -2.499999999999996447, -47.70833333060215153, 4.330127018922195425 ) ) ;
#5523=CARTESIAN_POINT ( 'NONE',  ( 5.000000000000000888, -48.58333333333332149, 2.886751345948126879 ) ) ;
#5526=CARTESIAN_POINT ( 'NONE',  ( 5.000000000000000000, -4.499999999999997335, -6.123233995736766282E-16 ) ) ;
#5527=CARTESIAN_POINT ( 'NONE',  ( -4.458734124999999437, -70.39583333196773651, -2.574251347313719407 ) ) ;
#5528=CARTESIAN_POINT ( 'NONE',  ( 4.458734124999999437, -143.7500000013655779, 1.846868145590737864 ) ) ;
#5529=CARTESIAN_POINT ( 'NONE',  ( 4.458734124999998549, -79.72916666530107932, -2.574251347313721627 ) ) ;
#5531=ADVANCED_FACE ( 'NONE', ( #28768 ), #34217, .T. ) ;
#5532=CARTESIAN_POINT ( 'NONE',  ( 4.458734124999998549, -31.97916666530107577, -2.574251347313721627 ) ) ;
#5533=CARTESIAN_POINT ( 'NONE',  ( 2.500000000000002220, -73.54166666393548724, 4.330127018922192761 ) ) ;
#5534=EDGE_LOOP ( 'NONE', ( #22129, #51968, #9111, #25877 ) ) ;
#5536=ORIENTED_EDGE ( 'NONE', *, *, #40165, .F. ) ;
#5537=EDGE_CURVE ( 'NONE', #34977, #43111, #40595, .T. ) ;
#5540=( NAMED_UNIT ( * ) PLANE_ANGLE_UNIT ( ) SI_UNIT ( $, .RADIAN. ) );
#5542=CARTESIAN_POINT ( 'NONE',  ( -1.339745962155613812, -39.20534180126147561, -5.000000000000000000 ) ) ;
#5543=CARTESIAN_POINT ( 'NONE',  ( -2.500000000000000444, -76.04166666393547303, -4.330127018922193649 ) ) ;
#5544=CARTESIAN_POINT ( 'NONE',  ( 4.458734124999998549, -57.97916666530107221, -2.574251347313721627 ) ) ;
#5546=ORIENTED_EDGE ( 'NONE', *, *, #50260, .F. ) ;
#5548=DIRECTION ( 'NONE',  ( -0.000000000000000000, 1.000000000000000000, -0.000000000000000000 ) ) ;
#5549=CARTESIAN_POINT ( 'NONE',  ( -2.229367062500000163, 15.52083333469892779, -3.861377020970580443 ) ) ;
#5551=CARTESIAN_POINT ( 'NONE',  ( -5.000000000000000000, -1.000000000000000888, 0.000000000000000000 ) ) ;
#5552=CARTESIAN_POINT ( 'NONE',  ( 2.730187237215162345E-16, -159.1875000013655779, -4.458734124999999437 ) ) ;
#5553=CARTESIAN_POINT ( 'NONE',  ( 0.000000000000000000, -170.0000000000000000, 0.000000000000000000 ) ) ;
#5554=ORIENTED_EDGE ( 'NONE', *, *, #59026, .F. ) ;
#5560=FACE_OUTER_BOUND ( 'NONE', #9988, .T. ) ;
#5568=CARTESIAN_POINT ( 'NONE',  ( 2.229367062500001939, 4.770833334698926897, 3.861377020970579999 ) ) ;
#5571=CARTESIAN_POINT ( 'NONE',  ( 3.061616997868383141E-16, -148.8750000027312126, -5.000000000000000000 ) ) ;
#5572=DIRECTION ( 'NONE',  ( -0.000000000000000000, 1.000000000000000000, -0.000000000000000000 ) ) ;
#5576=DIRECTION ( 'NONE',  ( -0.000000000000000000, 1.000000000000000000, -0.000000000000000000 ) ) ;
#5579=CARTESIAN_POINT ( 'NONE',  ( -4.458734125000000326, -166.1250000013656063, 1.846868145590734089 ) ) ;
#5580=CARTESIAN_POINT ( 'NONE',  ( -3.535533905932737309, -160.6250000000000284, -3.535533905932738197 ) ) ;
#5581=CARTESIAN_POINT ( 'NONE',  ( 1.339745962155615144, -45.58034179853028434, 4.999999999999999112 ) ) ;
#5583=CARTESIAN_POINT ( 'NONE',  ( 3.152801135295366208, -142.5625000013655779, 3.152801135295367985 ) ) ;
#5584=ORIENTED_EDGE ( 'NONE', *, *, #62908, .T. ) ;
#5585=CARTESIAN_POINT ( 'NONE',  ( -4.458734124999999437, 27.43750000136559208, 0.000000000000000000 ) ) ;
#5586=ORIENTED_EDGE ( 'NONE', *, *, #55068, .T. ) ;
#5587=CARTESIAN_POINT ( 'NONE',  ( 4.458734125000000326, -64.14583333196773651, 2.574251347313718519 ) ) ;
#5590=CARTESIAN_POINT ( 'NONE',  ( -4.999999999999999112, 12.08333333333333037, 2.886751345948131764 ) ) ;
#5593=CARTESIAN_POINT ( 'NONE',  ( 2.229367062499998831, -50.64583333196772941, -3.861377020970580887 ) ) ;
#5594=CARTESIAN_POINT ( 'NONE',  ( -4.458734124999999437, -12.39583333196774184, -2.574251347313719407 ) ) ;
#5595=CARTESIAN_POINT ( 'NONE',  ( -5.000000000000000000, -168.5000000000000000, -6.123233995736766282E-16 ) ) ;
#5603=EDGE_CURVE ( 'NONE', #51386, #61158, #23712, .T. ) ;
#5605=CARTESIAN_POINT ( 'NONE',  ( -4.458734124999999437, -56.31249999863440081, 0.000000000000000000 ) ) ;
#5606=CARTESIAN_POINT ( 'NONE',  ( -3.152801135295367096, -155.3125000013656063, -3.152801135295367541 ) ) ;
#5607=ADVANCED_FACE ( 'NONE', ( #790 ), #25535, .T. ) ;
#5610=CARTESIAN_POINT ( 'NONE',  ( 1.060575238724906964E-15, -56.62499999726880162, 5.773502691896257311 ) ) ;
#5611=EDGE_LOOP ( 'NONE', ( #59915, #55148, #5619, #18113 ) ) ;
#5613=CARTESIAN_POINT ( 'NONE',  ( -4.458734124999998549, 2.520833334698928674, 2.574251347313722516 ) ) ;
#5617=CARTESIAN_POINT ( 'NONE',  ( -4.458734124999999437, -154.9375000013655779, -5.460374474430324690E-16 ) ) ;
#5619=ORIENTED_EDGE ( 'NONE', *, *, #41684, .T. ) ;
#5624=CARTESIAN_POINT ( 'NONE',  ( 9.457646018065525792E-16, -44.31249999863440081, 5.148502694627439702 ) ) ;
#5627=CYLINDRICAL_SURFACE ( 'NONE', #49055, 5.000000000000000000 ) ;
#5629=CARTESIAN_POINT ( 'NONE',  ( -4.458734124999999437, -89.56249999863440792, 0.000000000000000000 ) ) ;
#5632=CARTESIAN_POINT ( 'NONE',  ( 0.000000000000000000, -170.0000000000000000, 0.000000000000000000 ) ) ;
#5639=CARTESIAN_POINT ( 'NONE',  ( 1.255007937094098239E-14, 24.75000000000000000, -4.999999999999999112 ) ) ;
#5640=CARTESIAN_POINT ( 'NONE',  ( 0.000000000000000000, -170.0000000000000000, 0.000000000000000000 ) ) ;
#5644=VERTEX_POINT ( 'NONE', #34873 ) ;
#5647=CARTESIAN_POINT ( 'NONE',  ( -5.000000000000000000, -159.6250000027311842, -6.123233995736766282E-16 ) ) ;
#5650=CARTESIAN_POINT ( 'NONE',  ( -1.339745962155623360, 22.20534180126147561, 4.999999999999991118 ) ) ;
#5652=CARTESIAN_POINT ( 'NONE',  ( -1.339745962155610925, -71.66965819600733312, 5.000000000000000000 ) ) ;
#5653=VECTOR ( 'NONE', #54026, 1000.000000000000000 ) ;
#5660=CARTESIAN_POINT ( 'NONE',  ( 4.458734125000000326, -21.89583333196773296, 2.574251347313718519 ) ) ;
#5661=CARTESIAN_POINT ( 'NONE',  ( 2.500000000000002220, -75.66666666666665719, 4.330127018922192761 ) ) ;
#5662=CARTESIAN_POINT ( 'NONE',  ( -5.000000000000000888, -155.5625000000000568, -2.071067811865475949 ) ) ;
#5664=CARTESIAN_POINT ( 'NONE',  ( 3.152801135295367541, -155.3125000013656063, -3.152801135295367541 ) ) ;
#5665=VERTEX_POINT ( 'NONE', #30994 ) ;
#5666=CARTESIAN_POINT ( 'NONE',  ( 4.458734125000000326, -47.14583333196774362, 2.574251347313718519 ) ) ;
#5667=( BOUNDED_CURVE ( )  B_SPLINE_CURVE ( 2, ( #26572, #12411, #22708, #2456, #57436, #32659, #52287, #7908, #32023 ),
 .UNSPECIFIED., .F., .F. ) 
 B_SPLINE_CURVE_WITH_KNOTS ( ( 3, 2, 2, 2, 3 ),
 ( 0.6020833333333333037, 0.6027777777777777457, 0.6041666666666666297, 0.6055555555555555136, 0.6062499999999999556 ),
 .UNSPECIFIED. ) 
 CURVE ( )  GEOMETRIC_REPRESENTATION_ITEM ( )  RATIONAL_B_SPLINE_CURVE ( ( 0.9330127018922194093, 0.9330127018922194093, 1.000000000000000000, 0.8660254037844387076, 1.000000000000000000, 0.8660254037844387076, 1.000000000000000000, 0.9330127018922194093, 0.9330127018922194093 ) ) 
 REPRESENTATION_ITEM ( '' )  );
#5668=CARTESIAN_POINT ( 'NONE',  ( 1.339745962155615144, -44.58034179853027723, 4.999999999999999112 ) ) ;
#5670=CARTESIAN_POINT ( 'NONE',  ( -3.535250795749689387E-16, 27.75000000000000000, -5.773502691896257311 ) ) ;
#5672=CARTESIAN_POINT ( 'NONE',  ( -4.458734124999998549, 8.770833334698927786, 2.574251347313722516 ) ) ;
#5674=CARTESIAN_POINT ( 'NONE',  ( -5.000000000000000000, -68.99999999999998579, 0.000000000000000000 ) ) ;
#5676=CARTESIAN_POINT ( 'NONE',  ( -4.458734124999998549, 20.52083333469892423, 2.574251347313722516 ) ) ;
#5678=CARTESIAN_POINT ( 'NONE',  ( -2.499999999999996447, 6.291666669397851130, 4.330127018922195425 ) ) ;
#5679=EDGE_LOOP ( 'NONE', ( #1672, #52977, #6660, #48571 ) ) ;
#5680=CARTESIAN_POINT ( 'NONE',  ( 5.000000000000000000, -162.1875000027311842, 2.071067811865478614 ) ) ;
#5683=CARTESIAN_POINT ( 'NONE',  ( 4.458734124999999437, -39.81249999863440081, -5.460374474430324690E-16 ) ) ;
#5684=CARTESIAN_POINT ( 'NONE',  ( -5.000000000000000000, -40.95833333060215153, -2.886751345948128211 ) ) ;
#5686=CARTESIAN_POINT ( 'NONE',  ( -2.229367062500000163, -12.47916666530107044, -3.861377020970580443 ) ) ;
#5687=CARTESIAN_POINT ( 'NONE',  ( -2.229367062499996610, -17.39583333196773651, 3.861377020970582219 ) ) ;
#5689=CARTESIAN_POINT ( 'NONE',  ( 2.499999999999998668, -83.33333333333332860, -4.330127018922193649 ) ) ;
#5690=CARTESIAN_POINT ( 'NONE',  ( -3.152801135295367985, -166.8125000013656063, 3.152801135295367096 ) ) ;
#5692=( BOUNDED_CURVE ( )  B_SPLINE_CURVE ( 2, ( #34292, #49729, #20469, #9840, #19819, #39428, #59069, #35899, #56160 ),
 .UNSPECIFIED., .F., .F. ) 
 B_SPLINE_CURVE_WITH_KNOTS ( ( 3, 2, 2, 2, 3 ),
 ( 0.5520833333333333703, 0.5527777777777778123, 0.5541666666666666963, 0.5555555555555555802, 0.5562500000000000222 ),
 .UNSPECIFIED. ) 
 CURVE ( )  GEOMETRIC_REPRESENTATION_ITEM ( )  RATIONAL_B_SPLINE_CURVE ( ( 0.9330127018922194093, 0.9330127018922194093, 1.000000000000000000, 0.8660254037844387076, 1.000000000000000000, 0.8660254037844387076, 1.000000000000000000, 0.9330127018922194093, 0.9330127018922194093 ) ) 
 REPRESENTATION_ITEM ( '' )  );
#5693=CARTESIAN_POINT ( 'NONE',  ( 2.500000000000002220, -88.54166666393548724, 4.330127018922192761 ) ) ;
#5694=CARTESIAN_POINT ( 'NONE',  ( -2.500000000000000444, -49.04166666393547303, -4.330127018922193649 ) ) ;
#5695=ORIENTED_EDGE ( 'NONE', *, *, #31000, .T. ) ;
#5697=CARTESIAN_POINT ( 'NONE',  ( 4.458734125000001214, -29.14583333196774362, 2.574251347313718519 ) ) ;
#5701=CARTESIAN_POINT ( 'NONE',  ( 1.846868145590735200, -162.5000000013655779, -4.458734125000000326 ) ) ;
#5703=CARTESIAN_POINT ( 'NONE',  ( 2.499999999999998668, -23.33333333333333215, -4.330127018922193649 ) ) ;
#5704=ORIENTED_EDGE ( 'NONE', *, *, #7073, .T. ) ;
#5706=CARTESIAN_POINT ( 'NONE',  ( -2.229367062500000163, -76.72916666530106511, -3.861377020970580443 ) ) ;
#5709=CARTESIAN_POINT ( 'NONE',  ( 2.730187237215162345E-16, -145.4375000013656063, -4.458734124999999437 ) ) ;
#5710=DIRECTION ( 'NONE',  ( -0.000000000000000000, 1.000000000000000000, -0.000000000000000000 ) ) ;
#5715=CARTESIAN_POINT ( 'NONE',  ( 2.730187237215162345E-16, -140.4375000013656063, -4.458734124999999437 ) ) ;
#5718=DIRECTION ( 'NONE',  ( -0.000000000000000000, 1.000000000000000000, -0.000000000000000000 ) ) ;
#5720=CARTESIAN_POINT ( 'NONE',  ( -4.458734124999999437, -75.56249999863440792, 0.000000000000000000 ) ) ;
#5722=DIRECTION ( 'NONE',  ( 0.000000000000000000, 0.000000000000000000, 1.000000000000000000 ) ) ;
#5723=CARTESIAN_POINT ( 'NONE',  ( 2.499999999999998668, 14.79166666939785202, -4.330127018922193649 ) ) ;
#5727=CARTESIAN_POINT ( 'NONE',  ( -2.499999999999996447, -14.70833333060214976, 4.330127018922195425 ) ) ;
#5732=CARTESIAN_POINT ( 'NONE',  ( -4.458734124999997661, 16.52083333469892779, 2.574251347313722516 ) ) ;
#5733=DIRECTION ( 'NONE',  ( 0.000000000000000000, 0.000000000000000000, 1.000000000000000000 ) ) ;
#5739=CARTESIAN_POINT ( 'NONE',  ( 9.457646018065525792E-16, -6.062499998634404363, 5.148502694627439702 ) ) ;
#5740=CARTESIAN_POINT ( 'NONE',  ( -4.458734124999999437, -30.64583333196774007, -2.574251347313719407 ) ) ;
#5745=CARTESIAN_POINT ( 'NONE',  ( -3.152548672688508926E-16, 23.43750000136559564, -5.148502694627439702 ) ) ;
#5748=CARTESIAN_POINT ( 'NONE',  ( -4.458734124999999437, -77.56249999863440792, 0.000000000000000000 ) ) ;
#5751=CARTESIAN_POINT ( 'NONE',  ( 2.499999999999998668, 23.79166666939785202, -4.330127018922193649 ) ) ;
#5752=ORIENTED_EDGE ( 'NONE', *, *, #13866, .F. ) ;
#5754=CARTESIAN_POINT ( 'NONE',  ( -1.339745962155613812, -57.08034179853028434, -5.000000000000000000 ) ) ;
#5755=CARTESIAN_POINT ( 'NONE',  ( -5.000000000000000000, -19.08333333333333570, -2.886751345948128211 ) ) ;
#5756=CARTESIAN_POINT ( 'NONE',  ( -3.152548672688508926E-16, -24.56249999863440792, -5.148502694627439702 ) ) ;
#5757=CARTESIAN_POINT ( 'NONE',  ( 9.457646018065525792E-16, -84.06249999863439371, 5.148502694627439702 ) ) ;
#5758=CARTESIAN_POINT ( 'NONE',  ( 2.499999999999998668, -25.20833333060214443, -4.330127018922193649 ) ) ;
#5759=CARTESIAN_POINT ( 'NONE',  ( 4.458734124999999437, -47.81249999863440792, -5.460374474430324690E-16 ) ) ;
#5760=VERTEX_POINT ( 'NONE', #49661 ) ;
#5762=CARTESIAN_POINT ( 'NONE',  ( 0.000000000000000000, -170.0000000000000000, 0.000000000000000000 ) ) ;
#5763=CARTESIAN_POINT ( 'NONE',  ( 2.229367062499998831, -1.895833331967737623, -3.861377020970580887 ) ) ;
#5764=ORIENTED_EDGE ( 'NONE', *, *, #35467, .F. ) ;
#5766=CARTESIAN_POINT ( 'NONE',  ( -4.999999999999999112, -65.91666666666665719, 2.886751345948131764 ) ) ;
#5767=CARTESIAN_POINT ( 'NONE',  ( 4.458734125000000326, -151.6250000013656063, -1.846868145590734978 ) ) ;
#5770=CARTESIAN_POINT ( 'NONE',  ( 5.000000000000000888, -159.9375000000000000, -2.071067811865475505 ) ) ;
#5771=CARTESIAN_POINT ( 'NONE',  ( -1.339745962155613812, 6.919658201469707670, -5.000000000000000000 ) ) ;
#5773=CARTESIAN_POINT ( 'NONE',  ( -3.152548672688508926E-16, -12.81249999863440259, -5.148502694627439702 ) ) ;
#5774=CARTESIAN_POINT ( 'NONE',  ( 4.458734124999998549, -44.97916666530107221, -2.574251347313721627 ) ) ;
#5775=CARTESIAN_POINT ( 'NONE',  ( -1.846868145590737420, -142.7500000013656063, 4.458734124999999437 ) ) ;
#5778=ORIENTED_EDGE ( 'NONE', *, *, #50340, .T. ) ;
#5779=CARTESIAN_POINT ( 'NONE',  ( -6.972266317189433020E-16, -33.12499999726880873, -5.000000000000000000 ) ) ;
#5780=DIRECTION ( 'NONE',  ( -0.8660254037844505870, -0.4999999999999792388, 0.000000000000000000 ) ) ;
#5783=CARTESIAN_POINT ( 'NONE',  ( -2.499999999999996447, -61.83333333333333570, 4.330127018922195425 ) ) ;
#5785=AXIS2_PLACEMENT_3D ( 'NONE', #45684, #30236, #40848 ) ;
#5787=VECTOR ( 'NONE', #42026, 1000.000000000000000 ) ;
#5791=CARTESIAN_POINT ( 'NONE',  ( -2.500000000000000444, 1.958333336064519647, -4.330127018922193649 ) ) ;
#5792=CARTESIAN_POINT ( 'NONE',  ( -4.458734124999999437, -7.395833331967734736, -2.574251347313719407 ) ) ;
#5794=CARTESIAN_POINT ( 'NONE',  ( 4.458734124999999437, -150.4375000013656063, 0.000000000000000000 ) ) ;
#5809=CARTESIAN_POINT ( 'NONE',  ( 2.229367062500001939, 12.02083333469892601, 3.861377020970579999 ) ) ;
#5812=CARTESIAN_POINT ( 'NONE',  ( -4.458734124999999437, -14.56249999863440436, 0.000000000000000000 ) ) ;
#5814=CARTESIAN_POINT ( 'NONE',  ( 4.458734124999999437, -165.4375000013655779, 0.000000000000000000 ) ) ;
#5815=CARTESIAN_POINT ( 'NONE',  ( 1.975475456537005874E-15, -40.62499999726879452, 5.000000000000000000 ) ) ;
#5820=EDGE_CURVE ( 'NONE', #23906, #25310, #54113, .T. ) ;
#5821=CARTESIAN_POINT ( 'NONE',  ( -4.729367062499999719, 29.28125000204839168, 0.000000000000000000 ) ) ;
#5825=CARTESIAN_POINT ( 'NONE',  ( 2.730187237215162345E-16, -151.4375000013656063, -4.458734124999999437 ) ) ;
#5827=CARTESIAN_POINT ( 'NONE',  ( 6.123233995736766282E-16, -170.0000000000000000, -5.000000000000000000 ) ) ;
#5833=CARTESIAN_POINT ( 'NONE',  ( -4.999999999999998224, -8.791666663935483683, 2.886751345948131764 ) ) ;
#5834=CARTESIAN_POINT ( 'NONE',  ( -4.999999999999999112, 0.08333333333333457771, 2.886751345948131764 ) ) ;
#5836=CARTESIAN_POINT ( 'NONE',  ( -2.229367062499996610, -66.14583333196773651, 3.861377020970582219 ) ) ;
#5839=CARTESIAN_POINT ( 'NONE',  ( 2.499999999999998668, -9.208333330602146205, -4.330127018922193649 ) ) ;
#5840=CARTESIAN_POINT ( 'NONE',  ( -4.458734124999998549, -33.22916666530107221, 2.574251347313722516 ) ) ;
#5844=CYLINDRICAL_SURFACE ( 'NONE', #63146, 5.000000000000000000 ) ;
#5848=CARTESIAN_POINT ( 'NONE',  ( 2.499999999999998668, -52.33333333333332860, -4.330127018922193649 ) ) ;
#5849=DIRECTION ( 'NONE',  ( -0.000000000000000000, 1.000000000000000000, -0.000000000000000000 ) ) ;
#5850=( BOUNDED_CURVE ( )  B_SPLINE_CURVE ( 2, ( #3334, #27131, #7206, #2692, #12961, #22634, #42233, #26817, #61238 ),
 .UNSPECIFIED., .F., .F. ) 
 B_SPLINE_CURVE_WITH_KNOTS ( ( 3, 2, 2, 2, 3 ),
 ( 0.8749999999999998890, 0.8791666666666665408, 0.8833333333333330817, 0.8874999999999997335, 0.8916666666666664964 ),
 .UNSPECIFIED. ) 
 CURVE ( )  GEOMETRIC_REPRESENTATION_ITEM ( )  RATIONAL_B_SPLINE_CURVE ( ( 1.000000000000001998, 0.9238795325112847401, 1.000000000000000000, 0.9238795325112867385, 1.000000000000000000, 0.9238795325112867385, 1.000000000000000000, 0.9238795325112908463, 0.9999999999999958922 ) ) 
 REPRESENTATION_ITEM ( '' )  );
#5853=CARTESIAN_POINT ( 'NONE',  ( -2.229367062500000163, -77.47916666530106511, -3.861377020970580443 ) ) ;
#5854=CARTESIAN_POINT ( 'NONE',  ( -1.846868145590737420, -144.0000000013655779, 4.458734124999999437 ) ) ;
#5855=CARTESIAN_POINT ( 'NONE',  ( 2.229367062499998831, -82.64583333196773651, -3.861377020970580887 ) ) ;
#5857=CARTESIAN_POINT ( 'NONE',  ( -2.229367062499996610, -30.39583333196773651, 3.861377020970582219 ) ) ;
#5859=ADVANCED_FACE ( 'NONE', ( #35834 ), #55455, .T. ) ;
#5861=ORIENTED_EDGE ( 'NONE', *, *, #52575, .T. ) ;
#5864=VERTEX_POINT ( 'NONE', #50940 ) ;
#5867=CARTESIAN_POINT ( 'NONE',  ( -2.229367062500000163, -62.72916666530106511, -3.861377020970580443 ) ) ;
#5870=CARTESIAN_POINT ( 'NONE',  ( 6.123233995736766282E-16, -170.0000000000000000, -5.000000000000000000 ) ) ;
#5872=( BOUNDED_CURVE ( )  B_SPLINE_CURVE ( 2, ( #28992, #15163, #48616, #19665, #4555, #24180, #53140, #43475, #5199 ),
 .UNSPECIFIED., .F., .F. ) 
 B_SPLINE_CURVE_WITH_KNOTS ( ( 3, 2, 2, 2, 3 ),
 ( 0.08125000000000000278, 0.08194444444444444475, 0.08333333333333332871, 0.08472222222222222654, 0.08541666666666666852 ),
 .UNSPECIFIED. ) 
 CURVE ( )  GEOMETRIC_REPRESENTATION_ITEM ( )  RATIONAL_B_SPLINE_CURVE ( ( 0.9330127018922194093, 0.9330127018922194093, 1.000000000000000000, 0.8660254037844387076, 1.000000000000000000, 0.8660254037844387076, 1.000000000000000000, 0.9330127018922194093, 0.9330127018922194093 ) ) 
 REPRESENTATION_ITEM ( '' )  );
#5873=CARTESIAN_POINT ( 'NONE',  ( 9.457646018065525792E-16, 10.93750000136559208, 5.148502694627439702 ) ) ;
#5876=CARTESIAN_POINT ( 'NONE',  ( -4.458734124999999437, -160.0000000013656063, -1.846868145590735644 ) ) ;
#5878=FACE_OUTER_BOUND ( 'NONE', #9161, .T. ) ;
#5879=VERTEX_POINT ( 'NONE', #46433 ) ;
#5883=EDGE_CURVE ( 'NONE', #60539, #47703, #34781, .T. ) ;
#5884=DIRECTION ( 'NONE',  ( -0.000000000000000000, 1.000000000000000000, -0.000000000000000000 ) ) ;
#5889=CARTESIAN_POINT ( 'NONE',  ( -1.339745962155613812, -73.08034179853029855, -5.000000000000000000 ) ) ;
#5892=CARTESIAN_POINT ( 'NONE',  ( 1.975475456537005874E-15, -58.75000000000000000, 5.000000000000000000 ) ) ;
#5895=CARTESIAN_POINT ( 'NONE',  ( -3.152548672688508926E-16, -0.8124999986344056957, -5.148502694627439702 ) ) ;
#5897=CARTESIAN_POINT ( 'NONE',  ( 3.535533905932736864, -151.1250000000000000, 3.535533905932738641 ) ) ;
#5899=CARTESIAN_POINT ( 'NONE',  ( 3.535533905932738197, -147.0000000027311842, -3.535533905932738197 ) ) ;
#5904=FACE_OUTER_BOUND ( 'NONE', #55077, .T. ) ;
#5906=EDGE_CURVE ( 'NONE', #29467, #44762, #17789, .T. ) ;
#5908=CARTESIAN_POINT ( 'NONE',  ( 1.846868145590736310, -163.8750000013656063, 4.458734124999997661 ) ) ;
#5909=CARTESIAN_POINT ( 'NONE',  ( -6.972266317189433020E-16, -33.24999999999999289, -5.000000000000000000 ) ) ;
#5912=CARTESIAN_POINT ( 'NONE',  ( 4.458734124999999437, -139.4375000013656063, 0.000000000000000000 ) ) ;
#5914=CARTESIAN_POINT ( 'NONE',  ( 4.458734125000001214, 20.85416666803226349, 2.574251347313718519 ) ) ;
#5915=ORIENTED_EDGE ( 'NONE', *, *, #30182, .F. ) ;
#5917=CARTESIAN_POINT ( 'NONE',  ( 2.229367062500001939, -63.22916666530106511, 3.861377020970579999 ) ) ;
#5920=CARTESIAN_POINT ( 'NONE',  ( -4.999999999999999112, 16.08333333333333215, 2.886751345948131764 ) ) ;
#5921=CARTESIAN_POINT ( 'NONE',  ( 2.229367062500001939, -49.97916666530107221, 3.861377020970579999 ) ) ;
#5922=CARTESIAN_POINT ( 'NONE',  ( -3.152548672688508926E-16, -10.56249999863440792, -5.148502694627439702 ) ) ;
#5924=CARTESIAN_POINT ( 'NONE',  ( -9.184850993605147944E-16, -158.3750000027311842, 5.000000000000000000 ) ) ;
#5925=CARTESIAN_POINT ( 'NONE',  ( -9.184850993605147944E-16, -147.2500000000000284, 5.000000000000000000 ) ) ;
#5926=CARTESIAN_POINT ( 'NONE',  ( -2.500000000000000444, -10.16666666666666430, -4.330127018922193649 ) ) ;
#5927=CARTESIAN_POINT ( 'NONE',  ( -2.499999999999996447, -58.83333333333333570, 4.330127018922195425 ) ) ;
#5931=CARTESIAN_POINT ( 'NONE',  ( -2.229367062499996610, -59.14583333196773651, 3.861377020970582219 ) ) ;
#5932=CARTESIAN_POINT ( 'NONE',  ( 4.458734124999999437, -156.6875000013655779, 0.000000000000000000 ) ) ;
#5933=EDGE_CURVE ( 'NONE', #31664, #15327, #31304, .T. ) ;
#5935=CARTESIAN_POINT ( 'NONE',  ( 5.000000000000000000, -54.37499999726880162, -6.123233995736766282E-16 ) ) ;
#5936=VERTEX_POINT ( 'NONE', #2380 ) ;
#5938=CARTESIAN_POINT ( 'NONE',  ( 4.458734124999998549, -2.979166665301069994, -2.574251347313721627 ) ) ;
#5939=ORIENTED_EDGE ( 'NONE', *, *, #49606, .F. ) ;
#5940=CARTESIAN_POINT ( 'NONE',  ( 3.061616997868383141E-16, -157.8750000027311842, -5.000000000000000000 ) ) ;
#5941=DIRECTION ( 'NONE',  ( 0.000000000000000000, -1.000000000000000000, 0.000000000000000000 ) ) ;
#5942=CARTESIAN_POINT ( 'NONE',  ( -4.458734124999999437, -155.9375000013655779, -5.460374474430324690E-16 ) ) ;
#5943=ORIENTED_EDGE ( 'NONE', *, *, #56408, .T. ) ;
#5947=CARTESIAN_POINT ( 'NONE',  ( 2.229367062500001939, -45.22916666530106511, 3.861377020970579999 ) ) ;
#5949=CARTESIAN_POINT ( 'NONE',  ( 2.500000000000002220, 10.45833333606451987, 4.330127018922192761 ) ) ;
#5951=CARTESIAN_POINT ( 'NONE',  ( 2.229367062500001939, 27.02083333469892423, 3.861377020970579999 ) ) ;
#5954=DIRECTION ( 'NONE',  ( 0.000000000000000000, 0.000000000000000000, 1.000000000000000000 ) ) ;
#5959=CARTESIAN_POINT ( 'NONE',  ( 1.975475456537005874E-15, -33.75000000000000000, 5.000000000000000000 ) ) ;
#5960=ADVANCED_FACE ( 'NONE', ( #42543 ), #61235, .T. ) ;
#5966=FACE_OUTER_BOUND ( 'NONE', #28260, .T. ) ;
#5967=CARTESIAN_POINT ( 'NONE',  ( 2.229367062500001939, -88.22916666530107932, 3.861377020970579999 ) ) ;
#5971=EDGE_CURVE ( 'NONE', #39210, #32568, #60723, .T. ) ;
#5973=CARTESIAN_POINT ( 'NONE',  ( -2.071067811865562991, -143.4375000027312410, 4.999999999999913847 ) ) ;
#5975=CARTESIAN_POINT ( 'NONE',  ( 5.000000000000000888, -156.0625000027312126, -2.071067811865475505 ) ) ;
#5981=ADVANCED_FACE ( 'NONE', ( #42230 ), #46744, .T. ) ;
#5982=CARTESIAN_POINT ( 'NONE',  ( -5.000000000000000000, -67.00000000000000000, 0.000000000000000000 ) ) ;
#5984=( BOUNDED_CURVE ( )  B_SPLINE_CURVE ( 2, ( #22550, #12256, #37642, #57598, #47914 ),
 .UNSPECIFIED., .F., .F. ) 
 B_SPLINE_CURVE_WITH_KNOTS ( ( 3, 2, 3 ),
 ( 0.000000000000000000, 0.001388888888888888942, 0.002083333333333333738 ),
 .UNSPECIFIED. ) 
 CURVE ( )  GEOMETRIC_REPRESENTATION_ITEM ( )  RATIONAL_B_SPLINE_CURVE ( ( 1.000000000000000000, 0.8660254037844387076, 1.000000000000000000, 0.9330127018922192983, 0.9330127018922194093 ) ) 
 REPRESENTATION_ITEM ( '' )  );
#5991=CARTESIAN_POINT ( 'NONE',  ( 1.975475456537005874E-15, -48.62499999726880162, 5.000000000000000000 ) ) ;
#5992=CARTESIAN_POINT ( 'NONE',  ( 2.229367062499998831, -18.64583333196774007, -3.861377020970580887 ) ) ;
#5994=CARTESIAN_POINT ( 'NONE',  ( 2.071067811865475505, -149.8125000000000284, -5.000000000000000888 ) ) ;
#5997=CARTESIAN_POINT ( 'NONE',  ( -4.458734125000001214, -153.8750000013655779, 1.846868145590734089 ) ) ;
#5998=ORIENTED_EDGE ( 'NONE', *, *, #53865, .T. ) ;
#5999=CARTESIAN_POINT ( 'NONE',  ( -4.458734124999997661, -48.47916666530106511, 2.574251347313722516 ) ) ;
#6001=EDGE_CURVE ( 'NONE', #20671, #10973, #3609, .T. ) ;
#6002=EDGE_CURVE ( 'NONE', #52361, #5879, #47687, .T. ) ;
#6003=CARTESIAN_POINT ( 'NONE',  ( -2.229367062499996610, -90.14583333196773651, 3.861377020970582219 ) ) ;
#6004=CARTESIAN_POINT ( 'NONE',  ( 2.229367062499998831, 5.354166668032261711, -3.861377020970580887 ) ) ;
#6006=CARTESIAN_POINT ( 'NONE',  ( -1.339745962155613812, -44.20534180126147561, -5.000000000000000000 ) ) ;
#6008=CARTESIAN_POINT ( 'NONE',  ( 1.975475456537005874E-15, -82.74999999999998579, 5.000000000000000000 ) ) ;
#6009=CARTESIAN_POINT ( 'NONE',  ( -4.458734124999998549, 18.52083333469892779, 2.574251347313722516 ) ) ;
#6011=CARTESIAN_POINT ( 'NONE',  ( 5.000000000000000000, 10.70833333606452165, -2.886751345948129988 ) ) ;
#6012=EDGE_LOOP ( 'NONE', ( #16142, #7599, #62247, #13225 ) ) ;
#6013=CARTESIAN_POINT ( 'NONE',  ( -5.000000000000000000, 7.916666666666665186, -2.886751345948128211 ) ) ;
#6016=CARTESIAN_POINT ( 'NONE',  ( -4.458734124999999437, -45.39583333196773651, -2.574251347313719407 ) ) ;
#6017=CARTESIAN_POINT ( 'NONE',  ( -3.535250795749689387E-16, -38.12499999726881583, -5.773502691896257311 ) ) ;
#6019=CARTESIAN_POINT ( 'NONE',  ( 4.458734125000001214, -16.89583333196773651, 2.574251347313718519 ) ) ;
#6020=ORIENTED_EDGE ( 'NONE', *, *, #25040, .F. ) ;
#6021=CARTESIAN_POINT ( 'NONE',  ( -4.999999999999999112, -81.91666666666665719, 2.886751345948131764 ) ) ;
#6022=CARTESIAN_POINT ( 'NONE',  ( 3.152801135295367541, -168.3125000013656063, -3.152801135295367541 ) ) ;
#6024=CARTESIAN_POINT ( 'NONE',  ( 5.000000000000000000, -85.29166666393547303, -2.886751345948129988 ) ) ;
#6025=CARTESIAN_POINT ( 'NONE',  ( 5.000000000000000000, -20.37499999726880873, -6.123233995736766282E-16 ) ) ;
#6028=VECTOR ( 'NONE', #41913, 1000.000000000000000 ) ;
#6029=CARTESIAN_POINT ( 'NONE',  ( -4.458734124999998549, -26.47916666530107221, 2.574251347313722516 ) ) ;
#6033=CARTESIAN_POINT ( 'NONE',  ( -1.846868145590734756, -164.3750000013656063, -4.458734125000000326 ) ) ;
#6035=ORIENTED_EDGE ( 'NONE', *, *, #23566, .T. ) ;
#6037=CARTESIAN_POINT ( 'NONE',  ( 4.458734125000001214, -76.14583333196773651, 2.574251347313718519 ) ) ;
#6040=CARTESIAN_POINT ( 'NONE',  ( -4.458734125000000326, -143.1250000013656063, 1.846868145590734089 ) ) ;
#6041=CARTESIAN_POINT ( 'NONE',  ( -4.999999999999998224, 23.08333333333333215, 2.886751345948131764 ) ) ;
#6046=CARTESIAN_POINT ( 'NONE',  ( 2.730187237215162345E-16, -141.4375000013656063, -4.458734124999999437 ) ) ;
#6049=CARTESIAN_POINT ( 'NONE',  ( -6.972266317189433020E-16, -40.12499999726880162, -5.000000000000000000 ) ) ;
#6051=CARTESIAN_POINT ( 'NONE',  ( 4.458734124999998549, -75.97916666530106511, -2.574251347313721627 ) ) ;
#6053=CARTESIAN_POINT ( 'NONE',  ( 1.339745962155602488, 14.41965820146970501, 5.000000000000007105 ) ) ;
#6055=( BOUNDED_CURVE ( )  B_SPLINE_CURVE ( 2, ( #62334, #17310, #18255, #36936, #42063, #27585, #52670, #37882, #61705 ),
 .UNSPECIFIED., .F., .F. ) 
 B_SPLINE_CURVE_WITH_KNOTS ( ( 3, 2, 2, 2, 3 ),
 ( 0.5437499999999999556, 0.5444444444444443976, 0.5458333333333332815, 0.5472222222222222765, 0.5479166666666667185 ),
 .UNSPECIFIED. ) 
 CURVE ( )  GEOMETRIC_REPRESENTATION_ITEM ( )  RATIONAL_B_SPLINE_CURVE ( ( 0.9330127018922194093, 0.9330127018922194093, 1.000000000000000000, 0.8660254037844387076, 1.000000000000000000, 0.8660254037844387076, 1.000000000000000000, 0.9330127018922194093, 0.9330127018922194093 ) ) 
 REPRESENTATION_ITEM ( '' )  );
#6056=VERTEX_POINT ( 'NONE', #54334 ) ;
#6057=CARTESIAN_POINT ( 'NONE',  ( -3.535533905932737309, -159.6250000000000284, -3.535533905932738197 ) ) ;
#6058=CARTESIAN_POINT ( 'NONE',  ( -5.000000000000000000, -60.00000000000000000, 0.000000000000000000 ) ) ;
#6062=CARTESIAN_POINT ( 'NONE',  ( -4.458734124999999437, 19.35416666803225993, -2.574251347313719407 ) ) ;
#6067=DIRECTION ( 'NONE',  ( -0.000000000000000000, 1.000000000000000000, -0.000000000000000000 ) ) ;
#6068=CARTESIAN_POINT ( 'NONE',  ( 4.458734124999999437, -87.81249999863439371, -5.460374474430324690E-16 ) ) ;
#6069=CARTESIAN_POINT ( 'NONE',  ( -4.458734124999999437, -4.395833331967740065, -2.574251347313719407 ) ) ;
#6072=CARTESIAN_POINT ( 'NONE',  ( -4.458734124999997661, -30.47916666530107221, 2.574251347313722516 ) ) ;
#6076=AXIS2_PLACEMENT_3D ( 'NONE', #33000, #47468, #33308 ) ;
#6077=CARTESIAN_POINT ( 'NONE',  ( 4.458734124999998549, 19.27083333469893134, -2.574251347313721627 ) ) ;
#6080=CARTESIAN_POINT ( 'NONE',  ( -2.499999999999996447, -25.70833333060214798, 4.330127018922195425 ) ) ;
#6081=CARTESIAN_POINT ( 'NONE',  ( 2.229367062500001939, -79.22916666530106511, 3.861377020970579999 ) ) ;
#6083=CARTESIAN_POINT ( 'NONE',  ( 5.000000000000000888, 24.54166666939784847, 2.886751345948126879 ) ) ;
#6085=( BOUNDED_CURVE ( )  B_SPLINE_CURVE ( 2, ( #6787, #1656, #16748, #12241, #16110, #55681, #31854, #35736, #36365 ),
 .UNSPECIFIED., .F., .F. ) 
 B_SPLINE_CURVE_WITH_KNOTS ( ( 3, 2, 2, 2, 3 ),
 ( 0.6687499999999999556, 0.6694444444444443976, 0.6708333333333332815, 0.6722222222222222765, 0.6729166666666667185 ),
 .UNSPECIFIED. ) 
 CURVE ( )  GEOMETRIC_REPRESENTATION_ITEM ( )  RATIONAL_B_SPLINE_CURVE ( ( 0.9330127018922194093, 0.9330127018922194093, 1.000000000000000000, 0.8660254037844387076, 1.000000000000000000, 0.8660254037844387076, 1.000000000000000000, 0.9330127018922194093, 0.9330127018922194093 ) ) 
 REPRESENTATION_ITEM ( '' )  );
#6086=CARTESIAN_POINT ( 'NONE',  ( 2.499999999999998668, -0.3333333333333348136, -4.330127018922193649 ) ) ;
#6087=CARTESIAN_POINT ( 'NONE',  ( -3.535250795749689387E-16, -17.25000000000000000, -5.773502691896257311 ) ) ;
#6088=CARTESIAN_POINT ( 'NONE',  ( -2.229367062499996610, -21.14583333196774007, 3.861377020970582219 ) ) ;
#6089=CARTESIAN_POINT ( 'NONE',  ( 2.229367062500001939, -84.97916666530107932, 3.861377020970579999 ) ) ;
#6090=CARTESIAN_POINT ( 'NONE',  ( 2.499999999999998668, -24.20833333060214443, -4.330127018922193649 ) ) ;
#6091=CARTESIAN_POINT ( 'NONE',  ( 2.229367062500001939, -56.97916666530107932, 3.861377020970579999 ) ) ;
#6093=CARTESIAN_POINT ( 'NONE',  ( 5.000000000000000000, -49.41666666666666430, -2.886751345948130876 ) ) ;
#6095=CARTESIAN_POINT ( 'NONE',  ( -4.458734124999999437, -1.645833331967737401, -2.574251347313719407 ) ) ;
#6098=CARTESIAN_POINT ( 'NONE',  ( 1.060575238724906964E-15, -66.75000000000000000, 5.773502691896257311 ) ) ;
#6099=CARTESIAN_POINT ( 'NONE',  ( 3.152801135295367541, -153.5625000013656063, -3.152801135295367541 ) ) ;
#6102=CARTESIAN_POINT ( 'NONE',  ( -3.535533905932738641, -158.3750000000000284, 3.535533905932737309 ) ) ;
#6105=CARTESIAN_POINT ( 'NONE',  ( -4.458734124999999437, -12.56249999863440259, 0.000000000000000000 ) ) ;
#6106=CARTESIAN_POINT ( 'NONE',  ( -2.229367062499996610, -49.39583333196772941, 3.861377020970582219 ) ) ;
#6108=CARTESIAN_POINT ( 'NONE',  ( 1.846868145590735200, -145.2500000013655779, -4.458734125000000326 ) ) ;
#6110=CARTESIAN_POINT ( 'NONE',  ( -1.339745962155623360, 21.33034180399265978, 4.999999999999991118 ) ) ;
#6113=CARTESIAN_POINT ( 'NONE',  ( -4.458734124999999437, 26.35416666803226349, -2.574251347313719407 ) ) ;
#6115=CARTESIAN_POINT ( 'NONE',  ( 1.975475456537005874E-15, -30.74999999999999645, 5.000000000000000000 ) ) ;
#6117=ORIENTED_EDGE ( 'NONE', *, *, #42476, .F. ) ;
#6122=CARTESIAN_POINT ( 'NONE',  ( 1.975475456537005874E-15, 11.37500000273118239, 5.000000000000000000 ) ) ;
#6123=CARTESIAN_POINT ( 'NONE',  ( 4.458734124999998549, -6.729166665301073103, -2.574251347313721627 ) ) ;
#6124=CARTESIAN_POINT ( 'NONE',  ( 2.730187237215162345E-16, -149.1875000013656063, -4.458734124999999437 ) ) ;
#6131=CARTESIAN_POINT ( 'NONE',  ( 5.000000000000000888, -88.45833333060214443, 2.886751345948126879 ) ) ;
#6136=DIRECTION ( 'NONE',  ( 0.000000000000000000, 0.000000000000000000, 1.000000000000000000 ) ) ;
#6138=CARTESIAN_POINT ( 'NONE',  ( -4.458734124999997661, 13.77083333469892779, 2.574251347313722516 ) ) ;
#6140=ORIENTED_EDGE ( 'NONE', *, *, #30712, .T. ) ;
#6141=CARTESIAN_POINT ( 'NONE',  ( 4.458734124999998549, -13.97916666530107221, -2.574251347313721627 ) ) ;
#6143=CARTESIAN_POINT ( 'NONE',  ( 4.458734124999999437, -162.4375000013655779, 0.000000000000000000 ) ) ;
#6150=DIRECTION ( 'NONE',  ( -0.000000000000000000, 1.000000000000000000, -0.000000000000000000 ) ) ;
#6152=CARTESIAN_POINT ( 'NONE',  ( 4.458734124999997661, -148.7500000013656063, 1.846868145590737864 ) ) ;
#6159=CARTESIAN_POINT ( 'NONE',  ( -1.339745962155613812, -9.080341798530296771, -5.000000000000000000 ) ) ;
#6160=CARTESIAN_POINT ( 'NONE',  ( 5.000000000000000000, -1.500000000000001332, -6.123233995736766282E-16 ) ) ;
#6162=CARTESIAN_POINT ( 'NONE',  ( 2.229367062499998831, -67.64583333196773651, -3.861377020970580887 ) ) ;
#6163=CARTESIAN_POINT ( 'NONE',  ( -5.000000000000000000, -8.958333330602146205, -2.886751345948128211 ) ) ;
#6164=CARTESIAN_POINT ( 'NONE',  ( 2.229367062500001939, -35.97916666530107221, 3.861377020970579999 ) ) ;
#6167=DIRECTION ( 'NONE',  ( -0.000000000000000000, 1.000000000000000000, -0.000000000000000000 ) ) ;
#6168=CARTESIAN_POINT ( 'NONE',  ( -4.458734124999999437, 13.43750000136559386, 0.000000000000000000 ) ) ;
#6171=CARTESIAN_POINT ( 'NONE',  ( 5.000000000000000000, -52.41666666666666430, -2.886751345948129988 ) ) ;
#6174=CARTESIAN_POINT ( 'NONE',  ( -4.458734124999999437, -76.31249999863440792, 0.000000000000000000 ) ) ;
#6175=CARTESIAN_POINT ( 'NONE',  ( -3.152801135295367985, -141.0625000013655779, 3.152801135295367096 ) ) ;
#6176=CARTESIAN_POINT ( 'NONE',  ( 4.458734125000001214, -82.89583333196772230, 2.574251347313718519 ) ) ;
#6179=AXIS2_PLACEMENT_3D ( 'NONE', #13849, #9335, #58552 ) ;
#6180=CARTESIAN_POINT ( 'NONE',  ( -4.458734124999999437, -31.56249999863440436, 0.000000000000000000 ) ) ;
#6184=ORIENTED_EDGE ( 'NONE', *, *, #35022, .T. ) ;
#6190=CARTESIAN_POINT ( 'NONE',  ( 4.458734124999998549, -63.97916666530107221, -2.574251347313721627 ) ) ;
#6193=CARTESIAN_POINT ( 'NONE',  ( -1.339745962155613812, 4.919658201469705006, -5.000000000000000000 ) ) ;
#6194=CARTESIAN_POINT ( 'NONE',  ( -4.458734124999999437, 9.604166668032259935, -2.574251347313719407 ) ) ;
#6196=CARTESIAN_POINT ( 'NONE',  ( -1.339745962155613812, -1.205341801261479828, -5.000000000000000000 ) ) ;
#6197=CARTESIAN_POINT ( 'NONE',  ( 1.846868145590736310, -161.6250000013656063, 4.458734124999997661 ) ) ;
#6198=DIRECTION ( 'NONE',  ( -0.000000000000000000, 1.000000000000000000, -0.000000000000000000 ) ) ;
#6201=CARTESIAN_POINT ( 'NONE',  ( 2.071067811865540342, -164.3125000027312410, 4.999999999999936051 ) ) ;
#6203=VECTOR ( 'NONE', #42521, 1000.000000000000000 ) ;
#6204=CARTESIAN_POINT ( 'NONE',  ( 5.000000000000000888, 25.54166666939784847, 2.886751345948126879 ) ) ;
#6205=DIRECTION ( 'NONE',  ( -0.000000000000000000, 1.000000000000000000, -0.000000000000000000 ) ) ;
#6208=CARTESIAN_POINT ( 'NONE',  ( -5.000000000000000000, -28.99999999999999645, 0.000000000000000000 ) ) ;
#6210=CARTESIAN_POINT ( 'NONE',  ( -5.000000000000000000, -82.95833333060214443, -2.886751345948128211 ) ) ;
#6211=CARTESIAN_POINT ( 'NONE',  ( 9.457646018065525792E-16, 26.93750000136559564, 5.148502694627439702 ) ) ;
#6214=CARTESIAN_POINT ( 'NONE',  ( 2.229367062499998831, 1.104166668032261711, -3.861377020970580887 ) ) ;
#6215=CARTESIAN_POINT ( 'NONE',  ( 5.000000000000000000, -151.0625000000000284, 2.071067811865478614 ) ) ;
#6217=CARTESIAN_POINT ( 'NONE',  ( 2.071067811865475505, -144.9375000027311842, -5.000000000000000888 ) ) ;
#6222=LINE ( 'NONE', #40621, #2141 ) ;
#6223=CARTESIAN_POINT ( 'NONE',  ( 2.499999999999998668, 3.666666666666665186, -4.330127018922193649 ) ) ;
#6225=CARTESIAN_POINT ( 'NONE',  ( -3.152801135295367985, -162.0625000013656063, 3.152801135295367096 ) ) ;
#6226=( BOUNDED_CURVE ( )  B_SPLINE_CURVE ( 2, ( #57614, #52776, #14779, #48248, #28319, #44045, #47936, #3889, #12 ),
 .UNSPECIFIED., .F., .F. ) 
 B_SPLINE_CURVE_WITH_KNOTS ( ( 3, 2, 2, 2, 3 ),
 ( 0.05833333333333338283, 0.06250000000000005551, 0.06666666666666672125, 0.07083333333333338699, 0.07500000000000005274 ),
 .UNSPECIFIED. ) 
 CURVE ( )  GEOMETRIC_REPRESENTATION_ITEM ( )  RATIONAL_B_SPLINE_CURVE ( ( 0.9999999999999991118, 0.9238795325112876267, 1.000000000000000000, 0.9238795325112867385, 1.000000000000000000, 0.9238795325112867385, 1.000000000000000000, 0.9238795325112857393, 1.000000000000001110 ) ) 
 REPRESENTATION_ITEM ( '' )  );
#6227=CARTESIAN_POINT ( 'NONE',  ( 1.975475456537005874E-15, -43.75000000000000000, 5.000000000000000000 ) ) ;
#6230=CARTESIAN_POINT ( 'NONE',  ( 1.975475456537005874E-15, -90.62499999726880162, 5.000000000000000000 ) ) ;
#6232=CARTESIAN_POINT ( 'NONE',  ( -4.458734124999998549, 25.52083333469893134, 2.574251347313722516 ) ) ;
#6233=ORIENTED_EDGE ( 'NONE', *, *, #13436, .T. ) ;
#6234=CARTESIAN_POINT ( 'NONE',  ( 9.457646018065525792E-16, -64.31249999863440792, 5.148502694627439702 ) ) ;
#6237=CARTESIAN_POINT ( 'NONE',  ( -6.972266317189433020E-16, -3.124999997268813612, -5.000000000000000000 ) ) ;
#6238=CARTESIAN_POINT ( 'NONE',  ( -5.000000000000000000, 15.91666666666666430, -2.886751345948128211 ) ) ;
#6239=CARTESIAN_POINT ( 'NONE',  ( 4.458734124999999437, -50.81249999863440792, -5.460374474430324690E-16 ) ) ;
#6240=CARTESIAN_POINT ( 'NONE',  ( -4.458734124999999437, -13.39583333196774184, -2.574251347313719407 ) ) ;
#6241=CARTESIAN_POINT ( 'NONE',  ( 1.975475456537005874E-15, -6.749999999999999112, 5.000000000000000000 ) ) ;
#6243=CARTESIAN_POINT ( 'NONE',  ( 1.975475456537005874E-15, -63.74999999999998579, 5.000000000000000000 ) ) ;
#6244=LINE ( 'NONE', #25854, #41211 ) ;
#6245=CARTESIAN_POINT ( 'NONE',  ( 2.499999999999998668, -34.33333333333332860, -4.330127018922193649 ) ) ;
#6246=CARTESIAN_POINT ( 'NONE',  ( 2.500000000000002220, -66.54166666393547303, 4.330127018922192761 ) ) ;
#6247=CARTESIAN_POINT ( 'NONE',  ( -2.500000000000000444, -34.16666666666666430, -4.330127018922193649 ) ) ;
#6249=CARTESIAN_POINT ( 'NONE',  ( -6.972266317189433020E-16, 2.875000002731185500, -5.000000000000000000 ) ) ;
#6250=CARTESIAN_POINT ( 'NONE',  ( 4.458734124999998549, -60.72916666530106511, -2.574251347313721627 ) ) ;
#6251=CARTESIAN_POINT ( 'NONE',  ( -4.458734125000001214, -150.1250000013655779, 1.846868145590734089 ) ) ;
#6253=CARTESIAN_POINT ( 'NONE',  ( 9.457646018065525792E-16, -64.06249999863440792, 5.148502694627439702 ) ) ;
#6255=CARTESIAN_POINT ( 'NONE',  ( -4.999999999999999112, -56.79166666393548013, 2.886751345948131764 ) ) ;
#6258=CARTESIAN_POINT ( 'NONE',  ( -2.229367062499996610, -1.395833331967737179, 3.861377020970582219 ) ) ;
#6259=VERTEX_POINT ( 'NONE', #50138 ) ;
#6260=( BOUNDED_CURVE ( )  B_SPLINE_CURVE ( 2, ( #14284, #4627, #63503, #4952, #34520, #39667, #49332, #38413, #15237 ),
 .UNSPECIFIED., .F., .F. ) 
 B_SPLINE_CURVE_WITH_KNOTS ( ( 3, 2, 2, 2, 3 ),
 ( 0.9937500000000000222, 0.9944444444444444642, 0.9958333333333333481, 0.9972222222222222321, 0.9979166666666666741 ),
 .UNSPECIFIED. ) 
 CURVE ( )  GEOMETRIC_REPRESENTATION_ITEM ( )  RATIONAL_B_SPLINE_CURVE ( ( 0.9330127018922194093, 0.9330127018922194093, 1.000000000000000000, 0.8660254037844387076, 1.000000000000000000, 0.8660254037844387076, 1.000000000000000000, 0.9330127018922194093, 0.9330127018922194093 ) ) 
 REPRESENTATION_ITEM ( '' )  );
#6262=CARTESIAN_POINT ( 'NONE',  ( 1.975475456537005874E-15, -70.62499999726880162, 5.000000000000000000 ) ) ;
#6263=CARTESIAN_POINT ( 'NONE',  ( -4.458734125000000326, -157.0000000013655779, -1.846868145590735644 ) ) ;
#6264=ORIENTED_EDGE ( 'NONE', *, *, #13364, .T. ) ;
#6265=EDGE_CURVE ( 'NONE', #19960, #43823, #45488, .T. ) ;
#6268=CARTESIAN_POINT ( 'NONE',  ( 2.499999999999998668, -80.20833333060213022, -4.330127018922193649 ) ) ;
#6269=CARTESIAN_POINT ( 'NONE',  ( 9.457646018065525792E-16, -50.31249999863440792, 5.148502694627439702 ) ) ;
#6271=CARTESIAN_POINT ( 'NONE',  ( -1.339745962155610925, 17.33034180399266688, 5.000000000000000000 ) ) ;
#6274=CARTESIAN_POINT ( 'NONE',  ( 4.458734125000001214, 23.10416666803225993, 2.574251347313718519 ) ) ;
#6280=FACE_OUTER_BOUND ( 'NONE', #42689, .T. ) ;
#6282=EDGE_CURVE ( 'NONE', #14071, #897, #58635, .T. ) ;
#6283=CARTESIAN_POINT ( 'NONE',  ( -1.339745962155610925, -78.66965819600731891, 5.000000000000000000 ) ) ;
#6284=CARTESIAN_POINT ( 'NONE',  ( 5.000000000000000000, -157.1875000027312126, 2.071067811865478614 ) ) ;
#6288=CARTESIAN_POINT ( 'NONE',  ( -6.972266317189433020E-16, -9.124999997268814056, -5.000000000000000000 ) ) ;
#6292=ORIENTED_EDGE ( 'NONE', *, *, #4725, .F. ) ;
#6295=CARTESIAN_POINT ( 'NONE',  ( 3.535533905932736864, -156.2500000027312126, 3.535533905932738641 ) ) ;
#6302=EDGE_CURVE ( 'NONE', #9342, #5864, #16048, .T. ) ;
#6306=CARTESIAN_POINT ( 'NONE',  ( 2.229367062500001939, -20.97916666530107221, 3.861377020970579999 ) ) ;
#6308=CARTESIAN_POINT ( 'NONE',  ( 3.061616997868383141E-16, -151.7500000000000284, -5.000000000000000000 ) ) ;
#6310=CARTESIAN_POINT ( 'NONE',  ( -3.152801135295367096, -150.0625000013655779, -3.152801135295367541 ) ) ;
#6311=ORIENTED_EDGE ( 'NONE', *, *, #16922, .T. ) ;
#6312=CARTESIAN_POINT ( 'NONE',  ( -4.458734124999999437, -48.56249999863440792, 0.000000000000000000 ) ) ;
#6313=DIRECTION ( 'NONE',  ( -0.000000000000000000, 1.000000000000000000, -0.000000000000000000 ) ) ;
#6315=CARTESIAN_POINT ( 'NONE',  ( 2.499999999999998668, 29.66666666666666430, -4.330127018922193649 ) ) ;
#6316=CARTESIAN_POINT ( 'NONE',  ( 2.229367062499998831, 2.354166668032262599, -3.861377020970580887 ) ) ;
#6318=CARTESIAN_POINT ( 'NONE',  ( 2.499999999999998668, 13.66666666666666785, -4.330127018922193649 ) ) ;
#6320=CARTESIAN_POINT ( 'NONE',  ( -2.229367062499996610, 13.60416666803226171, 3.861377020970582219 ) ) ;
#6322=CARTESIAN_POINT ( 'NONE',  ( 2.499999999999998668, 10.79166666939785202, -4.330127018922193649 ) ) ;
#6327=CARTESIAN_POINT ( 'NONE',  ( 2.229367062499998831, -43.64583333196773651, -3.861377020970580887 ) ) ;
#6328=CARTESIAN_POINT ( 'NONE',  ( 3.152801135295367541, -165.5625000013656063, -3.152801135295367541 ) ) ;
#6329=EDGE_CURVE ( 'NONE', #49174, #48477, #45639, .T. ) ;
#6330=CARTESIAN_POINT ( 'NONE',  ( 2.500000000000002220, -40.54166666393548013, 4.330127018922192761 ) ) ;
#6332=ORIENTED_EDGE ( 'NONE', *, *, #11330, .F. ) ;
#6333=CARTESIAN_POINT ( 'NONE',  ( 2.229367062500001939, -16.97916666530106866, 3.861377020970579999 ) ) ;
#6334=ORIENTED_EDGE ( 'NONE', *, *, #4349, .F. ) ;
#6335=CARTESIAN_POINT ( 'NONE',  ( 2.500000000000002220, -85.66666666666667140, 4.330127018922192761 ) ) ;
#6336=CARTESIAN_POINT ( 'NONE',  ( 4.458734124999999437, -168.4375000013656063, 0.000000000000000000 ) ) ;
#6337=CARTESIAN_POINT ( 'NONE',  ( 2.499999999999998668, -87.20833333060214443, -4.330127018922193649 ) ) ;
#6338=CARTESIAN_POINT ( 'NONE',  ( -6.972266317189433020E-16, -35.12499999726880873, -5.000000000000000000 ) ) ;
#6340=AXIS2_PLACEMENT_3D ( 'NONE', #55896, #51702, #27556 ) ;
#6342=CARTESIAN_POINT ( 'NONE',  ( -4.458734124999998549, -34.47916666530107221, 2.574251347313722516 ) ) ;
#6343=CARTESIAN_POINT ( 'NONE',  ( 1.339745962155612702, -29.29465819873852084, -5.000000000000000000 ) ) ;
#6344=EDGE_CURVE ( 'NONE', #38431, #5304, #1552, .T. ) ;
#6348=EDGE_CURVE ( 'NONE', #49819, #11304, #14663, .T. ) ;
#6350=CARTESIAN_POINT ( 'NONE',  ( 3.061616997868383141E-16, -147.7500000000000284, -5.000000000000000000 ) ) ;
#6354=CARTESIAN_POINT ( 'NONE',  ( -4.458734124999999437, -72.56249999863439371, 0.000000000000000000 ) ) ;
#6357=CARTESIAN_POINT ( 'NONE',  ( 1.846868145590735200, -140.5000000013655779, -4.458734124999999437 ) ) ;
#6358=CARTESIAN_POINT ( 'NONE',  ( -2.499999999999996447, -57.83333333333333570, 4.330127018922195425 ) ) ;
#6360=CARTESIAN_POINT ( 'NONE',  ( -3.152548672688508926E-16, -44.56249999863440081, -5.148502694627439702 ) ) ;
#6361=CARTESIAN_POINT ( 'NONE',  ( -6.972266317189433020E-16, -41.12499999726880162, -5.000000000000000000 ) ) ;
#6363=( BOUNDED_CURVE ( )  B_SPLINE_CURVE ( 2, ( #12659, #7843, #27445, #12017, #3027, #42243, #22643, #60617, #2391 ),
 .UNSPECIFIED., .F., .F. ) 
 B_SPLINE_CURVE_WITH_KNOTS ( ( 3, 2, 2, 2, 3 ),
 ( 0.6416666666666662744, 0.6458333333333329263, 0.6499999999999996891, 0.6541666666666663410, 0.6583333333333329929 ),
 .UNSPECIFIED. ) 
 CURVE ( )  GEOMETRIC_REPRESENTATION_ITEM ( )  RATIONAL_B_SPLINE_CURVE ( ( 1.000000000000008216, 0.9238795325112786339, 1.000000000000000000, 0.9238795325112867385, 1.000000000000000000, 0.9238795325112867385, 1.000000000000000000, 0.9238795325112928447, 0.9999999999999938938 ) ) 
 REPRESENTATION_ITEM ( '' )  );
#6369=CARTESIAN_POINT ( 'NONE',  ( 2.229367062500001939, -72.22916666530107932, 3.861377020970579999 ) ) ;
#6371=CARTESIAN_POINT ( 'NONE',  ( -2.498395430326213474E-14, 14.37500000273118417, 5.000000000000000000 ) ) ;
#6373=ORIENTED_EDGE ( 'NONE', *, *, #40167, .T. ) ;
#6375=CARTESIAN_POINT ( 'NONE',  ( 5.000000000000000000, 23.62500000273118417, -6.123233995736766282E-16 ) ) ;
#6380=CARTESIAN_POINT ( 'NONE',  ( 4.458734125000000326, 16.85416666803225993, 2.574251347313718519 ) ) ;
#6388=CARTESIAN_POINT ( 'NONE',  ( 2.229367062500001939, -87.97916666530107932, 3.861377020970579999 ) ) ;
#6389=CARTESIAN_POINT ( 'NONE',  ( 2.229367062500001939, -3.979166665301070438, 3.861377020970579999 ) ) ;
#6392=CARTESIAN_POINT ( 'NONE',  ( 4.458734125000000326, -29.14583333196774007, 2.574251347313718519 ) ) ;
#6396=CARTESIAN_POINT ( 'NONE',  ( 4.458734124999998549, 18.27083333469893134, -2.574251347313721627 ) ) ;
#6397=DIRECTION ( 'NONE',  ( -0.000000000000000000, 1.000000000000000000, -0.000000000000000000 ) ) ;
#6398=CARTESIAN_POINT ( 'NONE',  ( -6.972266317189433020E-16, -44.12499999726880162, -5.000000000000000000 ) ) ;
#6399=CARTESIAN_POINT ( 'NONE',  ( -2.229367062500000163, -77.72916666530106511, -3.861377020970580443 ) ) ;
#6402=CARTESIAN_POINT ( 'NONE',  ( 5.000000000000000000, 24.62500000273118417, -6.123233995736766282E-16 ) ) ;
#6404=CARTESIAN_POINT ( 'NONE',  ( 1.975475456537005874E-15, -65.74999999999998579, 5.000000000000000000 ) ) ;
#6406=CARTESIAN_POINT ( 'NONE',  ( -2.500000000000000444, -21.16666666666666785, -4.330127018922193649 ) ) ;
#6407=CARTESIAN_POINT ( 'NONE',  ( -4.458734124999999437, -28.31249999863440081, 0.000000000000000000 ) ) ;
#6408=CARTESIAN_POINT ( 'NONE',  ( -4.458734124999999437, -90.31249999863440792, 0.000000000000000000 ) ) ;
#6409=EDGE_CURVE ( 'NONE', #54241, #47490, #21262, .T. ) ;
#6410=CARTESIAN_POINT ( 'NONE',  ( 2.500000000000002220, -23.54166666393548368, 4.330127018922192761 ) ) ;
#6411=CARTESIAN_POINT ( 'NONE',  ( -2.229367062500000163, -55.47916666530107221, -3.861377020970580443 ) ) ;
#6413=CARTESIAN_POINT ( 'NONE',  ( 5.000000000000000888, -65.58333333333332860, 2.886751345948126879 ) ) ;
#6414=CARTESIAN_POINT ( 'NONE',  ( 0.000000000000000000, -170.0000000000000000, 0.000000000000000000 ) ) ;
#6415=AXIS2_PLACEMENT_3D ( 'NONE', #29129, #48752, #18855 ) ;
#6416=CARTESIAN_POINT ( 'NONE',  ( 9.457646018065525792E-16, -1.312499998634405918, 5.148502694627439702 ) ) ;
#6417=ORIENTED_EDGE ( 'NONE', *, *, #28314, .F. ) ;
#6418=CARTESIAN_POINT ( 'NONE',  ( 5.000000000000000000, -66.50000000000000000, -6.123233995736766282E-16 ) ) ;
#6419=CARTESIAN_POINT ( 'NONE',  ( 4.458734124999999437, -151.6875000013656063, 0.000000000000000000 ) ) ;
#6421=CARTESIAN_POINT ( 'NONE',  ( 5.000000000000000000, -157.0625000000000000, 2.071067811865478614 ) ) ;
#6422=CARTESIAN_POINT ( 'NONE',  ( 1.339745962155615144, -10.58034179853029144, 4.999999999999999112 ) ) ;
#6424=CARTESIAN_POINT ( 'NONE',  ( -4.458734124999999437, -18.64583333196774007, -2.574251347313719407 ) ) ;
#6425=CARTESIAN_POINT ( 'NONE',  ( -2.229367062500000163, -53.72916666530107221, -3.861377020970580443 ) ) ;
#6427=CARTESIAN_POINT ( 'NONE',  ( -4.458734124999999437, -142.9375000013656063, -5.460374474430324690E-16 ) ) ;
#6431=EDGE_CURVE ( 'NONE', #45099, #23665, #20510, .T. ) ;
#6433=CARTESIAN_POINT ( 'NONE',  ( -4.458734124999998549, 27.52083333469892779, 2.574251347313722516 ) ) ;
#6435=( BOUNDED_CURVE ( )  B_SPLINE_CURVE ( 2, ( #30058, #46141, #35219, #54839, #55799, #54521, #60634, #25883, #55486 ),
 .UNSPECIFIED., .F., .F. ) 
 B_SPLINE_CURVE_WITH_KNOTS ( ( 3, 2, 2, 2, 3 ),
 ( 0.5395833333333333037, 0.5402777777777777457, 0.5416666666666666297, 0.5430555555555555136, 0.5437499999999999556 ),
 .UNSPECIFIED. ) 
 CURVE ( )  GEOMETRIC_REPRESENTATION_ITEM ( )  RATIONAL_B_SPLINE_CURVE ( ( 0.9330127018922194093, 0.9330127018922194093, 1.000000000000000000, 0.8660254037844387076, 1.000000000000000000, 0.8660254037844387076, 1.000000000000000000, 0.9330127018922194093, 0.9330127018922194093 ) ) 
 REPRESENTATION_ITEM ( '' )  );
#6436=EDGE_CURVE ( 'NONE', #33038, #16025, #845, .T. ) ;
#6443=CARTESIAN_POINT ( 'NONE',  ( 1.339745962155615144, 11.41965820146970501, 4.999999999999999112 ) ) ;
#6444=CARTESIAN_POINT ( 'NONE',  ( -2.229367062499996610, -8.145833331967736513, 3.861377020970582219 ) ) ;
#6446=CARTESIAN_POINT ( 'NONE',  ( -4.458734125000000326, -150.8750000013655779, 1.846868145590734089 ) ) ;
#6449=CARTESIAN_POINT ( 'NONE',  ( 1.975475456537005874E-15, -62.62499999726880873, 5.000000000000000000 ) ) ;
#6453=CARTESIAN_POINT ( 'NONE',  ( -6.972266317189433020E-16, -88.12499999726880162, -5.000000000000000000 ) ) ;
#6458=DIRECTION ( 'NONE',  ( 0.000000000000000000, 0.000000000000000000, 1.000000000000000000 ) ) ;
#6460=CARTESIAN_POINT ( 'NONE',  ( 4.458734125000000326, 14.10416666803226349, 2.574251347313718519 ) ) ;
#6462=CARTESIAN_POINT ( 'NONE',  ( 9.457646018065525792E-16, -15.31249999863440436, 5.148502694627439702 ) ) ;
#6465=CARTESIAN_POINT ( 'NONE',  ( 3.152801135295367541, -162.3125000013656063, -3.152801135295367541 ) ) ;
#6469=CARTESIAN_POINT ( 'NONE',  ( 5.000000000000000888, -38.58333333333332149, 2.886751345948126879 ) ) ;
#6472=CARTESIAN_POINT ( 'NONE',  ( -2.229367062499996610, -37.14583333196773651, 3.861377020970582219 ) ) ;
#6473=DIRECTION ( 'NONE',  ( -0.000000000000000000, 1.000000000000000000, -0.000000000000000000 ) ) ;
#6475=DIRECTION ( 'NONE',  ( -0.000000000000000000, 1.000000000000000000, -0.000000000000000000 ) ) ;
#6481=CARTESIAN_POINT ( 'NONE',  ( 1.060575238724906964E-15, -7.749999999999999112, 5.773502691896257311 ) ) ;
#6482=CARTESIAN_POINT ( 'NONE',  ( 2.229367062500001939, -71.97916666530107932, 3.861377020970579999 ) ) ;
#6483=CARTESIAN_POINT ( 'NONE',  ( 2.500000000000002220, -22.54166666393548013, 4.330127018922192761 ) ) ;
#6484=CARTESIAN_POINT ( 'NONE',  ( -2.499999999999996447, -7.708333330602144429, 4.330127018922195425 ) ) ;
#6485=CARTESIAN_POINT ( 'NONE',  ( 4.458734124999998549, -39.72916666530107932, -2.574251347313721627 ) ) ;
#6488=CARTESIAN_POINT ( 'NONE',  ( 9.457646018065525792E-16, 11.68750000136559564, 5.148502694627439702 ) ) ;
#6489=ORIENTED_EDGE ( 'NONE', *, *, #19267, .T. ) ;
#6491=CARTESIAN_POINT ( 'NONE',  ( -4.999999999999999112, -47.91666666666667140, 2.886751345948131764 ) ) ;
#6494=CARTESIAN_POINT ( 'NONE',  ( -4.458734124999998549, -73.22916666530106511, 2.574251347313722516 ) ) ;
#6495=CARTESIAN_POINT ( 'NONE',  ( 4.458734124999999437, -140.6875000013656063, 0.000000000000000000 ) ) ;
#6496=CARTESIAN_POINT ( 'NONE',  ( -2.229367062499996610, -86.14583333196773651, 3.861377020970582219 ) ) ;
#6498=CARTESIAN_POINT ( 'NONE',  ( 2.229367062500001939, -37.22916666530107221, 3.861377020970579999 ) ) ;
#6504=ORIENTED_EDGE ( 'NONE', *, *, #27461, .T. ) ;
#6506=DIRECTION ( 'NONE',  ( 0.000000000000000000, 1.000000000000000000, 0.000000000000000000 ) ) ;
#6507=CARTESIAN_POINT ( 'NONE',  ( 4.458734124999999437, -62.06249999863440792, -5.460374474430324690E-16 ) ) ;
#6514=CARTESIAN_POINT ( 'NONE',  ( 2.229367062499998831, 6.354166668032262599, -3.861377020970580887 ) ) ;
#6515=CARTESIAN_POINT ( 'NONE',  ( -2.500000000000000444, -76.16666666666665719, -4.330127018922193649 ) ) ;
#6516=CARTESIAN_POINT ( 'NONE',  ( -1.846868145590734756, -159.1250000013656063, -4.458734124999999437 ) ) ;
#6517=DIRECTION ( 'NONE',  ( 0.000000000000000000, 0.000000000000000000, 1.000000000000000000 ) ) ;
#6518=ORIENTED_EDGE ( 'NONE', *, *, #58551, .F. ) ;
#6520=CARTESIAN_POINT ( 'NONE',  ( -9.184850993605147944E-16, -164.3750000027311842, 5.000000000000000000 ) ) ;
#6522=CARTESIAN_POINT ( 'NONE',  ( -4.764381983412779477E-15, 25.37500000273118062, 5.000000000000000000 ) ) ;
#6523=CARTESIAN_POINT ( 'NONE',  ( -2.499999999999996447, -67.83333333333332860, 4.330127018922195425 ) ) ;
#6529=CARTESIAN_POINT ( 'NONE',  ( -3.152548672688508926E-16, 3.187500001365594304, -5.148502694627439702 ) ) ;
#6532=CARTESIAN_POINT ( 'NONE',  ( -5.000000000000000888, -146.5625000027311842, 2.071067811865474617 ) ) ;
#6533=CARTESIAN_POINT ( 'NONE',  ( 5.000000000000000000, -33.29166666393547303, -2.886751345948130876 ) ) ;
#6537=VECTOR ( 'NONE', #21294, 1000.000000000000000 ) ;
#6538=DIRECTION ( 'NONE',  ( 0.000000000000000000, 0.000000000000000000, 1.000000000000000000 ) ) ;
#6541=CARTESIAN_POINT ( 'NONE',  ( -4.458734125000000326, -161.1250000013656063, 1.846868145590734089 ) ) ;
#6543=CARTESIAN_POINT ( 'NONE',  ( 1.975475456537005874E-15, -26.74999999999999645, 5.000000000000000000 ) ) ;
#6544=VERTEX_POINT ( 'NONE', #10149 ) ;
#6545=CARTESIAN_POINT ( 'NONE',  ( 2.229367062499998831, 23.10416666803225993, -3.861377020970580887 ) ) ;
#6546=ORIENTED_EDGE ( 'NONE', *, *, #54313, .F. ) ;
#6550=CARTESIAN_POINT ( 'NONE',  ( -4.999999999999999112, 14.08333333333333393, 2.886751345948131764 ) ) ;
#6551=CARTESIAN_POINT ( 'NONE',  ( -4.458734124999999437, -58.31249999863440081, 0.000000000000000000 ) ) ;
#6552=CARTESIAN_POINT ( 'NONE',  ( -4.458734124999999437, -9.395833331967736513, -2.574251347313719407 ) ) ;
#6553=( BOUNDED_CURVE ( )  B_SPLINE_CURVE ( 2, ( #18693, #4848, #23843, #19318, #3603, #62466, #14489, #23210, #57947 ),
 .UNSPECIFIED., .F., .F. ) 
 B_SPLINE_CURVE_WITH_KNOTS ( ( 3, 2, 2, 2, 3 ),
 ( 0.7770833333333333481, 0.7777777777777777901, 0.7791666666666666741, 0.7805555555555555580, 0.7812500000000000000 ),
 .UNSPECIFIED. ) 
 CURVE ( )  GEOMETRIC_REPRESENTATION_ITEM ( )  RATIONAL_B_SPLINE_CURVE ( ( 0.9330127018922194093, 0.9330127018922194093, 1.000000000000000000, 0.8660254037844387076, 1.000000000000000000, 0.8660254037844387076, 1.000000000000000000, 0.9330127018922194093, 0.9330127018922194093 ) ) 
 REPRESENTATION_ITEM ( '' )  );
#6557=CARTESIAN_POINT ( 'NONE',  ( 0.000000000000000000, -170.0000000000000000, 5.000000000000000000 ) ) ;
#6558=CARTESIAN_POINT ( 'NONE',  ( -2.500000000000000444, -36.16666666666666430, -4.330127018922193649 ) ) ;
#6559=CARTESIAN_POINT ( 'NONE',  ( 0.000000000000000000, -170.0000000000000000, 0.000000000000000000 ) ) ;
#6560=CARTESIAN_POINT ( 'NONE',  ( -4.999999999999998224, -58.91666666666665009, 2.886751345948131764 ) ) ;
#6563=CARTESIAN_POINT ( 'NONE',  ( -2.229367062500000163, -58.47916666530106511, -3.861377020970580443 ) ) ;
#6564=CARTESIAN_POINT ( 'NONE',  ( -8.190561711645485556E-16, -152.9375000013655779, 4.458734124999999437 ) ) ;
#6565=CARTESIAN_POINT ( 'NONE',  ( -4.458734124999999437, -67.31249999863440792, 0.000000000000000000 ) ) ;
#6567=CARTESIAN_POINT ( 'NONE',  ( -5.000000000000000000, -57.95833333060215153, -2.886751345948128211 ) ) ;
#6568=VECTOR ( 'NONE', #5169, 1000.000000000000000 ) ;
#6571=VERTEX_POINT ( 'NONE', #40047 ) ;
#6574=CARTESIAN_POINT ( 'NONE',  ( -4.458734125000001214, -151.8750000013655779, 1.846868145590734089 ) ) ;
#6576=CARTESIAN_POINT ( 'NONE',  ( 0.000000000000000000, -170.0000000000000000, 0.000000000000000000 ) ) ;
#6579=CARTESIAN_POINT ( 'NONE',  ( -3.152548672688508926E-16, -49.81249999863440081, -5.148502694627439702 ) ) ;
#6580=ORIENTED_EDGE ( 'NONE', *, *, #62460, .T. ) ;
#6583=CARTESIAN_POINT ( 'NONE',  ( 4.458734124999998549, 22.27083333469893134, -2.574251347313721627 ) ) ;
#6586=CARTESIAN_POINT ( 'NONE',  ( 5.275681513340003914E-14, 10.74999999999999645, -5.000000000000000000 ) ) ;
#6587=EDGE_LOOP ( 'NONE', ( #2879, #11073, #18018, #13981 ) ) ;
#6591=CARTESIAN_POINT ( 'NONE',  ( 5.000000000000000000, -63.41666666666666430, -2.886751345948130876 ) ) ;
#6592=CARTESIAN_POINT ( 'NONE',  ( -3.535533905932737309, -157.6250000000000284, -3.535533905932738197 ) ) ;
#6596=CARTESIAN_POINT ( 'NONE',  ( -2.500000000000000444, -20.04166666393548013, -4.330127018922193649 ) ) ;
#6600=( BOUNDED_CURVE ( )  B_SPLINE_CURVE ( 2, ( #49563, #25117, #44728, #20944, #2291, #21578, #46649, #36051, #31214 ),
 .UNSPECIFIED., .F., .F. ) 
 B_SPLINE_CURVE_WITH_KNOTS ( ( 3, 2, 2, 2, 3 ),
 ( 0.9812499999999999556, 0.9819444444444443976, 0.9833333333333332815, 0.9847222222222222765, 0.9854166666666667185 ),
 .UNSPECIFIED. ) 
 CURVE ( )  GEOMETRIC_REPRESENTATION_ITEM ( )  RATIONAL_B_SPLINE_CURVE ( ( 0.9330127018922194093, 0.9330127018922194093, 1.000000000000000000, 0.8660254037844387076, 1.000000000000000000, 0.8660254037844387076, 1.000000000000000000, 0.9330127018922194093, 0.9330127018922194093 ) ) 
 REPRESENTATION_ITEM ( '' )  );
#6604=CARTESIAN_POINT ( 'NONE',  ( 5.000000000000000000, -158.1250000027311842, 0.000000000000000000 ) ) ;
#6615=CARTESIAN_POINT ( 'NONE',  ( 9.457646018065525792E-16, -17.06249999863440792, 5.148502694627439702 ) ) ;
#6617=CARTESIAN_POINT ( 'NONE',  ( 2.071067811865475505, -150.8125000000000000, -5.000000000000000888 ) ) ;
#6619=CARTESIAN_POINT ( 'NONE',  ( 3.152801135295367541, -152.3125000013655779, -3.152801135295367541 ) ) ;
#6621=CARTESIAN_POINT ( 'NONE',  ( -4.458734124999997661, -46.47916666530106511, 2.574251347313722516 ) ) ;
#6623=CYLINDRICAL_SURFACE ( 'NONE', #62727, 5.000000000000000000 ) ;
#6624=CARTESIAN_POINT ( 'NONE',  ( 5.000000000000000888, 27.41666666666666785, 2.886751345948126879 ) ) ;
#6626=CARTESIAN_POINT ( 'NONE',  ( -3.152548672688508926E-16, 4.437500001365595637, -5.148502694627439702 ) ) ;
#6628=CARTESIAN_POINT ( 'NONE',  ( -9.184850993605147944E-16, -142.2500000000000284, 5.000000000000000000 ) ) ;
#6630=CARTESIAN_POINT ( 'NONE',  ( 1.975475456537005874E-15, -11.62499999726881406, 5.000000000000000000 ) ) ;
#6632=CARTESIAN_POINT ( 'NONE',  ( -2.229367062499996610, 17.60416666803225993, 3.861377020970582219 ) ) ;
#6634=CARTESIAN_POINT ( 'NONE',  ( 5.000000000000000000, 4.708333336064518093, -2.886751345948129988 ) ) ;
#6636=CARTESIAN_POINT ( 'NONE',  ( 5.000000000000000000, -162.1250000027311842, 0.000000000000000000 ) ) ;
#6638=CARTESIAN_POINT ( 'NONE',  ( 2.788906526875773208E-15, 27.87500000273118417, -5.000000000000000000 ) ) ;
#6639=CARTESIAN_POINT ( 'NONE',  ( -4.458734124999999437, -43.31249999863440081, 0.000000000000000000 ) ) ;
#6640=CARTESIAN_POINT ( 'NONE',  ( -1.846868145590734756, -162.3750000013655779, -4.458734125000000326 ) ) ;
#6641=EDGE_CURVE ( 'NONE', #51343, #59835, #22586, .T. ) ;
#6642=CARTESIAN_POINT ( 'NONE',  ( -5.000000000000000000, -36.95833333060213732, -2.886751345948128211 ) ) ;
#6643=ORIENTED_EDGE ( 'NONE', *, *, #9778, .T. ) ;
#6644=CARTESIAN_POINT ( 'NONE',  ( -4.458734124999999437, -18.39583333196774007, -2.574251347313719407 ) ) ;
#6645=ORIENTED_EDGE ( 'NONE', *, *, #33048, .F. ) ;
#6646=CARTESIAN_POINT ( 'NONE',  ( -2.499999999999996447, -88.83333333333332860, 4.330127018922195425 ) ) ;
#6647=CARTESIAN_POINT ( 'NONE',  ( -4.458734125000001214, -162.8750000013655779, 1.846868145590734089 ) ) ;
#6649=CARTESIAN_POINT ( 'NONE',  ( 5.000000000000000000, -87.37499999726880162, -6.123233995736766282E-16 ) ) ;
#6653=CARTESIAN_POINT ( 'NONE',  ( -3.152548672688508926E-16, -32.81249999863440792, -5.148502694627439702 ) ) ;
#6654=CARTESIAN_POINT ( 'NONE',  ( 1.339745962155615144, -29.70534180126147561, 4.999999999999999112 ) ) ;
#6656=ADVANCED_FACE ( 'NONE', ( #39635 ), #33873, .T. ) ;
#6660=ORIENTED_EDGE ( 'NONE', *, *, #32321, .T. ) ;
#6661=CARTESIAN_POINT ( 'NONE',  ( -5.000000000000000888, -161.5625000000000284, -2.071067811865475949 ) ) ;
#6663=CARTESIAN_POINT ( 'NONE',  ( 4.458734124999998549, -82.97916666530107932, -2.574251347313721627 ) ) ;
#6666=CARTESIAN_POINT ( 'NONE',  ( -4.458734125000000326, -144.1250000013655779, 1.846868145590734089 ) ) ;
#6667=CARTESIAN_POINT ( 'NONE',  ( -2.500000000000000444, 5.958333336064519870, -4.330127018922193649 ) ) ;
#6669=CARTESIAN_POINT ( 'NONE',  ( 9.457646018065525792E-16, -45.06249999863440081, 5.148502694627439702 ) ) ;
#6672=VECTOR ( 'NONE', #33074, 1000.000000000000000 ) ;
#6673=DIRECTION ( 'NONE',  ( 0.000000000000000000, 0.000000000000000000, 1.000000000000000000 ) ) ;
#6678=CARTESIAN_POINT ( 'NONE',  ( -4.458734124999999437, -80.64583333196773651, -2.574251347313719407 ) ) ;
#6681=CARTESIAN_POINT ( 'NONE',  ( 1.339745962155612702, -76.29465819873853150, -5.000000000000000000 ) ) ;
#6685=CARTESIAN_POINT ( 'NONE',  ( -1.339745962155610925, -59.79465819873851729, 5.000000000000000000 ) ) ;
#6687=CARTESIAN_POINT ( 'NONE',  ( 5.000000000000000000, -168.1875000027311842, 2.071067811865478614 ) ) ;
#6689=EDGE_CURVE ( 'NONE', #23665, #34156, #18438, .T. ) ;
#6690=CARTESIAN_POINT ( 'NONE',  ( 2.229367062499998831, 13.10416666803226171, -3.861377020970580887 ) ) ;
#6691=DIRECTION ( 'NONE',  ( -0.000000000000000000, 1.000000000000000000, -0.000000000000000000 ) ) ;
#6697=CARTESIAN_POINT ( 'NONE',  ( -9.184850993605147944E-16, -163.2500000000000000, 5.000000000000000000 ) ) ;
#6698=CARTESIAN_POINT ( 'NONE',  ( -4.458734124999998549, -86.22916666530106511, 2.574251347313722516 ) ) ;
#6699=CARTESIAN_POINT ( 'NONE',  ( -3.152548672688508926E-16, -4.562499998634401699, -5.148502694627439702 ) ) ;
#6702=CARTESIAN_POINT ( 'NONE',  ( -2.229367062500000163, -32.72916666530106511, -3.861377020970580443 ) ) ;
#6706=CARTESIAN_POINT ( 'NONE',  ( -2.229367062500000163, 19.52083333469893134, -3.861377020970580443 ) ) ;
#6708=EDGE_CURVE ( 'NONE', #12164, #37331, #57892, .T. ) ;
#6709=CARTESIAN_POINT ( 'NONE',  ( 1.339745962155615144, -28.70534180126147561, 4.999999999999999112 ) ) ;
#6710=CARTESIAN_POINT ( 'NONE',  ( 4.458734125000000326, -80.14583333196773651, 2.574251347313718519 ) ) ;
#6713=CARTESIAN_POINT ( 'NONE',  ( 2.500000000000002220, 25.45833333606451987, 4.330127018922192761 ) ) ;
#6714=ORIENTED_EDGE ( 'NONE', *, *, #31089, .F. ) ;
#6717=CARTESIAN_POINT ( 'NONE',  ( 2.500000000000002220, -25.66666666666666430, 4.330127018922192761 ) ) ;
#6718=CARTESIAN_POINT ( 'NONE',  ( -2.229367062499996610, -26.14583333196773651, 3.861377020970582219 ) ) ;
#6719=CARTESIAN_POINT ( 'NONE',  ( 2.229367062499998831, -88.64583333196773651, -3.861377020970580887 ) ) ;
#6720=AXIS2_PLACEMENT_3D ( 'NONE', #6576, #55787, #30697 ) ;
#6721=CARTESIAN_POINT ( 'NONE',  ( -2.500000000000000444, -23.04166666393548013, -4.330127018922193649 ) ) ;
#6722=CARTESIAN_POINT ( 'NONE',  ( -2.229367062499996610, -57.14583333196773651, 3.861377020970582219 ) ) ;
#6724=CARTESIAN_POINT ( 'NONE',  ( 1.339745962155661996, -27.29465819873851729, -4.999999999999970690 ) ) ;
#6725=DIRECTION ( 'NONE',  ( -0.000000000000000000, 1.000000000000000000, -0.000000000000000000 ) ) ;
#6726=CARTESIAN_POINT ( 'NONE',  ( -4.458734124999999437, -3.645833331967739621, -2.574251347313719407 ) ) ;
#6728=CARTESIAN_POINT ( 'NONE',  ( -2.500000000000000444, -70.16666666666667140, -4.330127018922193649 ) ) ;
#6729=CARTESIAN_POINT ( 'NONE',  ( -3.152801135295367096, -153.3125000013656063, -3.152801135295367541 ) ) ;
#6731=LINE ( 'NONE', #58055, #10135 ) ;
#6732=CARTESIAN_POINT ( 'NONE',  ( 3.061616997868383141E-16, -158.7500000000000000, -5.000000000000000000 ) ) ;
#6733=CARTESIAN_POINT ( 'NONE',  ( 5.000000000000000000, -72.29166666393547303, -2.886751345948129988 ) ) ;
#6734=CARTESIAN_POINT ( 'NONE',  ( 2.500000000000002220, -10.54166666393547835, 4.330127018922192761 ) ) ;
#6736=CARTESIAN_POINT ( 'NONE',  ( -3.152548672688508926E-16, -15.81249999863440436, -5.148502694627439702 ) ) ;
#6737=CARTESIAN_POINT ( 'NONE',  ( 9.457646018065525792E-16, -49.31249999863441502, 5.148502694627439702 ) ) ;
#6738=( BOUNDED_CURVE ( )  B_SPLINE_CURVE ( 2, ( #2014, #27696, #21617, #41210, #22252, #42802, #3582, #18982, #4510 ),
 .UNSPECIFIED., .F., .F. ) 
 B_SPLINE_CURVE_WITH_KNOTS ( ( 3, 2, 2, 2, 3 ),
 ( 0.3395833333333333481, 0.3402777777777777901, 0.3416666666666666741, 0.3430555555555555580, 0.3437500000000000000 ),
 .UNSPECIFIED. ) 
 CURVE ( )  GEOMETRIC_REPRESENTATION_ITEM ( )  RATIONAL_B_SPLINE_CURVE ( ( 0.9330127018922194093, 0.9330127018922194093, 1.000000000000000000, 0.8660254037844387076, 1.000000000000000000, 0.8660254037844387076, 1.000000000000000000, 0.9330127018922194093, 0.9330127018922194093 ) ) 
 REPRESENTATION_ITEM ( '' )  );
#6739=CARTESIAN_POINT ( 'NONE',  ( 2.500000000000002220, 10.33333333333333393, 4.330127018922192761 ) ) ;
#6740=CARTESIAN_POINT ( 'NONE',  ( 3.152801135295367541, -144.3125000013655779, -3.152801135295367541 ) ) ;
#6742=CARTESIAN_POINT ( 'NONE',  ( 5.000000000000000000, -158.0625000000000284, 2.071067811865478614 ) ) ;
#6743=ORIENTED_EDGE ( 'NONE', *, *, #28771, .F. ) ;
#6745=CARTESIAN_POINT ( 'NONE',  ( 4.458734125000001214, 26.85416666803225993, 2.574251347313718519 ) ) ;
#6751=CARTESIAN_POINT ( 'NONE',  ( 4.458734125000001214, -63.14583333196774362, 2.574251347313718519 ) ) ;
#6753=CARTESIAN_POINT ( 'NONE',  ( 9.457646018065525792E-16, -9.062499998634406140, 5.148502694627439702 ) ) ;
#6755=CARTESIAN_POINT ( 'NONE',  ( 2.730187237215162345E-16, -144.1875000013656063, -4.458734124999999437 ) ) ;
#6767=EDGE_CURVE ( 'NONE', #61101, #6968, #11482, .T. ) ;
#6771=CARTESIAN_POINT ( 'NONE',  ( 1.975475456537005874E-15, -3.750000000000001776, 5.000000000000000000 ) ) ;
#6772=CARTESIAN_POINT ( 'NONE',  ( 1.975475456537005874E-15, -14.74999999999999822, 5.000000000000000000 ) ) ;
#6773=EDGE_CURVE ( 'NONE', #53481, #48999, #58010, .T. ) ;
#6774=CARTESIAN_POINT ( 'NONE',  ( -3.152548672688508926E-16, 14.43750000136559386, -5.148502694627439702 ) ) ;
#6776=CARTESIAN_POINT ( 'NONE',  ( -4.458734124999999437, -13.56249999863440259, 0.000000000000000000 ) ) ;
#6779=CARTESIAN_POINT ( 'NONE',  ( 3.152801135295367541, -163.3125000013656063, -3.152801135295367541 ) ) ;
#6782=EDGE_CURVE ( 'NONE', #10271, #5022, #29113, .T. ) ;
#6783=ADVANCED_FACE ( 'NONE', ( #5560 ), #39957, .T. ) ;
#6784=CARTESIAN_POINT ( 'NONE',  ( -5.000000000000000000, 9.916666666666667851, -2.886751345948128211 ) ) ;
#6786=CARTESIAN_POINT ( 'NONE',  ( -4.458734124999999437, -36.31249999863440792, 0.000000000000000000 ) ) ;
#6787=CARTESIAN_POINT ( 'NONE',  ( -6.972266317189433020E-16, -51.12499999726880873, -5.000000000000000000 ) ) ;
#6790=EDGE_CURVE ( 'NONE', #37182, #733, #9406, .T. ) ;
#6791=CYLINDRICAL_SURFACE ( 'NONE', #40716, 5.000000000000000000 ) ;
#6796=ADVANCED_FACE ( 'NONE', ( #2902 ), #40602, .T. ) ;
#6797=CARTESIAN_POINT ( 'NONE',  ( 2.499999999999998668, -5.333333333333335702, -4.330127018922193649 ) ) ;
#6798=ADVANCED_FACE ( 'NONE', ( #20684 ), #30310, .T. ) ;
#6799=CARTESIAN_POINT ( 'NONE',  ( 2.229367062499998831, -72.64583333196773651, -3.861377020970580887 ) ) ;
#6801=CARTESIAN_POINT ( 'NONE',  ( -2.500000000000000444, -5.041666663935480130, -4.330127018922193649 ) ) ;
#6802=CARTESIAN_POINT ( 'NONE',  ( -2.229367062499996610, -37.14583333196773651, 3.861377020970582219 ) ) ;
#6803=ORIENTED_EDGE ( 'NONE', *, *, #28742, .F. ) ;
#6805=CARTESIAN_POINT ( 'NONE',  ( -4.458734124999999437, 10.35416666803225816, -2.574251347313719407 ) ) ;
#6806=ORIENTED_EDGE ( 'NONE', *, *, #30575, .T. ) ;
#6808=CARTESIAN_POINT ( 'NONE',  ( -2.500000000000000444, -54.16666666666667140, -4.330127018922193649 ) ) ;
#6810=CARTESIAN_POINT ( 'NONE',  ( -6.972266317189433020E-16, -60.24999999999999289, -5.000000000000000000 ) ) ;
#6811=CARTESIAN_POINT ( 'NONE',  ( 9.457646018065525792E-16, -78.06249999863440792, 5.148502694627439702 ) ) ;
#6812=( BOUNDED_CURVE ( )  B_SPLINE_CURVE ( 2, ( #32319, #4008, #7889, #3698, #13652, #38102, #23629, #63177, #33272 ),
 .UNSPECIFIED., .F., .F. ) 
 B_SPLINE_CURVE_WITH_KNOTS ( ( 3, 2, 2, 2, 3 ),
 ( 0.7062500000000000444, 0.7069444444444444864, 0.7083333333333333703, 0.7097222222222222543, 0.7104166666666666963 ),
 .UNSPECIFIED. ) 
 CURVE ( )  GEOMETRIC_REPRESENTATION_ITEM ( )  RATIONAL_B_SPLINE_CURVE ( ( 0.9330127018922194093, 0.9330127018922194093, 1.000000000000000000, 0.8660254037844387076, 1.000000000000000000, 0.8660254037844387076, 1.000000000000000000, 0.9330127018922194093, 0.9330127018922194093 ) ) 
 REPRESENTATION_ITEM ( '' )  );
#6813=AXIS2_PLACEMENT_3D ( 'NONE', #52280, #23014, #13033 ) ;
#6814=CARTESIAN_POINT ( 'NONE',  ( 2.071067811865475505, -168.8125000000000000, -5.000000000000000888 ) ) ;
#6815=CARTESIAN_POINT ( 'NONE',  ( -4.458734124999999437, -87.31249999863439371, 0.000000000000000000 ) ) ;
#6817=CIRCLE ( 'NONE', #53030, 5.000000000000000000 ) ;
#6818=CARTESIAN_POINT ( 'NONE',  ( 4.458734124999999437, -35.06249999863440792, -5.460374474430324690E-16 ) ) ;
#6819=CARTESIAN_POINT ( 'NONE',  ( 1.975475456537005874E-15, -74.62499999726880162, 5.000000000000000000 ) ) ;
#6823=ORIENTED_EDGE ( 'NONE', *, *, #7951, .T. ) ;
#6825=CARTESIAN_POINT ( 'NONE',  ( -1.049326080737009628E-13, -18.62499999726881583, 5.000000000000000000 ) ) ;
#6826=CARTESIAN_POINT ( 'NONE',  ( -4.458734124999999437, -63.64583333196773651, -2.574251347313719407 ) ) ;
#6828=ORIENTED_EDGE ( 'NONE', *, *, #27140, .T. ) ;
#6831=ORIENTED_EDGE ( 'NONE', *, *, #11412, .F. ) ;
#6833=CARTESIAN_POINT ( 'NONE',  ( -4.458734124999999437, 5.687500001365592972, 0.000000000000000000 ) ) ;
#6834=CARTESIAN_POINT ( 'NONE',  ( -5.000000000000000000, -32.95833333060215153, -2.886751345948128211 ) ) ;
#6835=CARTESIAN_POINT ( 'NONE',  ( 4.458734124999999437, -160.4375000013655779, 0.000000000000000000 ) ) ;
#6836=( BOUNDED_CURVE ( )  B_SPLINE_CURVE ( 2, ( #50726, #7630, #17266, #41382, #41696, #56837, #36891, #51050, #56520 ),
 .UNSPECIFIED., .F., .F. ) 
 B_SPLINE_CURVE_WITH_KNOTS ( ( 3, 2, 2, 2, 3 ),
 ( 0.07291666666666667129, 0.07361111111111111327, 0.07499999999999999722, 0.07638888888888889506, 0.07708333333333333703 ),
 .UNSPECIFIED. ) 
 CURVE ( )  GEOMETRIC_REPRESENTATION_ITEM ( )  RATIONAL_B_SPLINE_CURVE ( ( 0.9330127018922194093, 0.9330127018922200755, 1.000000000000000000, 0.8660254037844387076, 1.000000000000000000, 0.8660254037844387076, 1.000000000000000000, 0.9330127018922194093, 0.9330127018922194093 ) ) 
 REPRESENTATION_ITEM ( '' )  );
#6837=DIRECTION ( 'NONE',  ( 0.000000000000000000, 0.000000000000000000, 1.000000000000000000 ) ) ;
#6838=ORIENTED_EDGE ( 'NONE', *, *, #22536, .T. ) ;
#6840=CARTESIAN_POINT ( 'NONE',  ( 1.975475456537005874E-15, -31.62499999726880873, 5.000000000000000000 ) ) ;
#6843=DIRECTION ( 'NONE',  ( 0.000000000000000000, 0.000000000000000000, 1.000000000000000000 ) ) ;
#6846=CARTESIAN_POINT ( 'NONE',  ( -2.229367062500000163, 29.52083333469892779, -3.861377020970580443 ) ) ;
#6849=CARTESIAN_POINT ( 'NONE',  ( 4.458734124999999437, -0.06249999863440491854, -5.460374474430324690E-16 ) ) ;
#6852=CARTESIAN_POINT ( 'NONE',  ( -2.071067811865475061, -144.8125000027312410, -5.000000000000000888 ) ) ;
#6853=CARTESIAN_POINT ( 'NONE',  ( 0.000000000000000000, -170.0000000000000000, 0.000000000000000000 ) ) ;
#6858=CARTESIAN_POINT ( 'NONE',  ( -4.999999999999998224, -86.91666666666667140, 2.886751345948131764 ) ) ;
#6861=CARTESIAN_POINT ( 'NONE',  ( -4.458734124999999437, -162.1875000013655779, -5.460374474430324690E-16 ) ) ;
#6862=CARTESIAN_POINT ( 'NONE',  ( -3.535533905932737309, -159.7500000027312126, -3.535533905932738197 ) ) ;
#6864=CARTESIAN_POINT ( 'NONE',  ( -4.458734125000001214, -140.8750000013656063, 1.846868145590734089 ) ) ;
#6865=ORIENTED_EDGE ( 'NONE', *, *, #49530, .F. ) ;
#6866=CARTESIAN_POINT ( 'NONE',  ( 4.458734124999999437, 22.93750000136559564, -5.460374474430324690E-16 ) ) ;
#6872=CARTESIAN_POINT ( 'NONE',  ( -2.499999999999996447, 10.16666666666666785, 4.330127018922195425 ) ) ;
#6873=CARTESIAN_POINT ( 'NONE',  ( -4.458734124999997661, -55.22916666530107932, 2.574251347313722516 ) ) ;
#6874=CARTESIAN_POINT ( 'NONE',  ( 9.457646018065525792E-16, -14.06249999863440259, 5.148502694627439702 ) ) ;
#6875=CARTESIAN_POINT ( 'NONE',  ( 5.000000000000000000, -6.499999999999999112, -6.123233995736766282E-16 ) ) ;
#6878=CARTESIAN_POINT ( 'NONE',  ( -2.499999999999996447, 14.16666666666666785, 4.330127018922195425 ) ) ;
#6881=CARTESIAN_POINT ( 'NONE',  ( 1.060575238724906964E-15, -38.74999999999998579, 5.773502691896257311 ) ) ;
#6882=CARTESIAN_POINT ( 'NONE',  ( 3.535533905932738197, -148.8750000000000000, -3.535533905932738197 ) ) ;
#6885=CARTESIAN_POINT ( 'NONE',  ( 6.123233995736766282E-16, -170.0000000000000000, -5.000000000000000000 ) ) ;
#6886=CARTESIAN_POINT ( 'NONE',  ( -4.458734124999999437, -60.39583333196773651, -2.574251347313719407 ) ) ;
#6887=CARTESIAN_POINT ( 'NONE',  ( 4.458734124999999437, -152.7500000013656063, 1.846868145590737864 ) ) ;
#6888=CARTESIAN_POINT ( 'NONE',  ( -2.229367062499996610, -71.14583333196773651, 3.861377020970582219 ) ) ;
#6890=CARTESIAN_POINT ( 'NONE',  ( 2.229367062499998831, -18.89583333196774007, -3.861377020970580887 ) ) ;
#6891=CARTESIAN_POINT ( 'NONE',  ( 5.000000000000000000, -60.37499999726880873, -6.123233995736766282E-16 ) ) ;
#6893=DIRECTION ( 'NONE',  ( -0.000000000000000000, 1.000000000000000000, -0.000000000000000000 ) ) ;
#6897=CARTESIAN_POINT ( 'NONE',  ( 3.152801135295366208, -152.5625000013655779, 3.152801135295367985 ) ) ;
#6903=CARTESIAN_POINT ( 'NONE',  ( -4.458734124999999437, -48.64583333196773651, -2.574251347313719407 ) ) ;
#6905=EDGE_LOOP ( 'NONE', ( #29170, #59405, #17218, #45973 ) ) ;
#6906=VECTOR ( 'NONE', #29987, 1000.000000000000000 ) ;
#6909=CARTESIAN_POINT ( 'NONE',  ( 2.229367062500001939, 23.02083333469892423, 3.861377020970579999 ) ) ;
#6918=CARTESIAN_POINT ( 'NONE',  ( 1.975475456537005874E-15, -31.75000000000000000, 5.000000000000000000 ) ) ;
#6923=CARTESIAN_POINT ( 'NONE',  ( 1.975475456537005874E-15, -89.62499999726880162, 5.000000000000000000 ) ) ;
#6924=DIRECTION ( 'NONE',  ( -0.000000000000000000, 1.000000000000000000, -0.000000000000000000 ) ) ;
#6927=DIRECTION ( 'NONE',  ( -0.000000000000000000, 1.000000000000000000, -0.000000000000000000 ) ) ;
#6929=CARTESIAN_POINT ( 'NONE',  ( 3.061616997868383141E-16, -156.8750000027311842, -5.000000000000000000 ) ) ;
#6935=( BOUNDED_CURVE ( )  B_SPLINE_CURVE ( 2, ( #55425, #51549, #21325, #11654, #27097, #11342, #30965, #31274, #62780 ),
 .UNSPECIFIED., .F., .F. ) 
 B_SPLINE_CURVE_WITH_KNOTS ( ( 3, 2, 2, 2, 3 ),
 ( 0.6416666666666662744, 0.6458333333333329263, 0.6499999999999996891, 0.6541666666666663410, 0.6583333333333329929 ),
 .UNSPECIFIED. ) 
 CURVE ( )  GEOMETRIC_REPRESENTATION_ITEM ( )  RATIONAL_B_SPLINE_CURVE ( ( 1.000000000000008216, 0.9238795325112786339, 1.000000000000000000, 0.9238795325112867385, 1.000000000000000000, 0.9238795325112867385, 1.000000000000000000, 0.9238795325112928447, 0.9999999999999938938 ) ) 
 REPRESENTATION_ITEM ( '' )  );
#6940=CARTESIAN_POINT ( 'NONE',  ( 4.458734124999999437, -26.81249999863440081, -5.460374474430324690E-16 ) ) ;
#6942=CARTESIAN_POINT ( 'NONE',  ( -5.000000000000000888, -150.4375000000000000, 2.071067811865474617 ) ) ;
#6944=CARTESIAN_POINT ( 'NONE',  ( -3.152801135295367096, -153.0625000013656063, -3.152801135295367541 ) ) ;
#6946=CARTESIAN_POINT ( 'NONE',  ( -2.229367062499996610, -52.39583333196773651, 3.861377020970582219 ) ) ;
#6947=AXIS2_PLACEMENT_3D ( 'NONE', #49216, #5474, #20271 ) ;
#6950=CARTESIAN_POINT ( 'NONE',  ( -2.499999999999996447, 22.16666666666666785, 4.330127018922195425 ) ) ;
#6952=VECTOR ( 'NONE', #37802, 1000.000000000000000 ) ;
#6953=CARTESIAN_POINT ( 'NONE',  ( 0.000000000000000000, -170.0000000000000000, 0.000000000000000000 ) ) ;
#6954=CARTESIAN_POINT ( 'NONE',  ( 9.457646018065525792E-16, 6.937500001365594748, 5.148502694627439702 ) ) ;
#6955=CARTESIAN_POINT ( 'NONE',  ( -6.972266317189433020E-16, 19.75000000000000000, -5.000000000000000000 ) ) ;
#6956=VECTOR ( 'NONE', #5341, 1000.000000000000000 ) ;
#6957=CARTESIAN_POINT ( 'NONE',  ( 5.000000000000000000, 13.49999999999999822, -6.123233995736766282E-16 ) ) ;
#6958=CARTESIAN_POINT ( 'NONE',  ( 1.339745962155612702, -7.294658198738518173, -5.000000000000000000 ) ) ;
#6959=CARTESIAN_POINT ( 'NONE',  ( 2.229367062500001939, 17.77083333469892779, 3.861377020970579999 ) ) ;
#6960=CARTESIAN_POINT ( 'NONE',  ( -5.000000000000000000, 5.125000002731184168, 0.000000000000000000 ) ) ;
#6962=DIRECTION ( 'NONE',  ( -0.000000000000000000, 1.000000000000000000, -0.000000000000000000 ) ) ;
#6963=ORIENTED_EDGE ( 'NONE', *, *, #51137, .F. ) ;
#6965=CARTESIAN_POINT ( 'NONE',  ( -2.229367062500000163, -41.47916666530107932, -3.861377020970580443 ) ) ;
#6966=CARTESIAN_POINT ( 'NONE',  ( -3.152801135295367096, -164.3125000013656063, -3.152801135295367541 ) ) ;
#6967=CARTESIAN_POINT ( 'NONE',  ( 5.000000000000000888, -44.45833333060214443, 2.886751345948126879 ) ) ;
#6968=VERTEX_POINT ( 'NONE', #49931 ) ;
#6969=CARTESIAN_POINT ( 'NONE',  ( 4.458734125000001214, -15.89583333196773651, 2.574251347313718519 ) ) ;
#6971=CARTESIAN_POINT ( 'NONE',  ( -3.535250795749689387E-16, -88.25000000000000000, -5.773502691896257311 ) ) ;
#6972=CARTESIAN_POINT ( 'NONE',  ( 1.846868145590736310, -163.6250000013656063, 4.458734124999999437 ) ) ;
#6973=CARTESIAN_POINT ( 'NONE',  ( -4.999999999999998224, -18.91666666666666430, 2.886751345948131764 ) ) ;
#6977=CARTESIAN_POINT ( 'NONE',  ( 2.229367062499998831, -29.89583333196773296, -3.861377020970580887 ) ) ;
#6978=CYLINDRICAL_SURFACE ( 'NONE', #18647, 5.000000000000000000 ) ;
#6983=ORIENTED_EDGE ( 'NONE', *, *, #7932, .F. ) ;
#6984=CARTESIAN_POINT ( 'NONE',  ( -3.535533905932737309, -166.7500000027312126, -3.535533905932738197 ) ) ;
#6986=CARTESIAN_POINT ( 'NONE',  ( 4.458734125000001214, -82.14583333196772230, 2.574251347313718519 ) ) ;
#6989=CARTESIAN_POINT ( 'NONE',  ( -8.190561711645485556E-16, -140.9375000013656063, 4.458734124999999437 ) ) ;
#6991=VECTOR ( 'NONE', #45192, 1000.000000000000000 ) ;
#6992=DIRECTION ( 'NONE',  ( -0.000000000000000000, 1.000000000000000000, -0.000000000000000000 ) ) ;
#6994=CARTESIAN_POINT ( 'NONE',  ( 4.458734124999998549, -44.72916666530106511, -2.574251347313721627 ) ) ;
#6997=CARTESIAN_POINT ( 'NONE',  ( 5.000000000000000888, -3.583333333333333925, 2.886751345948126879 ) ) ;
#7000=CARTESIAN_POINT ( 'NONE',  ( -6.972266317189433020E-16, -73.25000000000000000, -5.000000000000000000 ) ) ;
#7002=CARTESIAN_POINT ( 'NONE',  ( -3.152548672688508926E-16, -76.81249999863440792, -5.148502694627439702 ) ) ;
#7008=CARTESIAN_POINT ( 'NONE',  ( 5.000000000000000000, -47.50000000000000000, -6.123233995736766282E-16 ) ) ;
#7012=CARTESIAN_POINT ( 'NONE',  ( 4.458734125000000326, 13.85416666803225993, 2.574251347313718519 ) ) ;
#7019=CARTESIAN_POINT ( 'NONE',  ( 2.229367062500001939, -85.97916666530107932, 3.861377020970579999 ) ) ;
#7020=CARTESIAN_POINT ( 'NONE',  ( 2.229367062500001939, -10.97916666530107044, 3.861377020970579999 ) ) ;
#7023=CARTESIAN_POINT ( 'NONE',  ( 2.229367062499998831, -33.89583333196772941, -3.861377020970580887 ) ) ;
#7027=CARTESIAN_POINT ( 'NONE',  ( 4.458734124999999437, 18.18750000136559564, -5.460374474430324690E-16 ) ) ;
#7030=CARTESIAN_POINT ( 'NONE',  ( 4.458734124999998549, -77.97916666530106511, -2.574251347313721627 ) ) ;
#7032=CARTESIAN_POINT ( 'NONE',  ( 0.000000000000000000, -170.0000000000000000, 5.000000000000000000 ) ) ;
#7033=CARTESIAN_POINT ( 'NONE',  ( 5.000000000000000000, 21.70833333606451987, -2.886751345948129988 ) ) ;
#7035=CARTESIAN_POINT ( 'NONE',  ( 5.000000000000000000, -1.374999997268814500, -6.123233995736766282E-16 ) ) ;
#7038=CYLINDRICAL_SURFACE ( 'NONE', #15382, 5.000000000000000000 ) ;
#7039=CARTESIAN_POINT ( 'NONE',  ( -2.499999999999996447, -22.83333333333333215, 4.330127018922195425 ) ) ;
#7040=CARTESIAN_POINT ( 'NONE',  ( -2.229367062499996610, -27.14583333196774007, 3.861377020970582219 ) ) ;
#7041=CARTESIAN_POINT ( 'NONE',  ( 2.229367062500001939, -88.97916666530106511, 3.861377020970579999 ) ) ;
#7042=CARTESIAN_POINT ( 'NONE',  ( -4.999999999999999112, -30.79166666393548013, 2.886751345948131764 ) ) ;
#7043=CARTESIAN_POINT ( 'NONE',  ( -2.229367062499996610, -55.14583333196773651, 3.861377020970582219 ) ) ;
#7044=VERTEX_POINT ( 'NONE', #55089 ) ;
#7045=CARTESIAN_POINT ( 'NONE',  ( 5.000000000000000000, -27.49999999999999645, -6.123233995736766282E-16 ) ) ;
#7046=CARTESIAN_POINT ( 'NONE',  ( -3.152548672688508926E-16, -4.812499998634402587, -5.148502694627439702 ) ) ;
#7048=CARTESIAN_POINT ( 'NONE',  ( -2.499999999999996447, -69.83333333333332860, 4.330127018922195425 ) ) ;
#7051=FACE_OUTER_BOUND ( 'NONE', #53473, .T. ) ;
#7052=CARTESIAN_POINT ( 'NONE',  ( -4.999999999999999112, -69.79166666393547303, 2.886751345948131764 ) ) ;
#7055=EDGE_CURVE ( 'NONE', #59659, #27072, #791, .T. ) ;
#7056=CARTESIAN_POINT ( 'NONE',  ( 4.458734125000001214, -14.14583333196774184, 2.574251347313718519 ) ) ;
#7058=CARTESIAN_POINT ( 'NONE',  ( -4.458734124999999437, -52.64583333196773651, -2.574251347313719407 ) ) ;
#7060=CARTESIAN_POINT ( 'NONE',  ( -3.152801135295367985, -141.8125000013655779, 3.152801135295367096 ) ) ;
#7062=CARTESIAN_POINT ( 'NONE',  ( 2.071067811865603403, -158.1874999999999716, 4.999999999999872990 ) ) ;
#7063=ORIENTED_EDGE ( 'NONE', *, *, #49954, .F. ) ;
#7065=CARTESIAN_POINT ( 'NONE',  ( 4.458734125000001214, 23.85416666803225993, 2.574251347313718519 ) ) ;
#7067=ADVANCED_FACE ( 'NONE', ( #45755 ), #17364, .T. ) ;
#7068=CARTESIAN_POINT ( 'NONE',  ( 1.339745962155615144, -50.70534180126148271, 4.999999999999999112 ) ) ;
#7071=CARTESIAN_POINT ( 'NONE',  ( 2.730187237215162345E-16, -147.4375000013656063, -4.458734124999999437 ) ) ;
#7073=EDGE_CURVE ( 'NONE', #17293, #53696, #25006, .T. ) ;
#7074=DIRECTION ( 'NONE',  ( 0.000000000000000000, 0.000000000000000000, 1.000000000000000000 ) ) ;
#7075=CARTESIAN_POINT ( 'NONE',  ( 4.458734124999999437, -63.06249999863440792, -5.460374474430324690E-16 ) ) ;
#7078=CARTESIAN_POINT ( 'NONE',  ( 4.458734124999999437, -144.4375000013656063, 0.000000000000000000 ) ) ;
#7082=CARTESIAN_POINT ( 'NONE',  ( -3.535533905932737309, -164.7500000027312126, -3.535533905932738197 ) ) ;
#7085=CARTESIAN_POINT ( 'NONE',  ( -4.458734124999999437, 28.35416666803225993, -2.574251347313719407 ) ) ;
#7092=DIRECTION ( 'NONE',  ( -0.000000000000000000, 1.000000000000000000, -0.000000000000000000 ) ) ;
#7093=CARTESIAN_POINT ( 'NONE',  ( 2.626220312808019583E-14, 21.75000000000000000, -5.000000000000000000 ) ) ;
#7094=CARTESIAN_POINT ( 'NONE',  ( 9.457646018065525792E-16, 10.93750000136559208, 5.148502694627439702 ) ) ;
#7096=CARTESIAN_POINT ( 'NONE',  ( 4.458734125000000326, -14.14583333196774184, 2.574251347313718519 ) ) ;
#7098=CARTESIAN_POINT ( 'NONE',  ( -4.458734125000001214, -160.8750000013655779, 1.846868145590734089 ) ) ;
#7102=ADVANCED_FACE ( 'NONE', ( #28579 ), #53343, .T. ) ;
#7104=CARTESIAN_POINT ( 'NONE',  ( -5.000000000000000000, -36.00000000000000711, 0.000000000000000000 ) ) ;
#7105=CARTESIAN_POINT ( 'NONE',  ( 2.229367062500001939, -34.97916666530107221, 3.861377020970579999 ) ) ;
#7112=CARTESIAN_POINT ( 'NONE',  ( 2.071067811865392461, -144.3125000027312410, 5.000000000000084377 ) ) ;
#7113=CARTESIAN_POINT ( 'NONE',  ( 2.500000000000002220, -8.666666666666669627, 4.330127018922192761 ) ) ;
#7114=CARTESIAN_POINT ( 'NONE',  ( -3.152548672688508926E-16, -74.56249999863442213, -5.148502694627439702 ) ) ;
#7117=CARTESIAN_POINT ( 'NONE',  ( -4.999999999999999112, -6.791666663935481907, 2.886751345948131764 ) ) ;
#7118=CARTESIAN_POINT ( 'NONE',  ( 4.458734125000001214, -38.89583333196773651, 2.574251347313718519 ) ) ;
#7121=CARTESIAN_POINT ( 'NONE',  ( 2.229367062500001939, 12.77083333469892779, 3.861377020970579999 ) ) ;
#7123=CARTESIAN_POINT ( 'NONE',  ( 2.500000000000002220, -81.54166666393547303, 4.330127018922192761 ) ) ;
#7124=CARTESIAN_POINT ( 'NONE',  ( 5.000000000000000000, -56.49999999999999289, -6.123233995736766282E-16 ) ) ;
#7125=CARTESIAN_POINT ( 'NONE',  ( 3.152801135295366208, -161.8125000013656063, 3.152801135295367985 ) ) ;
#7127=CARTESIAN_POINT ( 'NONE',  ( -6.972266317189433020E-16, -35.25000000000000000, -5.000000000000000000 ) ) ;
#7128=CARTESIAN_POINT ( 'NONE',  ( -2.229367062500000163, -82.47916666530106511, -3.861377020970580443 ) ) ;
#7129=CARTESIAN_POINT ( 'NONE',  ( 5.000000000000000000, -170.0000000000000000, 0.000000000000000000 ) ) ;
#7130=CARTESIAN_POINT ( 'NONE',  ( 4.458734124999999437, -88.81249999863439371, -5.460374474430324690E-16 ) ) ;
#7132=CARTESIAN_POINT ( 'NONE',  ( -3.152548672688508926E-16, -34.81249999863440792, -5.148502694627439702 ) ) ;
#7140=VERTEX_POINT ( 'NONE', #52418 ) ;
#7141=CARTESIAN_POINT ( 'NONE',  ( -5.000000000000000000, -3.874999997268816720, 0.000000000000000000 ) ) ;
#7143=CARTESIAN_POINT ( 'NONE',  ( -4.458734124999999437, -66.64583333196773651, -2.574251347313719407 ) ) ;
#7148=DIRECTION ( 'NONE',  ( -0.000000000000000000, 1.000000000000000000, -0.000000000000000000 ) ) ;
#7154=CARTESIAN_POINT ( 'NONE',  ( -2.229367062500000163, 9.520833334698927786, -3.861377020970580443 ) ) ;
#7155=DIRECTION ( 'NONE',  ( 0.000000000000000000, 0.000000000000000000, 1.000000000000000000 ) ) ;
#7156=CARTESIAN_POINT ( 'NONE',  ( -4.458734125000000326, -156.8750000013655779, 1.846868145590734089 ) ) ;
#7157=CARTESIAN_POINT ( 'NONE',  ( -5.000000000000000000, 19.12500000273118772, 0.000000000000000000 ) ) ;
#7169=CARTESIAN_POINT ( 'NONE',  ( 4.458734124999999437, 29.18750000136559208, -5.460374474430324690E-16 ) ) ;
#7172=CARTESIAN_POINT ( 'NONE',  ( -4.458734124999997661, 3.520833334698929118, 2.574251347313722516 ) ) ;
#7175=CARTESIAN_POINT ( 'NONE',  ( 3.061616997868383141E-16, -146.8750000027312126, -5.000000000000000000 ) ) ;
#7177=VECTOR ( 'NONE', #35024, 1000.000000000000000 ) ;
#7182=CARTESIAN_POINT ( 'NONE',  ( -1.339745962155613812, -88.20534180126146850, -5.000000000000000000 ) ) ;
#7184=CARTESIAN_POINT ( 'NONE',  ( 4.458734124999999437, -163.6250000013656063, -1.846868145590734978 ) ) ;
#7187=CARTESIAN_POINT ( 'NONE',  ( -4.458734125000001214, -139.8750000013656063, 1.846868145590734089 ) ) ;
#7188=VERTEX_POINT ( 'NONE', #37929 ) ;
#7189=CARTESIAN_POINT ( 'NONE',  ( -4.458734124999999437, 21.43750000136559208, 0.000000000000000000 ) ) ;
#7190=VERTEX_POINT ( 'NONE', #57562 ) ;
#7195=CARTESIAN_POINT ( 'NONE',  ( -3.535250795749689387E-16, 6.749999999999999112, -5.773502691896257311 ) ) ;
#7196=CARTESIAN_POINT ( 'NONE',  ( 4.458734124999998549, -53.72916666530107932, -2.574251347313721627 ) ) ;
#7197=DIRECTION ( 'NONE',  ( -0.000000000000000000, 1.000000000000000000, -0.000000000000000000 ) ) ;
#7198=FACE_OUTER_BOUND ( 'NONE', #59652, .T. ) ;
#7199=CARTESIAN_POINT ( 'NONE',  ( 5.000000000000000888, 7.541666669397851130, 2.886751345948126879 ) ) ;
#7200=CARTESIAN_POINT ( 'NONE',  ( -6.972266317189433020E-16, -0.1249999972688142363, -5.000000000000000000 ) ) ;
#7202=CARTESIAN_POINT ( 'NONE',  ( -5.000000000000000000, -41.08333333333333570, -2.886751345948128211 ) ) ;
#7204=CARTESIAN_POINT ( 'NONE',  ( -5.000000000000000000, -45.08333333333333570, -2.886751345948128211 ) ) ;
#7206=CARTESIAN_POINT ( 'NONE',  ( -3.535533905932737309, -143.6250000000000000, -3.535533905932738197 ) ) ;
#7207=CARTESIAN_POINT ( 'NONE',  ( 4.458734124999999437, -60.81249999863440081, -5.460374474430324690E-16 ) ) ;
#7208=CARTESIAN_POINT ( 'NONE',  ( -4.458734124999999437, -151.1875000013656063, -5.460374474430324690E-16 ) ) ;
#7209=CARTESIAN_POINT ( 'NONE',  ( 4.458734124999999437, -70.81249999863439371, -5.460374474430324690E-16 ) ) ;
#7211=CARTESIAN_POINT ( 'NONE',  ( 2.229367062500001939, -17.22916666530106866, 3.861377020970579999 ) ) ;
#7212=CARTESIAN_POINT ( 'NONE',  ( 5.000000000000000000, -58.29166666393548724, -2.886751345948129988 ) ) ;
#7216=VERTEX_POINT ( 'NONE', #10233 ) ;
#7220=CARTESIAN_POINT ( 'NONE',  ( 2.730187237215162345E-16, -154.1875000013656063, -4.458734124999999437 ) ) ;
#7223=LINE ( 'NONE', #46452, #57055 ) ;
#7225=CARTESIAN_POINT ( 'NONE',  ( 1.339745962155612702, -8.294658198738519062, -5.000000000000000000 ) ) ;
#7226=AXIS2_PLACEMENT_3D ( 'NONE', #34869, #25212, #39043 ) ;
#7227=CARTESIAN_POINT ( 'NONE',  ( 4.458734124999999437, -46.06249999863440081, -5.460374474430324690E-16 ) ) ;
#7232=CARTESIAN_POINT ( 'NONE',  ( 4.458734125000001214, 22.10416666803225993, 2.574251347313718519 ) ) ;
#7241=CARTESIAN_POINT ( 'NONE',  ( 1.339745962155612702, -63.29465819873851729, -5.000000000000000000 ) ) ;
#7243=CARTESIAN_POINT ( 'NONE',  ( 3.535533905932738197, -157.0000000027312126, -3.535533905932738197 ) ) ;
#7248=DIRECTION ( 'NONE',  ( 0.000000000000000000, 0.000000000000000000, 1.000000000000000000 ) ) ;
#7253=CARTESIAN_POINT ( 'NONE',  ( -9.184850993605147944E-16, -159.3750000027311842, 5.000000000000000000 ) ) ;
#7259=CARTESIAN_POINT ( 'NONE',  ( -2.071067811865475061, -147.6875000000000284, -5.000000000000000888 ) ) ;
#7263=CARTESIAN_POINT ( 'NONE',  ( 2.229367062499998831, -24.64583333196773651, -3.861377020970580887 ) ) ;
#7265=CARTESIAN_POINT ( 'NONE',  ( -5.000000000000000888, -150.5625000000000284, -2.071067811865475949 ) ) ;
#7267=CARTESIAN_POINT ( 'NONE',  ( -1.846868145590737420, -153.7500000013656063, 4.458734124999999437 ) ) ;
#7268=ORIENTED_EDGE ( 'NONE', *, *, #54712, .F. ) ;
#7270=CARTESIAN_POINT ( 'NONE',  ( 4.458734124999998549, -50.97916666530107221, -2.574251347313721627 ) ) ;
#7271=DIRECTION ( 'NONE',  ( 0.000000000000000000, 0.000000000000000000, 1.000000000000000000 ) ) ;
#7273=CARTESIAN_POINT ( 'NONE',  ( -4.999999999999999112, 25.08333333333333215, 2.886751345948131764 ) ) ;
#7276=CARTESIAN_POINT ( 'NONE',  ( -4.458734124999998549, 6.770833334698928674, 2.574251347313722516 ) ) ;
#7277=CARTESIAN_POINT ( 'NONE',  ( 5.000000000000000000, 19.58333333333333215, -2.886751345948130876 ) ) ;
#7278=CARTESIAN_POINT ( 'NONE',  ( 5.000000000000000000, -11.29166666393547835, -2.886751345948130876 ) ) ;
#7280=CARTESIAN_POINT ( 'NONE',  ( 4.458734124999998549, 16.02083333469892423, -2.574251347313721627 ) ) ;
#7281=CARTESIAN_POINT ( 'NONE',  ( -4.999999999999999112, 2.208333336064519870, 2.886751345948131764 ) ) ;
#7284=ORIENTED_EDGE ( 'NONE', *, *, #8824, .F. ) ;
#7285=CARTESIAN_POINT ( 'NONE',  ( -5.000000000000000000, -71.00000000000000000, 0.000000000000000000 ) ) ;
#7286=CARTESIAN_POINT ( 'NONE',  ( 9.457646018065525792E-16, -43.06249999863440081, 5.148502694627439702 ) ) ;
#7287=CARTESIAN_POINT ( 'NONE',  ( 3.152801135295366208, -164.8125000013656063, 3.152801135295367985 ) ) ;
#7289=CARTESIAN_POINT ( 'NONE',  ( -5.000000000000000000, -45.95833333060214443, -2.886751345948128211 ) ) ;
#7290=ORIENTED_EDGE ( 'NONE', *, *, #29069, .F. ) ;
#7291=CARTESIAN_POINT ( 'NONE',  ( -3.152548672688508926E-16, -15.56249999863440614, -5.148502694627439702 ) ) ;
#7292=ORIENTED_EDGE ( 'NONE', *, *, #44069, .T. ) ;
#7293=CARTESIAN_POINT ( 'NONE',  ( -4.999999999999999112, -86.91666666666667140, 2.886751345948131764 ) ) ;
#7294=CARTESIAN_POINT ( 'NONE',  ( -1.846868145590737420, -162.7500000013655779, 4.458734124999999437 ) ) ;
#7295=CARTESIAN_POINT ( 'NONE',  ( -5.000000000000000000, -60.95833333060214443, -2.886751345948128211 ) ) ;
#7298=CARTESIAN_POINT ( 'NONE',  ( -2.229367062499996610, -33.39583333196772941, 3.861377020970582219 ) ) ;
#7305=VERTEX_POINT ( 'NONE', #4764 ) ;
#7306=CARTESIAN_POINT ( 'NONE',  ( -5.000000000000000888, -166.6875000027311842, -2.071067811865475949 ) ) ;
#7308=CARTESIAN_POINT ( 'NONE',  ( -4.458734124999999437, -81.64583333196773651, -2.574251347313719407 ) ) ;
#7311=CARTESIAN_POINT ( 'NONE',  ( 4.458734124999999437, -139.6875000013656063, 0.000000000000000000 ) ) ;
#7312=CARTESIAN_POINT ( 'NONE',  ( 2.499999999999998668, -84.20833333060214443, -4.330127018922193649 ) ) ;
#7314=CARTESIAN_POINT ( 'NONE',  ( 4.458734125000000326, -44.89583333196774362, 2.574251347313718519 ) ) ;
#7315=AXIS2_PLACEMENT_3D ( 'NONE', #51495, #56326, #31542 ) ;
#7318=( BOUNDED_CURVE ( )  B_SPLINE_CURVE ( 2, ( #19474, #23991, #8573, #63238, #42979, #33023, #39088, #14018, #34261 ),
 .UNSPECIFIED., .F., .F. ) 
 B_SPLINE_CURVE_WITH_KNOTS ( ( 3, 2, 2, 2, 3 ),
 ( 0.3812499999999999778, 0.3819444444444444198, 0.3833333333333333592, 0.3847222222222222432, 0.3854166666666666852 ),
 .UNSPECIFIED. ) 
 CURVE ( )  GEOMETRIC_REPRESENTATION_ITEM ( )  RATIONAL_B_SPLINE_CURVE ( ( 0.9330127018922194093, 0.9330127018922194093, 1.000000000000000000, 0.8660254037844387076, 1.000000000000000000, 0.8660254037844387076, 1.000000000000000000, 0.9330127018922194093, 0.9330127018922194093 ) ) 
 REPRESENTATION_ITEM ( '' )  );
#7319=CARTESIAN_POINT ( 'NONE',  ( 0.000000000000000000, -170.0000000000000000, 0.000000000000000000 ) ) ;
#7324=CARTESIAN_POINT ( 'NONE',  ( 2.229367062500001939, -79.22916666530106511, 3.861377020970579999 ) ) ;
#7332=CARTESIAN_POINT ( 'NONE',  ( -5.000000000000000888, -167.6875000027311842, -2.071067811865475949 ) ) ;
#7334=CARTESIAN_POINT ( 'NONE',  ( -3.152548672688508926E-16, 14.18750000136559386, -5.148502694627439702 ) ) ;
#7340=CARTESIAN_POINT ( 'NONE',  ( 9.457646018065525792E-16, -85.06249999863440792, 5.148502694627439702 ) ) ;
#7341=CARTESIAN_POINT ( 'NONE',  ( -2.229367062500000163, -10.47916666530106866, -3.861377020970580443 ) ) ;
#7343=ORIENTED_EDGE ( 'NONE', *, *, #7055, .T. ) ;
#7344=CARTESIAN_POINT ( 'NONE',  ( -3.152548672688508926E-16, -34.81249999863440792, -5.148502694627439702 ) ) ;
#7349=CARTESIAN_POINT ( 'NONE',  ( 3.152801135295366208, -150.8125000013655779, 3.152801135295367985 ) ) ;
#7350=CARTESIAN_POINT ( 'NONE',  ( -4.458734124999998549, 17.77083333469892779, 2.574251347313722516 ) ) ;
#7352=CARTESIAN_POINT ( 'NONE',  ( 1.975475456537005874E-15, -25.62499999726881228, 5.000000000000000000 ) ) ;
#7353=CARTESIAN_POINT ( 'NONE',  ( 2.229367062500001939, -84.22916666530107932, 3.861377020970579999 ) ) ;
#7355=CARTESIAN_POINT ( 'NONE',  ( 2.500000000000002220, -72.54166666393548724, 4.330127018922192761 ) ) ;
#7356=CARTESIAN_POINT ( 'NONE',  ( 2.499999999999998668, 18.79166666939785202, -4.330127018922193649 ) ) ;
#7357=ORIENTED_EDGE ( 'NONE', *, *, #29069, .T. ) ;
#7358=CARTESIAN_POINT ( 'NONE',  ( 5.000000000000000000, -147.1250000027312126, 0.000000000000000000 ) ) ;
#7361=CARTESIAN_POINT ( 'NONE',  ( -5.000000000000000000, -21.08333333333333570, -2.886751345948128211 ) ) ;
#7362=CARTESIAN_POINT ( 'NONE',  ( -4.458734124999999437, -27.39583333196773651, -2.574251347313719407 ) ) ;
#7363=AXIS2_PLACEMENT_3D ( 'NONE', #32581, #8769, #52835 ) ;
#7364=CARTESIAN_POINT ( 'NONE',  ( -4.458734124999997661, -87.22916666530107932, 2.574251347313722516 ) ) ;
#7365=CARTESIAN_POINT ( 'NONE',  ( -2.500000000000000444, -27.04166666393548013, -4.330127018922193649 ) ) ;
#7366=CARTESIAN_POINT ( 'NONE',  ( 4.458734124999998549, -55.72916666530107221, -2.574251347313721627 ) ) ;
#7367=EDGE_LOOP ( 'NONE', ( #14906, #42399, #35386, #23747 ) ) ;
#7369=CARTESIAN_POINT ( 'NONE',  ( 9.457646018065525792E-16, -7.312499998634405252, 5.148502694627439702 ) ) ;
#7370=ORIENTED_EDGE ( 'NONE', *, *, #33473, .T. ) ;
#7371=CARTESIAN_POINT ( 'NONE',  ( -5.000000000000000000, -72.08333333333332860, -2.886751345948128211 ) ) ;
#7374=CARTESIAN_POINT ( 'NONE',  ( 6.123233995736766282E-16, -170.0000000000000000, -5.000000000000000000 ) ) ;
#7376=CARTESIAN_POINT ( 'NONE',  ( -5.000000000000000000, -77.95833333060214443, -2.886751345948128211 ) ) ;
#7378=CARTESIAN_POINT ( 'NONE',  ( 2.229367062499998831, -16.89583333196773651, -3.861377020970580887 ) ) ;
#7379=CARTESIAN_POINT ( 'NONE',  ( -2.229367062499996610, -50.39583333196772941, 3.861377020970582219 ) ) ;
#7382=CARTESIAN_POINT ( 'NONE',  ( -3.152801135295367096, -142.0625000013655779, -3.152801135295367541 ) ) ;
#7384=DIRECTION ( 'NONE',  ( -0.000000000000000000, 1.000000000000000000, -0.000000000000000000 ) ) ;
#7385=ORIENTED_EDGE ( 'NONE', *, *, #6790, .F. ) ;
#7386=CARTESIAN_POINT ( 'NONE',  ( 0.000000000000000000, -170.0000000000000000, 0.000000000000000000 ) ) ;
#7388=CARTESIAN_POINT ( 'NONE',  ( 0.000000000000000000, -170.0000000000000000, 0.000000000000000000 ) ) ;
#7391=CARTESIAN_POINT ( 'NONE',  ( -4.458734124999999437, -148.1875000013656063, -5.460374474430324690E-16 ) ) ;
#7395=CARTESIAN_POINT ( 'NONE',  ( -4.458734124999999437, -62.64583333196774362, -2.574251347313719407 ) ) ;
#7396=CARTESIAN_POINT ( 'NONE',  ( -5.000000000000000000, -154.6250000027311842, -6.123233995736766282E-16 ) ) ;
#7397=CARTESIAN_POINT ( 'NONE',  ( 6.123233995736766282E-16, -170.0000000000000000, -5.000000000000000000 ) ) ;
#7398=CARTESIAN_POINT ( 'NONE',  ( 4.458734124999997661, -143.5000000013655779, 1.846868145590737864 ) ) ;
#7400=ORIENTED_EDGE ( 'NONE', *, *, #6641, .F. ) ;
#7406=CARTESIAN_POINT ( 'NONE',  ( -6.972266317189433020E-16, -7.249999999999998224, -5.000000000000000000 ) ) ;
#7407=CARTESIAN_POINT ( 'NONE',  ( 5.000000000000000000, -76.37499999726880162, -6.123233995736766282E-16 ) ) ;
#7411=CARTESIAN_POINT ( 'NONE',  ( 6.123233995736766282E-16, -170.0000000000000000, -5.000000000000000000 ) ) ;
#7413=CARTESIAN_POINT ( 'NONE',  ( -2.229367062499996610, 6.854166668032259935, 3.861377020970582219 ) ) ;
#7415=CARTESIAN_POINT ( 'NONE',  ( -4.458734124999999437, -18.64583333196774362, -2.574251347313719407 ) ) ;
#7416=( BOUNDED_CURVE ( )  B_SPLINE_CURVE ( 2, ( #12138, #17912, #52339, #8273, #3449, #23063, #42668, #46878, #18230 ),
 .UNSPECIFIED., .F., .F. ) 
 B_SPLINE_CURVE_WITH_KNOTS ( ( 3, 2, 2, 2, 3 ),
 ( 0.3812499999999999778, 0.3819444444444444198, 0.3833333333333333592, 0.3847222222222222432, 0.3854166666666666852 ),
 .UNSPECIFIED. ) 
 CURVE ( )  GEOMETRIC_REPRESENTATION_ITEM ( )  RATIONAL_B_SPLINE_CURVE ( ( 0.9330127018922194093, 0.9330127018922194093, 1.000000000000000000, 0.8660254037844387076, 1.000000000000000000, 0.8660254037844387076, 1.000000000000000000, 0.9330127018922194093, 0.9330127018922194093 ) ) 
 REPRESENTATION_ITEM ( '' )  );
#7418=CARTESIAN_POINT ( 'NONE',  ( 3.152801135295366208, -160.5625000013656063, 3.152801135295367985 ) ) ;
#7424=CARTESIAN_POINT ( 'NONE',  ( 2.229367062500001939, -37.97916666530107221, 3.861377020970579999 ) ) ;
#7426=CARTESIAN_POINT ( 'NONE',  ( 2.229367062499998831, -65.89583333196773651, -3.861377020970580887 ) ) ;
#7430=DIRECTION ( 'NONE',  ( 0.000000000000000000, 0.000000000000000000, 1.000000000000000000 ) ) ;
#7432=CARTESIAN_POINT ( 'NONE',  ( -9.184850993605147944E-16, -144.3750000027312126, 5.000000000000000000 ) ) ;
#7433=CARTESIAN_POINT ( 'NONE',  ( 5.000000000000000888, -6.583333333333329485, 2.886751345948126879 ) ) ;
#7434=CARTESIAN_POINT ( 'NONE',  ( -2.229367062499996610, -71.14583333196773651, 3.861377020970582219 ) ) ;
#7436=EDGE_CURVE ( 'NONE', #38838, #51005, #27080, .T. ) ;
#7437=CARTESIAN_POINT ( 'NONE',  ( -5.000000000000000000, -11.95833333060214976, -2.886751345948128211 ) ) ;
#7438=CARTESIAN_POINT ( 'NONE',  ( 2.229367062499998831, -38.64583333196773651, -3.861377020970580887 ) ) ;
#7439=VERTEX_POINT ( 'NONE', #40766 ) ;
#7440=FACE_OUTER_BOUND ( 'NONE', #1102, .T. ) ;
#7441=ADVANCED_FACE ( 'NONE', ( #31428 ), #2500, .T. ) ;
#7442=CARTESIAN_POINT ( 'NONE',  ( -3.152548672688508926E-16, 10.18750000136559564, -5.148502694627439702 ) ) ;
#7443=VERTEX_POINT ( 'NONE', #26293 ) ;
#7444=CARTESIAN_POINT ( 'NONE',  ( 1.339745962155612702, -81.29465819873850307, -5.000000000000000000 ) ) ;
#7445=CARTESIAN_POINT ( 'NONE',  ( 5.000000000000000000, -53.49999999999999289, -6.123233995736766282E-16 ) ) ;
#7446=CARTESIAN_POINT ( 'NONE',  ( -4.458734124999999437, -161.1875000013655779, -5.460374474430324690E-16 ) ) ;
#7448=CARTESIAN_POINT ( 'NONE',  ( 5.000000000000000888, -144.9375000000000000, -2.071067811865475505 ) ) ;
#7449=CARTESIAN_POINT ( 'NONE',  ( 4.458734125000001214, -78.89583333196772230, 2.574251347313718519 ) ) ;
#7450=CARTESIAN_POINT ( 'NONE',  ( -9.184850993605147944E-16, -165.2500000000000000, 5.000000000000000000 ) ) ;
#7451=CARTESIAN_POINT ( 'NONE',  ( 2.229367062499998831, -87.64583333196773651, -3.861377020970580887 ) ) ;
#7453=CARTESIAN_POINT ( 'NONE',  ( -2.229367062499996610, 0.6041666680322611560, 3.861377020970582219 ) ) ;
#7455=CARTESIAN_POINT ( 'NONE',  ( 2.229367062500001939, -33.22916666530106511, 3.861377020970579999 ) ) ;
#7456=CARTESIAN_POINT ( 'NONE',  ( 1.975475456537005874E-15, -72.75000000000000000, 5.000000000000000000 ) ) ;
#7458=CARTESIAN_POINT ( 'NONE',  ( 1.975475456537005874E-15, -86.75000000000001421, 5.000000000000000000 ) ) ;
#7462=CARTESIAN_POINT ( 'NONE',  ( -2.229367062500000163, -71.72916666530107932, -3.861377020970580443 ) ) ;
#7467=DIRECTION ( 'NONE',  ( 0.000000000000000000, -0.000000000000000000, 1.000000000000000000 ) ) ;
#7468=CARTESIAN_POINT ( 'NONE',  ( 4.458734124999998549, 10.27083333469892779, -2.574251347313721627 ) ) ;
#7469=LINE ( 'NONE', #47018, #56261 ) ;
#7470=CARTESIAN_POINT ( 'NONE',  ( -3.152801135295367096, -157.0625000013656063, -3.152801135295367541 ) ) ;
#7475=CARTESIAN_POINT ( 'NONE',  ( 5.000000000000000000, -140.0625000000000000, 2.071067811865478614 ) ) ;
#7480=CARTESIAN_POINT ( 'NONE',  ( -4.458734124999999437, 24.60416666803225993, -2.574251347313719407 ) ) ;
#7483=CARTESIAN_POINT ( 'NONE',  ( 2.229367062499998831, -3.895833331967739177, -3.861377020970580887 ) ) ;
#7484=CARTESIAN_POINT ( 'NONE',  ( 5.000000000000000000, -0.2916666639354824619, -2.886751345948130876 ) ) ;
#7486=CARTESIAN_POINT ( 'NONE',  ( 5.000000000000000000, -141.1875000027312126, 2.071067811865478614 ) ) ;
#7487=CARTESIAN_POINT ( 'NONE',  ( 2.499999999999998668, -33.20833333060215153, -4.330127018922193649 ) ) ;
#7493=CARTESIAN_POINT ( 'NONE',  ( -5.000000000000000000, -87.08333333333331439, -2.886751345948128211 ) ) ;
#7494=ADVANCED_FACE ( 'NONE', ( #25984 ), #33644, .T. ) ;
#7496=EDGE_CURVE ( 'NONE', #20545, #11671, #31207, .T. ) ;
#7498=CARTESIAN_POINT ( 'NONE',  ( 1.846868145590735200, -163.5000000013655779, -4.458734124999999437 ) ) ;
#7500=CARTESIAN_POINT ( 'NONE',  ( -5.000000000000000888, -147.4375000000000000, 2.071067811865474617 ) ) ;
#7502=CARTESIAN_POINT ( 'NONE',  ( 2.229367062500001939, 17.77083333469892779, 3.861377020970579999 ) ) ;
#7503=ORIENTED_EDGE ( 'NONE', *, *, #45964, .F. ) ;
#7508=CARTESIAN_POINT ( 'NONE',  ( 1.060575238724906964E-15, 7.249999999999999112, 5.773502691896257311 ) ) ;
#7510=CARTESIAN_POINT ( 'NONE',  ( 2.229367062500001939, -56.97916666530107932, 3.861377020970579999 ) ) ;
#7513=CARTESIAN_POINT ( 'NONE',  ( -1.339745962155613812, -38.08034179853029144, -5.000000000000000000 ) ) ;
#7517=CARTESIAN_POINT ( 'NONE',  ( -4.999999999999999112, -38.91666666666667140, 2.886751345948131764 ) ) ;
#7518=CARTESIAN_POINT ( 'NONE',  ( -6.972266317189433020E-16, 12.87500000273118417, -5.000000000000000000 ) ) ;
#7519=CARTESIAN_POINT ( 'NONE',  ( 1.975475456537005874E-15, -47.74999999999999289, 5.000000000000000000 ) ) ;
#7522=CARTESIAN_POINT ( 'NONE',  ( -2.229367062499996610, -67.14583333196773651, 3.861377020970582219 ) ) ;
#7523=CARTESIAN_POINT ( 'NONE',  ( 2.730187237215162345E-16, -151.4375000013656063, -4.458734124999999437 ) ) ;
#7524=CARTESIAN_POINT ( 'NONE',  ( 4.458734124999998549, -68.72916666530106511, -2.574251347313721627 ) ) ;
#7526=CARTESIAN_POINT ( 'NONE',  ( -3.152548672688508926E-16, -19.81249999863440436, -5.148502694627439702 ) ) ;
#7527=CARTESIAN_POINT ( 'NONE',  ( -3.535250795749689387E-16, -62.12499999726880873, -5.773502691896257311 ) ) ;
#7529=CARTESIAN_POINT ( 'NONE',  ( -1.339745962155613812, -49.20534180126148271, -5.000000000000000000 ) ) ;
#7532=CARTESIAN_POINT ( 'NONE',  ( 5.000000000000000000, -149.1875000027312410, 2.071067811865478614 ) ) ;
#7533=CARTESIAN_POINT ( 'NONE',  ( -1.846868145590737420, -153.7500000013656063, 4.458734124999999437 ) ) ;
#7534=ORIENTED_EDGE ( 'NONE', *, *, #56397, .T. ) ;
#7537=CARTESIAN_POINT ( 'NONE',  ( -2.500000000000000444, -75.04166666393547303, -4.330127018922193649 ) ) ;
#7538=CARTESIAN_POINT ( 'NONE',  ( -3.152548672688508926E-16, -55.81249999863440081, -5.148502694627439702 ) ) ;
#7539=ORIENTED_EDGE ( 'NONE', *, *, #27180, .T. ) ;
#7540=CYLINDRICAL_SURFACE ( 'NONE', #55243, 5.000000000000000000 ) ;
#7543=CARTESIAN_POINT ( 'NONE',  ( -3.152548672688508926E-16, 21.43750000136559564, -5.148502694627439702 ) ) ;
#7546=CARTESIAN_POINT ( 'NONE',  ( -1.846868145590737420, -167.7500000013655779, 4.458734124999997661 ) ) ;
#7547=ORIENTED_EDGE ( 'NONE', *, *, #25532, .T. ) ;
#7551=AXIS2_PLACEMENT_3D ( 'NONE', #61178, #17101, #36085 ) ;
#7552=CARTESIAN_POINT ( 'NONE',  ( 0.000000000000000000, -170.0000000000000000, 0.000000000000000000 ) ) ;
#7556=CARTESIAN_POINT ( 'NONE',  ( 2.071067811865370256, -160.8125000000000284, -5.000000000000105693 ) ) ;
#7560=VERTEX_POINT ( 'NONE', #6543 ) ;
#7561=CARTESIAN_POINT ( 'NONE',  ( 1.975475456537005874E-15, -26.62499999726881228, 5.000000000000000000 ) ) ;
#7563=CARTESIAN_POINT ( 'NONE',  ( -3.535533905932737309, -154.7500000027312126, -3.535533905932738197 ) ) ;
#7564=ORIENTED_EDGE ( 'NONE', *, *, #48070, .F. ) ;
#7569=CARTESIAN_POINT ( 'NONE',  ( -3.535533905932738641, -148.3750000000000000, 3.535533905932737309 ) ) ;
#7570=EDGE_CURVE ( 'NONE', #39600, #9299, #35724, .T. ) ;
#7574=CARTESIAN_POINT ( 'NONE',  ( 4.458734125000000326, -23.89583333196773651, 2.574251347313718519 ) ) ;
#7578=CARTESIAN_POINT ( 'NONE',  ( -3.152801135295367096, -152.0625000013655779, -3.152801135295367541 ) ) ;
#7581=CARTESIAN_POINT ( 'NONE',  ( -2.229367062500000163, -49.72916666530107221, -3.861377020970580443 ) ) ;
#7585=CARTESIAN_POINT ( 'NONE',  ( -5.000000000000000000, 22.00000000000000000, 0.000000000000000000 ) ) ;
#7586=MANIFOLD_SOLID_BREP ( 'Thread2', #31553 ) ;
#7588=EDGE_CURVE ( 'NONE', #51364, #24132, #31586, .T. ) ;
#7589=CARTESIAN_POINT ( 'NONE',  ( 0.000000000000000000, -170.0000000000000000, 5.000000000000000000 ) ) ;
#7590=CARTESIAN_POINT ( 'NONE',  ( 4.458734124999998549, 1.270833334698927342, -2.574251347313721627 ) ) ;
#7591=CARTESIAN_POINT ( 'NONE',  ( -2.071067811865559882, -160.8125000027312126, -4.999999999999914735 ) ) ;
#7594=CARTESIAN_POINT ( 'NONE',  ( -4.458734124999999437, 15.35416666803225993, -2.574251347313719407 ) ) ;
#7595=CARTESIAN_POINT ( 'NONE',  ( -2.499999999999996447, 3.291666669397851575, 4.330127018922195425 ) ) ;
#7596=ADVANCED_FACE ( 'NONE', ( #62792 ), #18404, .T. ) ;
#7599=ORIENTED_EDGE ( 'NONE', *, *, #21436, .T. ) ;
#7600=( BOUNDED_CURVE ( )  B_SPLINE_CURVE ( 2, ( #34406, #9973, #53722, #662, #35069, #59841, #54686, #63389, #20601 ),
 .UNSPECIFIED., .F., .F. ) 
 B_SPLINE_CURVE_WITH_KNOTS ( ( 3, 2, 2, 2, 3 ),
 ( 0.8520833333333333037, 0.8527777777777777457, 0.8541666666666666297, 0.8555555555555555136, 0.8562499999999999556 ),
 .UNSPECIFIED. ) 
 CURVE ( )  GEOMETRIC_REPRESENTATION_ITEM ( )  RATIONAL_B_SPLINE_CURVE ( ( 0.9330127018922194093, 0.9330127018922194093, 1.000000000000000000, 0.8660254037844387076, 1.000000000000000000, 0.8660254037844387076, 1.000000000000000000, 0.9330127018922194093, 0.9330127018922194093 ) ) 
 REPRESENTATION_ITEM ( '' )  );
#7601=CARTESIAN_POINT ( 'NONE',  ( -2.229367062500000163, -46.47916666530106511, -3.861377020970580443 ) ) ;
#7602=ADVANCED_FACE ( 'NONE', ( #27112 ), #47981, .T. ) ;
#7603=CARTESIAN_POINT ( 'NONE',  ( 3.152801135295366208, -162.8125000013656063, 3.152801135295367985 ) ) ;
#7606=CARTESIAN_POINT ( 'NONE',  ( 2.499999999999998668, -43.20833333060214443, -4.330127018922193649 ) ) ;
#7607=VERTEX_POINT ( 'NONE', #39586 ) ;
#7608=CARTESIAN_POINT ( 'NONE',  ( -4.458734124999999437, -24.31249999863440436, 0.000000000000000000 ) ) ;
#7609=EDGE_LOOP ( 'NONE', ( #34633, #61310, #4342, #27176 ) ) ;
#7610=CARTESIAN_POINT ( 'NONE',  ( 1.060575238724906964E-15, -85.74999999999998579, 5.773502691896257311 ) ) ;
#7611=CARTESIAN_POINT ( 'NONE',  ( 2.730187237215162345E-16, -164.1875000013655779, -4.458734124999999437 ) ) ;
#7614=CARTESIAN_POINT ( 'NONE',  ( 9.457646018065525792E-16, -33.31249999863440792, 5.148502694627439702 ) ) ;
#7615=CARTESIAN_POINT ( 'NONE',  ( -9.184850993605147944E-16, -147.3750000027312126, 5.000000000000000000 ) ) ;
#7616=VERTEX_POINT ( 'NONE', #59223 ) ;
#7619=CARTESIAN_POINT ( 'NONE',  ( -2.500000000000000444, -29.04166666393548013, -4.330127018922193649 ) ) ;
#7623=CARTESIAN_POINT ( 'NONE',  ( 2.229367062499998831, -78.89583333196773651, -3.861377020970580887 ) ) ;
#7626=CARTESIAN_POINT ( 'NONE',  ( -5.000000000000000000, -158.6250000027311842, -6.123233995736766282E-16 ) ) ;
#7627=CARTESIAN_POINT ( 'NONE',  ( 5.000000000000000000, 20.58333333333333215, -2.886751345948130876 ) ) ;
#7629=CARTESIAN_POINT ( 'NONE',  ( 9.457646018065525792E-16, -48.06249999863440792, 5.148502694627439702 ) ) ;
#7630=CARTESIAN_POINT ( 'NONE',  ( -1.339745962155623360, 21.20534180126147561, 4.999999999999991118 ) ) ;
#7632=CARTESIAN_POINT ( 'NONE',  ( -1.339745962155636017, 4.205341801261478274, 4.999999999999985789 ) ) ;
#7635=CARTESIAN_POINT ( 'NONE',  ( 6.123233995736766282E-16, -170.0000000000000000, -5.000000000000000000 ) ) ;
#7637=CARTESIAN_POINT ( 'NONE',  ( -3.152548672688508926E-16, -78.81249999863440792, -5.148502694627439702 ) ) ;
#7641=VERTEX_POINT ( 'NONE', #33514 ) ;
#7646=CARTESIAN_POINT ( 'NONE',  ( 4.458734124999999437, 14.93750000136559386, -5.460374474430324690E-16 ) ) ;
#7653=CARTESIAN_POINT ( 'NONE',  ( 1.975475456537005874E-15, -13.62499999726881228, 5.000000000000000000 ) ) ;
#7654=CARTESIAN_POINT ( 'NONE',  ( 1.339745962155615144, 17.29465819873852084, 4.999999999999999112 ) ) ;
#7655=CARTESIAN_POINT ( 'NONE',  ( -2.229367062500000163, -6.479166665301072214, -3.861377020970580443 ) ) ;
#7657=ORIENTED_EDGE ( 'NONE', *, *, #28417, .F. ) ;
#7658=CARTESIAN_POINT ( 'NONE',  ( 2.229367062500001939, -33.22916666530106511, 3.861377020970579999 ) ) ;
#7663=CARTESIAN_POINT ( 'NONE',  ( -4.458734125000000326, -150.1250000013655779, 1.846868145590734089 ) ) ;
#7664=CARTESIAN_POINT ( 'NONE',  ( -3.152548672688508926E-16, 12.43750000136559564, -5.148502694627439702 ) ) ;
#7665=LINE ( 'NONE', #16358, #990 ) ;
#7666=CARTESIAN_POINT ( 'NONE',  ( 1.975475456537005874E-15, -28.74999999999999645, 5.000000000000000000 ) ) ;
#7667=CARTESIAN_POINT ( 'NONE',  ( -4.458734124999999437, -85.64583333196773651, -2.574251347313719407 ) ) ;
#7670=CARTESIAN_POINT ( 'NONE',  ( -5.000000000000000000, 19.12500000273118772, 0.000000000000000000 ) ) ;
#7671=ORIENTED_EDGE ( 'NONE', *, *, #38989, .T. ) ;
#7675=CARTESIAN_POINT ( 'NONE',  ( 2.500000000000002220, -23.66666666666666785, 4.330127018922192761 ) ) ;
#7676=CARTESIAN_POINT ( 'NONE',  ( -4.458734124999998549, -30.22916666530106866, 2.574251347313722516 ) ) ;
#7677=CARTESIAN_POINT ( 'NONE',  ( 1.339745962155615144, 0.2946581987385212820, 4.999999999999999112 ) ) ;
#7678=( BOUNDED_CURVE ( )  B_SPLINE_CURVE ( 2, ( #31110, #1546, #59440, #915, #30796, #40754, #45906, #584, #6049 ),
 .UNSPECIFIED., .F., .F. ) 
 B_SPLINE_CURVE_WITH_KNOTS ( ( 3, 2, 2, 2, 3 ),
 ( 0.5729166666666666297, 0.5736111111111110716, 0.5749999999999999556, 0.5763888888888888395, 0.5770833333333332815 ),
 .UNSPECIFIED. ) 
 CURVE ( )  GEOMETRIC_REPRESENTATION_ITEM ( )  RATIONAL_B_SPLINE_CURVE ( ( 0.9330127018922194093, 0.9330127018922194093, 1.000000000000000000, 0.8660254037844387076, 1.000000000000000000, 0.8660254037844387076, 1.000000000000000000, 0.9330127018922194093, 0.9330127018922194093 ) ) 
 REPRESENTATION_ITEM ( '' )  );
#7680=CARTESIAN_POINT ( 'NONE',  ( 5.000000000000000888, -28.45833333060214443, 2.886751345948126879 ) ) ;
#7681=CARTESIAN_POINT ( 'NONE',  ( 2.229367062499998831, -58.64583333196773651, -3.861377020970580887 ) ) ;
#7682=ORIENTED_EDGE ( 'NONE', *, *, #52400, .T. ) ;
#7684=CARTESIAN_POINT ( 'NONE',  ( 2.229367062500001939, -10.22916666530106866, 3.861377020970579999 ) ) ;
#7685=ORIENTED_EDGE ( 'NONE', *, *, #50325, .T. ) ;
#7686=CARTESIAN_POINT ( 'NONE',  ( 5.000000000000000000, -71.41666666666665719, -2.886751345948129988 ) ) ;
#7689=CARTESIAN_POINT ( 'NONE',  ( 5.000000000000000000, -79.29166666393548724, -2.886751345948129988 ) ) ;
#7690=CARTESIAN_POINT ( 'NONE',  ( 5.000000000000000000, -10.29166666393547658, -2.886751345948130876 ) ) ;
#7691=ORIENTED_EDGE ( 'NONE', *, *, #22457, .F. ) ;
#7693=CARTESIAN_POINT ( 'NONE',  ( -4.458734124999999437, -14.56249999863440436, 0.000000000000000000 ) ) ;
#7694=CARTESIAN_POINT ( 'NONE',  ( 2.229367062500001939, -58.22916666530107932, 3.861377020970579999 ) ) ;
#7696=( BOUNDED_CURVE ( )  B_SPLINE_CURVE ( 2, ( #21390, #7241, #23203, #6591, #1789, #18378, #26207, #60955, #11407 ),
 .UNSPECIFIED., .F., .F. ) 
 B_SPLINE_CURVE_WITH_KNOTS ( ( 3, 2, 2, 2, 3 ),
 ( 0.7770833333333333481, 0.7777777777777777901, 0.7791666666666666741, 0.7805555555555555580, 0.7812500000000000000 ),
 .UNSPECIFIED. ) 
 CURVE ( )  GEOMETRIC_REPRESENTATION_ITEM ( )  RATIONAL_B_SPLINE_CURVE ( ( 0.9330127018922194093, 0.9330127018922194093, 1.000000000000000000, 0.8660254037844387076, 1.000000000000000000, 0.8660254037844387076, 1.000000000000000000, 0.9330127018922194093, 0.9330127018922194093 ) ) 
 REPRESENTATION_ITEM ( '' )  );
#7697=CARTESIAN_POINT ( 'NONE',  ( -5.000000000000000000, -29.95833333060214443, -2.886751345948128211 ) ) ;
#7699=CARTESIAN_POINT ( 'NONE',  ( 2.730187237215162345E-16, -169.4375000013656063, -4.458734124999999437 ) ) ;
#7702=ORIENTED_EDGE ( 'NONE', *, *, #33394, .F. ) ;
#7705=FACE_OUTER_BOUND ( 'NONE', #62871, .T. ) ;
#7708=CARTESIAN_POINT ( 'NONE',  ( -8.190561711645485556E-16, -146.9375000013656063, 4.458734124999999437 ) ) ;
#7710=CYLINDRICAL_SURFACE ( 'NONE', #45786, 5.000000000000000000 ) ;
#7712=CARTESIAN_POINT ( 'NONE',  ( -2.229367062499996610, -62.39583333196774362, 3.861377020970582219 ) ) ;
#7713=DIRECTION ( 'NONE',  ( 0.000000000000000000, 0.000000000000000000, -1.000000000000000000 ) ) ;
#7715=CARTESIAN_POINT ( 'NONE',  ( -4.458734124999999437, -146.9375000013656063, -5.460374474430324690E-16 ) ) ;
#7717=ORIENTED_EDGE ( 'NONE', *, *, #5820, .T. ) ;
#7723=CARTESIAN_POINT ( 'NONE',  ( -4.458734124999997661, 28.52083333469892423, 2.574251347313722516 ) ) ;
#7727=LINE ( 'NONE', #41802, #61268 ) ;
#7728=CARTESIAN_POINT ( 'NONE',  ( -2.500000000000000444, -15.16666666666666785, -4.330127018922193649 ) ) ;
#7729=CARTESIAN_POINT ( 'NONE',  ( 4.458734125000000326, 9.104166668032261711, 2.574251347313718519 ) ) ;
#7731=CARTESIAN_POINT ( 'NONE',  ( -4.458734124999999437, -19.56249999863440081, 0.000000000000000000 ) ) ;
#7733=CARTESIAN_POINT ( 'NONE',  ( -1.846868145590737420, -161.7500000013655495, 4.458734124999999437 ) ) ;
#7737=CARTESIAN_POINT ( 'NONE',  ( 5.000000000000000000, -139.1250000027312126, 0.000000000000000000 ) ) ;
#7738=CARTESIAN_POINT ( 'NONE',  ( -4.458734124999999437, -39.31249999863440081, 0.000000000000000000 ) ) ;
#7740=CARTESIAN_POINT ( 'NONE',  ( -4.458734124999999437, -65.56249999863440792, 0.000000000000000000 ) ) ;
#7743=ORIENTED_EDGE ( 'NONE', *, *, #13991, .T. ) ;
#7744=DIRECTION ( 'NONE',  ( -0.000000000000000000, 1.000000000000000000, -0.000000000000000000 ) ) ;
#7745=( BOUNDED_CURVE ( )  B_SPLINE_CURVE ( 2, ( #54384, #25103, #5489, #10623, #35396, #39887, #26382, #50831, #676 ),
 .UNSPECIFIED., .F., .F. ) 
 B_SPLINE_CURVE_WITH_KNOTS ( ( 3, 2, 2, 2, 3 ),
 ( 0.9895833333333333703, 0.9902777777777778123, 0.9916666666666666963, 0.9930555555555555802, 0.9937500000000000222 ),
 .UNSPECIFIED. ) 
 CURVE ( )  GEOMETRIC_REPRESENTATION_ITEM ( )  RATIONAL_B_SPLINE_CURVE ( ( 0.9330127018922194093, 0.9330127018922194093, 1.000000000000000000, 0.8660254037844387076, 1.000000000000000000, 0.8660254037844387076, 1.000000000000000000, 0.9330127018922194093, 0.9330127018922194093 ) ) 
 REPRESENTATION_ITEM ( '' )  );
#7746=CARTESIAN_POINT ( 'NONE',  ( -4.999999999999999112, -9.916666666666662522, 2.886751345948131764 ) ) ;
#7747=CARTESIAN_POINT ( 'NONE',  ( -4.458734124999999437, -72.39583333196773651, -2.574251347313719407 ) ) ;
#7749=CARTESIAN_POINT ( 'NONE',  ( -4.999999999999999112, -13.79166666393548191, 2.886751345948131764 ) ) ;
#7750=CARTESIAN_POINT ( 'NONE',  ( 2.229367062500001939, -41.97916666530107932, 3.861377020970579999 ) ) ;
#7751=ORIENTED_EDGE ( 'NONE', *, *, #5971, .T. ) ;
#7752=DIRECTION ( 'NONE',  ( 0.000000000000000000, 0.000000000000000000, 1.000000000000000000 ) ) ;
#7753=CARTESIAN_POINT ( 'NONE',  ( 2.229367062499998831, 8.104166668032261711, -3.861377020970580887 ) ) ;
#7755=CARTESIAN_POINT ( 'NONE',  ( 5.000000000000000000, -34.29166666393547303, -2.886751345948130876 ) ) ;
#7756=CARTESIAN_POINT ( 'NONE',  ( 5.000000000000000888, -54.58333333333332860, 2.886751345948126879 ) ) ;
#7757=CARTESIAN_POINT ( 'NONE',  ( 4.458734125000000326, -161.6250000013656063, -1.846868145590734978 ) ) ;
#7760=CARTESIAN_POINT ( 'NONE',  ( 2.229367062500001939, -81.97916666530106511, 3.861377020970579999 ) ) ;
#7761=CARTESIAN_POINT ( 'NONE',  ( -5.000000000000000888, -164.4375000000000284, 2.071067811865474617 ) ) ;
#7762=CARTESIAN_POINT ( 'NONE',  ( 9.457646018065525792E-16, -89.06249999863439371, 5.148502694627439702 ) ) ;
#7764=CARTESIAN_POINT ( 'NONE',  ( -4.458734124999999437, -1.645833331967737401, -2.574251347313719407 ) ) ;
#7765=CARTESIAN_POINT ( 'NONE',  ( 4.458734124999999437, -42.06249999863440081, -5.460374474430324690E-16 ) ) ;
#7766=CARTESIAN_POINT ( 'NONE',  ( 2.500000000000002220, -16.54166666393548368, 4.330127018922192761 ) ) ;
#7768=VERTEX_POINT ( 'NONE', #58277 ) ;
#7771=LINE ( 'NONE', #56030, #16815 ) ;
#7772=CARTESIAN_POINT ( 'NONE',  ( -2.229367062500000163, -67.72916666530106511, -3.861377020970580443 ) ) ;
#7776=ORIENTED_EDGE ( 'NONE', *, *, #57913, .T. ) ;
#7777=AXIS2_PLACEMENT_3D ( 'NONE', #22627, #12641, #32256 ) ;
#7782=CARTESIAN_POINT ( 'NONE',  ( -3.152548672688508926E-16, 4.437500001365595637, -5.148502694627439702 ) ) ;
#7783=CARTESIAN_POINT ( 'NONE',  ( 3.535533905932736864, -154.1250000000000000, 3.535533905932738641 ) ) ;
#7784=CARTESIAN_POINT ( 'NONE',  ( -3.152801135295367096, -158.0625000013656063, -3.152801135295367541 ) ) ;
#7792=ADVANCED_FACE ( 'NONE', ( #10329 ), #29619, .T. ) ;
#7799=CARTESIAN_POINT ( 'NONE',  ( 4.458734124999998549, 23.27083333469892423, -2.574251347313721627 ) ) ;
#7801=CARTESIAN_POINT ( 'NONE',  ( -3.152548672688508926E-16, -2.812499998634407472, -5.148502694627439702 ) ) ;
#7804=CARTESIAN_POINT ( 'NONE',  ( 3.061616997868383141E-16, -140.8750000027312126, -5.000000000000000000 ) ) ;
#7805=CARTESIAN_POINT ( 'NONE',  ( -4.999999999999998224, -20.79166666393548013, 2.886751345948131764 ) ) ;
#7810=CARTESIAN_POINT ( 'NONE',  ( 0.000000000000000000, -170.0000000000000000, 5.000000000000000000 ) ) ;
#7813=CARTESIAN_POINT ( 'NONE',  ( -4.458734124999999437, -156.1875000013655779, -5.460374474430324690E-16 ) ) ;
#7816=CARTESIAN_POINT ( 'NONE',  ( -2.229367062500000163, 16.27083333469892779, -3.861377020970580443 ) ) ;
#7817=ORIENTED_EDGE ( 'NONE', *, *, #51420, .F. ) ;
#7822=CARTESIAN_POINT ( 'NONE',  ( -5.000000000000000000, 5.916666666666666963, -2.886751345948128211 ) ) ;
#7823=CARTESIAN_POINT ( 'NONE',  ( 4.458734124999999437, -57.81249999863440081, -5.460374474430324690E-16 ) ) ;
#7831=CARTESIAN_POINT ( 'NONE',  ( -5.000000000000000000, -38.08333333333333570, -2.886751345948128211 ) ) ;
#7832=CARTESIAN_POINT ( 'NONE',  ( -5.000000000000000000, 13.12500000273118417, 0.000000000000000000 ) ) ;
#7836=CARTESIAN_POINT ( 'NONE',  ( -2.229367062499996610, -64.14583333196773651, 3.861377020970582219 ) ) ;
#7837=CARTESIAN_POINT ( 'NONE',  ( -8.190561711645485556E-16, -148.9375000013656063, 4.458734124999999437 ) ) ;
#7838=CARTESIAN_POINT ( 'NONE',  ( 4.458734124999999437, -72.81249999863439371, -5.460374474430324690E-16 ) ) ;
#7840=CARTESIAN_POINT ( 'NONE',  ( -4.458734124999999437, -17.64583333196773651, -2.574251347313719407 ) ) ;
#7841=CARTESIAN_POINT ( 'NONE',  ( 5.000000000000000888, -60.45833333060213732, 2.886751345948126879 ) ) ;
#7842=ORIENTED_EDGE ( 'NONE', *, *, #38979, .T. ) ;
#7843=CARTESIAN_POINT ( 'NONE',  ( -2.071067811865306307, -150.6875000000000853, -5.000000000000171418 ) ) ;
#7846=LINE ( 'NONE', #57062, #15281 ) ;
#7851=CARTESIAN_POINT ( 'NONE',  ( -6.972266317189433020E-16, -43.25000000000000000, -5.000000000000000000 ) ) ;
#7852=CARTESIAN_POINT ( 'NONE',  ( 4.458734124999999437, -56.06249999863440081, -5.460374474430324690E-16 ) ) ;
#7853=EDGE_CURVE ( 'NONE', #1043, #21692, #26711, .T. ) ;
#7857=CARTESIAN_POINT ( 'NONE',  ( -4.458734124999998549, 18.77083333469893134, 2.574251347313722516 ) ) ;
#7859=CARTESIAN_POINT ( 'NONE',  ( 1.339745962155615144, -13.58034179853029322, 4.999999999999999112 ) ) ;
#7860=CARTESIAN_POINT ( 'NONE',  ( 4.458734124999999437, -168.4375000013656063, 0.000000000000000000 ) ) ;
#7864=CARTESIAN_POINT ( 'NONE',  ( 1.975475456537005874E-15, -30.62499999726881228, 5.000000000000000000 ) ) ;
#7877=EDGE_LOOP ( 'NONE', ( #5385, #57966, #29265, #47841 ) ) ;
#7880=CARTESIAN_POINT ( 'NONE',  ( 3.061616997868383141E-16, -153.8750000027311842, -5.000000000000000000 ) ) ;
#7886=CARTESIAN_POINT ( 'NONE',  ( 2.071067811865475505, -145.8125000000000284, -5.000000000000000888 ) ) ;
#7889=CARTESIAN_POINT ( 'NONE',  ( -2.499999999999996447, -54.83333333333332860, 4.330127018922195425 ) ) ;
#7890=CARTESIAN_POINT ( 'NONE',  ( -3.152548672688508926E-16, -25.56249999863440792, -5.148502694627439702 ) ) ;
#7891=CARTESIAN_POINT ( 'NONE',  ( -4.999999999999998224, 9.208333336064519870, 2.886751345948131764 ) ) ;
#7893=CARTESIAN_POINT ( 'NONE',  ( 3.152801135295366208, -148.5625000013655779, 3.152801135295367985 ) ) ;
#7896=CARTESIAN_POINT ( 'NONE',  ( -4.458734124999997661, -53.47916666530107221, 2.574251347313722516 ) ) ;
#7897=CARTESIAN_POINT ( 'NONE',  ( 5.000000000000000000, -58.37499999726880873, -6.123233995736766282E-16 ) ) ;
#7899=CARTESIAN_POINT ( 'NONE',  ( 5.000000000000000888, 25.41666666666666430, 2.886751345948126879 ) ) ;
#7902=CARTESIAN_POINT ( 'NONE',  ( 4.458734124999999437, -2.812499998634407472, -5.460374474430324690E-16 ) ) ;
#7904=CARTESIAN_POINT ( 'NONE',  ( 3.535533905932738197, -140.8750000000000000, -3.535533905932738197 ) ) ;
#7906=CARTESIAN_POINT ( 'NONE',  ( 4.458734125000001214, 7.854166668032260823, 2.574251347313718519 ) ) ;
#7907=ORIENTED_EDGE ( 'NONE', *, *, #12317, .T. ) ;
#7908=CARTESIAN_POINT ( 'NONE',  ( 1.339745962155615144, -42.70534180126148982, 4.999999999999999112 ) ) ;
#7911=CARTESIAN_POINT ( 'NONE',  ( 4.458734125000001214, -46.89583333196773651, 2.574251347313718519 ) ) ;
#7912=CARTESIAN_POINT ( 'NONE',  ( -3.152801135295367985, -159.0625000013656063, 3.152801135295367096 ) ) ;
#7913=AXIS2_PLACEMENT_3D ( 'NONE', #6559, #26173, #46111 ) ;
#7915=CARTESIAN_POINT ( 'NONE',  ( 2.499999999999998668, -44.20833333060214443, -4.330127018922193649 ) ) ;
#7917=CARTESIAN_POINT ( 'NONE',  ( -2.229367062500000163, -25.47916666530106866, -3.861377020970580443 ) ) ;
#7918=VERTEX_POINT ( 'NONE', #40239 ) ;
#7919=( BOUNDED_CURVE ( )  B_SPLINE_CURVE ( 2, ( #37666, #8097, #12903, #31898, #61502, #27381, #28013, #41853, #17432 ),
 .UNSPECIFIED., .F., .F. ) 
 B_SPLINE_CURVE_WITH_KNOTS ( ( 3, 2, 2, 2, 3 ),
 ( 0.1916666666666668462, 0.1958333333333334980, 0.2000000000000001776, 0.2041666666666668295, 0.2083333333333335091 ),
 .UNSPECIFIED. ) 
 CURVE ( )  GEOMETRIC_REPRESENTATION_ITEM ( )  RATIONAL_B_SPLINE_CURVE ( ( 0.9999999999999970024, 0.9238795325112897361, 1.000000000000000000, 0.9238795325112867385, 1.000000000000000000, 0.9238795325112867385, 1.000000000000000000, 0.9238795325112837409, 1.000000000000003109 ) ) 
 REPRESENTATION_ITEM ( '' )  );
#7921=CARTESIAN_POINT ( 'NONE',  ( -3.152801135295367985, -165.8125000013656063, 3.152801135295367096 ) ) ;
#7922=DIRECTION ( 'NONE',  ( 0.000000000000000000, 0.000000000000000000, 1.000000000000000000 ) ) ;
#7924=CARTESIAN_POINT ( 'NONE',  ( 2.229367062499998831, -39.89583333196773651, -3.861377020970580887 ) ) ;
#7925=DIRECTION ( 'NONE',  ( 0.000000000000000000, 0.000000000000000000, 1.000000000000000000 ) ) ;
#7927=EDGE_CURVE ( 'NONE', #14051, #592, #46810, .T. ) ;
#7931=CARTESIAN_POINT ( 'NONE',  ( 5.000000000000000000, -140.0000000000000000, 0.000000000000000000 ) ) ;
#7932=EDGE_CURVE ( 'NONE', #33925, #20951, #50532, .T. ) ;
#7936=CARTESIAN_POINT ( 'NONE',  ( 4.458734125000001214, -81.14583333196773651, 2.574251347313718519 ) ) ;
#7938=CARTESIAN_POINT ( 'NONE',  ( 3.535533905932736864, -143.1250000000000000, 3.535533905932738641 ) ) ;
#7944=CARTESIAN_POINT ( 'NONE',  ( 1.339745962155612702, -3.294658198738522170, -5.000000000000000000 ) ) ;
#7950=CARTESIAN_POINT ( 'NONE',  ( 4.458734124999999437, -81.06249999863440792, -5.460374474430324690E-16 ) ) ;
#7951=EDGE_CURVE ( 'NONE', #49521, #2442, #39832, .T. ) ;
#7958=CARTESIAN_POINT ( 'NONE',  ( -5.000000000000000888, -163.6875000027311842, -2.071067811865475949 ) ) ;
#7960=CARTESIAN_POINT ( 'NONE',  ( 4.458734124999998549, 15.02083333469892779, -2.574251347313721627 ) ) ;
#7961=DIRECTION ( 'NONE',  ( 0.000000000000000000, 0.000000000000000000, 1.000000000000000000 ) ) ;
#7968=CARTESIAN_POINT ( 'NONE',  ( -6.972266317189433020E-16, 17.75000000000000355, -5.000000000000000000 ) ) ;
#7969=CARTESIAN_POINT ( 'NONE',  ( -2.229367062500000163, -9.479166665301068662, -3.861377020970580443 ) ) ;
#7971=ORIENTED_EDGE ( 'NONE', *, *, #21290, .F. ) ;
#7972=CARTESIAN_POINT ( 'NONE',  ( 4.458734124999999437, -37.06249999863440792, -5.460374474430324690E-16 ) ) ;
#7973=( BOUNDED_CURVE ( )  B_SPLINE_CURVE ( 2, ( #18561, #43613, #63255, #8904, #48757, #28520, #4699, #19173, #38788 ),
 .UNSPECIFIED., .F., .F. ) 
 B_SPLINE_CURVE_WITH_KNOTS ( ( 3, 2, 2, 2, 3 ),
 ( 0.9354166666666666741, 0.9361111111111111160, 0.9375000000000000000, 0.9388888888888888840, 0.9395833333333333259 ),
 .UNSPECIFIED. ) 
 CURVE ( )  GEOMETRIC_REPRESENTATION_ITEM ( )  RATIONAL_B_SPLINE_CURVE ( ( 0.9330127018922194093, 0.9330127018922194093, 1.000000000000000000, 0.8660254037844387076, 1.000000000000000000, 0.8660254037844387076, 1.000000000000000000, 0.9330127018922194093, 0.9330127018922194093 ) ) 
 REPRESENTATION_ITEM ( '' )  );
#7978=CARTESIAN_POINT ( 'NONE',  ( -4.458734124999999437, -150.1875000013656063, -5.460374474430324690E-16 ) ) ;
#7979=CARTESIAN_POINT ( 'NONE',  ( -4.458734124999999437, 14.68750000136559386, 0.000000000000000000 ) ) ;
#7980=CARTESIAN_POINT ( 'NONE',  ( -6.972266317189433020E-16, -82.12499999726881583, -5.000000000000000000 ) ) ;
#7982=CARTESIAN_POINT ( 'NONE',  ( -3.152548672688508926E-16, -85.81249999863440792, -5.148502694627439702 ) ) ;
#7984=CARTESIAN_POINT ( 'NONE',  ( -2.499999999999996447, -1.708333330602145761, 4.330127018922195425 ) ) ;
#7985=CARTESIAN_POINT ( 'NONE',  ( -4.999999999999999112, 21.20833333606451987, 2.886751345948131764 ) ) ;
#7988=CARTESIAN_POINT ( 'NONE',  ( 1.975475456537005874E-15, -52.75000000000000000, 5.000000000000000000 ) ) ;
#7989=CARTESIAN_POINT ( 'NONE',  ( 5.000000000000000000, -27.41666666666666785, -2.886751345948129988 ) ) ;
#7990=CARTESIAN_POINT ( 'NONE',  ( -2.229367062499996610, -33.14583333196772941, 3.861377020970582219 ) ) ;
#7991=CYLINDRICAL_SURFACE ( 'NONE', #57279, 5.000000000000000000 ) ;
#7992=CARTESIAN_POINT ( 'NONE',  ( -3.535250795749689387E-16, -29.12499999726881228, -5.773502691896257311 ) ) ;
#7993=CARTESIAN_POINT ( 'NONE',  ( 2.229367062499998831, -59.64583333196774362, -3.861377020970580887 ) ) ;
#7995=CARTESIAN_POINT ( 'NONE',  ( 5.000000000000000000, -62.29166666393547303, -2.886751345948130876 ) ) ;
#7996=CARTESIAN_POINT ( 'NONE',  ( -4.458734124999999437, -9.562499998634406140, 0.000000000000000000 ) ) ;
#7998=CARTESIAN_POINT ( 'NONE',  ( -3.535250795749689387E-16, -75.25000000000001421, -5.773502691896257311 ) ) ;
#8001=VECTOR ( 'NONE', #51309, 1000.000000000000114 ) ;
#8002=CARTESIAN_POINT ( 'NONE',  ( 1.060575238724906964E-15, -76.62499999726881583, 5.773502691896257311 ) ) ;
#8003=DIRECTION ( 'NONE',  ( -0.000000000000000000, 1.000000000000000000, -0.000000000000000000 ) ) ;
#8007=CARTESIAN_POINT ( 'NONE',  ( -2.229367062499996610, -19.39583333196774007, 3.861377020970582219 ) ) ;
#8008=CARTESIAN_POINT ( 'NONE',  ( 4.458734124999998549, -56.97916666530107932, -2.574251347313721627 ) ) ;
#8010=FILL_AREA_STYLE ('',( #27613 ) ) ;
#8011=CARTESIAN_POINT ( 'NONE',  ( 3.152801135295366208, -141.5625000013655779, 3.152801135295367985 ) ) ;
#8013=LINE ( 'NONE', #60783, #15331 ) ;
#8020=CARTESIAN_POINT ( 'NONE',  ( -1.846868145590734756, -146.3750000013655779, -4.458734125000000326 ) ) ;
#8022=FACE_OUTER_BOUND ( 'NONE', #92, .T. ) ;
#8024=CARTESIAN_POINT ( 'NONE',  ( -3.152548672688508926E-16, -63.81249999863440792, -5.148502694627439702 ) ) ;
#8025=EDGE_CURVE ( 'NONE', #53443, #38064, #1980, .T. ) ;
#8027=CARTESIAN_POINT ( 'NONE',  ( 1.846868145590736310, -144.6250000013655779, 4.458734124999997661 ) ) ;
#8032=CARTESIAN_POINT ( 'NONE',  ( 1.339745962155602488, 16.29465819873851373, 5.000000000000007105 ) ) ;
#8037=CARTESIAN_POINT ( 'NONE',  ( -2.229367062500000163, 26.27083333469892779, -3.861377020970580443 ) ) ;
#8038=CARTESIAN_POINT ( 'NONE',  ( 1.975475456537005874E-15, -17.62499999726881938, 5.000000000000000000 ) ) ;
#8044=CARTESIAN_POINT ( 'NONE',  ( -4.458734124999999437, 5.604166668032261711, -2.574251347313719407 ) ) ;
#8046=CARTESIAN_POINT ( 'NONE',  ( -2.229367062500000163, -20.72916666530107221, -3.861377020970580443 ) ) ;
#8047=AXIS2_PLACEMENT_3D ( 'NONE', #4472, #38874, #54638 ) ;
#8049=CARTESIAN_POINT ( 'NONE',  ( 2.730187237215162345E-16, -159.1875000013655779, -4.458734124999999437 ) ) ;
#8050=DIRECTION ( 'NONE',  ( -0.000000000000000000, 1.000000000000000000, -0.000000000000000000 ) ) ;
#8056=CARTESIAN_POINT ( 'NONE',  ( -2.229367062500000163, -40.47916666530107221, -3.861377020970580443 ) ) ;
#8058=CARTESIAN_POINT ( 'NONE',  ( 4.458734125000000326, -70.14583333196773651, 2.574251347313718519 ) ) ;
#8061=CARTESIAN_POINT ( 'NONE',  ( 5.000000000000000000, -36.29166666393547303, -2.886751345948130876 ) ) ;
#8065=CARTESIAN_POINT ( 'NONE',  ( -5.000000000000000000, -15.00000000000000000, 0.000000000000000000 ) ) ;
#8066=CARTESIAN_POINT ( 'NONE',  ( -4.458734124999998549, -16.22916666530107577, 2.574251347313722516 ) ) ;
#8067=CARTESIAN_POINT ( 'NONE',  ( 2.229367062500001939, -76.97916666530106511, 3.861377020970579999 ) ) ;
#8069=LINE ( 'NONE', #52755, #13406 ) ;
#8070=CARTESIAN_POINT ( 'NONE',  ( -3.535250795749689387E-16, -15.12499999726881406, -5.773502691896257311 ) ) ;
#8071=CARTESIAN_POINT ( 'NONE',  ( -4.458734124999999437, -45.31249999863440081, 0.000000000000000000 ) ) ;
#8073=CARTESIAN_POINT ( 'NONE',  ( 2.071067811865517694, -143.8125000000000000, -4.999999999999958256 ) ) ;
#8074=CARTESIAN_POINT ( 'NONE',  ( -2.229367062499996610, 6.604166668032259935, 3.861377020970582219 ) ) ;
#8075=ORIENTED_EDGE ( 'NONE', *, *, #61113, .F. ) ;
#8076=CARTESIAN_POINT ( 'NONE',  ( -5.000000000000000000, -151.5000000000000284, -6.123233995736766282E-16 ) ) ;
#8077=CARTESIAN_POINT ( 'NONE',  ( 2.500000000000002220, -53.66666666666667140, 4.330127018922192761 ) ) ;
#8078=CARTESIAN_POINT ( 'NONE',  ( 2.730187237215162345E-16, -160.4375000013655779, -4.458734124999999437 ) ) ;
#8081=CARTESIAN_POINT ( 'NONE',  ( -3.152548672688508926E-16, -78.56249999863440792, -5.148502694627439702 ) ) ;
#8082=CARTESIAN_POINT ( 'NONE',  ( -3.535533905932738641, -167.3750000000000284, 3.535533905932737309 ) ) ;
#8085=CARTESIAN_POINT ( 'NONE',  ( -2.229367062500000163, -2.729166665301069550, -3.861377020970580443 ) ) ;
#8086=CARTESIAN_POINT ( 'NONE',  ( 4.458734124999999437, -41.06249999863440081, -5.460374474430324690E-16 ) ) ;
#8089=DIRECTION ( 'NONE',  ( -0.000000000000000000, 1.000000000000000000, -0.000000000000000000 ) ) ;
#8090=ORIENTED_EDGE ( 'NONE', *, *, #33768, .F. ) ;
#8093=CARTESIAN_POINT ( 'NONE',  ( -4.458734124999999437, -67.56249999863440792, 0.000000000000000000 ) ) ;
#8094=AXIS2_PLACEMENT_3D ( 'NONE', #33290, #39363, #28769 ) ;
#8097=CARTESIAN_POINT ( 'NONE',  ( 2.071067811865540342, -164.1875000000000000, 4.999999999999936051 ) ) ;
#8100=DIRECTION ( 'NONE',  ( 1.000000000000000000, 0.000000000000000000, -0.000000000000000000 ) ) ;
#8101=CARTESIAN_POINT ( 'NONE',  ( 4.458734124999999437, 0.1875000013655953035, -5.460374474430324690E-16 ) ) ;
#8102=CARTESIAN_POINT ( 'NONE',  ( 1.975475456537005874E-15, -42.75000000000000000, 5.000000000000000000 ) ) ;
#8103=CARTESIAN_POINT ( 'NONE',  ( -8.190561711645485556E-16, -156.6875000013655779, 4.458734124999999437 ) ) ;
#8105=VERTEX_POINT ( 'NONE', #37010 ) ;
#8107=CARTESIAN_POINT ( 'NONE',  ( -5.000000000000000000, -25.00000000000000000, 0.000000000000000000 ) ) ;
#8116=CARTESIAN_POINT ( 'NONE',  ( -4.458734124999997661, 20.77083333469892779, 2.574251347313722516 ) ) ;
#8118=CARTESIAN_POINT ( 'NONE',  ( 4.458734125000000326, -3.145833331967738289, 2.574251347313718519 ) ) ;
#8120=LINE ( 'NONE', #42828, #48329 ) ;
#8122=CARTESIAN_POINT ( 'NONE',  ( 5.000000000000000000, -143.1875000027312126, 2.071067811865478614 ) ) ;
#8123=CARTESIAN_POINT ( 'NONE',  ( 0.000000000000000000, -170.0000000000000000, 5.000000000000000000 ) ) ;
#8127=CARTESIAN_POINT ( 'NONE',  ( -1.339745962155610925, -86.79465819873851729, 5.000000000000000000 ) ) ;
#8128=DIRECTION ( 'NONE',  ( -0.000000000000000000, 1.000000000000000000, -0.000000000000000000 ) ) ;
#8130=CARTESIAN_POINT ( 'NONE',  ( 4.458734124999997661, -155.7500000013656063, 1.846868145590737864 ) ) ;
#8132=CARTESIAN_POINT ( 'NONE',  ( -5.000000000000000000, -147.5000000000000284, -6.123233995736766282E-16 ) ) ;
#8133=ORIENTED_EDGE ( 'NONE', *, *, #7073, .F. ) ;
#8134=CARTESIAN_POINT ( 'NONE',  ( 4.458734125000001214, 17.85416666803225993, 2.574251347313718519 ) ) ;
#8135=EDGE_LOOP ( 'NONE', ( #50665, #37197, #38735 ) ) ;
#8138=VECTOR ( 'NONE', #55451, 1000.000000000000000 ) ;
#8141=CARTESIAN_POINT ( 'NONE',  ( -2.500000000000000444, 8.833333333333332149, -4.330127018922193649 ) ) ;
#8144=CARTESIAN_POINT ( 'NONE',  ( -4.458734124999999437, -61.31249999863440081, 0.000000000000000000 ) ) ;
#8145=CARTESIAN_POINT ( 'NONE',  ( -6.972266317189433020E-16, -8.249999999999998224, -5.000000000000000000 ) ) ;
#8147=CARTESIAN_POINT ( 'NONE',  ( 4.458734124999999437, -30.81249999863440436, -5.460374474430324690E-16 ) ) ;
#8148=CARTESIAN_POINT ( 'NONE',  ( -6.972266317189433020E-16, -38.12499999726880873, -5.000000000000000000 ) ) ;
#8151=CARTESIAN_POINT ( 'NONE',  ( -2.499999999999996447, -40.83333333333333570, 4.330127018922195425 ) ) ;
#8153=( BOUNDED_CURVE ( )  B_SPLINE_CURVE ( 2, ( #22628, #37407, #57042, #29632, #59234, #4258, #47996, #48620, #23873 ),
 .UNSPECIFIED., .F., .F. ) 
 B_SPLINE_CURVE_WITH_KNOTS ( ( 3, 2, 2, 2, 3 ),
 ( 0.5250000000000004663, 0.5291666666666671182, 0.5333333333333338810, 0.5375000000000005329, 0.5416666666666671848 ),
 .UNSPECIFIED. ) 
 CURVE ( )  GEOMETRIC_REPRESENTATION_ITEM ( )  RATIONAL_B_SPLINE_CURVE ( ( 0.9999999999999918954, 0.9238795325112948431, 1.000000000000000000, 0.9238795325112867385, 1.000000000000000000, 0.9238795325112867385, 1.000000000000000000, 0.9238795325112766355, 1.000000000000010214 ) ) 
 REPRESENTATION_ITEM ( '' )  );
#8154=CARTESIAN_POINT ( 'NONE',  ( -5.000000000000000000, -48.08333333333332860, -2.886751345948128211 ) ) ;
#8156=CARTESIAN_POINT ( 'NONE',  ( -2.500000000000000444, 12.83333333333333215, -4.330127018922193649 ) ) ;
#8157=CARTESIAN_POINT ( 'NONE',  ( -2.229367062500000163, -67.47916666530106511, -3.861377020970580443 ) ) ;
#8158=CARTESIAN_POINT ( 'NONE',  ( -1.846868145590737420, -148.0000000013655779, 4.458734124999999437 ) ) ;
#8159=CARTESIAN_POINT ( 'NONE',  ( -4.458734124999998549, -72.22916666530107932, 2.574251347313722516 ) ) ;
#8161=CARTESIAN_POINT ( 'NONE',  ( 4.458734124999998549, -25.97916666530106866, -2.574251347313721627 ) ) ;
#8162=CARTESIAN_POINT ( 'NONE',  ( -3.535250795749689387E-16, -64.12499999726881583, -5.773502691896257311 ) ) ;
#8167=CARTESIAN_POINT ( 'NONE',  ( 2.500000000000002220, -21.54166666393548013, 4.330127018922192761 ) ) ;
#8172=CARTESIAN_POINT ( 'NONE',  ( -4.458734124999998549, -52.47916666530107221, 2.574251347313722516 ) ) ;
#8173=VERTEX_POINT ( 'NONE', #57586 ) ;
#8174=DIRECTION ( 'NONE',  ( -0.000000000000000000, 1.000000000000000000, -0.000000000000000000 ) ) ;
#8176=CARTESIAN_POINT ( 'NONE',  ( -4.458734124999999437, 18.60416666803225993, -2.574251347313719407 ) ) ;
#8178=DIRECTION ( 'NONE',  ( -0.000000000000000000, 1.000000000000000000, -0.000000000000000000 ) ) ;
#8181=CARTESIAN_POINT ( 'NONE',  ( -1.339745962155613812, -40.20534180126147561, -5.000000000000000000 ) ) ;
#8183=VECTOR ( 'NONE', #20867, 1000.000000000000000 ) ;
#8184=CARTESIAN_POINT ( 'NONE',  ( 2.499999999999998668, -69.20833333060214443, -4.330127018922193649 ) ) ;
#8187=CARTESIAN_POINT ( 'NONE',  ( 2.500000000000002220, 4.333333333333331261, 4.330127018922192761 ) ) ;
#8189=CARTESIAN_POINT ( 'NONE',  ( 5.000000000000000000, -76.41666666666665719, -2.886751345948130876 ) ) ;
#8190=DIRECTION ( 'NONE',  ( -0.000000000000000000, 1.000000000000000000, -0.000000000000000000 ) ) ;
#8193=VERTEX_POINT ( 'NONE', #32811 ) ;
#8196=CARTESIAN_POINT ( 'NONE',  ( 2.071067811865476394, -153.3125000027311842, 5.000000000000000000 ) ) ;
#8197=ORIENTED_EDGE ( 'NONE', *, *, #14608, .F. ) ;
#8202=CARTESIAN_POINT ( 'NONE',  ( 3.535533905932736864, -146.1250000000000000, 3.535533905932738641 ) ) ;
#8205=CARTESIAN_POINT ( 'NONE',  ( 4.458734124999999437, -168.6875000013656063, 0.000000000000000000 ) ) ;
#8206=CARTESIAN_POINT ( 'NONE',  ( -4.458734124999999437, -22.39583333196773651, -2.574251347313719407 ) ) ;
#8207=CARTESIAN_POINT ( 'NONE',  ( 5.000000000000000000, -147.0625000000000000, 2.071067811865478614 ) ) ;
#8210=CARTESIAN_POINT ( 'NONE',  ( -4.458734125000000326, -147.0000000013655779, -1.846868145590735644 ) ) ;
#8211=ORIENTED_EDGE ( 'NONE', *, *, #29539, .F. ) ;
#8213=CARTESIAN_POINT ( 'NONE',  ( 4.458734124999999437, -54.06249999863440081, -5.460374474430324690E-16 ) ) ;
#8216=CARTESIAN_POINT ( 'NONE',  ( -5.000000000000000000, 23.91666666666666785, -2.886751345948128211 ) ) ;
#8217=EDGE_CURVE ( 'NONE', #4014, #57905, #47290, .T. ) ;
#8219=CARTESIAN_POINT ( 'NONE',  ( -4.458734124999998549, -1.229166665301071326, 2.574251347313722516 ) ) ;
#8222=CARTESIAN_POINT ( 'NONE',  ( -4.458734124999999437, 12.43750000136559564, 0.000000000000000000 ) ) ;
#8227=CARTESIAN_POINT ( 'NONE',  ( 2.229367062499998831, -47.64583333196774362, -3.861377020970580887 ) ) ;
#8228=CARTESIAN_POINT ( 'NONE',  ( -4.458734124999999437, -161.1875000013655779, -5.460374474430324690E-16 ) ) ;
#8230=EDGE_CURVE ( 'NONE', #1775, #52605, #53367, .T. ) ;
#8231=CARTESIAN_POINT ( 'NONE',  ( -5.000000000000000000, -42.95833333060214443, -2.886751345948128211 ) ) ;
#8233=CARTESIAN_POINT ( 'NONE',  ( -2.229367062500000163, -24.47916666530106866, -3.861377020970580443 ) ) ;
#8237=CARTESIAN_POINT ( 'NONE',  ( 2.730187237215162345E-16, -162.1875000013655779, -4.458734124999999437 ) ) ;
#8240=CARTESIAN_POINT ( 'NONE',  ( -4.458734124999999437, -39.56249999863440081, 0.000000000000000000 ) ) ;
#8241=CARTESIAN_POINT ( 'NONE',  ( -5.000000000000000000, 20.12500000273118772, 0.000000000000000000 ) ) ;
#8243=EDGE_CURVE ( 'NONE', #58694, #49521, #62411, .T. ) ;
#8244=( BOUNDED_CURVE ( )  B_SPLINE_CURVE ( 2, ( #44129, #38369, #57995, #43498, #48020, #96, #57378, #58310, #33858 ),
 .UNSPECIFIED., .F., .F. ) 
 B_SPLINE_CURVE_WITH_KNOTS ( ( 3, 2, 2, 2, 3 ),
 ( 0.9395833333333333259, 0.9402777777777777679, 0.9416666666666666519, 0.9430555555555555358, 0.9437499999999999778 ),
 .UNSPECIFIED. ) 
 CURVE ( )  GEOMETRIC_REPRESENTATION_ITEM ( )  RATIONAL_B_SPLINE_CURVE ( ( 0.9330127018922194093, 0.9330127018922194093, 1.000000000000000000, 0.8660254037844387076, 1.000000000000000000, 0.8660254037844387076, 1.000000000000000000, 0.9330127018922194093, 0.9330127018922194093 ) ) 
 REPRESENTATION_ITEM ( '' )  );
#8247=DIRECTION ( 'NONE',  ( -0.000000000000000000, 1.000000000000000000, -0.000000000000000000 ) ) ;
#8249=FACE_OUTER_BOUND ( 'NONE', #52274, .T. ) ;
#8251=CARTESIAN_POINT ( 'NONE',  ( -4.458734124999998549, -88.47916666530107932, 2.574251347313722516 ) ) ;
#8254=CARTESIAN_POINT ( 'NONE',  ( -4.458734125000000326, -140.1250000013656347, 1.846868145590734089 ) ) ;
#8255=CARTESIAN_POINT ( 'NONE',  ( 1.975475456537005874E-15, -57.74999999999999289, 5.000000000000000000 ) ) ;
#8263=DIRECTION ( 'NONE',  ( -0.000000000000000000, 1.000000000000000000, -0.000000000000000000 ) ) ;
#8264=CARTESIAN_POINT ( 'NONE',  ( -1.339745962155610925, -45.66965819600733312, 5.000000000000000000 ) ) ;
#8265=CARTESIAN_POINT ( 'NONE',  ( 2.229367062499998831, -84.89583333196773651, -3.861377020970580887 ) ) ;
#8270=CARTESIAN_POINT ( 'NONE',  ( 3.535533905932738197, -167.0000000027312126, -3.535533905932738197 ) ) ;
#8272=CARTESIAN_POINT ( 'NONE',  ( -4.458734124999999437, 8.354166668032261711, -2.574251347313719407 ) ) ;
#8273=CARTESIAN_POINT ( 'NONE',  ( -4.999999999999998224, -15.91666666666666963, 2.886751345948131764 ) ) ;
#8279=CARTESIAN_POINT ( 'NONE',  ( -6.972266317189433020E-16, -57.25000000000000000, -5.000000000000000000 ) ) ;
#8280=CARTESIAN_POINT ( 'NONE',  ( 9.457646018065525792E-16, -7.062499998634404363, 5.148502694627439702 ) ) ;
#8283=CARTESIAN_POINT ( 'NONE',  ( 9.457646018065525792E-16, -33.31249999863440792, 5.148502694627439702 ) ) ;
#8290=CARTESIAN_POINT ( 'NONE',  ( -4.458734124999999437, 17.60416666803225993, -2.574251347313719407 ) ) ;
#8291=EDGE_CURVE ( 'NONE', #39751, #32568, #34366, .T. ) ;
#8292=EDGE_CURVE ( 'NONE', #34281, #23906, #46435, .T. ) ;
#8294=FACE_OUTER_BOUND ( 'NONE', #507, .T. ) ;
#8295=CARTESIAN_POINT ( 'NONE',  ( -4.458734124999999437, -83.64583333196773651, -2.574251347313719407 ) ) ;
#8298=CARTESIAN_POINT ( 'NONE',  ( -2.499999999999996447, 18.29166666939785202, 4.330127018922195425 ) ) ;
#8299=EDGE_LOOP ( 'NONE', ( #44587, #31261, #60241, #38502 ) ) ;
#8304=CARTESIAN_POINT ( 'NONE',  ( -2.499999999999996447, -30.83333333333333215, 4.330127018922195425 ) ) ;
#8305=CARTESIAN_POINT ( 'NONE',  ( -4.458734124999999437, -35.31249999863440792, 0.000000000000000000 ) ) ;
#8307=CARTESIAN_POINT ( 'NONE',  ( 5.000000000000000000, -30.29166666393548013, -2.886751345948129988 ) ) ;
#8308=CARTESIAN_POINT ( 'NONE',  ( 4.458734124999998549, -58.72916666530106511, -2.574251347313721627 ) ) ;
#8310=CARTESIAN_POINT ( 'NONE',  ( 1.339745962155615144, -62.58034179853028434, 4.999999999999999112 ) ) ;
#8312=CARTESIAN_POINT ( 'NONE',  ( -2.229367062500000163, -6.729166665301073103, -3.861377020970580443 ) ) ;
#8314=CARTESIAN_POINT ( 'NONE',  ( -5.000000000000000000, -78.00000000000000000, 0.000000000000000000 ) ) ;
#8318=CARTESIAN_POINT ( 'NONE',  ( -2.499999999999996447, -76.70833333060214443, 4.330127018922195425 ) ) ;
#8320=VECTOR ( 'NONE', #20232, 1000.000000000000000 ) ;
#8322=CARTESIAN_POINT ( 'NONE',  ( -2.229367062499996610, -22.39583333196773651, 3.861377020970582219 ) ) ;
#8323=CARTESIAN_POINT ( 'NONE',  ( -4.458734124999999437, -58.64583333196774362, -2.574251347313719407 ) ) ;
#8324=EDGE_LOOP ( 'NONE', ( #18507, #1669, #56165, #24416 ) ) ;
#8326=CARTESIAN_POINT ( 'NONE',  ( -3.152801135295367096, -169.3125000013656063, -3.152801135295367541 ) ) ;
#8336=CARTESIAN_POINT ( 'NONE',  ( -4.458734125000000326, -147.2500000013656063, -1.846868145590735644 ) ) ;
#8338=CARTESIAN_POINT ( 'NONE',  ( 0.000000000000000000, -170.0000000000000000, 5.000000000000000000 ) ) ;
#8340=CARTESIAN_POINT ( 'NONE',  ( 9.457646018065525792E-16, -69.31249999863440792, 5.148502694627439702 ) ) ;
#8343=CARTESIAN_POINT ( 'NONE',  ( -3.152801135295367096, -142.0625000013655779, -3.152801135295367541 ) ) ;
#8346=ORIENTED_EDGE ( 'NONE', *, *, #18460, .T. ) ;
#8347=CARTESIAN_POINT ( 'NONE',  ( -2.499999999999996447, -49.70833333060213732, 4.330127018922195425 ) ) ;
#8348=CYLINDRICAL_SURFACE ( 'NONE', #53566, 5.000000000000000000 ) ;
#8352=CARTESIAN_POINT ( 'NONE',  ( 2.229367062499998831, 28.10416666803225993, -3.861377020970580887 ) ) ;
#8353=DIRECTION ( 'NONE',  ( 0.000000000000000000, 0.000000000000000000, 1.000000000000000000 ) ) ;
#8358=CARTESIAN_POINT ( 'NONE',  ( -4.458734124999997661, 7.770833334698926009, 2.574251347313722516 ) ) ;
#8360=CARTESIAN_POINT ( 'NONE',  ( 2.229367062500001939, -19.22916666530106866, 3.861377020970579999 ) ) ;
#8362=CARTESIAN_POINT ( 'NONE',  ( 1.846868145590735200, -160.2500000013656063, -4.458734125000000326 ) ) ;
#8363=DIRECTION ( 'NONE',  ( -0.000000000000000000, 1.000000000000000000, -0.000000000000000000 ) ) ;
#8367=CARTESIAN_POINT ( 'NONE',  ( -2.229367062500000163, 29.52083333469892779, -3.861377020970580443 ) ) ;
#8368=CARTESIAN_POINT ( 'NONE',  ( 4.458734125000000326, -41.89583333196772941, 2.574251347313718519 ) ) ;
#8369=EDGE_CURVE ( 'NONE', #2611, #56591, #2862, .T. ) ;
#8372=CARTESIAN_POINT ( 'NONE',  ( -4.458734124999999437, -66.56249999863440792, 0.000000000000000000 ) ) ;
#8375=CARTESIAN_POINT ( 'NONE',  ( 5.000000000000000000, -89.50000000000000000, -6.123233995736766282E-16 ) ) ;
#8377=CARTESIAN_POINT ( 'NONE',  ( -1.339745962155610925, -84.79465819873851729, 5.000000000000000000 ) ) ;
#8378=CARTESIAN_POINT ( 'NONE',  ( 5.000000000000000888, -6.458333330602150646, 2.886751345948126879 ) ) ;
#8379=CARTESIAN_POINT ( 'NONE',  ( 5.000000000000000888, -12.58333333333333570, 2.886751345948126879 ) ) ;
#8380=CARTESIAN_POINT ( 'NONE',  ( 4.458734124999999437, -16.81249999863440436, -5.460374474430324690E-16 ) ) ;
#8381=ADVANCED_FACE ( 'NONE', ( #18644 ), #29220, .T. ) ;
#8382=CARTESIAN_POINT ( 'NONE',  ( 4.458734124999998549, -79.72916666530106511, -2.574251347313721627 ) ) ;
#8384=CARTESIAN_POINT ( 'NONE',  ( -4.999999999999999112, -10.79166666393547658, 2.886751345948131764 ) ) ;
#8385=CARTESIAN_POINT ( 'NONE',  ( 9.457646018065525792E-16, -46.06249999863440081, 5.148502694627439702 ) ) ;
#8386=EDGE_LOOP ( 'NONE', ( #30287, #34861, #16786, #58999 ) ) ;
#8387=CARTESIAN_POINT ( 'NONE',  ( -2.229367062500000163, 5.270833334698927786, -3.861377020970580443 ) ) ;
#8390=CARTESIAN_POINT ( 'NONE',  ( -2.499999999999996447, -61.83333333333333570, 4.330127018922195425 ) ) ;
#8392=CARTESIAN_POINT ( 'NONE',  ( -3.152801135295367096, -161.3125000013656063, -3.152801135295367541 ) ) ;
#8394=CARTESIAN_POINT ( 'NONE',  ( 5.000000000000000000, -14.49999999999999822, -6.123233995736766282E-16 ) ) ;
#8395=CARTESIAN_POINT ( 'NONE',  ( 9.457646018065525792E-16, -81.06249999863440792, 5.148502694627439702 ) ) ;
#8396=CARTESIAN_POINT ( 'NONE',  ( -5.000000000000000000, -164.5000000000000000, -6.123233995736766282E-16 ) ) ;
#8400=CARTESIAN_POINT ( 'NONE',  ( -4.458734124999999437, -3.645833331967739621, -2.574251347313719407 ) ) ;
#8401=CARTESIAN_POINT ( 'NONE',  ( -2.229367062499996610, -39.39583333196773651, 3.861377020970582219 ) ) ;
#8405=ORIENTED_EDGE ( 'NONE', *, *, #34651, .F. ) ;
#8408=CARTESIAN_POINT ( 'NONE',  ( 9.457646018065525792E-16, -69.31249999863440792, 5.148502694627439702 ) ) ;
#8409=CARTESIAN_POINT ( 'NONE',  ( -4.458734124999999437, -148.2500000013656347, -1.846868145590735644 ) ) ;
#8410=EDGE_LOOP ( 'NONE', ( #34007, #59252, #7370, #43942 ) ) ;
#8411=CYLINDRICAL_SURFACE ( 'NONE', #43103, 5.000000000000000000 ) ;
#8415=CARTESIAN_POINT ( 'NONE',  ( 9.457646018065525792E-16, -0.06249999863440491854, 5.148502694627439702 ) ) ;
#8416=CARTESIAN_POINT ( 'NONE',  ( -3.152801135295367096, -155.0625000013656063, -3.152801135295367541 ) ) ;
#8421=CARTESIAN_POINT ( 'NONE',  ( -6.972266317189433020E-16, -85.12499999726880162, -5.000000000000000000 ) ) ;
#8423=DIRECTION ( 'NONE',  ( -0.000000000000000000, 1.000000000000000000, -0.000000000000000000 ) ) ;
#8430=CARTESIAN_POINT ( 'NONE',  ( 5.000000000000000000, -10.50000000000000178, -6.123233995736766282E-16 ) ) ;
#8431=CARTESIAN_POINT ( 'NONE',  ( -4.458734124999999437, 20.60416666803225993, -2.574251347313719407 ) ) ;
#8433=CARTESIAN_POINT ( 'NONE',  ( 2.229367062500001939, -1.229166665301071548, 3.861377020970579999 ) ) ;
#8434=CARTESIAN_POINT ( 'NONE',  ( -5.000000000000000000, -63.08333333333331439, -2.886751345948128211 ) ) ;
#8436=CARTESIAN_POINT ( 'NONE',  ( 3.061616997868383141E-16, -142.8750000027312126, -5.000000000000000000 ) ) ;
#8443=( BOUNDED_CURVE ( )  B_SPLINE_CURVE ( 2, ( #44417, #39910, #45386, #5833, #54727, #35110, #60199, #6159, #16440 ),
 .UNSPECIFIED., .F., .F. ) 
 B_SPLINE_CURVE_WITH_KNOTS ( ( 3, 2, 2, 2, 3 ),
 ( 0.3145833333333333259, 0.3152777777777777679, 0.3166666666666666519, 0.3180555555555555358, 0.3187499999999999778 ),
 .UNSPECIFIED. ) 
 CURVE ( )  GEOMETRIC_REPRESENTATION_ITEM ( )  RATIONAL_B_SPLINE_CURVE ( ( 0.9330127018922194093, 0.9330127018922194093, 1.000000000000000000, 0.8660254037844387076, 1.000000000000000000, 0.8660254037844387076, 1.000000000000000000, 0.9330127018922194093, 0.9330127018922194093 ) ) 
 REPRESENTATION_ITEM ( '' )  );
#8445=CARTESIAN_POINT ( 'NONE',  ( 2.730187237215162345E-16, -156.4375000013655779, -4.458734124999999437 ) ) ;
#8447=DIRECTION ( 'NONE',  ( -0.000000000000000000, 1.000000000000000000, -0.000000000000000000 ) ) ;
#8449=CARTESIAN_POINT ( 'NONE',  ( -4.458734124999998549, 16.52083333469892779, 2.574251347313722516 ) ) ;
#8450=VERTEX_POINT ( 'NONE', #60436 ) ;
#8455=CARTESIAN_POINT ( 'NONE',  ( 5.000000000000000000, 4.500000000000000888, -6.123233995736766282E-16 ) ) ;
#8456=CARTESIAN_POINT ( 'NONE',  ( -4.458734124999997661, -61.22916666530106511, 2.574251347313722516 ) ) ;
#8458=CARTESIAN_POINT ( 'NONE',  ( 9.457646018065525792E-16, -28.06249999863440081, 5.148502694627439702 ) ) ;
#8459=CARTESIAN_POINT ( 'NONE',  ( 5.000000000000000000, 7.708333336064518093, -2.886751345948130876 ) ) ;
#8461=CARTESIAN_POINT ( 'NONE',  ( -3.535250795749689387E-16, -46.25000000000000000, -5.773502691896257311 ) ) ;
#8463=CARTESIAN_POINT ( 'NONE',  ( 1.339745962155661996, -26.16965819600733667, -4.999999999999970690 ) ) ;
#8465=DIRECTION ( 'NONE',  ( 0.000000000000000000, 0.000000000000000000, 1.000000000000000000 ) ) ;
#8466=CARTESIAN_POINT ( 'NONE',  ( -4.458734124999999437, -63.31249999863440792, 0.000000000000000000 ) ) ;
#8467=CARTESIAN_POINT ( 'NONE',  ( -3.152801135295367985, -147.0625000013655779, 3.152801135295367096 ) ) ;
#8468=CARTESIAN_POINT ( 'NONE',  ( -4.458734124999998549, -74.22916666530106511, 2.574251347313722516 ) ) ;
#8470=CARTESIAN_POINT ( 'NONE',  ( -3.152548672688508926E-16, -23.81249999863440792, -5.148502694627439702 ) ) ;
#8471=CARTESIAN_POINT ( 'NONE',  ( 5.000000000000000888, -67.45833333060213022, 2.886751345948126879 ) ) ;
#8472=ORIENTED_EDGE ( 'NONE', *, *, #10072, .F. ) ;
#8476=CARTESIAN_POINT ( 'NONE',  ( 1.975475456537005874E-15, -21.62499999726880873, 5.000000000000000000 ) ) ;
#8478=CARTESIAN_POINT ( 'NONE',  ( 0.000000000000000000, -170.0000000000000000, 0.000000000000000000 ) ) ;
#8479=CARTESIAN_POINT ( 'NONE',  ( 4.458734124999999437, -53.06249999863440792, -5.460374474430324690E-16 ) ) ;
#8481=ORIENTED_EDGE ( 'NONE', *, *, #62538, .F. ) ;
#8484=CARTESIAN_POINT ( 'NONE',  ( -4.458734124999999437, 18.68750000136559564, 0.000000000000000000 ) ) ;
#8487=CARTESIAN_POINT ( 'NONE',  ( -9.184850993605147944E-16, -148.2500000000000284, 5.000000000000000000 ) ) ;
#8489=ORIENTED_EDGE ( 'NONE', *, *, #16582, .T. ) ;
#8491=CARTESIAN_POINT ( 'NONE',  ( -2.500000000000000444, -40.16666666666667140, -4.330127018922193649 ) ) ;
#8498=CARTESIAN_POINT ( 'NONE',  ( 6.123233995736766282E-16, -170.0000000000000000, -5.000000000000000000 ) ) ;
#8499=FACE_OUTER_BOUND ( 'NONE', #46368, .T. ) ;
#8500=CARTESIAN_POINT ( 'NONE',  ( -5.000000000000000888, -159.4375000000000000, 2.071067811865474617 ) ) ;
#8503=DIRECTION ( 'NONE',  ( 0.000000000000000000, 0.000000000000000000, 1.000000000000000000 ) ) ;
#8505=CARTESIAN_POINT ( 'NONE',  ( 3.535533905932736864, -152.2500000027312126, 3.535533905932738641 ) ) ;
#8511=CARTESIAN_POINT ( 'NONE',  ( 5.000000000000000888, -147.9374999999999716, -2.071067811865475505 ) ) ;
#8514=CARTESIAN_POINT ( 'NONE',  ( 1.255007937094098239E-14, 22.87500000273118772, -4.999999999999999112 ) ) ;
#8515=CARTESIAN_POINT ( 'NONE',  ( -3.152548672688508926E-16, -28.56249999863440081, -5.148502694627439702 ) ) ;
#8517=CARTESIAN_POINT ( 'NONE',  ( 1.975475456537005874E-15, 9.375000002731185944, 5.000000000000000000 ) ) ;
#8519=CARTESIAN_POINT ( 'NONE',  ( -1.846868145590737420, -149.7500000013656063, 4.458734124999999437 ) ) ;
#8522=CARTESIAN_POINT ( 'NONE',  ( -3.152548672688508926E-16, -58.81249999863440081, -5.148502694627439702 ) ) ;
#8523=( BOUNDED_CURVE ( )  B_SPLINE_CURVE ( 2, ( #59796, #15717, #35336, #10885, #41420, #16673, #12159, #26640, #11831 ),
 .UNSPECIFIED., .F., .F. ) 
 B_SPLINE_CURVE_WITH_KNOTS ( ( 3, 2, 2, 2, 3 ),
 ( 0.7749999999999998002, 0.7791666666666664520, 0.7833333333333331039, 0.7874999999999997558, 0.7916666666666664076 ),
 .UNSPECIFIED. ) 
 CURVE ( )  GEOMETRIC_REPRESENTATION_ITEM ( )  RATIONAL_B_SPLINE_CURVE ( ( 1.000000000000003997, 0.9238795325112826307, 1.000000000000000000, 0.9238795325112867385, 1.000000000000000000, 0.9238795325112867385, 1.000000000000000000, 0.9238795325112908463, 0.9999999999999958922 ) ) 
 REPRESENTATION_ITEM ( '' )  );
#8525=LINE ( 'NONE', #17856, #20668 ) ;
#8526=CARTESIAN_POINT ( 'NONE',  ( -4.999999999999999112, 20.08333333333333215, 2.886751345948131764 ) ) ;
#8527=LINE ( 'NONE', #14595, #49941 ) ;
#8528=CARTESIAN_POINT ( 'NONE',  ( 2.229367062499998831, 1.354166668032261933, -3.861377020970580887 ) ) ;
#8529=CARTESIAN_POINT ( 'NONE',  ( 1.975475456537005874E-15, -10.75000000000000000, 5.000000000000000000 ) ) ;
#8530=CYLINDRICAL_SURFACE ( 'NONE', #11199, 5.000000000000000000 ) ;
#8531=CARTESIAN_POINT ( 'NONE',  ( -2.229367062500000163, 9.270833334698927786, -3.861377020970580443 ) ) ;
#8535=CARTESIAN_POINT ( 'NONE',  ( 5.000000000000000888, -7.458333330602142652, 2.886751345948126879 ) ) ;
#8536=CARTESIAN_POINT ( 'NONE',  ( 2.229367062500001939, -48.97916666530107221, 3.861377020970579999 ) ) ;
#8537=CARTESIAN_POINT ( 'NONE',  ( 4.458734124999999437, -160.6875000013655779, 0.000000000000000000 ) ) ;
#8538=CARTESIAN_POINT ( 'NONE',  ( 1.060575238724906964E-15, -51.62499999726881583, 5.773502691896257311 ) ) ;
#8540=CARTESIAN_POINT ( 'NONE',  ( 4.458734124999999437, -20.81249999863440081, -5.460374474430324690E-16 ) ) ;
#8541=VERTEX_POINT ( 'NONE', #15405 ) ;
#8544=CARTESIAN_POINT ( 'NONE',  ( 3.152801135295366208, -161.5625000013656063, 3.152801135295367985 ) ) ;
#8545=CARTESIAN_POINT ( 'NONE',  ( -6.972266317189433020E-16, -39.12499999726880162, -5.000000000000000000 ) ) ;
#8547=CARTESIAN_POINT ( 'NONE',  ( 2.229367062500001939, -36.22916666530107221, 3.861377020970579999 ) ) ;
#8548=ORIENTED_EDGE ( 'NONE', *, *, #51420, .T. ) ;
#8554=CARTESIAN_POINT ( 'NONE',  ( 4.458734125000001214, -86.14583333196775072, 2.574251347313718519 ) ) ;
#8557=CARTESIAN_POINT ( 'NONE',  ( -4.458734124999999437, -140.2500000013656063, -1.846868145590735644 ) ) ;
#8558=CARTESIAN_POINT ( 'NONE',  ( 5.000000000000000888, -57.58333333333332860, 2.886751345948126879 ) ) ;
#8562=ADVANCED_FACE ( 'NONE', ( #40156 ), #60114, .T. ) ;
#8563=DIRECTION ( 'NONE',  ( -0.000000000000000000, 1.000000000000000000, -0.000000000000000000 ) ) ;
#8569=CARTESIAN_POINT ( 'NONE',  ( 4.458734124999999437, -87.06249999863439371, -5.460374474430324690E-16 ) ) ;
#8573=CARTESIAN_POINT ( 'NONE',  ( -2.499999999999996447, -16.70833333060214443, 4.330127018922195425 ) ) ;
#8575=CARTESIAN_POINT ( 'NONE',  ( 2.071067811865476394, -166.3125000027312410, 5.000000000000000000 ) ) ;
#8578=CARTESIAN_POINT ( 'NONE',  ( -2.500000000000000444, -30.16666666666666785, -4.330127018922193649 ) ) ;
#8585=CARTESIAN_POINT ( 'NONE',  ( 1.975475456537005874E-15, -86.62499999726880162, 5.000000000000000000 ) ) ;
#8586=CARTESIAN_POINT ( 'NONE',  ( -9.184850993605147944E-16, -152.2500000000000000, 5.000000000000000000 ) ) ;
#8587=CARTESIAN_POINT ( 'NONE',  ( 2.229367062500001939, -13.97916666530107221, 3.861377020970579999 ) ) ;
#8588=CYLINDRICAL_SURFACE ( 'NONE', #36041, 5.000000000000000000 ) ;
#8590=CARTESIAN_POINT ( 'NONE',  ( -4.458734124999999437, -39.64583333196773651, -2.574251347313719407 ) ) ;
#8592=CYLINDRICAL_SURFACE ( 'NONE', #41772, 5.000000000000000000 ) ;
#8593=CARTESIAN_POINT ( 'NONE',  ( -6.972266317189433020E-16, -28.25000000000000000, -5.000000000000000000 ) ) ;
#8597=CARTESIAN_POINT ( 'NONE',  ( 2.229367062499998831, 16.35416666803225993, -3.861377020970580887 ) ) ;
#8599=CARTESIAN_POINT ( 'NONE',  ( -2.499999999999996447, -64.70833333060213022, 4.330127018922195425 ) ) ;
#8600=CARTESIAN_POINT ( 'NONE',  ( 4.458734125000000326, -84.14583333196773651, 2.574251347313718519 ) ) ;
#8602=CARTESIAN_POINT ( 'NONE',  ( -2.499999999999996447, 13.29166666939785379, 4.330127018922195425 ) ) ;
#8603=VERTEX_POINT ( 'NONE', #26321 ) ;
#8604=CARTESIAN_POINT ( 'NONE',  ( 1.339745962155661996, -25.29465819873852794, -4.999999999999970690 ) ) ;
#8605=CARTESIAN_POINT ( 'NONE',  ( -2.498395430326213474E-14, 16.24999999999999645, 5.000000000000000000 ) ) ;
#8607=CARTESIAN_POINT ( 'NONE',  ( 2.499999999999998668, -30.33333333333332860, -4.330127018922193649 ) ) ;
#8608=CARTESIAN_POINT ( 'NONE',  ( -4.458734124999999437, -30.31249999863440436, 0.000000000000000000 ) ) ;
#8609=DIRECTION ( 'NONE',  ( 0.000000000000000000, 0.000000000000000000, 1.000000000000000000 ) ) ;
#8611=CARTESIAN_POINT ( 'NONE',  ( -4.999999999999999112, -32.79166666393547303, 2.886751345948131764 ) ) ;
#8613=CARTESIAN_POINT ( 'NONE',  ( 9.457646018065525792E-16, -61.06249999863440081, 5.148502694627439702 ) ) ;
#8614=ORIENTED_EDGE ( 'NONE', *, *, #449, .F. ) ;
#8616=CARTESIAN_POINT ( 'NONE',  ( -4.458734124999999437, -7.562499998634404363, 0.000000000000000000 ) ) ;
#8617=VERTEX_POINT ( 'NONE', #20872 ) ;
#8618=CARTESIAN_POINT ( 'NONE',  ( 5.000000000000000000, -75.41666666666667140, -2.886751345948129988 ) ) ;
#8621=CARTESIAN_POINT ( 'NONE',  ( 5.000000000000000888, -74.45833333060214443, 2.886751345948126879 ) ) ;
#8622=CARTESIAN_POINT ( 'NONE',  ( 6.123233995736766282E-16, -170.0000000000000000, -5.000000000000000000 ) ) ;
#8625=CARTESIAN_POINT ( 'NONE',  ( 2.229367062500001939, -23.22916666530107221, 3.861377020970579999 ) ) ;
#8626=CARTESIAN_POINT ( 'NONE',  ( 2.229367062499998831, -56.89583333196773651, -3.861377020970580887 ) ) ;
#8628=CARTESIAN_POINT ( 'NONE',  ( -1.846868145590737420, -167.0000000013655779, 4.458734124999999437 ) ) ;
#8630=CARTESIAN_POINT ( 'NONE',  ( -2.071067811865459518, -167.4375000027312126, 5.000000000000019540 ) ) ;
#8631=ORIENTED_EDGE ( 'NONE', *, *, #61486, .T. ) ;
#8635=EDGE_CURVE ( 'NONE', #45572, #20487, #59586, .T. ) ;
#8638=CARTESIAN_POINT ( 'NONE',  ( 4.458734125000000326, -144.6250000013655779, -1.846868145590734978 ) ) ;
#8640=CARTESIAN_POINT ( 'NONE',  ( 6.123233995736766282E-16, -170.0000000000000000, -5.000000000000000000 ) ) ;
#8642=CARTESIAN_POINT ( 'NONE',  ( -4.458734124999999437, -70.64583333196773651, -2.574251347313719407 ) ) ;
#8645=CARTESIAN_POINT ( 'NONE',  ( -1.846868145590737420, -141.7500000013655779, 4.458734124999997661 ) ) ;
#8654=CARTESIAN_POINT ( 'NONE',  ( -4.458734124999999437, 23.43750000136559564, 0.000000000000000000 ) ) ;
#8662=CARTESIAN_POINT ( 'NONE',  ( 9.457646018065525792E-16, 4.937500001365595637, 5.148502694627439702 ) ) ;
#8664=CARTESIAN_POINT ( 'NONE',  ( -2.229367062500000163, -25.72916666530106866, -3.861377020970580443 ) ) ;
#8666=CARTESIAN_POINT ( 'NONE',  ( 1.846868145590735200, -157.2500000013656063, -4.458734125000000326 ) ) ;
#8670=CARTESIAN_POINT ( 'NONE',  ( 2.229367062499998831, -39.64583333196773651, -3.861377020970580887 ) ) ;
#8671=CARTESIAN_POINT ( 'NONE',  ( -1.339745962155610925, -83.79465819873851729, 5.000000000000000000 ) ) ;
#8673=CARTESIAN_POINT ( 'NONE',  ( 2.229367062500001939, -69.22916666530107932, 3.861377020970579999 ) ) ;
#8676=CYLINDRICAL_SURFACE ( 'NONE', #15054, 5.000000000000000000 ) ;
#8679=CARTESIAN_POINT ( 'NONE',  ( -5.147856630858197489E-14, 2.375000002731183724, 5.000000000000000000 ) ) ;
#8680=CARTESIAN_POINT ( 'NONE',  ( 5.000000000000000000, -15.50000000000000000, -6.123233995736766282E-16 ) ) ;
#8681=CARTESIAN_POINT ( 'NONE',  ( 4.458734125000001214, -18.89583333196773651, 2.574251347313718519 ) ) ;
#8682=EDGE_CURVE ( 'NONE', #54505, #38362, #17307, .T. ) ;
#8683=CARTESIAN_POINT ( 'NONE',  ( 4.458734125000000326, -78.89583333196775072, 2.574251347313718519 ) ) ;
#8684=CARTESIAN_POINT ( 'NONE',  ( -6.972266317189433020E-16, -59.12499999726880873, -5.000000000000000000 ) ) ;
#8685=CARTESIAN_POINT ( 'NONE',  ( 2.499999999999998668, -14.20833333060214976, -4.330127018922193649 ) ) ;
#8686=CARTESIAN_POINT ( 'NONE',  ( 4.458734125000001214, -46.89583333196773651, 2.574251347313718519 ) ) ;
#8687=VERTEX_POINT ( 'NONE', #12480 ) ;
#8689=CARTESIAN_POINT ( 'NONE',  ( 4.458734125000001214, 6.854166668032259935, 2.574251347313718519 ) ) ;
#8692=CARTESIAN_POINT ( 'NONE',  ( 1.060575238724906964E-15, -58.75000000000000000, 5.773502691896257311 ) ) ;
#8693=CARTESIAN_POINT ( 'NONE',  ( -4.458734124999999437, -156.1875000013655779, -5.460374474430324690E-16 ) ) ;
#8696=CARTESIAN_POINT ( 'NONE',  ( -5.000000000000000888, -166.4375000000000568, 2.071067811865474617 ) ) ;
#8697=CARTESIAN_POINT ( 'NONE',  ( 5.000000000000000000, -168.0000000000000000, 0.000000000000000000 ) ) ;
#8699=CARTESIAN_POINT ( 'NONE',  ( 4.458734124999998549, -7.979166665301073991, -2.574251347313721627 ) ) ;
#8700=CARTESIAN_POINT ( 'NONE',  ( 2.229367062499998831, -41.89583333196773651, -3.861377020970580887 ) ) ;
#8702=CARTESIAN_POINT ( 'NONE',  ( -4.458734125000000326, -154.0000000013655779, -1.846868145590735644 ) ) ;
#8705=ORIENTED_EDGE ( 'NONE', *, *, #46518, .F. ) ;
#8709=CARTESIAN_POINT ( 'NONE',  ( 4.458734124999998549, -69.97916666530107932, -2.574251347313721627 ) ) ;
#8710=CARTESIAN_POINT ( 'NONE',  ( -4.458734124999999437, -145.1875000013656063, -5.460374474430324690E-16 ) ) ;
#8711=ORIENTED_EDGE ( 'NONE', *, *, #8292, .F. ) ;
#8714=CYLINDRICAL_SURFACE ( 'NONE', #32894, 5.000000000000000000 ) ;
#8717=CARTESIAN_POINT ( 'NONE',  ( 1.975475456537005874E-15, 17.25000000000000000, 5.000000000000000000 ) ) ;
#8718=CARTESIAN_POINT ( 'NONE',  ( -2.229367062500000163, 4.520833334698926897, -3.861377020970580443 ) ) ;
#8719=CARTESIAN_POINT ( 'NONE',  ( -5.000000000000000000, -80.08333333333332860, -2.886751345948128211 ) ) ;
#8720=CARTESIAN_POINT ( 'NONE',  ( 2.730187237215162345E-16, -152.1875000013656063, -4.458734124999999437 ) ) ;
#8728=EDGE_CURVE ( 'NONE', #7140, #60995, #3160, .T. ) ;
#8729=CARTESIAN_POINT ( 'NONE',  ( 1.975475456537005874E-15, -37.74999999999999289, 5.000000000000000000 ) ) ;
#8738=CARTESIAN_POINT ( 'NONE',  ( 2.229367062499998831, 24.35416666803225993, -3.861377020970580887 ) ) ;
#8739=EDGE_CURVE ( 'NONE', #13144, #55337, #15615, .T. ) ;
#8741=CARTESIAN_POINT ( 'NONE',  ( -2.229367062499996610, -3.395833331967738733, 3.861377020970582219 ) ) ;
#8743=EDGE_CURVE ( 'NONE', #7560, #14071, #5286, .T. ) ;
#8744=CARTESIAN_POINT ( 'NONE',  ( -3.535533905932737309, -140.7500000027311842, -3.535533905932738197 ) ) ;
#8753=CARTESIAN_POINT ( 'NONE',  ( 4.458734124999999437, -158.6875000013655779, 0.000000000000000000 ) ) ;
#8756=CARTESIAN_POINT ( 'NONE',  ( -4.458734124999999437, 16.35416666803225993, -2.574251347313719407 ) ) ;
#8757=ORIENTED_EDGE ( 'NONE', *, *, #34543, .F. ) ;
#8761=CARTESIAN_POINT ( 'NONE',  ( 1.975475456537005874E-15, 7.249999999999998224, 5.000000000000000000 ) ) ;
#8762=CARTESIAN_POINT ( 'NONE',  ( -2.499999999999996447, 4.166666666666666075, 4.330127018922195425 ) ) ;
#8763=CARTESIAN_POINT ( 'NONE',  ( 4.458734124999999437, -60.81249999863440081, -5.460374474430324690E-16 ) ) ;
#8765=CARTESIAN_POINT ( 'NONE',  ( -5.000000000000000000, 2.125000002731185056, 0.000000000000000000 ) ) ;
#8766=CARTESIAN_POINT ( 'NONE',  ( -4.458734124999999437, -27.39583333196773651, -2.574251347313719407 ) ) ;
#8769=DIRECTION ( 'NONE',  ( -0.000000000000000000, 1.000000000000000000, -0.000000000000000000 ) ) ;
#8770=CARTESIAN_POINT ( 'NONE',  ( 5.000000000000000888, -43.58333333333333570, 2.886751345948126879 ) ) ;
#8773=CARTESIAN_POINT ( 'NONE',  ( -6.972266317189433020E-16, -64.24999999999998579, -5.000000000000000000 ) ) ;
#8774=CARTESIAN_POINT ( 'NONE',  ( -2.229367062500000163, -66.47916666530106511, -3.861377020970580443 ) ) ;
#8775=CARTESIAN_POINT ( 'NONE',  ( -4.458734124999999437, -146.1875000013656063, -5.460374474430324690E-16 ) ) ;
#8776=CARTESIAN_POINT ( 'NONE',  ( -4.458734124999998549, -78.22916666530106511, 2.574251347313722516 ) ) ;
#8778=CARTESIAN_POINT ( 'NONE',  ( 9.457646018065525792E-16, -27.31249999863440436, 5.148502694627439702 ) ) ;
#8779=CARTESIAN_POINT ( 'NONE',  ( 5.000000000000000888, -65.45833333060214443, 2.886751345948126879 ) ) ;
#8780=ORIENTED_EDGE ( 'NONE', *, *, #35360, .F. ) ;
#8781=CARTESIAN_POINT ( 'NONE',  ( 1.339745962155612702, -1.294658198738520172, -5.000000000000000000 ) ) ;
#8782=ORIENTED_EDGE ( 'NONE', *, *, #37063, .T. ) ;
#8784=LINE ( 'NONE', #13614, #58446 ) ;
#8787=FACE_OUTER_BOUND ( 'NONE', #46513, .T. ) ;
#8788=CARTESIAN_POINT ( 'NONE',  ( 2.229367062499998831, -52.89583333196773651, -3.861377020970580887 ) ) ;
#8790=ORIENTED_EDGE ( 'NONE', *, *, #27471, .F. ) ;
#8794=CARTESIAN_POINT ( 'NONE',  ( 4.458734124999998549, 16.27083333469892779, -2.574251347313721627 ) ) ;
#8797=CARTESIAN_POINT ( 'NONE',  ( 1.846868145590736310, -166.6250000013656063, 4.458734124999997661 ) ) ;
#8800=DIRECTION ( 'NONE',  ( -0.000000000000000000, 1.000000000000000000, -0.000000000000000000 ) ) ;
#8802=( BOUNDED_CURVE ( )  B_SPLINE_CURVE ( 2, ( #22383, #9768, #23947, #49336, #34524, #465, #30345, #44501, #4327 ),
 .UNSPECIFIED., .F., .F. ) 
 B_SPLINE_CURVE_WITH_KNOTS ( ( 3, 2, 2, 2, 3 ),
 ( 0.2062499999999999889, 0.2069444444444444309, 0.2083333333333333426, 0.2097222222222222265, 0.2104166666666666685 ),
 .UNSPECIFIED. ) 
 CURVE ( )  GEOMETRIC_REPRESENTATION_ITEM ( )  RATIONAL_B_SPLINE_CURVE ( ( 0.9330127018922194093, 0.9330127018922194093, 1.000000000000000000, 0.8660254037844387076, 1.000000000000000000, 0.8660254037844387076, 1.000000000000000000, 0.9330127018922194093, 0.9330127018922194093 ) ) 
 REPRESENTATION_ITEM ( '' )  );
#8803=CARTESIAN_POINT ( 'NONE',  ( -5.000000000000000000, -162.6250000027311842, -6.123233995736766282E-16 ) ) ;
#8806=CARTESIAN_POINT ( 'NONE',  ( 1.975475456537005874E-15, 1.375000002731185500, 5.000000000000000000 ) ) ;
#8810=DIRECTION ( 'NONE',  ( -0.000000000000000000, 1.000000000000000000, -0.000000000000000000 ) ) ;
#8811=EDGE_CURVE ( 'NONE', #13416, #59564, #409, .T. ) ;
#8816=CARTESIAN_POINT ( 'NONE',  ( -2.071067811865475061, -153.8125000027311842, -5.000000000000000888 ) ) ;
#8823=CARTESIAN_POINT ( 'NONE',  ( 5.000000000000000000, -141.0625000000000000, 2.071067811865478614 ) ) ;
#8824=EDGE_CURVE ( 'NONE', #46916, #53830, #13555, .T. ) ;
#8827=CARTESIAN_POINT ( 'NONE',  ( 5.000000000000000888, 22.54166666939785202, 2.886751345948126879 ) ) ;
#8828=CARTESIAN_POINT ( 'NONE',  ( -2.229367062500000163, -30.47916666530107221, -3.861377020970580443 ) ) ;
#8832=CARTESIAN_POINT ( 'NONE',  ( -3.152801135295367096, -146.0625000013655779, -3.152801135295367541 ) ) ;
#8833=ORIENTED_EDGE ( 'NONE', *, *, #9370, .T. ) ;
#8835=CARTESIAN_POINT ( 'NONE',  ( 9.457646018065525792E-16, -59.31249999863440081, 5.148502694627439702 ) ) ;
#8837=CARTESIAN_POINT ( 'NONE',  ( -5.000000000000000000, -162.5000000000000000, -6.123233995736766282E-16 ) ) ;
#8838=CARTESIAN_POINT ( 'NONE',  ( 5.000000000000000888, 20.41666666666666430, 2.886751345948126879 ) ) ;
#8840=CARTESIAN_POINT ( 'NONE',  ( -3.152548672688508926E-16, -2.562499998634407028, -5.148502694627439702 ) ) ;
#8843=CARTESIAN_POINT ( 'NONE',  ( 9.457646018065525792E-16, 12.68750000136559208, 5.148502694627439702 ) ) ;
#8847=CARTESIAN_POINT ( 'NONE',  ( -2.229367062500000163, -51.47916666530107221, -3.861377020970580443 ) ) ;
#8848=CARTESIAN_POINT ( 'NONE',  ( 3.152801135295367541, -161.5625000013656063, -3.152801135295367541 ) ) ;
#8849=CARTESIAN_POINT ( 'NONE',  ( -2.499999999999996447, -47.70833333060215153, 4.330127018922195425 ) ) ;
#8851=CARTESIAN_POINT ( 'NONE',  ( -4.458734124999999437, -23.31249999863440436, 0.000000000000000000 ) ) ;
#8852=ORIENTED_EDGE ( 'NONE', *, *, #52242, .T. ) ;
#8854=CARTESIAN_POINT ( 'NONE',  ( -4.458734125000000326, -162.0000000013655779, -1.846868145590735644 ) ) ;
#8855=VERTEX_POINT ( 'NONE', #55493 ) ;
#8856=( BOUNDED_CURVE ( )  B_SPLINE_CURVE ( 2, ( #18237, #13721, #62938, #37861, #9211, #57494, #33034, #52650, #8585 ),
 .UNSPECIFIED., .F., .F. ) 
 B_SPLINE_CURVE_WITH_KNOTS ( ( 3, 2, 2, 2, 3 ),
 ( 0.9604166666666666963, 0.9611111111111111382, 0.9625000000000000222, 0.9638888888888889062, 0.9645833333333333481 ),
 .UNSPECIFIED. ) 
 CURVE ( )  GEOMETRIC_REPRESENTATION_ITEM ( )  RATIONAL_B_SPLINE_CURVE ( ( 0.9330127018922194093, 0.9330127018922194093, 1.000000000000000000, 0.8660254037844387076, 1.000000000000000000, 0.8660254037844387076, 1.000000000000000000, 0.9330127018922194093, 0.9330127018922194093 ) ) 
 REPRESENTATION_ITEM ( '' )  );
#8857=VECTOR ( 'NONE', #46815, 1000.000000000000000 ) ;
#8858=CARTESIAN_POINT ( 'NONE',  ( 1.975475456537005874E-15, -39.62499999726880162, 5.000000000000000000 ) ) ;
#8860=CARTESIAN_POINT ( 'NONE',  ( -4.458734124999998549, -36.47916666530107221, 2.574251347313722516 ) ) ;
#8861=VECTOR ( 'NONE', #26646, 1000.000000000000000 ) ;
#8866=VERTEX_POINT ( 'NONE', #21070 ) ;
#8868=CARTESIAN_POINT ( 'NONE',  ( 2.229367062499998831, -86.89583333196773651, -3.861377020970580887 ) ) ;
#8871=CARTESIAN_POINT ( 'NONE',  ( -1.339745962155613812, -7.205341801261479162, -5.000000000000000000 ) ) ;
#8872=CARTESIAN_POINT ( 'NONE',  ( 1.975475456537005874E-15, -46.62499999726880873, 5.000000000000000000 ) ) ;
#8874=CARTESIAN_POINT ( 'NONE',  ( 2.499999999999998668, -37.33333333333332860, -4.330127018922193649 ) ) ;
#8880=DIRECTION ( 'NONE',  ( -0.000000000000000000, 1.000000000000000000, -0.000000000000000000 ) ) ;
#8881=CARTESIAN_POINT ( 'NONE',  ( -5.000000000000000000, -61.08333333333333570, -2.886751345948128211 ) ) ;
#8882=CARTESIAN_POINT ( 'NONE',  ( 4.458734124999998549, -84.97916666530106511, -2.574251347313721627 ) ) ;
#8884=( BOUNDED_CURVE ( )  B_SPLINE_CURVE ( 2, ( #44580, #5032, #48461, #9538, #38795, #40071, #54234, #14671, #5355 ),
 .UNSPECIFIED., .F., .F. ) 
 B_SPLINE_CURVE_WITH_KNOTS ( ( 3, 2, 2, 2, 3 ),
 ( 0.1083333333333334203, 0.1125000000000000999, 0.1166666666666667657, 0.1208333333333334314, 0.1250000000000001110 ),
 .UNSPECIFIED. ) 
 CURVE ( )  GEOMETRIC_REPRESENTATION_ITEM ( )  RATIONAL_B_SPLINE_CURVE ( ( 0.9999999999999984457, 0.9238795325112882928, 1.000000000000000000, 0.9238795325112867385, 1.000000000000000000, 0.9238795325112867385, 1.000000000000000000, 0.9238795325112847401, 1.000000000000001998 ) ) 
 REPRESENTATION_ITEM ( '' )  );
#8889=CARTESIAN_POINT ( 'NONE',  ( 3.061616997868383141E-16, -164.8750000027311842, -5.000000000000000000 ) ) ;
#8892=CARTESIAN_POINT ( 'NONE',  ( -6.972266317189433020E-16, -30.25000000000000000, -5.000000000000000000 ) ) ;
#8898=CARTESIAN_POINT ( 'NONE',  ( -4.999999999999998224, -19.91666666666666430, 2.886751345948131764 ) ) ;
#8899=CARTESIAN_POINT ( 'NONE',  ( 4.458734124999999437, -12.81249999863440259, -5.460374474430324690E-16 ) ) ;
#8900=CYLINDRICAL_SURFACE ( 'NONE', #6415, 5.000000000000000000 ) ;
#8902=CARTESIAN_POINT ( 'NONE',  ( 4.458734124999999437, -43.06249999863440081, -5.460374474430324690E-16 ) ) ;
#8904=CARTESIAN_POINT ( 'NONE',  ( 5.000000000000000000, -83.29166666393547303, -2.886751345948130876 ) ) ;
#8909=AXIS2_PLACEMENT_3D ( 'NONE', #41908, #17487, #12958 ) ;
#8911=CARTESIAN_POINT ( 'NONE',  ( -4.458734124999998549, 13.77083333469892779, 2.574251347313722516 ) ) ;
#8914=CARTESIAN_POINT ( 'NONE',  ( 1.975475456537005874E-15, -64.62499999726880162, 5.000000000000000000 ) ) ;
#8915=CARTESIAN_POINT ( 'NONE',  ( 4.458734124999999437, -88.06249999863439371, -5.460374474430324690E-16 ) ) ;
#8917=CARTESIAN_POINT ( 'NONE',  ( -2.500000000000000444, 11.95833333606451809, -4.330127018922193649 ) ) ;
#8920=CYLINDRICAL_SURFACE ( 'NONE', #11423, 5.000000000000000000 ) ;
#8921=CARTESIAN_POINT ( 'NONE',  ( 5.000000000000000000, -29.50000000000000000, -6.123233995736766282E-16 ) ) ;
#8922=CARTESIAN_POINT ( 'NONE',  ( 4.458734124999999437, -30.81249999863440436, -5.460374474430324690E-16 ) ) ;
#8924=CARTESIAN_POINT ( 'NONE',  ( -2.499999999999996447, -35.70833333060213732, 4.330127018922195425 ) ) ;
#8925=CARTESIAN_POINT ( 'NONE',  ( 4.458734125000001214, -62.89583333196775072, 2.574251347313718519 ) ) ;
#8926=ORIENTED_EDGE ( 'NONE', *, *, #10765, .F. ) ;
#8928=CARTESIAN_POINT ( 'NONE',  ( -2.229367062500000163, -11.72916666530107044, -3.861377020970580443 ) ) ;
#8929=ORIENTED_EDGE ( 'NONE', *, *, #12668, .T. ) ;
#8930=CARTESIAN_POINT ( 'NONE',  ( 5.000000000000000888, -74.58333333333332860, 2.886751345948126879 ) ) ;
#8933=CARTESIAN_POINT ( 'NONE',  ( -5.000000000000000000, -80.87499999726881583, 0.000000000000000000 ) ) ;
#8937=CARTESIAN_POINT ( 'NONE',  ( 4.458734124999999437, -21.06249999863440436, -5.460374474430324690E-16 ) ) ;
#8938=CARTESIAN_POINT ( 'NONE',  ( 4.458734125000001214, -57.14583333196773651, 2.574251347313718519 ) ) ;
#8939=EDGE_LOOP ( 'NONE', ( #25843, #807, #15291, #7817 ) ) ;
#8940=CARTESIAN_POINT ( 'NONE',  ( 4.458734124999999437, -168.6875000013656063, 0.000000000000000000 ) ) ;
#8942=CARTESIAN_POINT ( 'NONE',  ( -2.071067811865491493, -167.8125000027311842, -4.999999999999985789 ) ) ;
#8943=ORIENTED_EDGE ( 'NONE', *, *, #1200, .F. ) ;
#8947=AXIS2_PLACEMENT_3D ( 'NONE', #27536, #2793, #61651 ) ;
#8949=AXIS2_PLACEMENT_3D ( 'NONE', #56709, #3311, #37706 ) ;
#8953=CARTESIAN_POINT ( 'NONE',  ( 4.458734124999999437, -143.7500000013655779, 1.846868145590737864 ) ) ;
#8958=CARTESIAN_POINT ( 'NONE',  ( -4.458734124999999437, -66.64583333196773651, -2.574251347313719407 ) ) ;
#8961=CARTESIAN_POINT ( 'NONE',  ( 3.152801135295366208, -141.5625000013655779, 3.152801135295367985 ) ) ;
#8963=VERTEX_POINT ( 'NONE', #26530 ) ;
#8968=CARTESIAN_POINT ( 'NONE',  ( 1.339745962155615144, -14.58034179853029322, 4.999999999999999112 ) ) ;
#8970=CARTESIAN_POINT ( 'NONE',  ( -4.458734124999997661, 21.52083333469893134, 2.574251347313722516 ) ) ;
#8972=( BOUNDED_CURVE ( )  B_SPLINE_CURVE ( 2, ( #55977, #31507, #21878, #20922, #41473, #51153, #21236, #16090, #40214 ),
 .UNSPECIFIED., .F., .F. ) 
 B_SPLINE_CURVE_WITH_KNOTS ( ( 3, 2, 2, 2, 3 ),
 ( 0.2979166666666666630, 0.2986111111111111049, 0.2999999999999999889, 0.3013888888888888729, 0.3020833333333333148 ),
 .UNSPECIFIED. ) 
 CURVE ( )  GEOMETRIC_REPRESENTATION_ITEM ( )  RATIONAL_B_SPLINE_CURVE ( ( 0.9330127018922194093, 0.9330127018922194093, 1.000000000000000000, 0.8660254037844387076, 1.000000000000000000, 0.8660254037844387076, 1.000000000000000000, 0.9330127018922194093, 0.9330127018922194093 ) ) 
 REPRESENTATION_ITEM ( '' )  );
#8978=CARTESIAN_POINT ( 'NONE',  ( -2.229367062499996610, -0.1458333319677394824, 3.861377020970582219 ) ) ;
#8979=CARTESIAN_POINT ( 'NONE',  ( -2.229367062500000163, -26.72916666530106866, -3.861377020970580443 ) ) ;
#8980=CARTESIAN_POINT ( 'NONE',  ( -1.846868145590734756, -156.1250000013655779, -4.458734125000000326 ) ) ;
#8983=( BOUNDED_CURVE ( )  B_SPLINE_CURVE ( 2, ( #48659, #38082, #23293, #9118, #28106, #28726, #58954, #58013, #43830 ),
 .UNSPECIFIED., .F., .F. ) 
 B_SPLINE_CURVE_WITH_KNOTS ( ( 3, 2, 2, 2, 3 ),
 ( 0.4187500000000000111, 0.4194444444444444531, 0.4208333333333333370, 0.4222222222222222210, 0.4229166666666666630 ),
 .UNSPECIFIED. ) 
 CURVE ( )  GEOMETRIC_REPRESENTATION_ITEM ( )  RATIONAL_B_SPLINE_CURVE ( ( 0.9330127018922194093, 0.9330127018922194093, 1.000000000000000000, 0.8660254037844387076, 1.000000000000000000, 0.8660254037844387076, 1.000000000000000000, 0.9330127018922194093, 0.9330127018922194093 ) ) 
 REPRESENTATION_ITEM ( '' )  );
#8984=CARTESIAN_POINT ( 'NONE',  ( -3.152548672688508926E-16, 29.43750000136559564, -5.148502694627439702 ) ) ;
#8987=CARTESIAN_POINT ( 'NONE',  ( -4.458734124999999437, -75.56249999863440792, 0.000000000000000000 ) ) ;
#8989=CARTESIAN_POINT ( 'NONE',  ( -6.972266317189433020E-16, -73.25000000000000000, -5.000000000000000000 ) ) ;
#8990=CARTESIAN_POINT ( 'NONE',  ( -4.999999999999999112, 27.20833333606451987, 2.886751345948131764 ) ) ;
#8993=CARTESIAN_POINT ( 'NONE',  ( 2.500000000000002220, -6.541666663935481019, 4.330127018922192761 ) ) ;
#8994=CARTESIAN_POINT ( 'NONE',  ( -4.999999999999999112, -10.91666666666666607, 2.886751345948131764 ) ) ;
#8995=CARTESIAN_POINT ( 'NONE',  ( -4.458734124999999437, -19.39583333196774007, -2.574251347313719407 ) ) ;
#8997=CARTESIAN_POINT ( 'NONE',  ( 9.457646018065525792E-16, -76.06249999863440792, 5.148502694627439702 ) ) ;
#8999=CARTESIAN_POINT ( 'NONE',  ( -1.846868145590737420, -167.0000000013655779, 4.458734124999999437 ) ) ;
#9000=CARTESIAN_POINT ( 'NONE',  ( 1.060575238724906964E-15, -20.62499999726880873, 5.773502691896257311 ) ) ;
#9001=CARTESIAN_POINT ( 'NONE',  ( 4.458734124999999437, -45.81249999863440081, -5.460374474430324690E-16 ) ) ;
#9004=CARTESIAN_POINT ( 'NONE',  ( 9.457646018065525792E-16, 6.687500001365594748, 5.148502694627439702 ) ) ;
#9007=CARTESIAN_POINT ( 'NONE',  ( -2.500000000000000444, -60.16666666666665719, -4.330127018922193649 ) ) ;
#9008=CARTESIAN_POINT ( 'NONE',  ( 3.152801135295367541, -157.5625000013656063, -3.152801135295367541 ) ) ;
#9010=CARTESIAN_POINT ( 'NONE',  ( -5.000000000000000000, -56.08333333333332860, -2.886751345948128211 ) ) ;
#9011=CARTESIAN_POINT ( 'NONE',  ( -3.535533905932738641, -164.3750000000000284, 3.535533905932737309 ) ) ;
#9012=ADVANCED_FACE ( 'NONE', ( #18457 ), #31985, .T. ) ;
#9015=CARTESIAN_POINT ( 'NONE',  ( 2.229367062500001939, -7.229166665301073103, 3.861377020970579999 ) ) ;
#9016=CARTESIAN_POINT ( 'NONE',  ( 4.458734125000001214, -39.14583333196773651, 2.574251347313718519 ) ) ;
#9018=CARTESIAN_POINT ( 'NONE',  ( 4.458734124999999437, -147.5000000013656063, 1.846868145590737864 ) ) ;
#9019=ADVANCED_FACE ( 'NONE', ( #52243 ), #28103, .T. ) ;
#9021=CARTESIAN_POINT ( 'NONE',  ( -4.458734124999999437, 29.43750000136559208, 0.000000000000000000 ) ) ;
#9022=ORIENTED_EDGE ( 'NONE', *, *, #59246, .T. ) ;
#9026=CARTESIAN_POINT ( 'NONE',  ( -4.458734124999998549, -77.47916666530106511, 2.574251347313722516 ) ) ;
#9028=FACE_OUTER_BOUND ( 'NONE', #28391, .T. ) ;
#9030=CARTESIAN_POINT ( 'NONE',  ( 1.339745962155615144, -79.58034179853028434, 4.999999999999999112 ) ) ;
#9031=CARTESIAN_POINT ( 'NONE',  ( 4.458734124999999437, 3.187500001365594304, -5.460374474430324690E-16 ) ) ;
#9032=DIRECTION ( 'NONE',  ( 0.000000000000000000, 0.000000000000000000, 1.000000000000000000 ) ) ;
#9033=CARTESIAN_POINT ( 'NONE',  ( 3.152801135295367541, -152.3125000013655779, -3.152801135295367541 ) ) ;
#9036=VERTEX_POINT ( 'NONE', #57079 ) ;
#9038=CARTESIAN_POINT ( 'NONE',  ( 6.123233995736766282E-16, -170.0000000000000000, -5.000000000000000000 ) ) ;
#9042=CARTESIAN_POINT ( 'NONE',  ( 0.000000000000000000, -170.0000000000000000, 5.000000000000000000 ) ) ;
#9043=FACE_OUTER_BOUND ( 'NONE', #19641, .T. ) ;
#9045=ADVANCED_FACE ( 'NONE', ( #32937 ), #41618, .T. ) ;
#9049=CARTESIAN_POINT ( 'NONE',  ( 4.458734124999998549, 20.27083333469892779, -2.574251347313721627 ) ) ;
#9051=CARTESIAN_POINT ( 'NONE',  ( -4.458734124999999437, -11.56249999863440792, 0.000000000000000000 ) ) ;
#9052=DIRECTION ( 'NONE',  ( -0.000000000000000000, 1.000000000000000000, -0.000000000000000000 ) ) ;
#9054=CARTESIAN_POINT ( 'NONE',  ( -4.458734125000000326, -168.0000000013655779, -1.846868145590735644 ) ) ;
#9057=VECTOR ( 'NONE', #51541, 1000.000000000000000 ) ;
#9062=CARTESIAN_POINT ( 'NONE',  ( -4.458734124999999437, -159.2500000013656063, -1.846868145590735644 ) ) ;
#9066=VERTEX_POINT ( 'NONE', #13316 ) ;
#9070=DIRECTION ( 'NONE',  ( -0.000000000000000000, 1.000000000000000000, -0.000000000000000000 ) ) ;
#9071=CARTESIAN_POINT ( 'NONE',  ( 5.000000000000000888, 2.416666666666667851, 2.886751345948126879 ) ) ;
#9072=CARTESIAN_POINT ( 'NONE',  ( -4.458734124999999437, -59.39583333196773651, -2.574251347313719407 ) ) ;
#9074=EDGE_CURVE ( 'NONE', #44817, #43815, #20115, .T. ) ;
#9075=EDGE_CURVE ( 'NONE', #21118, #47300, #62218, .T. ) ;
#9076=CARTESIAN_POINT ( 'NONE',  ( 2.500000000000002220, -0.5416666639354792423, 4.330127018922192761 ) ) ;
#9077=CARTESIAN_POINT ( 'NONE',  ( 4.458734124999998549, -30.72916666530107221, -2.574251347313721627 ) ) ;
#9079=CARTESIAN_POINT ( 'NONE',  ( -6.972266317189433020E-16, -23.12499999726880873, -5.000000000000000000 ) ) ;
#9080=CARTESIAN_POINT ( 'NONE',  ( -9.184850993605147944E-16, -151.2500000000000284, 5.000000000000000000 ) ) ;
#9081=CARTESIAN_POINT ( 'NONE',  ( -2.499999999999996447, -46.83333333333333570, 4.330127018922195425 ) ) ;
#9084=CARTESIAN_POINT ( 'NONE',  ( 1.339745962155612702, -64.29465819873851729, -5.000000000000000000 ) ) ;
#9085=CARTESIAN_POINT ( 'NONE',  ( -4.458734124999998549, -69.22916666530107932, 2.574251347313722516 ) ) ;
#9087=CARTESIAN_POINT ( 'NONE',  ( 3.152801135295366208, -148.8125000013655779, 3.152801135295367985 ) ) ;
#9088=CARTESIAN_POINT ( 'NONE',  ( 9.457646018065525792E-16, -78.06249999863440792, 5.148502694627439702 ) ) ;
#9092=CARTESIAN_POINT ( 'NONE',  ( 2.229367062499998831, -22.89583333196773651, -3.861377020970580887 ) ) ;
#9093=CARTESIAN_POINT ( 'NONE',  ( 5.000000000000000000, -66.29166666393547303, -2.886751345948129988 ) ) ;
#9094=ORIENTED_EDGE ( 'NONE', *, *, #31450, .T. ) ;
#9096=EDGE_CURVE ( 'NONE', #49104, #1040, #9773, .T. ) ;
#9102=CARTESIAN_POINT ( 'NONE',  ( 9.457646018065525792E-16, -60.31249999863440792, 5.148502694627439702 ) ) ;
#9104=EDGE_LOOP ( 'NONE', ( #3981, #60628, #887, #6580 ) ) ;
#9106=CARTESIAN_POINT ( 'NONE',  ( 0.000000000000000000, -170.0000000000000000, 0.000000000000000000 ) ) ;
#9107=CARTESIAN_POINT ( 'NONE',  ( 9.457646018065525792E-16, 20.93750000136558853, 5.148502694627439702 ) ) ;
#9109=CARTESIAN_POINT ( 'NONE',  ( 5.000000000000000000, 20.62500000273118772, -6.123233995736766282E-16 ) ) ;
#9110=CARTESIAN_POINT ( 'NONE',  ( 3.152801135295366208, -166.5625000013656063, 3.152801135295367985 ) ) ;
#9111=ORIENTED_EDGE ( 'NONE', *, *, #53943, .F. ) ;
#9113=CARTESIAN_POINT ( 'NONE',  ( 1.975475456537005874E-15, -39.75000000000000000, 5.000000000000000000 ) ) ;
#9115=CARTESIAN_POINT ( 'NONE',  ( 2.499999999999998668, -40.20833333060214443, -4.330127018922193649 ) ) ;
#9118=CARTESIAN_POINT ( 'NONE',  ( 5.000000000000000000, -20.41666666666666785, -2.886751345948130876 ) ) ;
#9121=CARTESIAN_POINT ( 'NONE',  ( 1.339745962155565406, -18.58034179853029855, 5.000000000000028422 ) ) ;
#9122=CARTESIAN_POINT ( 'NONE',  ( -2.071067811865372921, -159.3125000000000000, 5.000000000000104805 ) ) ;
#9126=CARTESIAN_POINT ( 'NONE',  ( 1.339745962155615144, 11.29465819873851906, 4.999999999999999112 ) ) ;
#9128=CARTESIAN_POINT ( 'NONE',  ( -2.071067811865478170, -149.4375000027312410, 5.000000000000000000 ) ) ;
#9130=AXIS2_PLACEMENT_3D ( 'NONE', #15902, #21368, #26510 ) ;
#9134=CARTESIAN_POINT ( 'NONE',  ( -5.000000000000000888, -142.4375000000000000, 2.071067811865474617 ) ) ;
#9136=CARTESIAN_POINT ( 'NONE',  ( -4.458734124999999437, -168.2500000013656063, -1.846868145590735644 ) ) ;
#9137=CARTESIAN_POINT ( 'NONE',  ( 9.457646018065525792E-16, -29.06249999863440436, 5.148502694627439702 ) ) ;
#9138=DIRECTION ( 'NONE',  ( -0.000000000000000000, 1.000000000000000000, -0.000000000000000000 ) ) ;
#9139=CYLINDRICAL_SURFACE ( 'NONE', #14309, 5.000000000000000000 ) ;
#9141=CARTESIAN_POINT ( 'NONE',  ( -4.458734125000000326, -148.0000000013655779, -1.846868145590735644 ) ) ;
#9142=ORIENTED_EDGE ( 'NONE', *, *, #25492, .F. ) ;
#9143=CARTESIAN_POINT ( 'NONE',  ( -2.500000000000000444, -90.04166666393547303, -4.330127018922193649 ) ) ;
#9145=CARTESIAN_POINT ( 'NONE',  ( 4.458734124999999437, -58.06249999863440081, -5.460374474430324690E-16 ) ) ;
#9148=CARTESIAN_POINT ( 'NONE',  ( 2.500000000000002220, 20.33333333333333215, 4.330127018922192761 ) ) ;
#9149=DIRECTION ( 'NONE',  ( 0.000000000000000000, 0.000000000000000000, 1.000000000000000000 ) ) ;
#9150=CARTESIAN_POINT ( 'NONE',  ( 4.458734124999999437, -6.812499998634404363, -5.460374474430324690E-16 ) ) ;
#9151=CARTESIAN_POINT ( 'NONE',  ( -2.071067811865308972, -154.3125000000000000, 5.000000000000169642 ) ) ;
#9153=CARTESIAN_POINT ( 'NONE',  ( 2.229367062500001939, 8.770833334698927786, 3.861377020970579999 ) ) ;
#9154=LINE ( 'NONE', #13669, #37696 ) ;
#9155=ORIENTED_EDGE ( 'NONE', *, *, #14240, .F. ) ;
#9156=DIRECTION ( 'NONE',  ( 0.000000000000000000, 1.000000000000000000, 0.000000000000000000 ) ) ;
#9157=CARTESIAN_POINT ( 'NONE',  ( 4.458734124999999437, -56.81249999863440081, -5.460374474430324690E-16 ) ) ;
#9158=CARTESIAN_POINT ( 'NONE',  ( 1.846868145590736310, -160.8750000013655779, 4.458734124999999437 ) ) ;
#9160=CARTESIAN_POINT ( 'NONE',  ( -4.999999999999999112, -52.79166666393547303, 2.886751345948131764 ) ) ;
#9161=EDGE_LOOP ( 'NONE', ( #6803, #44772, #40941, #25872 ) ) ;
#9162=CARTESIAN_POINT ( 'NONE',  ( -2.229367062500000163, 6.270833334698928674, -3.861377020970580443 ) ) ;
#9164=CARTESIAN_POINT ( 'NONE',  ( -6.972266317189433020E-16, 13.74999999999999822, -5.000000000000000000 ) ) ;
#9166=CARTESIAN_POINT ( 'NONE',  ( -3.152801135295367985, -160.8125000013656063, 3.152801135295367096 ) ) ;
#9167=EDGE_CURVE ( 'NONE', #9668, #19705, #12371, .T. ) ;
#9171=CARTESIAN_POINT ( 'NONE',  ( 2.499999999999998668, -87.20833333060214443, -4.330127018922193649 ) ) ;
#9175=CARTESIAN_POINT ( 'NONE',  ( 4.458734124999998549, -36.97916666530107221, -2.574251347313721627 ) ) ;
#9176=EDGE_LOOP ( 'NONE', ( #2541, #52857, #17906, #7268 ) ) ;
#9177=EDGE_CURVE ( 'NONE', #62942, #37665, #36098, .T. ) ;
#9180=CARTESIAN_POINT ( 'NONE',  ( -2.071067811865602071, -156.8125000027311842, -4.999999999999874767 ) ) ;
#9182=CARTESIAN_POINT ( 'NONE',  ( -4.458734124999998549, -83.47916666530107932, 2.574251347313722516 ) ) ;
#9184=CARTESIAN_POINT ( 'NONE',  ( -4.999999999999998224, 25.20833333606451987, 2.886751345948131764 ) ) ;
#9188=CARTESIAN_POINT ( 'NONE',  ( 3.061616997868383141E-16, -143.8750000027312126, -5.000000000000000000 ) ) ;
#9191=CARTESIAN_POINT ( 'NONE',  ( -6.972266317189433020E-16, -40.24999999999999289, -5.000000000000000000 ) ) ;
#9194=CARTESIAN_POINT ( 'NONE',  ( 0.000000000000000000, -170.0000000000000000, 5.000000000000000000 ) ) ;
#9196=CARTESIAN_POINT ( 'NONE',  ( 4.458734125000001214, -85.14583333196773651, 2.574251347313718519 ) ) ;
#9199=ORIENTED_EDGE ( 'NONE', *, *, #40356, .T. ) ;
#9202=CARTESIAN_POINT ( 'NONE',  ( -3.535533905932737309, -166.7500000027312126, -3.535533905932738197 ) ) ;
#9211=CARTESIAN_POINT ( 'NONE',  ( 5.000000000000000000, -86.37499999726880162, -6.123233995736766282E-16 ) ) ;
#9212=CARTESIAN_POINT ( 'NONE',  ( -2.229367062499996610, -12.14583333196774007, 3.861377020970582219 ) ) ;
#9213=LINE ( 'NONE', #24316, #34113 ) ;
#9214=ORIENTED_EDGE ( 'NONE', *, *, #4211, .T. ) ;
#9215=CARTESIAN_POINT ( 'NONE',  ( 2.229367062499998831, -38.89583333196773651, -3.861377020970580887 ) ) ;
#9216=CARTESIAN_POINT ( 'NONE',  ( -8.190561711645485556E-16, -154.9375000013655779, 4.458734124999999437 ) ) ;
#9217=FACE_OUTER_BOUND ( 'NONE', #5611, .T. ) ;
#9218=CARTESIAN_POINT ( 'NONE',  ( 1.975475456537005874E-15, -46.74999999999999289, 5.000000000000000000 ) ) ;
#9222=CARTESIAN_POINT ( 'NONE',  ( 4.458734124999998549, 12.27083333469892423, -2.574251347313721627 ) ) ;
#9223=EDGE_CURVE ( 'NONE', #7560, #27699, #38178, .T. ) ;
#9225=CARTESIAN_POINT ( 'NONE',  ( 4.458734124999999437, -90.06249999863440792, -5.460374474430324690E-16 ) ) ;
#9227=CARTESIAN_POINT ( 'NONE',  ( 2.499999999999998668, 12.79166666939785379, -4.330127018922193649 ) ) ;
#9231=CARTESIAN_POINT ( 'NONE',  ( 3.061616997868383141E-16, -166.7500000000000000, -5.000000000000000000 ) ) ;
#9233=CARTESIAN_POINT ( 'NONE',  ( 5.000000000000000888, -85.58333333333332860, 2.886751345948126879 ) ) ;
#9234=CARTESIAN_POINT ( 'NONE',  ( 2.499999999999998668, -29.33333333333332860, -4.330127018922193649 ) ) ;
#9235=CARTESIAN_POINT ( 'NONE',  ( 4.458734124999998549, -33.72916666530106511, -2.574251347313721627 ) ) ;
#9236=CARTESIAN_POINT ( 'NONE',  ( -2.500000000000000444, -35.04166666393547303, -4.330127018922193649 ) ) ;
#9237=CARTESIAN_POINT ( 'NONE',  ( -2.229367062499996610, -64.14583333196773651, 3.861377020970582219 ) ) ;
#9238=ORIENTED_EDGE ( 'NONE', *, *, #42910, .T. ) ;
#9240=CARTESIAN_POINT ( 'NONE',  ( 2.229367062499998831, -14.89583333196773474, -3.861377020970580887 ) ) ;
#9242=CARTESIAN_POINT ( 'NONE',  ( 2.499999999999998668, -77.33333333333334281, -4.330127018922193649 ) ) ;
#9245=CARTESIAN_POINT ( 'NONE',  ( -4.999999999999999112, -80.79166666393547303, 2.886751345948131764 ) ) ;
#9246=CARTESIAN_POINT ( 'NONE',  ( -1.339745962155610925, -31.79465819873851373, 5.000000000000000000 ) ) ;
#9249=CARTESIAN_POINT ( 'NONE',  ( -3.152548672688508926E-16, -23.81249999863440792, -5.148502694627439702 ) ) ;
#9250=CARTESIAN_POINT ( 'NONE',  ( -2.229367062500000163, -59.72916666530106511, -3.861377020970580443 ) ) ;
#9253=CARTESIAN_POINT ( 'NONE',  ( 3.152801135295366208, -167.8125000013656063, 3.152801135295367985 ) ) ;
#9256=ORIENTED_EDGE ( 'NONE', *, *, #24032, .T. ) ;
#9264=CARTESIAN_POINT ( 'NONE',  ( -8.190561711645485556E-16, -144.9375000013656063, 4.458734124999999437 ) ) ;
#9268=CARTESIAN_POINT ( 'NONE',  ( -4.458734124999999437, -68.56249999863439371, 0.000000000000000000 ) ) ;
#9270=CARTESIAN_POINT ( 'NONE',  ( -4.458734125000000326, -140.8750000013656063, 1.846868145590734089 ) ) ;
#9277=DIRECTION ( 'NONE',  ( 0.000000000000000000, 0.000000000000000000, 1.000000000000000000 ) ) ;
#9279=ADVANCED_FACE ( 'NONE', ( #2509 ), #27567, .T. ) ;
#9280=CARTESIAN_POINT ( 'NONE',  ( 4.458734124999999437, 20.93750000136559208, -5.460374474430324690E-16 ) ) ;
#9281=CARTESIAN_POINT ( 'NONE',  ( 1.339745962155615144, -18.70534180126147916, 4.999999999999999112 ) ) ;
#9286=CARTESIAN_POINT ( 'NONE',  ( 1.339745962155615144, -80.70534180126146850, 4.999999999999999112 ) ) ;
#9287=CARTESIAN_POINT ( 'NONE',  ( -4.458734124999999437, 1.604166668032262155, -2.574251347313719407 ) ) ;
#9288=CARTESIAN_POINT ( 'NONE',  ( 9.457646018065525792E-16, -23.31249999863440436, 5.148502694627439702 ) ) ;
#9289=CARTESIAN_POINT ( 'NONE',  ( 4.458734125000000326, -157.3750000013656347, -1.846868145590734978 ) ) ;
#9292=LINE ( 'NONE', #47284, #33696 ) ;
#9295=CARTESIAN_POINT ( 'NONE',  ( -4.458734124999999437, -70.56249999863439371, 0.000000000000000000 ) ) ;
#9297=CARTESIAN_POINT ( 'NONE',  ( 0.000000000000000000, -170.0000000000000000, 0.000000000000000000 ) ) ;
#9298=FACE_OUTER_BOUND ( 'NONE', #41505, .T. ) ;
#9299=VERTEX_POINT ( 'NONE', #8279 ) ;
#9300=LINE ( 'NONE', #24105, #50976 ) ;
#9303=CARTESIAN_POINT ( 'NONE',  ( 5.000000000000000000, -12.41666666666666607, -2.886751345948129988 ) ) ;
#9304=CARTESIAN_POINT ( 'NONE',  ( -3.152548672688508926E-16, -14.56249999863440436, -5.148502694627439702 ) ) ;
#9305=VECTOR ( 'NONE', #55369, 1000.000000000000000 ) ;
#9306=CARTESIAN_POINT ( 'NONE',  ( 2.229367062499998831, -77.64583333196773651, -3.861377020970580887 ) ) ;
#9307=CARTESIAN_POINT ( 'NONE',  ( 2.730187237215162345E-16, -168.4375000013656063, -4.458734124999999437 ) ) ;
#9308=CARTESIAN_POINT ( 'NONE',  ( -3.535250795749689387E-16, -18.12499999726881228, -5.773502691896257311 ) ) ;
#9309=CARTESIAN_POINT ( 'NONE',  ( 4.458734124999998549, -46.72916666530106511, -2.574251347313721627 ) ) ;
#9312=CARTESIAN_POINT ( 'NONE',  ( -4.458734124999999437, 0.3541666680322609340, -2.574251347313719407 ) ) ;
#9315=CARTESIAN_POINT ( 'NONE',  ( -2.500000000000000444, -62.16666666666666430, -4.330127018922193649 ) ) ;
#9316=CARTESIAN_POINT ( 'NONE',  ( -1.846868145590734756, -157.3750000013656347, -4.458734125000000326 ) ) ;
#9318=CARTESIAN_POINT ( 'NONE',  ( -1.339745962155613812, -65.20534180126146850, -5.000000000000000000 ) ) ;
#9319=CARTESIAN_POINT ( 'NONE',  ( 2.071067811865475505, -161.8125000000000284, -5.000000000000000888 ) ) ;
#9320=CARTESIAN_POINT ( 'NONE',  ( 2.071067811865455077, -167.8124999999999716, -5.000000000000022204 ) ) ;
#9322=CARTESIAN_POINT ( 'NONE',  ( 9.457646018065525792E-16, -5.312499998634402587, 5.148502694627439702 ) ) ;
#9323=CARTESIAN_POINT ( 'NONE',  ( 2.229367062500001939, -47.22916666530106511, 3.861377020970579999 ) ) ;
#9324=CARTESIAN_POINT ( 'NONE',  ( 1.339745962155615144, -67.58034179853029855, 4.999999999999999112 ) ) ;
#9325=CARTESIAN_POINT ( 'NONE',  ( -3.152801135295367096, -149.0625000013655779, -3.152801135295367541 ) ) ;
#9329=CARTESIAN_POINT ( 'NONE',  ( 5.000000000000000888, -155.0625000027311842, -2.071067811865475505 ) ) ;
#9330=CARTESIAN_POINT ( 'NONE',  ( -1.339745962155610925, -68.66965819600733312, 5.000000000000000000 ) ) ;
#9333=EDGE_LOOP ( 'NONE', ( #37046, #50243, #37709, #22033 ) ) ;
#9334=( BOUNDED_CURVE ( )  B_SPLINE_CURVE ( 2, ( #32698, #60717, #16640, #17272, #61036, #12759, #36262, #12446, #32382 ),
 .UNSPECIFIED., .F., .F. ) 
 B_SPLINE_CURVE_WITH_KNOTS ( ( 3, 2, 2, 2, 3 ),
 ( 0.1020833333333333315, 0.1027777777777777735, 0.1041666666666666713, 0.1055555555555555552, 0.1062499999999999972 ),
 .UNSPECIFIED. ) 
 CURVE ( )  GEOMETRIC_REPRESENTATION_ITEM ( )  RATIONAL_B_SPLINE_CURVE ( ( 0.9330127018922194093, 0.9330127018922194093, 1.000000000000000000, 0.8660254037844387076, 1.000000000000000000, 0.8660254037844387076, 1.000000000000000000, 0.9330127018922194093, 0.9330127018922194093 ) ) 
 REPRESENTATION_ITEM ( '' )  );
#9335=DIRECTION ( 'NONE',  ( -0.000000000000000000, 1.000000000000000000, -0.000000000000000000 ) ) ;
#9338=CARTESIAN_POINT ( 'NONE',  ( -4.458734124999999437, -3.312499998634407916, 0.000000000000000000 ) ) ;
#9340=CARTESIAN_POINT ( 'NONE',  ( 1.846868145590735200, -154.2500000013656063, -4.458734124999999437 ) ) ;
#9342=VERTEX_POINT ( 'NONE', #42992 ) ;
#9346=AXIS2_PLACEMENT_3D ( 'NONE', #37251, #52049, #31785 ) ;
#9347=EDGE_CURVE ( 'NONE', #47748, #8541, #11856, .T. ) ;
#9349=CARTESIAN_POINT ( 'NONE',  ( 1.975475456537005874E-15, 8.375000002731187720, 5.000000000000000000 ) ) ;
#9356=ORIENTED_EDGE ( 'NONE', *, *, #36609, .F. ) ;
#9357=CARTESIAN_POINT ( 'NONE',  ( -3.152548672688508926E-16, 15.43750000136559564, -5.148502694627439702 ) ) ;
#9359=CARTESIAN_POINT ( 'NONE',  ( -2.229367062499996610, -7.395833331967735624, 3.861377020970582219 ) ) ;
#9360=CARTESIAN_POINT ( 'NONE',  ( -1.339745962155613812, -63.20534180126146850, -5.000000000000000000 ) ) ;
#9362=CARTESIAN_POINT ( 'NONE',  ( -3.152801135295367096, -169.0625000013656063, -3.152801135295367541 ) ) ;
#9363=CARTESIAN_POINT ( 'NONE',  ( 5.000000000000000000, -88.50000000000000000, -6.123233995736766282E-16 ) ) ;
#9370=EDGE_CURVE ( 'NONE', #3859, #27694, #24251, .T. ) ;
#9372=CARTESIAN_POINT ( 'NONE',  ( -4.458734124999999437, -153.1875000013656063, -5.460374474430324690E-16 ) ) ;
#9378=CARTESIAN_POINT ( 'NONE',  ( 5.000000000000000000, -162.0625000000000000, 2.071067811865478614 ) ) ;
#9379=CARTESIAN_POINT ( 'NONE',  ( 5.000000000000000000, 1.583333333333332593, -2.886751345948129988 ) ) ;
#9380=EDGE_CURVE ( 'NONE', #21022, #45244, #45670, .T. ) ;
#9381=CARTESIAN_POINT ( 'NONE',  ( 2.229367062500001939, -61.97916666530106511, 3.861377020970579999 ) ) ;
#9383=CARTESIAN_POINT ( 'NONE',  ( -5.000000000000000000, -4.874999997268810503, 0.000000000000000000 ) ) ;
#9384=CARTESIAN_POINT ( 'NONE',  ( 9.457646018065525792E-16, -29.06249999863440081, 5.148502694627439702 ) ) ;
#9386=CYLINDRICAL_SURFACE ( 'NONE', #46702, 5.000000000000000000 ) ;
#9388=CARTESIAN_POINT ( 'NONE',  ( -5.000000000000000000, -43.08333333333332860, -2.886751345948128211 ) ) ;
#9391=CARTESIAN_POINT ( 'NONE',  ( 4.458734124999999437, -71.81249999863439371, -5.460374474430324690E-16 ) ) ;
#9392=CARTESIAN_POINT ( 'NONE',  ( 1.846868145590735200, -145.5000000013655779, -4.458734125000000326 ) ) ;
#9394=CARTESIAN_POINT ( 'NONE',  ( 4.458734124999998549, -78.72916666530106511, -2.574251347313721627 ) ) ;
#9396=CARTESIAN_POINT ( 'NONE',  ( 2.229367062500001939, -25.22916666530106866, 3.861377020970579999 ) ) ;
#9397=CARTESIAN_POINT ( 'NONE',  ( 5.000000000000000000, -67.37499999726881583, -6.123233995736766282E-16 ) ) ;
#9401=ORIENTED_EDGE ( 'NONE', *, *, #62908, .F. ) ;
#9403=CARTESIAN_POINT ( 'NONE',  ( 2.071067811865433317, -165.8125000000000000, -5.000000000000041744 ) ) ;
#9405=CARTESIAN_POINT ( 'NONE',  ( 1.062108568985190270E-13, -25.25000000000000355, -4.999999999999999112 ) ) ;
#9406=( BOUNDED_CURVE ( )  B_SPLINE_CURVE ( 2, ( #54771, #25172, #50257, #46955, #29990, #45113, #10703, #17682, #10381 ),
 .UNSPECIFIED., .F., .F. ) 
 B_SPLINE_CURVE_WITH_KNOTS ( ( 3, 2, 2, 2, 3 ),
 ( 0.5520833333333333703, 0.5527777777777778123, 0.5541666666666666963, 0.5555555555555555802, 0.5562500000000000222 ),
 .UNSPECIFIED. ) 
 CURVE ( )  GEOMETRIC_REPRESENTATION_ITEM ( )  RATIONAL_B_SPLINE_CURVE ( ( 0.9330127018922194093, 0.9330127018922194093, 1.000000000000000000, 0.8660254037844387076, 1.000000000000000000, 0.8660254037844387076, 1.000000000000000000, 0.9330127018922194093, 0.9330127018922194093 ) ) 
 REPRESENTATION_ITEM ( '' )  );
#9407=CARTESIAN_POINT ( 'NONE',  ( -4.999999999999998224, -2.916666666666664742, 2.886751345948131764 ) ) ;
#9408=CARTESIAN_POINT ( 'NONE',  ( 2.229367062500001939, -60.22916666530106511, 3.861377020970579999 ) ) ;
#9410=ORIENTED_EDGE ( 'NONE', *, *, #51133, .F. ) ;
#9412=CARTESIAN_POINT ( 'NONE',  ( 4.458734124999998549, 12.27083333469892423, -2.574251347313721627 ) ) ;
#9415=CARTESIAN_POINT ( 'NONE',  ( 3.152801135295367541, -166.3125000013656063, -3.152801135295367541 ) ) ;
#9418=CARTESIAN_POINT ( 'NONE',  ( -2.500000000000000444, -70.04166666393547303, -4.330127018922193649 ) ) ;
#9422=CARTESIAN_POINT ( 'NONE',  ( 5.000000000000000888, -40.45833333060214443, 2.886751345948126879 ) ) ;
#9428=LINE ( 'NONE', #57711, #30616 ) ;
#9432=CARTESIAN_POINT ( 'NONE',  ( -3.152548672688508926E-16, 8.187500001365595637, -5.148502694627439702 ) ) ;
#9435=CARTESIAN_POINT ( 'NONE',  ( 5.000000000000000888, -151.0625000027312126, -2.071067811865475505 ) ) ;
#9436=CARTESIAN_POINT ( 'NONE',  ( 3.061616997868383141E-16, -156.8750000027311842, -5.000000000000000000 ) ) ;
#9440=CARTESIAN_POINT ( 'NONE',  ( 2.071067811865476394, -141.1875000000000284, 5.000000000000000000 ) ) ;
#9443=CARTESIAN_POINT ( 'NONE',  ( 4.458734124999999437, -165.6875000013655779, 0.000000000000000000 ) ) ;
#9444=CARTESIAN_POINT ( 'NONE',  ( -2.229367062499996610, -28.14583333196774007, 3.861377020970582219 ) ) ;
#9448=CARTESIAN_POINT ( 'NONE',  ( -3.152801135295367985, -142.8125000013655779, 3.152801135295367096 ) ) ;
#9449=ORIENTED_EDGE ( 'NONE', *, *, #28771, .T. ) ;
#9450=CARTESIAN_POINT ( 'NONE',  ( -2.229367062500000163, 26.27083333469892779, -3.861377020970580443 ) ) ;
#9452=CARTESIAN_POINT ( 'NONE',  ( -4.458734124999999437, -55.64583333196773651, -2.574251347313719407 ) ) ;
#9454=( BOUNDED_CURVE ( )  B_SPLINE_CURVE ( 2, ( #50333, #1149, #40354, #41303, #11086, #22022, #20749, #30708, #55167 ),
 .UNSPECIFIED., .F., .F. ) 
 B_SPLINE_CURVE_WITH_KNOTS ( ( 3, 2, 2, 2, 3 ),
 ( 0.2395833333333333426, 0.2402777777777777846, 0.2416666666666666685, 0.2430555555555555525, 0.2437499999999999944 ),
 .UNSPECIFIED. ) 
 CURVE ( )  GEOMETRIC_REPRESENTATION_ITEM ( )  RATIONAL_B_SPLINE_CURVE ( ( 0.9330127018922194093, 0.9330127018922194093, 1.000000000000000000, 0.8660254037844387076, 1.000000000000000000, 0.8660254037844387076, 1.000000000000000000, 0.9330127018922194093, 0.9330127018922194093 ) ) 
 REPRESENTATION_ITEM ( '' )  );
#9455=CARTESIAN_POINT ( 'NONE',  ( 1.339745962155612702, 13.83034180399266333, -5.000000000000000000 ) ) ;
#9456=CARTESIAN_POINT ( 'NONE',  ( 5.000000000000000000, 20.58333333333333570, -2.886751345948129988 ) ) ;
#9457=CARTESIAN_POINT ( 'NONE',  ( -4.999999999999998224, -36.79166666393548013, 2.886751345948131764 ) ) ;
#9458=CARTESIAN_POINT ( 'NONE',  ( 2.229367062499998831, -8.645833331967736513, -3.861377020970580887 ) ) ;
#9459=CARTESIAN_POINT ( 'NONE',  ( -2.499999999999996447, -22.83333333333333215, 4.330127018922195425 ) ) ;
#9465=CARTESIAN_POINT ( 'NONE',  ( 9.457646018065525792E-16, -54.06249999863440081, 5.148502694627439702 ) ) ;
#9466=CARTESIAN_POINT ( 'NONE',  ( -1.846868145590737420, -155.0000000013656063, 4.458734124999999437 ) ) ;
#9467=CARTESIAN_POINT ( 'NONE',  ( -2.499999999999996447, -50.70833333060213732, 4.330127018922195425 ) ) ;
#9468=ORIENTED_EDGE ( 'NONE', *, *, #23681, .T. ) ;
#9469=CARTESIAN_POINT ( 'NONE',  ( 2.229367062499998831, 7.104166668032259935, -3.861377020970580887 ) ) ;
#9473=CARTESIAN_POINT ( 'NONE',  ( -8.190561711645485556E-16, -161.6875000013655779, 4.458734124999999437 ) ) ;
#9477=CARTESIAN_POINT ( 'NONE',  ( 5.000000000000000000, -47.29166666393547303, -2.886751345948130876 ) ) ;
#9478=CARTESIAN_POINT ( 'NONE',  ( -3.152548672688508926E-16, -44.81249999863440792, -5.148502694627439702 ) ) ;
#9480=CARTESIAN_POINT ( 'NONE',  ( 5.000000000000000000, 9.708333336064519870, -2.886751345948130876 ) ) ;
#9484=CARTESIAN_POINT ( 'NONE',  ( 2.229367062500001939, 28.02083333469892779, 3.861377020970579999 ) ) ;
#9492=FACE_OUTER_BOUND ( 'NONE', #59076, .T. ) ;
#9498=LINE ( 'NONE', #58402, #49949 ) ;
#9499=CARTESIAN_POINT ( 'NONE',  ( -2.499999999999996447, -60.83333333333333570, 4.330127018922195425 ) ) ;
#9500=CARTESIAN_POINT ( 'NONE',  ( -4.458734124999999437, -83.64583333196773651, -2.574251347313719407 ) ) ;
#9504=EDGE_CURVE ( 'NONE', #30240, #24529, #34561, .T. ) ;
#9508=CARTESIAN_POINT ( 'NONE',  ( 3.061616997868383141E-16, -162.8750000027311842, -5.000000000000000000 ) ) ;
#9512=EDGE_CURVE ( 'NONE', #25897, #32533, #11097, .T. ) ;
#9520=CYLINDRICAL_SURFACE ( 'NONE', #32561, 5.000000000000000000 ) ;
#9521=CARTESIAN_POINT ( 'NONE',  ( 4.458734125000000326, -12.89583333196774362, 2.574251347313718519 ) ) ;
#9522=DIRECTION ( 'NONE',  ( -0.000000000000000000, 1.000000000000000000, -0.000000000000000000 ) ) ;
#9523=CARTESIAN_POINT ( 'NONE',  ( 3.061616997868383141E-16, -153.7500000000000000, -5.000000000000000000 ) ) ;
#9525=EDGE_CURVE ( 'NONE', #61372, #29467, #52624, .T. ) ;
#9527=CARTESIAN_POINT ( 'NONE',  ( -4.458734124999999437, -39.56249999863440081, 0.000000000000000000 ) ) ;
#9529=EDGE_CURVE ( 'NONE', #859, #29294, #11663, .T. ) ;
#9534=( BOUNDED_CURVE ( )  B_SPLINE_CURVE ( 2, ( #34095, #53720, #9651, #24452, #23, #44059, #19624, #29582, #58860 ),
 .UNSPECIFIED., .F., .F. ) 
 B_SPLINE_CURVE_WITH_KNOTS ( ( 3, 2, 2, 2, 3 ),
 ( 0.6729166666666667185, 0.6736111111111111605, 0.6750000000000000444, 0.6763888888888889284, 0.6770833333333333703 ),
 .UNSPECIFIED. ) 
 CURVE ( )  GEOMETRIC_REPRESENTATION_ITEM ( )  RATIONAL_B_SPLINE_CURVE ( ( 0.9330127018922194093, 0.9330127018922194093, 1.000000000000000000, 0.8660254037844387076, 1.000000000000000000, 0.8660254037844387076, 1.000000000000000000, 0.9330127018922194093, 0.9330127018922194093 ) ) 
 REPRESENTATION_ITEM ( '' )  );
#9535=CARTESIAN_POINT ( 'NONE',  ( 4.458734124999999437, 10.18750000136559386, -5.460374474430324690E-16 ) ) ;
#9537=CARTESIAN_POINT ( 'NONE',  ( 1.975475456537005874E-15, -43.75000000000000000, 5.000000000000000000 ) ) ;
#9538=CARTESIAN_POINT ( 'NONE',  ( -5.000000000000000888, -165.6875000027311842, -2.071067811865475949 ) ) ;
#9539=CARTESIAN_POINT ( 'NONE',  ( 4.458734124999999437, -87.06249999863439371, -5.460374474430324690E-16 ) ) ;
#9540=CARTESIAN_POINT ( 'NONE',  ( -4.458734124999999437, 21.43750000136559208, 0.000000000000000000 ) ) ;
#9542=CARTESIAN_POINT ( 'NONE',  ( 1.060575238724906964E-15, 15.37500000273118417, 5.773502691896257311 ) ) ;
#9544=CARTESIAN_POINT ( 'NONE',  ( 1.339745962155615144, -79.70534180126146850, 4.999999999999999112 ) ) ;
#9545=VERTEX_POINT ( 'NONE', #21333 ) ;
#9546=CARTESIAN_POINT ( 'NONE',  ( 0.000000000000000000, -170.0000000000000000, 0.000000000000000000 ) ) ;
#9547=CARTESIAN_POINT ( 'NONE',  ( -2.500000000000000444, -33.16666666666666430, -4.330127018922193649 ) ) ;
#9548=CARTESIAN_POINT ( 'NONE',  ( 4.458734124999999437, -38.81249999863440081, -5.460374474430324690E-16 ) ) ;
#9549=CARTESIAN_POINT ( 'NONE',  ( 2.499999999999998668, -32.20833333060215153, -4.330127018922193649 ) ) ;
#9550=CARTESIAN_POINT ( 'NONE',  ( -3.152548672688508926E-16, -67.56249999863440792, -5.148502694627439702 ) ) ;
#9553=CARTESIAN_POINT ( 'NONE',  ( -2.229367062499996610, -10.14583333196773829, 3.861377020970582219 ) ) ;
#9554=CARTESIAN_POINT ( 'NONE',  ( -4.458734124999999437, -16.64583333196773651, -2.574251347313719407 ) ) ;
#9556=CARTESIAN_POINT ( 'NONE',  ( -3.535250795749689387E-16, -83.25000000000000000, -5.773502691896257311 ) ) ;
#9559=CARTESIAN_POINT ( 'NONE',  ( -2.499999999999996447, -80.70833333060213022, 4.330127018922195425 ) ) ;
#9563=CARTESIAN_POINT ( 'NONE',  ( 2.229367062500001939, -25.22916666530106866, 3.861377020970579999 ) ) ;
#9566=CARTESIAN_POINT ( 'NONE',  ( -1.846868145590734756, -167.3750000013656347, -4.458734125000000326 ) ) ;
#9568=CARTESIAN_POINT ( 'NONE',  ( 1.975475456537005874E-15, 18.24999999999999645, 5.000000000000000000 ) ) ;
#9574=CARTESIAN_POINT ( 'NONE',  ( 2.499999999999998668, -3.208333330602147093, -4.330127018922193649 ) ) ;
#9579=CARTESIAN_POINT ( 'NONE',  ( -3.152801135295367985, -145.0625000013655779, 3.152801135295367096 ) ) ;
#9583=( BOUNDED_CURVE ( )  B_SPLINE_CURVE ( 2, ( #26015, #31147, #50131, #11840, #1276, #31459, #51099, #2226, #25698 ),
 .UNSPECIFIED., .F., .F. ) 
 B_SPLINE_CURVE_WITH_KNOTS ( ( 3, 2, 2, 2, 3 ),
 ( 0.6749999999999996003, 0.6791666666666662522, 0.6833333333333329040, 0.6874999999999996669, 0.6916666666666663188 ),
 .UNSPECIFIED. ) 
 CURVE ( )  GEOMETRIC_REPRESENTATION_ITEM ( )  RATIONAL_B_SPLINE_CURVE ( ( 1.000000000000008216, 0.9238795325112786339, 1.000000000000000000, 0.9238795325112867385, 1.000000000000000000, 0.9238795325112867385, 1.000000000000000000, 0.9238795325112928447, 0.9999999999999938938 ) ) 
 REPRESENTATION_ITEM ( '' )  );
#9584=CARTESIAN_POINT ( 'NONE',  ( 2.229367062499998831, -68.89583333196773651, -3.861377020970580887 ) ) ;
#9586=CARTESIAN_POINT ( 'NONE',  ( -1.339745962155613812, -1.080341798530293218, -5.000000000000000000 ) ) ;
#9587=CARTESIAN_POINT ( 'NONE',  ( -4.458734124999999437, -143.0000000013655779, -1.846868145590735644 ) ) ;
#9590=CARTESIAN_POINT ( 'NONE',  ( -1.339745962155613812, -50.08034179853029855, -5.000000000000000000 ) ) ;
#9595=CARTESIAN_POINT ( 'NONE',  ( -3.152548672688508926E-16, 24.18750000136559564, -5.148502694627439702 ) ) ;
#9602=CARTESIAN_POINT ( 'NONE',  ( 9.457646018065525792E-16, 1.937500001365593416, 5.148502694627439702 ) ) ;
#9604=CARTESIAN_POINT ( 'NONE',  ( -4.458734124999999437, -27.56249999863440081, 0.000000000000000000 ) ) ;
#9607=CARTESIAN_POINT ( 'NONE',  ( -4.458734124999999437, 27.68750000136559208, 0.000000000000000000 ) ) ;
#9611=CARTESIAN_POINT ( 'NONE',  ( -2.229367062500000163, -71.72916666530107932, -3.861377020970580443 ) ) ;
#9614=CYLINDRICAL_SURFACE ( 'NONE', #17127, 5.000000000000000000 ) ;
#9615=ORIENTED_EDGE ( 'NONE', *, *, #22108, .F. ) ;
#9616=CARTESIAN_POINT ( 'NONE',  ( 2.499999999999998668, 6.666666666666667851, -4.330127018922193649 ) ) ;
#9617=CARTESIAN_POINT ( 'NONE',  ( 2.500000000000002220, -89.54166666393547303, 4.330127018922192761 ) ) ;
#9618=CARTESIAN_POINT ( 'NONE',  ( 5.000000000000000000, -18.41666666666666430, -2.886751345948129988 ) ) ;
#9619=CARTESIAN_POINT ( 'NONE',  ( 4.458734125000001214, -24.89583333196773651, 2.574251347313718519 ) ) ;
#9620=CARTESIAN_POINT ( 'NONE',  ( -3.152548672688508926E-16, -80.56249999863440792, -5.148502694627439702 ) ) ;
#9621=CARTESIAN_POINT ( 'NONE',  ( 3.152801135295367541, -169.5625000013656063, -3.152801135295367541 ) ) ;
#9622=CARTESIAN_POINT ( 'NONE',  ( 2.500000000000002220, -17.54166666393547658, 4.330127018922192761 ) ) ;
#9623=CARTESIAN_POINT ( 'NONE',  ( 2.229367062499998831, -52.64583333196773651, -3.861377020970580887 ) ) ;
#9624=ORIENTED_EDGE ( 'NONE', *, *, #23606, .T. ) ;
#9626=LINE ( 'NONE', #43714, #58997 ) ;
#9627=CARTESIAN_POINT ( 'NONE',  ( -4.458734124999998549, 1.520833334698927342, 2.574251347313722516 ) ) ;
#9630=CARTESIAN_POINT ( 'NONE',  ( 5.000000000000000000, -59.41666666666665719, -2.886751345948129988 ) ) ;
#9631=CARTESIAN_POINT ( 'NONE',  ( -8.190561711645485556E-16, -155.9375000013655779, 4.458734124999999437 ) ) ;
#9633=( BOUNDED_CURVE ( )  B_SPLINE_CURVE ( 2, ( #8102, #18681, #48259, #14163, #4217, #17746, #63078, #3283, #47947 ),
 .UNSPECIFIED., .F., .F. ) 
 B_SPLINE_CURVE_WITH_KNOTS ( ( 3, 2, 2, 2, 3 ),
 ( 0.6062499999999999556, 0.6069444444444443976, 0.6083333333333332815, 0.6097222222222222765, 0.6104166666666667185 ),
 .UNSPECIFIED. ) 
 CURVE ( )  GEOMETRIC_REPRESENTATION_ITEM ( )  RATIONAL_B_SPLINE_CURVE ( ( 0.9330127018922194093, 0.9330127018922194093, 1.000000000000000000, 0.8660254037844387076, 1.000000000000000000, 0.8660254037844387076, 1.000000000000000000, 0.9330127018922194093, 0.9330127018922194093 ) ) 
 REPRESENTATION_ITEM ( '' )  );
#9634=CARTESIAN_POINT ( 'NONE',  ( -2.071067811865475061, -163.6875000000000000, -5.000000000000000888 ) ) ;
#9635=CARTESIAN_POINT ( 'NONE',  ( -1.339745962155589165, 10.79465819873851729, -5.000000000000014211 ) ) ;
#9637=CARTESIAN_POINT ( 'NONE',  ( 4.458734124999999437, -8.062499998634404363, -5.460374474430324690E-16 ) ) ;
#9638=CARTESIAN_POINT ( 'NONE',  ( -4.458734124999998549, -48.47916666530106511, 2.574251347313722516 ) ) ;
#9640=CARTESIAN_POINT ( 'NONE',  ( -9.184850993605147944E-16, -162.3750000027311842, 5.000000000000000000 ) ) ;
#9641=CARTESIAN_POINT ( 'NONE',  ( -1.846868145590734756, -147.1250000013656063, -4.458734125000000326 ) ) ;
#9643=CARTESIAN_POINT ( 'NONE',  ( 5.000000000000000888, 8.416666666666666075, 2.886751345948126879 ) ) ;
#9644=ORIENTED_EDGE ( 'NONE', *, *, #23528, .F. ) ;
#9647=CARTESIAN_POINT ( 'NONE',  ( 5.000000000000000000, -2.291666663935477466, -2.886751345948130876 ) ) ;
#9648=ORIENTED_EDGE ( 'NONE', *, *, #57116, .F. ) ;
#9651=CARTESIAN_POINT ( 'NONE',  ( -2.499999999999996447, -50.83333333333332860, 4.330127018922195425 ) ) ;
#9652=CARTESIAN_POINT ( 'NONE',  ( 2.229367062499998831, -0.6458333319677399542, -3.861377020970580887 ) ) ;
#9653=CYLINDRICAL_SURFACE ( 'NONE', #6947, 5.000000000000000000 ) ;
#9654=CARTESIAN_POINT ( 'NONE',  ( 3.152801135295367541, -154.3125000013656063, -3.152801135295367541 ) ) ;
#9656=ORIENTED_EDGE ( 'NONE', *, *, #10148, .F. ) ;
#9659=CARTESIAN_POINT ( 'NONE',  ( 1.339745962155615144, -40.70534180126147561, 4.999999999999999112 ) ) ;
#9662=CARTESIAN_POINT ( 'NONE',  ( 1.339745962155613146, 29.70534180126147561, -4.999999999999999112 ) ) ;
#9668=VERTEX_POINT ( 'NONE', #61533 ) ;
#9669=CARTESIAN_POINT ( 'NONE',  ( -4.458734124999997661, 16.77083333469892779, 2.574251347313722516 ) ) ;
#9671=CARTESIAN_POINT ( 'NONE',  ( -4.458734124999999437, -7.562499998634404363, 0.000000000000000000 ) ) ;
#9674=CARTESIAN_POINT ( 'NONE',  ( -4.458734124999999437, -168.9375000013656063, -5.460374474430324690E-16 ) ) ;
#9680=CARTESIAN_POINT ( 'NONE',  ( 1.975475456537005874E-15, -54.62499999726880873, 5.000000000000000000 ) ) ;
#9681=CARTESIAN_POINT ( 'NONE',  ( 1.339745962155612702, -69.29465819873850307, -5.000000000000000000 ) ) ;
#9682=CARTESIAN_POINT ( 'NONE',  ( -4.458734125000000326, -152.1250000013655779, 1.846868145590734089 ) ) ;
#9684=CARTESIAN_POINT ( 'NONE',  ( -6.972266317189433020E-16, -46.24999999999999289, -5.000000000000000000 ) ) ;
#9686=ORIENTED_EDGE ( 'NONE', *, *, #37074, .T. ) ;
#9689=CARTESIAN_POINT ( 'NONE',  ( -5.000000000000000000, -87.95833333060213022, -2.886751345948128211 ) ) ;
#9690=CARTESIAN_POINT ( 'NONE',  ( -4.999999999999999112, 5.083333333333332149, 2.886751345948131764 ) ) ;
#9692=CARTESIAN_POINT ( 'NONE',  ( 9.457646018065525792E-16, -66.06249999863440792, 5.148502694627439702 ) ) ;
#9694=CARTESIAN_POINT ( 'NONE',  ( -5.000000000000000000, -0.8749999972688139449, 0.000000000000000000 ) ) ;
#9695=CARTESIAN_POINT ( 'NONE',  ( 4.458734124999999437, -35.81249999863440792, -5.460374474430324690E-16 ) ) ;
#9697=CARTESIAN_POINT ( 'NONE',  ( 5.000000000000000888, 17.54166666939785557, 2.886751345948126879 ) ) ;
#9698=CARTESIAN_POINT ( 'NONE',  ( 0.000000000000000000, -170.0000000000000000, 0.000000000000000000 ) ) ;
#9700=CARTESIAN_POINT ( 'NONE',  ( 5.000000000000000888, -47.58333333333333570, 2.886751345948126879 ) ) ;
#9701=DIRECTION ( 'NONE',  ( -0.000000000000000000, 1.000000000000000000, -0.000000000000000000 ) ) ;
#9703=CARTESIAN_POINT ( 'NONE',  ( 5.000000000000000000, -64.50000000000000000, -6.123233995736766282E-16 ) ) ;
#9704=CARTESIAN_POINT ( 'NONE',  ( 4.458734124999999437, -68.81249999863439371, -5.460374474430324690E-16 ) ) ;
#9705=CARTESIAN_POINT ( 'NONE',  ( -4.458734125000001214, -145.1250000013655779, 1.846868145590734089 ) ) ;
#9706=CARTESIAN_POINT ( 'NONE',  ( -4.458734124999999437, -79.31249999863440792, 0.000000000000000000 ) ) ;
#9707=EDGE_CURVE ( 'NONE', #36379, #32107, #60893, .T. ) ;
#9709=( BOUNDED_CURVE ( )  B_SPLINE_CURVE ( 2, ( #348, #48899, #52795, #39560, #58564, #38315, #24463, #19950, #59202 ),
 .UNSPECIFIED., .F., .F. ) 
 B_SPLINE_CURVE_WITH_KNOTS ( ( 3, 2, 2, 2, 3 ),
 ( 0.006250000000000000347, 0.006944444444444444059, 0.008333333333333333218, 0.009722222222222222376, 0.01041666666666666782 ),
 .UNSPECIFIED. ) 
 CURVE ( )  GEOMETRIC_REPRESENTATION_ITEM ( )  RATIONAL_B_SPLINE_CURVE ( ( 0.9330127018922194093, 0.9330127018922194093, 1.000000000000000000, 0.8660254037844387076, 1.000000000000000000, 0.8660254037844387076, 1.000000000000000000, 0.9330127018922191873, 0.9330127018922192983 ) ) 
 REPRESENTATION_ITEM ( '' )  );
#9710=CARTESIAN_POINT ( 'NONE',  ( -2.229367062500000163, -30.72916666530107221, -3.861377020970580443 ) ) ;
#9711=CARTESIAN_POINT ( 'NONE',  ( -2.500000000000000444, -69.04166666393547303, -4.330127018922193649 ) ) ;
#9712=ORIENTED_EDGE ( 'NONE', *, *, #16715, .F. ) ;
#9714=VERTEX_POINT ( 'NONE', #16817 ) ;
#9717=ORIENTED_EDGE ( 'NONE', *, *, #30182, .T. ) ;
#9719=CARTESIAN_POINT ( 'NONE',  ( -2.500000000000000444, -3.166666666666664742, -4.330127018922193649 ) ) ;
#9720=CARTESIAN_POINT ( 'NONE',  ( -3.152548672688508926E-16, -61.81249999863440081, -5.148502694627439702 ) ) ;
#9723=( BOUNDED_CURVE ( )  B_SPLINE_CURVE ( 2, ( #12133, #46234, #51388, #56533, #7008, #47491, #21482, #61046, #36272 ),
 .UNSPECIFIED., .F., .F. ) 
 B_SPLINE_CURVE_WITH_KNOTS ( ( 3, 2, 2, 2, 3 ),
 ( 0.6437500000000000444, 0.6444444444444444864, 0.6458333333333333703, 0.6472222222222222543, 0.6479166666666666963 ),
 .UNSPECIFIED. ) 
 CURVE ( )  GEOMETRIC_REPRESENTATION_ITEM ( )  RATIONAL_B_SPLINE_CURVE ( ( 0.9330127018922194093, 0.9330127018922194093, 1.000000000000000000, 0.8660254037844387076, 1.000000000000000000, 0.8660254037844387076, 1.000000000000000000, 0.9330127018922194093, 0.9330127018922194093 ) ) 
 REPRESENTATION_ITEM ( '' )  );
#9725=CARTESIAN_POINT ( 'NONE',  ( 6.123233995736766282E-16, -170.0000000000000000, -5.000000000000000000 ) ) ;
#9726=CARTESIAN_POINT ( 'NONE',  ( 1.975475456537005874E-15, -59.62499999726880873, 5.000000000000000000 ) ) ;
#9727=CARTESIAN_POINT ( 'NONE',  ( -2.229367062499996610, 13.85416666803226171, 3.861377020970582219 ) ) ;
#9729=CARTESIAN_POINT ( 'NONE',  ( 5.000000000000000000, -32.41666666666666430, -2.886751345948130876 ) ) ;
#9730=CARTESIAN_POINT ( 'NONE',  ( -4.458734124999999437, -167.0000000013655779, -1.846868145590735644 ) ) ;
#9733=CARTESIAN_POINT ( 'NONE',  ( -4.999999999999998224, -51.79166666393547303, 2.886751345948131764 ) ) ;
#9743=CARTESIAN_POINT ( 'NONE',  ( 2.229367062499998831, 9.104166668032261711, -3.861377020970580887 ) ) ;
#9744=CARTESIAN_POINT ( 'NONE',  ( 1.975475456537005874E-15, -9.624999997268814056, 5.000000000000000000 ) ) ;
#9746=CARTESIAN_POINT ( 'NONE',  ( -3.535533905932738641, -147.5000000027311842, 3.535533905932737309 ) ) ;
#9751=CARTESIAN_POINT ( 'NONE',  ( 5.000000000000000000, -143.0625000000000000, 2.071067811865478614 ) ) ;
#9753=CARTESIAN_POINT ( 'NONE',  ( 4.458734124999999437, -166.6875000013655779, 0.000000000000000000 ) ) ;
#9754=CARTESIAN_POINT ( 'NONE',  ( -2.229367062500000163, -32.47916666530106511, -3.861377020970580443 ) ) ;
#9756=CYLINDRICAL_SURFACE ( 'NONE', #5093, 5.000000000000000000 ) ;
#9758=CARTESIAN_POINT ( 'NONE',  ( 2.730187237215162345E-16, -143.1875000013656063, -4.458734124999999437 ) ) ;
#9760=CARTESIAN_POINT ( 'NONE',  ( 2.229367062499998831, 27.10416666803225993, -3.861377020970580887 ) ) ;
#9761=EDGE_LOOP ( 'NONE', ( #2779, #52298, #17042, #23263 ) ) ;
#9762=CARTESIAN_POINT ( 'NONE',  ( 2.229367062499998831, -61.89583333196774362, -3.861377020970580887 ) ) ;
#9764=CARTESIAN_POINT ( 'NONE',  ( -2.499999999999996447, 21.16666666666666785, 4.330127018922195425 ) ) ;
#9767=CARTESIAN_POINT ( 'NONE',  ( 4.458734125000001214, -8.895833331967736513, 2.574251347313718519 ) ) ;
#9768=CARTESIAN_POINT ( 'NONE',  ( -1.339745962155610925, 4.330341803992665106, 5.000000000000000000 ) ) ;
#9769=FACE_OUTER_BOUND ( 'NONE', #32489, .T. ) ;
#9773=( BOUNDED_CURVE ( )  B_SPLINE_CURVE ( 2, ( #27786, #37763, #42265, #3676, #57394, #52560, #47411, #56763, #12684 ),
 .UNSPECIFIED., .F., .F. ) 
 B_SPLINE_CURVE_WITH_KNOTS ( ( 3, 2, 2, 2, 3 ),
 ( 0.9583333333333331483, 0.9624999999999998002, 0.9666666666666665630, 0.9708333333333332149, 0.9749999999999998668 ),
 .UNSPECIFIED. ) 
 CURVE ( )  GEOMETRIC_REPRESENTATION_ITEM ( )  RATIONAL_B_SPLINE_CURVE ( ( 1.000000000000003997, 0.9238795325112826307, 1.000000000000000000, 0.9238795325112867385, 1.000000000000000000, 0.9238795325112867385, 1.000000000000000000, 0.9238795325112887369, 0.9999999999999980016 ) ) 
 REPRESENTATION_ITEM ( '' )  );
#9776=CARTESIAN_POINT ( 'NONE',  ( 2.229367062499998831, -56.64583333196773651, -3.861377020970580887 ) ) ;
#9777=CARTESIAN_POINT ( 'NONE',  ( 1.846868145590736310, -157.8750000013656063, 4.458734124999999437 ) ) ;
#9778=EDGE_CURVE ( 'NONE', #24820, #7044, #22928, .T. ) ;
#9779=CARTESIAN_POINT ( 'NONE',  ( 2.499999999999998668, -51.20833333060213732, -4.330127018922193649 ) ) ;
#9780=ORIENTED_EDGE ( 'NONE', *, *, #22199, .T. ) ;
#9781=CARTESIAN_POINT ( 'NONE',  ( 4.458734124999998549, 7.020833334698929562, -2.574251347313721627 ) ) ;
#9783=CARTESIAN_POINT ( 'NONE',  ( 2.500000000000002220, -56.66666666666667140, 4.330127018922192761 ) ) ;
#9784=CARTESIAN_POINT ( 'NONE',  ( -1.846868145590734756, -156.1250000013655779, -4.458734125000000326 ) ) ;
#9789=DIRECTION ( 'NONE',  ( -0.000000000000000000, 1.000000000000000000, -0.000000000000000000 ) ) ;
#9790=CARTESIAN_POINT ( 'NONE',  ( 9.457646018065525792E-16, -41.31249999863440081, 5.148502694627439702 ) ) ;
#9791=ORIENTED_EDGE ( 'NONE', *, *, #45389, .F. ) ;
#9792=CARTESIAN_POINT ( 'NONE',  ( 6.123233995736766282E-16, -170.0000000000000000, -5.000000000000000000 ) ) ;
#9793=ADVANCED_FACE ( 'NONE', ( #62159 ), #57961, .T. ) ;
#9797=CARTESIAN_POINT ( 'NONE',  ( -4.458734124999999437, 27.60416666803226349, -2.574251347313719407 ) ) ;
#9799=DIRECTION ( 'NONE',  ( 0.000000000000000000, 0.000000000000000000, 1.000000000000000000 ) ) ;
#9800=CARTESIAN_POINT ( 'NONE',  ( 5.275681513340003914E-14, 10.87500000273118239, -5.000000000000000000 ) ) ;
#9801=CARTESIAN_POINT ( 'NONE',  ( 2.499999999999998668, -52.20833333060213732, -4.330127018922193649 ) ) ;
#9809=CARTESIAN_POINT ( 'NONE',  ( -2.500000000000000444, -61.16666666666666430, -4.330127018922193649 ) ) ;
#9810=CARTESIAN_POINT ( 'NONE',  ( -4.458734124999999437, -89.64583333196773651, -2.574251347313719407 ) ) ;
#9813=ORIENTED_EDGE ( 'NONE', *, *, #44502, .T. ) ;
#9815=CARTESIAN_POINT ( 'NONE',  ( 5.000000000000000000, -163.1250000027311842, 0.000000000000000000 ) ) ;
#9817=EDGE_CURVE ( 'NONE', #37570, #60372, #37700, .T. ) ;
#9827=CARTESIAN_POINT ( 'NONE',  ( 4.458734124999999437, -11.81249999863440081, -5.460374474430324690E-16 ) ) ;
#9829=CARTESIAN_POINT ( 'NONE',  ( -5.000000000000000888, -156.5625000000000284, -2.071067811865475949 ) ) ;
#9831=ORIENTED_EDGE ( 'NONE', *, *, #13105, .F. ) ;
#9832=CARTESIAN_POINT ( 'NONE',  ( -2.229367062499996610, -41.39583333196773651, 3.861377020970582219 ) ) ;
#9838=CARTESIAN_POINT ( 'NONE',  ( -2.229367062499996610, 7.854166668032260823, 3.861377020970582219 ) ) ;
#9840=CARTESIAN_POINT ( 'NONE',  ( 5.000000000000000000, -37.29166666393548724, -2.886751345948130876 ) ) ;
#9841=CARTESIAN_POINT ( 'NONE',  ( 4.458734124999998549, -89.97916666530106511, -2.574251347313721627 ) ) ;
#9842=CARTESIAN_POINT ( 'NONE',  ( 4.458734124999998549, 21.02083333469892779, -2.574251347313721627 ) ) ;
#9844=CARTESIAN_POINT ( 'NONE',  ( -5.000000000000000000, 12.12500000273118772, 0.000000000000000000 ) ) ;
#9845=ORIENTED_EDGE ( 'NONE', *, *, #27519, .T. ) ;
#9846=CARTESIAN_POINT ( 'NONE',  ( -1.339745962155613812, -7.080341798530293218, -5.000000000000000000 ) ) ;
#9847=ORIENTED_EDGE ( 'NONE', *, *, #23689, .T. ) ;
#9849=CARTESIAN_POINT ( 'NONE',  ( -5.000000000000000000, -35.08333333333332149, -2.886751345948128211 ) ) ;
#9850=CARTESIAN_POINT ( 'NONE',  ( -2.229367062499996610, -40.14583333196773651, 3.861377020970582219 ) ) ;
#9854=CARTESIAN_POINT ( 'NONE',  ( -2.500000000000000444, -33.04166666393547303, -4.330127018922193649 ) ) ;
#9856=CARTESIAN_POINT ( 'NONE',  ( -4.458734124999998549, -67.22916666530106511, 2.574251347313722516 ) ) ;
#9859=CARTESIAN_POINT ( 'NONE',  ( -4.458734124999999437, -13.39583333196774184, -2.574251347313719407 ) ) ;
#9860=CARTESIAN_POINT ( 'NONE',  ( -2.229367062499996610, -13.39583333196774007, 3.861377020970582219 ) ) ;
#9861=ORIENTED_EDGE ( 'NONE', *, *, #27594, .F. ) ;
#9862=EDGE_CURVE ( 'NONE', #20081, #44647, #23857, .T. ) ;
#9863=CARTESIAN_POINT ( 'NONE',  ( -2.500000000000000444, -81.16666666666667140, -4.330127018922193649 ) ) ;
#9864=CARTESIAN_POINT ( 'NONE',  ( 4.458734124999999437, -167.4375000013655779, 0.000000000000000000 ) ) ;
#9866=CARTESIAN_POINT ( 'NONE',  ( -2.499999999999996447, -81.70833333060213022, 4.330127018922195425 ) ) ;
#9867=CARTESIAN_POINT ( 'NONE',  ( -2.500000000000000444, -18.16666666666666430, -4.330127018922193649 ) ) ;
#9870=CARTESIAN_POINT ( 'NONE',  ( -4.458734124999999437, -24.64583333196773651, -2.574251347313719407 ) ) ;
#9874=CARTESIAN_POINT ( 'NONE',  ( -8.190561711645485556E-16, -165.9375000013655779, 4.458734124999999437 ) ) ;
#9877=CARTESIAN_POINT ( 'NONE',  ( 5.000000000000000888, -55.45833333060214443, 2.886751345948126879 ) ) ;
#9883=CARTESIAN_POINT ( 'NONE',  ( -1.846868145590734756, -145.3750000013656063, -4.458734124999999437 ) ) ;
#9889=ORIENTED_EDGE ( 'NONE', *, *, #16937, .T. ) ;
#9890=CARTESIAN_POINT ( 'NONE',  ( 4.458734124999999437, -140.6875000013656063, 0.000000000000000000 ) ) ;
#9895=CARTESIAN_POINT ( 'NONE',  ( 4.458734124999999437, -73.06249999863439371, -5.460374474430324690E-16 ) ) ;
#9896=CARTESIAN_POINT ( 'NONE',  ( -5.000000000000000000, -144.6250000027312126, -6.123233995736766282E-16 ) ) ;
#9897=CARTESIAN_POINT ( 'NONE',  ( 2.500000000000002220, -54.54166666393548013, 4.330127018922192761 ) ) ;
#9900=ORIENTED_EDGE ( 'NONE', *, *, #58890, .F. ) ;
#9906=CARTESIAN_POINT ( 'NONE',  ( -4.458734124999999437, 21.35416666803225993, -2.574251347313719407 ) ) ;
#9907=CARTESIAN_POINT ( 'NONE',  ( -2.500000000000000444, 22.95833333606451632, -4.330127018922193649 ) ) ;
#9909=( BOUNDED_CURVE ( )  B_SPLINE_CURVE ( 2, ( #47161, #60698, #26589, #21773, #61010, #4581, #20012, #5542, #54102 ),
 .UNSPECIFIED., .F., .F. ) 
 B_SPLINE_CURVE_WITH_KNOTS ( ( 3, 2, 2, 2, 3 ),
 ( 0.5729166666666666297, 0.5736111111111110716, 0.5749999999999999556, 0.5763888888888888395, 0.5770833333333332815 ),
 .UNSPECIFIED. ) 
 CURVE ( )  GEOMETRIC_REPRESENTATION_ITEM ( )  RATIONAL_B_SPLINE_CURVE ( ( 0.9330127018922194093, 0.9330127018922194093, 1.000000000000000000, 0.8660254037844387076, 1.000000000000000000, 0.8660254037844387076, 1.000000000000000000, 0.9330127018922194093, 0.9330127018922194093 ) ) 
 REPRESENTATION_ITEM ( '' )  );
#9914=CARTESIAN_POINT ( 'NONE',  ( 2.229367062499998831, 2.354166668032262599, -3.861377020970580887 ) ) ;
#9915=CARTESIAN_POINT ( 'NONE',  ( -3.152548672688508926E-16, -24.81249999863440436, -5.148502694627439702 ) ) ;
#9918=CARTESIAN_POINT ( 'NONE',  ( 4.458734124999999437, 28.18750000136559208, -5.460374474430324690E-16 ) ) ;
#9920=CARTESIAN_POINT ( 'NONE',  ( -6.972266317189433020E-16, -80.12499999726881583, -5.000000000000000000 ) ) ;
#9921=CARTESIAN_POINT ( 'NONE',  ( 2.229367062499998831, -74.89583333196773651, -3.861377020970580887 ) ) ;
#9925=DIRECTION ( 'NONE',  ( 0.000000000000000000, 0.000000000000000000, 1.000000000000000000 ) ) ;
#9926=ORIENTED_EDGE ( 'NONE', *, *, #9504, .T. ) ;
#9929=CARTESIAN_POINT ( 'NONE',  ( -5.000000000000000000, -18.00000000000000355, 0.000000000000000000 ) ) ;
#9930=CARTESIAN_POINT ( 'NONE',  ( 9.457646018065525792E-16, -23.06249999863440792, 5.148502694627439702 ) ) ;
#9931=CARTESIAN_POINT ( 'NONE',  ( -4.458734124999997661, -85.22916666530107932, 2.574251347313722516 ) ) ;
#9932=CARTESIAN_POINT ( 'NONE',  ( -4.458734125000001214, -166.1250000013655779, 1.846868145590734089 ) ) ;
#9933=ADVANCED_FACE ( 'NONE', ( #19336 ), #52183, .T. ) ;
#9934=CARTESIAN_POINT ( 'NONE',  ( -4.999999999999999112, -18.79166666393547658, 2.886751345948131764 ) ) ;
#9935=CARTESIAN_POINT ( 'NONE',  ( -4.458734124999999437, -50.39583333196773651, -2.574251347313719407 ) ) ;
#9936=ORIENTED_EDGE ( 'NONE', *, *, #35825, .T. ) ;
#9938=CARTESIAN_POINT ( 'NONE',  ( 5.000000000000000000, -15.29166666393548191, -2.886751345948130876 ) ) ;
#9939=CARTESIAN_POINT ( 'NONE',  ( -2.229367062499996610, 1.604166668032262155, 3.861377020970582219 ) ) ;
#9940=ORIENTED_EDGE ( 'NONE', *, *, #22922, .T. ) ;
#9942=CARTESIAN_POINT ( 'NONE',  ( -2.499999999999996447, -65.83333333333332860, 4.330127018922195425 ) ) ;
#9943=CARTESIAN_POINT ( 'NONE',  ( 4.458734124999999437, -155.7500000013655779, 1.846868145590737864 ) ) ;
#9945=CARTESIAN_POINT ( 'NONE',  ( 1.975475456537005874E-15, -80.62499999726881583, 5.000000000000000000 ) ) ;
#9946=VECTOR ( 'NONE', #8050, 1000.000000000000000 ) ;
#9947=CARTESIAN_POINT ( 'NONE',  ( -5.000000000000000888, -162.4375000000000568, 2.071067811865474617 ) ) ;
#9951=CARTESIAN_POINT ( 'NONE',  ( 4.458734124999999437, -12.06249999863440081, -5.460374474430324690E-16 ) ) ;
#9952=AXIS2_PLACEMENT_3D ( 'NONE', #26448, #46069, #35153 ) ;
#9953=CARTESIAN_POINT ( 'NONE',  ( -4.458734124999998549, -44.47916666530106511, 2.574251347313722516 ) ) ;
#9955=CARTESIAN_POINT ( 'NONE',  ( 3.152801135295366208, -146.5625000013655779, 3.152801135295367985 ) ) ;
#9959=ORIENTED_EDGE ( 'NONE', *, *, #27519, .F. ) ;
#9969=CARTESIAN_POINT ( 'NONE',  ( 0.000000000000000000, -170.0000000000000000, 0.000000000000000000 ) ) ;
#9972=CARTESIAN_POINT ( 'NONE',  ( 4.458734124999999437, -2.812499998634407472, -5.460374474430324690E-16 ) ) ;
#9973=CARTESIAN_POINT ( 'NONE',  ( 1.339745962155612702, -73.16965819600734733, -5.000000000000000000 ) ) ;
#9974=CARTESIAN_POINT ( 'NONE',  ( -3.152801135295367096, -149.0625000013655779, -3.152801135295367541 ) ) ;
#9976=ORIENTED_EDGE ( 'NONE', *, *, #20106, .T. ) ;
#9978=CARTESIAN_POINT ( 'NONE',  ( -6.972266317189433020E-16, -47.24999999999999289, -5.000000000000000000 ) ) ;
#9982=CARTESIAN_POINT ( 'NONE',  ( -2.500000000000000444, -13.16666666666666607, -4.330127018922193649 ) ) ;
#9987=CARTESIAN_POINT ( 'NONE',  ( -2.500000000000000444, -72.16666666666667140, -4.330127018922193649 ) ) ;
#9988=EDGE_LOOP ( 'NONE', ( #43197, #26517, #28393, #52012 ) ) ;
#9989=CARTESIAN_POINT ( 'NONE',  ( 4.458734125000000326, 17.10416666803225993, 2.574251347313718519 ) ) ;
#9992=CARTESIAN_POINT ( 'NONE',  ( 4.458734124999998549, -7.979166665301073991, -2.574251347313721627 ) ) ;
#9995=CARTESIAN_POINT ( 'NONE',  ( 1.846868145590735200, -167.2500000013655779, -4.458734125000000326 ) ) ;
#9996=CARTESIAN_POINT ( 'NONE',  ( -6.972266317189433020E-16, -21.12499999726881228, -5.000000000000000000 ) ) ;
#9999=AXIS2_PLACEMENT_3D ( 'NONE', #49623, #16165, #40290 ) ;
#10001=CARTESIAN_POINT ( 'NONE',  ( -2.499999999999996447, -76.83333333333334281, 4.330127018922195425 ) ) ;
#10002=CARTESIAN_POINT ( 'NONE',  ( 1.975475456537005874E-15, 11.24999999999999822, 5.000000000000000000 ) ) ;
#10004=AXIS2_PLACEMENT_3D ( 'NONE', #5632, #44858, #821 ) ;
#10005=CARTESIAN_POINT ( 'NONE',  ( 4.458734124999997661, -151.7500000013656063, 1.846868145590737864 ) ) ;
#10013=LINE ( 'NONE', #53446, #57633 ) ;
#10014=CARTESIAN_POINT ( 'NONE',  ( -2.500000000000000444, -0.1666666666666656582, -4.330127018922193649 ) ) ;
#10015=CARTESIAN_POINT ( 'NONE',  ( 2.229367062500001939, -67.97916666530106511, 3.861377020970579999 ) ) ;
#10018=CARTESIAN_POINT ( 'NONE',  ( -5.000000000000000000, 0.1250000027311869155, 0.000000000000000000 ) ) ;
#10019=CARTESIAN_POINT ( 'NONE',  ( -4.458734124999999437, -32.39583333196773651, -2.574251347313719407 ) ) ;
#10021=FACE_OUTER_BOUND ( 'NONE', #20874, .T. ) ;
#10022=CARTESIAN_POINT ( 'NONE',  ( -5.000000000000000000, -47.87499999726880873, 0.000000000000000000 ) ) ;
#10024=CARTESIAN_POINT ( 'NONE',  ( 5.000000000000000000, -51.41666666666666430, -2.886751345948129988 ) ) ;
#10025=CARTESIAN_POINT ( 'NONE',  ( -6.972266317189433020E-16, -17.12499999726881583, -5.000000000000000000 ) ) ;
#10027=CARTESIAN_POINT ( 'NONE',  ( -6.972266317189433020E-16, -64.12499999726880162, -5.000000000000000000 ) ) ;
#10028=CARTESIAN_POINT ( 'NONE',  ( 4.458734124999998549, -70.72916666530107932, -2.574251347313721627 ) ) ;
#10029=CARTESIAN_POINT ( 'NONE',  ( 1.846868145590736310, -142.8750000013656063, 4.458734124999999437 ) ) ;
#10030=CARTESIAN_POINT ( 'NONE',  ( -2.229367062500000163, -83.47916666530106511, -3.861377020970580443 ) ) ;
#10032=CARTESIAN_POINT ( 'NONE',  ( 4.458734125000001214, -28.14583333196774007, 2.574251347313718519 ) ) ;
#10033=CARTESIAN_POINT ( 'NONE',  ( 2.500000000000002220, -70.54166666393547303, 4.330127018922192761 ) ) ;
#10040=CARTESIAN_POINT ( 'NONE',  ( -6.972266317189433020E-16, -32.12499999726880873, -5.000000000000000000 ) ) ;
#10042=CARTESIAN_POINT ( 'NONE',  ( 1.975475456537005874E-15, -75.62499999726880162, 5.000000000000000000 ) ) ;
#10043=CARTESIAN_POINT ( 'NONE',  ( 4.458734124999998549, -56.97916666530107932, -2.574251347313721627 ) ) ;
#10044=VECTOR ( 'NONE', #38949, 1000.000000000000000 ) ;
#10046=ORIENTED_EDGE ( 'NONE', *, *, #17824, .F. ) ;
#10049=CARTESIAN_POINT ( 'NONE',  ( 2.229367062500001939, 14.02083333469892779, 3.861377020970579999 ) ) ;
#10051=CARTESIAN_POINT ( 'NONE',  ( 1.339745962155612702, -32.29465819873852439, -5.000000000000000000 ) ) ;
#10052=CARTESIAN_POINT ( 'NONE',  ( -4.458734125000000326, -163.8750000013656063, 1.846868145590734089 ) ) ;
#10055=CARTESIAN_POINT ( 'NONE',  ( 1.975475456537005874E-15, -69.62499999726880162, 5.000000000000000000 ) ) ;
#10061=CARTESIAN_POINT ( 'NONE',  ( -6.972266317189433020E-16, -21.24999999999999289, -5.000000000000000000 ) ) ;
#10067=CARTESIAN_POINT ( 'NONE',  ( 4.458734124999998549, 6.020833334698928674, -2.574251347313721627 ) ) ;
#10070=CARTESIAN_POINT ( 'NONE',  ( -5.000000000000000888, -149.5625000027311842, 2.071067811865474617 ) ) ;
#10072=EDGE_CURVE ( 'NONE', #31090, #45744, #17693, .T. ) ;
#10076=CARTESIAN_POINT ( 'NONE',  ( 2.071067811865475505, -143.8125000000000000, -5.000000000000000888 ) ) ;
#10079=CARTESIAN_POINT ( 'NONE',  ( 4.458734124999997661, -163.7500000013655779, 1.846868145590737864 ) ) ;
#10080=CARTESIAN_POINT ( 'NONE',  ( -4.458734124999999437, -37.39583333196773651, -2.574251347313719407 ) ) ;
#10084=CARTESIAN_POINT ( 'NONE',  ( -3.152801135295367096, -142.0625000013655779, -3.152801135295367541 ) ) ;
#10085=VERTEX_POINT ( 'NONE', #50199 ) ;
#10086=CARTESIAN_POINT ( 'NONE',  ( -4.458734124999999437, 29.43750000136559208, 0.000000000000000000 ) ) ;
#10088=CARTESIAN_POINT ( 'NONE',  ( 9.457646018065525792E-16, -63.31249999863440792, 5.148502694627439702 ) ) ;
#10092=CARTESIAN_POINT ( 'NONE',  ( 1.060575238724906964E-15, 11.25000000000000000, 5.773502691896257311 ) ) ;
#10095=CARTESIAN_POINT ( 'NONE',  ( -2.229367062500000163, -48.47916666530106511, -3.861377020970580443 ) ) ;
#10096=CARTESIAN_POINT ( 'NONE',  ( -4.458734124999999437, -6.395833331967740953, -2.574251347313719407 ) ) ;
#10101=CARTESIAN_POINT ( 'NONE',  ( 5.000000000000000000, 21.70833333606451987, -2.886751345948130876 ) ) ;
#10104=CARTESIAN_POINT ( 'NONE',  ( 4.458734124999998549, -53.72916666530106511, -2.574251347313721627 ) ) ;
#10105=CARTESIAN_POINT ( 'NONE',  ( -8.190561711645485556E-16, -155.9375000013655779, 4.458734124999999437 ) ) ;
#10108=CARTESIAN_POINT ( 'NONE',  ( -2.500000000000000444, -58.04166666393548013, -4.330127018922193649 ) ) ;
#10111=CARTESIAN_POINT ( 'NONE',  ( -4.458734124999998549, 5.520833334698927786, 2.574251347313722516 ) ) ;
#10113=DIRECTION ( 'NONE',  ( 0.000000000000000000, 0.000000000000000000, 1.000000000000000000 ) ) ;
#10114=CARTESIAN_POINT ( 'NONE',  ( -9.184850993605147944E-16, -160.3750000027311842, 5.000000000000000000 ) ) ;
#10115=CARTESIAN_POINT ( 'NONE',  ( -4.458734124999999437, -157.9375000013655779, -5.460374474430324690E-16 ) ) ;
#10116=ORIENTED_EDGE ( 'NONE', *, *, #16497, .T. ) ;
#10119=CARTESIAN_POINT ( 'NONE',  ( 3.535533905932738197, -161.0000000027312126, -3.535533905932738197 ) ) ;
#10120=CARTESIAN_POINT ( 'NONE',  ( 2.229367062500001939, -44.22916666530106511, 3.861377020970579999 ) ) ;
#10121=ORIENTED_EDGE ( 'NONE', *, *, #20868, .T. ) ;
#10126=CARTESIAN_POINT ( 'NONE',  ( 2.229367062499998831, -89.89583333196773651, -3.861377020970580887 ) ) ;
#10135=VECTOR ( 'NONE', #44199, 1000.000000000000000 ) ;
#10136=CARTESIAN_POINT ( 'NONE',  ( -6.972266317189433020E-16, -79.12499999726881583, -5.000000000000000000 ) ) ;
#10140=FACE_OUTER_BOUND ( 'NONE', #36728, .T. ) ;
#10144=CARTESIAN_POINT ( 'NONE',  ( -5.000000000000000888, -143.6875000027312126, -2.071067811865475949 ) ) ;
#10146=CARTESIAN_POINT ( 'NONE',  ( -9.184850993605147944E-16, -162.3750000027311842, 5.000000000000000000 ) ) ;
#10148=EDGE_CURVE ( 'NONE', #8617, #45777, #59220, .T. ) ;
#10149=CARTESIAN_POINT ( 'NONE',  ( 3.061616997868383141E-16, -158.7500000000000000, -5.000000000000000000 ) ) ;
#10151=CARTESIAN_POINT ( 'NONE',  ( -6.972266317189433020E-16, -15.12499999726881050, -5.000000000000000000 ) ) ;
#10158=CARTESIAN_POINT ( 'NONE',  ( -6.972266317189433020E-16, -54.24999999999999289, -5.000000000000000000 ) ) ;
#10159=CARTESIAN_POINT ( 'NONE',  ( -4.458734124999999437, -20.39583333196774362, -2.574251347313719407 ) ) ;
#10161=CARTESIAN_POINT ( 'NONE',  ( 3.061616997868383141E-16, -155.7500000000000000, -5.000000000000000000 ) ) ;
#10164=CARTESIAN_POINT ( 'NONE',  ( 2.229367062500001939, -45.22916666530106511, 3.861377020970579999 ) ) ;
#10168=CARTESIAN_POINT ( 'NONE',  ( -1.339745962155613146, 27.33034180399266333, 5.000000000000000000 ) ) ;
#10171=CARTESIAN_POINT ( 'NONE',  ( 2.229367062500001939, 11.02083333469892956, 3.861377020970579999 ) ) ;
#10172=EDGE_CURVE ( 'NONE', #23665, #57819, #14822, .T. ) ;
#10176=CARTESIAN_POINT ( 'NONE',  ( -4.458734124999999437, -89.64583333196773651, -2.574251347313719407 ) ) ;
#10177=CARTESIAN_POINT ( 'NONE',  ( 9.457646018065525792E-16, 20.68750000136559564, 5.148502694627439702 ) ) ;
#10179=CARTESIAN_POINT ( 'NONE',  ( -3.535250795749689387E-16, 8.875000002731184168, -5.773502691896257311 ) ) ;
#10181=CARTESIAN_POINT ( 'NONE',  ( -5.000000000000000000, -6.958333330602150646, -2.886751345948128211 ) ) ;
#10182=EDGE_LOOP ( 'NONE', ( #25107, #46829, #33374, #28603 ) ) ;
#10184=CARTESIAN_POINT ( 'NONE',  ( -2.499999999999996447, -31.83333333333333215, 4.330127018922195425 ) ) ;
#10185=CARTESIAN_POINT ( 'NONE',  ( 2.229367062500001939, -35.97916666530107221, 3.861377020970579999 ) ) ;
#10188=CARTESIAN_POINT ( 'NONE',  ( 2.499999999999998668, -37.20833333060213732, -4.330127018922193649 ) ) ;
#10191=CARTESIAN_POINT ( 'NONE',  ( -2.229367062499996610, -14.14583333196774184, 3.861377020970582219 ) ) ;
#10192=CARTESIAN_POINT ( 'NONE',  ( 2.229367062500001939, -12.22916666530107044, 3.861377020970579999 ) ) ;
#10194=CARTESIAN_POINT ( 'NONE',  ( 5.000000000000000000, -84.41666666666667140, -2.886751345948129988 ) ) ;
#10195=CARTESIAN_POINT ( 'NONE',  ( -3.152801135295367096, -167.0625000013656063, -3.152801135295367541 ) ) ;
#10197=CARTESIAN_POINT ( 'NONE',  ( -3.535250795749689387E-16, -83.12499999726880162, -5.773502691896257311 ) ) ;
#10201=CARTESIAN_POINT ( 'NONE',  ( -2.229367062500000163, -26.72916666530106866, -3.861377020970580443 ) ) ;
#10204=CARTESIAN_POINT ( 'NONE',  ( 4.458734124999999437, -162.6875000013655779, 0.000000000000000000 ) ) ;
#10205=EDGE_CURVE ( 'NONE', #16047, #41941, #29616, .T. ) ;
#10207=CARTESIAN_POINT ( 'NONE',  ( 5.000000000000000888, -147.9375000000000000, -2.071067811865475505 ) ) ;
#10208=VERTEX_POINT ( 'NONE', #34773 ) ;
#10210=CARTESIAN_POINT ( 'NONE',  ( 2.229367062499998831, -72.89583333196773651, -3.861377020970580887 ) ) ;
#10213=CARTESIAN_POINT ( 'NONE',  ( 1.846868145590735200, -146.5000000013656347, -4.458734124999999437 ) ) ;
#10214=CYLINDRICAL_SURFACE ( 'NONE', #45604, 5.000000000000000000 ) ;
#10222=CARTESIAN_POINT ( 'NONE',  ( -2.229367062499996610, -72.39583333196773651, 3.861377020970582219 ) ) ;
#10225=FACE_OUTER_BOUND ( 'NONE', #39134, .T. ) ;
#10226=CARTESIAN_POINT ( 'NONE',  ( 1.060575238724906964E-15, -68.74999999999998579, 5.773502691896257311 ) ) ;
#10233=CARTESIAN_POINT ( 'NONE',  ( -6.972266317189433020E-16, -16.12499999726881228, -5.000000000000000000 ) ) ;
#10235=EDGE_CURVE ( 'NONE', #45336, #50575, #6600, .T. ) ;
#10236=CARTESIAN_POINT ( 'NONE',  ( -3.152548672688508926E-16, 17.18750000136559564, -5.148502694627439702 ) ) ;
#10237=CARTESIAN_POINT ( 'NONE',  ( -5.000000000000000000, 27.00000000000000000, 0.000000000000000000 ) ) ;
#10245=CARTESIAN_POINT ( 'NONE',  ( -2.229367062500000163, 2.520833334698928230, -3.861377020970580443 ) ) ;
#10246=ORIENTED_EDGE ( 'NONE', *, *, #43342, .F. ) ;
#10247=CARTESIAN_POINT ( 'NONE',  ( 4.458734125000000326, -31.14583333196773651, 2.574251347313718519 ) ) ;
#10251=CARTESIAN_POINT ( 'NONE',  ( 4.458734124999999437, 26.18750000136559564, -5.460374474430324690E-16 ) ) ;
#10253=EDGE_CURVE ( 'NONE', #7188, #37182, #50171, .T. ) ;
#10255=CARTESIAN_POINT ( 'NONE',  ( -2.229367062499996610, -71.39583333196773651, 3.861377020970582219 ) ) ;
#10257=CARTESIAN_POINT ( 'NONE',  ( -2.500000000000000444, -66.04166666393547303, -4.330127018922193649 ) ) ;
#10258=CARTESIAN_POINT ( 'NONE',  ( 2.499999999999998668, 26.79166666939785202, -4.330127018922193649 ) ) ;
#10260=CARTESIAN_POINT ( 'NONE',  ( 1.339745962155615144, 6.294658198738519062, 4.999999999999999112 ) ) ;
#10262=CARTESIAN_POINT ( 'NONE',  ( 5.000000000000000000, -19.41666666666666075, -2.886751345948129988 ) ) ;
#10263=CARTESIAN_POINT ( 'NONE',  ( 2.229367062499998831, -19.64583333196774007, -3.861377020970580887 ) ) ;
#10264=CARTESIAN_POINT ( 'NONE',  ( 2.229367062499998831, -81.64583333196773651, -3.861377020970580887 ) ) ;
#10265=CARTESIAN_POINT ( 'NONE',  ( -3.535250795749689387E-16, -20.12499999726881228, -5.773502691896257311 ) ) ;
#10266=CARTESIAN_POINT ( 'NONE',  ( -4.458734124999998549, -51.22916666530107221, 2.574251347313722516 ) ) ;
#10270=CARTESIAN_POINT ( 'NONE',  ( 2.229367062499998831, 2.104166668032262599, -3.861377020970580887 ) ) ;
#10271=VERTEX_POINT ( 'NONE', #46334 ) ;
#10273=CARTESIAN_POINT ( 'NONE',  ( -5.000000000000000000, -66.00000000000000000, 0.000000000000000000 ) ) ;
#10274=CARTESIAN_POINT ( 'NONE',  ( -4.458734125000000326, -152.2500000013656347, -1.846868145590735644 ) ) ;
#10276=CARTESIAN_POINT ( 'NONE',  ( -5.000000000000000888, -162.5625000000000000, -2.071067811865475949 ) ) ;
#10277=CARTESIAN_POINT ( 'NONE',  ( 3.061616997868383141E-16, -158.8750000027311842, -5.000000000000000000 ) ) ;
#10280=CARTESIAN_POINT ( 'NONE',  ( -2.229367062499996610, -9.395833331967736513, 3.861377020970582219 ) ) ;
#10281=CARTESIAN_POINT ( 'NONE',  ( 2.229367062500001939, -44.22916666530106511, 3.861377020970579999 ) ) ;
#10282=CYLINDRICAL_SURFACE ( 'NONE', #22182, 5.000000000000000000 ) ;
#10283=CARTESIAN_POINT ( 'NONE',  ( -4.458734125000001214, -147.8750000013656063, 1.846868145590734089 ) ) ;
#10285=CARTESIAN_POINT ( 'NONE',  ( -4.999999999999998224, 21.20833333606451987, 2.886751345948131764 ) ) ;
#10288=CARTESIAN_POINT ( 'NONE',  ( -5.000000000000000000, -5.958333330602149758, -2.886751345948128211 ) ) ;
#10294=CARTESIAN_POINT ( 'NONE',  ( 5.000000000000000000, -19.49999999999999645, -6.123233995736766282E-16 ) ) ;
#10296=CARTESIAN_POINT ( 'NONE',  ( 4.458734125000001214, -4.895833331967740065, 2.574251347313718519 ) ) ;
#10298=CARTESIAN_POINT ( 'NONE',  ( 4.458734124999999437, -150.3750000013655779, -1.846868145590734978 ) ) ;
#10300=ORIENTED_EDGE ( 'NONE', *, *, #9707, .F. ) ;
#10308=CARTESIAN_POINT ( 'NONE',  ( 1.975475456537005874E-15, -74.75000000000000000, 5.000000000000000000 ) ) ;
#10310=CARTESIAN_POINT ( 'NONE',  ( 0.000000000000000000, -170.0000000000000000, 0.000000000000000000 ) ) ;
#10311=CARTESIAN_POINT ( 'NONE',  ( -3.152548672688508926E-16, 16.43750000136559564, -5.148502694627439702 ) ) ;
#10313=ORIENTED_EDGE ( 'NONE', *, *, #14877, .F. ) ;
#10315=CARTESIAN_POINT ( 'NONE',  ( 2.229367062499998831, -9.895833331967738289, -3.861377020970580887 ) ) ;
#10316=EDGE_CURVE ( 'NONE', #22477, #12901, #32520, .T. ) ;
#10318=CARTESIAN_POINT ( 'NONE',  ( 4.458734124999999437, -168.4375000013656063, 0.000000000000000000 ) ) ;
#10324=CARTESIAN_POINT ( 'NONE',  ( 2.499999999999998668, -38.33333333333332860, -4.330127018922193649 ) ) ;
#10327=CARTESIAN_POINT ( 'NONE',  ( 1.846868145590735200, -154.5000000013656347, -4.458734124999999437 ) ) ;
#10329=FACE_OUTER_BOUND ( 'NONE', #24922, .T. ) ;
#10336=CARTESIAN_POINT ( 'NONE',  ( 5.000000000000000000, -4.416666666666666075, -2.886751345948129988 ) ) ;
#10337=CARTESIAN_POINT ( 'NONE',  ( -4.458734124999999437, -66.39583333196773651, -2.574251347313719407 ) ) ;
#10340=CARTESIAN_POINT ( 'NONE',  ( -2.499999999999996447, -3.708333330602147537, 4.330127018922195425 ) ) ;
#10341=CARTESIAN_POINT ( 'NONE',  ( -2.229367062500000163, -34.47916666530107221, -3.861377020970580443 ) ) ;
#10342=ORIENTED_EDGE ( 'NONE', *, *, #19755, .F. ) ;
#10343=CARTESIAN_POINT ( 'NONE',  ( -5.000000000000000000, -78.08333333333332860, -2.886751345948128211 ) ) ;
#10345=( BOUNDED_CURVE ( )  B_SPLINE_CURVE ( 2, ( #44434, #44752, #55381, #55058, #59241, #395, #19997, #39925, #39605 ),
 .UNSPECIFIED., .F., .F. ) 
 B_SPLINE_CURVE_WITH_KNOTS ( ( 3, 2, 2, 2, 3 ),
 ( 0.2812500000000000000, 0.2819444444444444420, 0.2833333333333333259, 0.2847222222222222099, 0.2854166666666666519 ),
 .UNSPECIFIED. ) 
 CURVE ( )  GEOMETRIC_REPRESENTATION_ITEM ( )  RATIONAL_B_SPLINE_CURVE ( ( 0.9330127018922194093, 0.9330127018922194093, 1.000000000000000000, 0.8660254037844387076, 1.000000000000000000, 0.8660254037844387076, 1.000000000000000000, 0.9330127018922194093, 0.9330127018922194093 ) ) 
 REPRESENTATION_ITEM ( '' )  );
#10346=CARTESIAN_POINT ( 'NONE',  ( -5.000000000000000000, -52.08333333333332860, -2.886751345948128211 ) ) ;
#10348=( BOUNDED_CURVE ( )  B_SPLINE_CURVE ( 2, ( #22391, #56167, #12090, #51346, #7285, #41992, #52289, #46514, #37488 ),
 .UNSPECIFIED., .F., .F. ) 
 B_SPLINE_CURVE_WITH_KNOTS ( ( 3, 2, 2, 2, 3 ),
 ( 0.8395833333333333481, 0.8402777777777777901, 0.8416666666666666741, 0.8430555555555555580, 0.8437500000000000000 ),
 .UNSPECIFIED. ) 
 CURVE ( )  GEOMETRIC_REPRESENTATION_ITEM ( )  RATIONAL_B_SPLINE_CURVE ( ( 0.9330127018922194093, 0.9330127018922194093, 1.000000000000000000, 0.8660254037844387076, 1.000000000000000000, 0.8660254037844387076, 1.000000000000000000, 0.9330127018922194093, 0.9330127018922194093 ) ) 
 REPRESENTATION_ITEM ( '' )  );
#10350=CARTESIAN_POINT ( 'NONE',  ( -5.000000000000000000, -41.87499999726880873, 0.000000000000000000 ) ) ;
#10351=CARTESIAN_POINT ( 'NONE',  ( -2.229367062499996610, -70.14583333196773651, 3.861377020970582219 ) ) ;
#10352=CARTESIAN_POINT ( 'NONE',  ( 2.730187237215162345E-16, -142.4375000013656063, -4.458734124999999437 ) ) ;
#10353=CARTESIAN_POINT ( 'NONE',  ( -4.458734124999998549, -84.22916666530107932, 2.574251347313722516 ) ) ;
#10355=CARTESIAN_POINT ( 'NONE',  ( -3.152548672688508926E-16, -28.81249999863440436, -5.148502694627439702 ) ) ;
#10356=CARTESIAN_POINT ( 'NONE',  ( 1.060575238724906964E-15, -70.62499999726881583, 5.773502691896257311 ) ) ;
#10357=VERTEX_POINT ( 'NONE', #52111 ) ;
#10358=DIRECTION ( 'NONE',  ( -0.000000000000000000, 1.000000000000000000, -0.000000000000000000 ) ) ;
#10362=ORIENTED_EDGE ( 'NONE', *, *, #6436, .T. ) ;
#10364=CARTESIAN_POINT ( 'NONE',  ( 1.339745962155615144, -12.70534180126147739, 4.999999999999999112 ) ) ;
#10366=CARTESIAN_POINT ( 'NONE',  ( -4.458734124999999437, -57.64583333196773651, -2.574251347313719407 ) ) ;
#10368=EDGE_LOOP ( 'NONE', ( #48610, #7682, #55698, #21779 ) ) ;
#10370=CYLINDRICAL_SURFACE ( 'NONE', #29444, 5.000000000000000000 ) ;
#10371=( BOUNDED_CURVE ( )  B_SPLINE_CURVE ( 2, ( #14205, #19986, #29300, #4878, #39913, #43786, #24499, #54079, #702 ),
 .UNSPECIFIED., .F., .F. ) 
 B_SPLINE_CURVE_WITH_KNOTS ( ( 3, 2, 2, 2, 3 ),
 ( 0.4979166666666666741, 0.4986111111111111160, 0.5000000000000000000, 0.5013888888888888840, 0.5020833333333333259 ),
 .UNSPECIFIED. ) 
 CURVE ( )  GEOMETRIC_REPRESENTATION_ITEM ( )  RATIONAL_B_SPLINE_CURVE ( ( 0.9330127018922194093, 0.9330127018922194093, 1.000000000000000000, 0.8660254037844387076, 1.000000000000000000, 0.8660254037844387076, 1.000000000000000000, 0.9330127018922194093, 0.9330127018922194093 ) ) 
 REPRESENTATION_ITEM ( '' )  );
#10372=CARTESIAN_POINT ( 'NONE',  ( -2.229367062500000163, 11.52083333469892601, -3.861377020970580443 ) ) ;
#10375=CARTESIAN_POINT ( 'NONE',  ( 1.846868145590735200, -160.2500000013656063, -4.458734124999999437 ) ) ;
#10378=CARTESIAN_POINT ( 'NONE',  ( 6.123233995736766282E-16, -170.0000000000000000, -5.000000000000000000 ) ) ;
#10381=CARTESIAN_POINT ( 'NONE',  ( 1.975475456537005874E-15, -36.75000000000000000, 5.000000000000000000 ) ) ;
#10384=CARTESIAN_POINT ( 'NONE',  ( -1.339745962155610925, -72.66965819600733312, 5.000000000000000000 ) ) ;
#10390=CARTESIAN_POINT ( 'NONE',  ( -2.229367062499996610, 5.604166668032261711, 3.861377020970582219 ) ) ;
#10391=( BOUNDED_CURVE ( )  B_SPLINE_CURVE ( 2, ( #27964, #27028, #62398, #56630, #27654, #47587, #3538, #23147, #2917 ),
 .UNSPECIFIED., .F., .F. ) 
 B_SPLINE_CURVE_WITH_KNOTS ( ( 3, 2, 2, 2, 3 ),
 ( 0.3750000000000002776, 0.3791666666666669294, 0.3833333333333336368, 0.3875000000000003442, 0.3916666666666669960 ),
 .UNSPECIFIED. ) 
 CURVE ( )  GEOMETRIC_REPRESENTATION_ITEM ( )  RATIONAL_B_SPLINE_CURVE ( ( 0.9999999999999948930, 0.9238795325112918455, 1.000000000000000000, 0.9238795325112867385, 1.000000000000000000, 0.9238795325112867385, 1.000000000000000000, 0.9238795325112806323, 1.000000000000005995 ) ) 
 REPRESENTATION_ITEM ( '' )  );
#10392=DIRECTION ( 'NONE',  ( -0.000000000000000000, 1.000000000000000000, -0.000000000000000000 ) ) ;
#10394=CARTESIAN_POINT ( 'NONE',  ( 3.535533905932738197, -151.0000000027312126, -3.535533905932738197 ) ) ;
#10399=DIRECTION ( 'NONE',  ( 0.000000000000000000, 0.000000000000000000, 1.000000000000000000 ) ) ;
#10402=CARTESIAN_POINT ( 'NONE',  ( -4.458734124999999437, -165.1875000013655779, -5.460374474430324690E-16 ) ) ;
#10406=CARTESIAN_POINT ( 'NONE',  ( -4.458734124999999437, -142.9375000013656063, -5.460374474430324690E-16 ) ) ;
#10407=EDGE_LOOP ( 'NONE', ( #50431, #38786, #27522, #52949 ) ) ;
#10408=CARTESIAN_POINT ( 'NONE',  ( 2.500000000000002220, -90.54166666393547303, 4.330127018922192761 ) ) ;
#10410=CARTESIAN_POINT ( 'NONE',  ( -2.229367062500000163, -63.72916666530106511, -3.861377020970580443 ) ) ;
#10413=CARTESIAN_POINT ( 'NONE',  ( -2.500000000000000444, 12.83333333333333215, -4.330127018922193649 ) ) ;
#10415=CARTESIAN_POINT ( 'NONE',  ( 4.458734124999999437, -49.81249999863440792, -5.460374474430324690E-16 ) ) ;
#10416=CARTESIAN_POINT ( 'NONE',  ( 4.458734124999998549, -7.729166665301073103, -2.574251347313721627 ) ) ;
#10417=CARTESIAN_POINT ( 'NONE',  ( 3.535533905932736864, -166.2500000027312126, 3.535533905932738641 ) ) ;
#10421=CARTESIAN_POINT ( 'NONE',  ( -5.000000000000000000, -59.08333333333332860, -2.886751345948128211 ) ) ;
#10423=CARTESIAN_POINT ( 'NONE',  ( 2.229367062499998831, -53.64583333196773651, -3.861377020970580887 ) ) ;
#10424=CARTESIAN_POINT ( 'NONE',  ( -1.846868145590734756, -154.3750000013655779, -4.458734125000000326 ) ) ;
#10425=CARTESIAN_POINT ( 'NONE',  ( 2.500000000000002220, -55.54166666393548013, 4.330127018922192761 ) ) ;
#10426=ORIENTED_EDGE ( 'NONE', *, *, #41745, .F. ) ;
#10428=CARTESIAN_POINT ( 'NONE',  ( 4.458734124999998549, 3.020833334698928674, -2.574251347313721627 ) ) ;
#10430=CARTESIAN_POINT ( 'NONE',  ( 1.975475456537005874E-15, -56.75000000000000000, 5.000000000000000000 ) ) ;
#10432=CARTESIAN_POINT ( 'NONE',  ( -1.846868145590737420, -157.7500000013656063, 4.458734124999999437 ) ) ;
#10437=CARTESIAN_POINT ( 'NONE',  ( -2.229367062499996610, -41.39583333196773651, 3.861377020970582219 ) ) ;
#10439=CARTESIAN_POINT ( 'NONE',  ( 1.339745962155637349, 9.830341803992661553, -4.999999999999985789 ) ) ;
#10441=CARTESIAN_POINT ( 'NONE',  ( -4.458734124999999437, 29.68750000136559208, 0.000000000000000000 ) ) ;
#10443=LINE ( 'NONE', #59992, #53164 ) ;
#10445=CARTESIAN_POINT ( 'NONE',  ( -5.000000000000000000, 24.00000000000000000, 0.000000000000000000 ) ) ;
#10447=CYLINDRICAL_SURFACE ( 'NONE', #16120, 5.000000000000000000 ) ;
#10451=CARTESIAN_POINT ( 'NONE',  ( -4.999999999999998224, 5.083333333333332149, 2.886751345948131764 ) ) ;
#10452=FACE_OUTER_BOUND ( 'NONE', #1736, .T. ) ;
#10453=CARTESIAN_POINT ( 'NONE',  ( 2.229367062499998831, -87.89583333196773651, -3.861377020970580887 ) ) ;
#10454=CARTESIAN_POINT ( 'NONE',  ( -2.500000000000000444, 10.95833333606451632, -4.330127018922193649 ) ) ;
#10456=ORIENTED_EDGE ( 'NONE', *, *, #35457, .T. ) ;
#10459=CARTESIAN_POINT ( 'NONE',  ( 3.535533905932738197, -161.0000000027312126, -3.535533905932738197 ) ) ;
#10460=EDGE_LOOP ( 'NONE', ( #44461, #9847, #1211, #1520 ) ) ;
#10462=CARTESIAN_POINT ( 'NONE',  ( 5.000000000000000000, -49.29166666393547303, -2.886751345948130876 ) ) ;
#10464=CARTESIAN_POINT ( 'NONE',  ( 1.975475456537005874E-15, -71.62499999726878741, 5.000000000000000000 ) ) ;
#10471=DIRECTION ( 'NONE',  ( -0.000000000000000000, 1.000000000000000000, -0.000000000000000000 ) ) ;
#10472=CARTESIAN_POINT ( 'NONE',  ( 4.458734124999999437, -18.81249999863440792, -5.460374474430324690E-16 ) ) ;
#10473=CARTESIAN_POINT ( 'NONE',  ( 1.975475456537005874E-15, -75.74999999999998579, 5.000000000000000000 ) ) ;
#10474=CARTESIAN_POINT ( 'NONE',  ( -2.071067811865475061, -154.6875000000000568, -5.000000000000000888 ) ) ;
#10476=CARTESIAN_POINT ( 'NONE',  ( -4.458734124999999437, -155.9375000013655779, -5.460374474430324690E-16 ) ) ;
#10477=ORIENTED_EDGE ( 'NONE', *, *, #14502, .F. ) ;
#10478=CARTESIAN_POINT ( 'NONE',  ( 9.457646018065525792E-16, -45.31249999863440081, 5.148502694627439702 ) ) ;
#10479=CARTESIAN_POINT ( 'NONE',  ( 5.000000000000000888, -44.45833333060214443, 2.886751345948126879 ) ) ;
#10481=CARTESIAN_POINT ( 'NONE',  ( 2.229367062499998831, -89.64583333196773651, -3.861377020970580887 ) ) ;
#10484=CARTESIAN_POINT ( 'NONE',  ( -4.458734124999999437, 10.60416666803225993, -2.574251347313719407 ) ) ;
#10485=( BOUNDED_CURVE ( )  B_SPLINE_CURVE ( 2, ( #57672, #32260, #62180, #51889, #57045, #22946, #31947, #18419, #41581 ),
 .UNSPECIFIED., .F., .F. ) 
 B_SPLINE_CURVE_WITH_KNOTS ( ( 3, 2, 2, 2, 3 ),
 ( 0.5750000000000005107, 0.5791666666666672736, 0.5833333333333339255, 0.5875000000000004663, 0.5916666666666671182 ),
 .UNSPECIFIED. ) 
 CURVE ( )  GEOMETRIC_REPRESENTATION_ITEM ( )  RATIONAL_B_SPLINE_CURVE ( ( 0.9999999999999898970, 0.9238795325112968415, 1.000000000000000000, 0.9238795325112867385, 1.000000000000000000, 0.9238795325112867385, 1.000000000000000000, 0.9238795325112786339, 1.000000000000008216 ) ) 
 REPRESENTATION_ITEM ( '' )  );
#10487=CARTESIAN_POINT ( 'NONE',  ( -2.229367062499996610, 18.60416666803225993, 3.861377020970582219 ) ) ;
#10489=CARTESIAN_POINT ( 'NONE',  ( -4.999999999999999112, 9.208333336064519870, 2.886751345948131764 ) ) ;
#10490=ORIENTED_EDGE ( 'NONE', *, *, #28417, .T. ) ;
#10491=CARTESIAN_POINT ( 'NONE',  ( 1.975475456537005874E-15, 8.249999999999998224, 5.000000000000000000 ) ) ;
#10494=CARTESIAN_POINT ( 'NONE',  ( 4.458734125000001214, -38.89583333196773651, 2.574251347313718519 ) ) ;
#10495=CARTESIAN_POINT ( 'NONE',  ( -2.499999999999996447, -39.70833333060214443, 4.330127018922195425 ) ) ;
#10497=CARTESIAN_POINT ( 'NONE',  ( -3.152548672688508926E-16, -10.56249999863440792, -5.148502694627439702 ) ) ;
#10498=CARTESIAN_POINT ( 'NONE',  ( 2.229367062500001939, -21.22916666530107221, 3.861377020970579999 ) ) ;
#10500=CARTESIAN_POINT ( 'NONE',  ( -5.000000000000000000, -80.08333333333332860, -2.886751345948128211 ) ) ;
#10501=CARTESIAN_POINT ( 'NONE',  ( -4.458734125000000326, -169.0000000013655779, -1.846868145590735644 ) ) ;
#10503=CARTESIAN_POINT ( 'NONE',  ( -5.000000000000000000, -87.95833333060213022, -2.886751345948128211 ) ) ;
#10504=CARTESIAN_POINT ( 'NONE',  ( 0.000000000000000000, -170.0000000000000000, 5.000000000000000000 ) ) ;
#10507=EDGE_CURVE ( 'NONE', #54676, #18754, #9292, .T. ) ;
#10508=CARTESIAN_POINT ( 'NONE',  ( 2.229367062499998831, -25.89583333196773651, -3.861377020970580887 ) ) ;
#10509=CARTESIAN_POINT ( 'NONE',  ( 5.000000000000000000, -5.291666663935480130, -2.886751345948130876 ) ) ;
#10510=ORIENTED_EDGE ( 'NONE', *, *, #38873, .T. ) ;
#10512=CARTESIAN_POINT ( 'NONE',  ( -3.152801135295367985, -164.0625000013656063, 3.152801135295367096 ) ) ;
#10514=FACE_OUTER_BOUND ( 'NONE', #34226, .T. ) ;
#10515=ORIENTED_EDGE ( 'NONE', *, *, #9347, .F. ) ;
#10517=CARTESIAN_POINT ( 'NONE',  ( 2.229367062499998831, -73.89583333196773651, -3.861377020970580887 ) ) ;
#10520=CARTESIAN_POINT ( 'NONE',  ( 1.846868145590736310, -146.8750000013656063, 4.458734124999997661 ) ) ;
#10521=CARTESIAN_POINT ( 'NONE',  ( -5.000000000000000000, 22.91666666666666430, -2.886751345948128211 ) ) ;
#10526=ADVANCED_FACE ( 'NONE', ( #4169 ), #42441, .T. ) ;
#10527=CARTESIAN_POINT ( 'NONE',  ( -4.458734125000000326, -141.2500000013656063, -1.846868145590735644 ) ) ;
#10531=CARTESIAN_POINT ( 'NONE',  ( 1.975475456537005874E-15, -52.75000000000000000, 5.000000000000000000 ) ) ;
#10533=CARTESIAN_POINT ( 'NONE',  ( 9.457646018065525792E-16, -73.31249999863440792, 5.148502694627439702 ) ) ;
#10535=CYLINDRICAL_SURFACE ( 'NONE', #45959, 5.000000000000000000 ) ;
#10539=ORIENTED_EDGE ( 'NONE', *, *, #27184, .T. ) ;
#10540=CARTESIAN_POINT ( 'NONE',  ( 3.061616997868383141E-16, -145.7500000000000284, -5.000000000000000000 ) ) ;
#10541=CARTESIAN_POINT ( 'NONE',  ( -1.339745962155610925, -14.66965819600733667, 5.000000000000000000 ) ) ;
#10546=CARTESIAN_POINT ( 'NONE',  ( 4.458734125000000326, 17.85416666803225993, 2.574251347313718519 ) ) ;
#10548=EDGE_CURVE ( 'NONE', #59225, #44836, #54306, .T. ) ;
#10554=CARTESIAN_POINT ( 'NONE',  ( 4.458734125000000326, -3.895833331967739177, 2.574251347313718519 ) ) ;
#10555=CARTESIAN_POINT ( 'NONE',  ( 2.229367062500001939, -29.22916666530107221, 3.861377020970579999 ) ) ;
#10559=CARTESIAN_POINT ( 'NONE',  ( 4.458734124999998549, 26.27083333469893134, -2.574251347313721627 ) ) ;
#10560=CARTESIAN_POINT ( 'NONE',  ( 5.000000000000000000, 26.62500000273118772, -6.123233995736766282E-16 ) ) ;
#10561=ADVANCED_FACE ( 'NONE', ( #57264 ), #50562, .T. ) ;
#10563=CARTESIAN_POINT ( 'NONE',  ( -4.458734124999999437, -75.64583333196773651, -2.574251347313719407 ) ) ;
#10566=CARTESIAN_POINT ( 'NONE',  ( -5.000000000000000000, 22.12500000273118417, 0.000000000000000000 ) ) ;
#10569=( BOUNDED_CURVE ( )  B_SPLINE_CURVE ( 2, ( #55480, #6271, #16863, #40985, #56109, #12031, #25878, #35855, #11397 ),
 .UNSPECIFIED., .F., .F. ) 
 B_SPLINE_CURVE_WITH_KNOTS ( ( 3, 2, 2, 2, 3 ),
 ( 0.09791666666666666574, 0.09861111111111110772, 0.1000000000000000056, 0.1013888888888888895, 0.1020833333333333315 ),
 .UNSPECIFIED. ) 
 CURVE ( )  GEOMETRIC_REPRESENTATION_ITEM ( )  RATIONAL_B_SPLINE_CURVE ( ( 0.9330127018922194093, 0.9330127018922194093, 1.000000000000000000, 0.8660254037844387076, 1.000000000000000000, 0.8660254037844387076, 1.000000000000000000, 0.9330127018922194093, 0.9330127018922194093 ) ) 
 REPRESENTATION_ITEM ( '' )  );
#10570=CARTESIAN_POINT ( 'NONE',  ( 1.975475456537005874E-15, -56.62499999726880162, 5.000000000000000000 ) ) ;
#10571=CARTESIAN_POINT ( 'NONE',  ( 2.500000000000002220, -20.66666666666666785, 4.330127018922192761 ) ) ;
#10572=CARTESIAN_POINT ( 'NONE',  ( -3.152548672688508926E-16, -22.56249999863440081, -5.148502694627439702 ) ) ;
#10573=CARTESIAN_POINT ( 'NONE',  ( 2.229367062500001939, -82.97916666530106511, 3.861377020970579999 ) ) ;
#10574=CARTESIAN_POINT ( 'NONE',  ( -5.000000000000000000, -24.95833333060214798, -2.886751345948128211 ) ) ;
#10575=CARTESIAN_POINT ( 'NONE',  ( -4.458734124999998549, -49.22916666530106511, 2.574251347313722516 ) ) ;
#10577=DIRECTION ( 'NONE',  ( -0.000000000000000000, 1.000000000000000000, -0.000000000000000000 ) ) ;
#10578=CARTESIAN_POINT ( 'NONE',  ( -4.458734124999999437, 2.354166668032262599, -2.574251347313719407 ) ) ;
#10581=CARTESIAN_POINT ( 'NONE',  ( -3.535250795749689387E-16, -66.25000000000000000, -5.773502691896257311 ) ) ;
#10582=CARTESIAN_POINT ( 'NONE',  ( -4.458734125000000326, -153.2500000013655779, -1.846868145590735644 ) ) ;
#10584=CARTESIAN_POINT ( 'NONE',  ( 1.062108568985190270E-13, -27.25000000000000000, -4.999999999999999112 ) ) ;
#10585=CARTESIAN_POINT ( 'NONE',  ( -9.184850993605147944E-16, -159.2500000000000000, 5.000000000000000000 ) ) ;
#10586=CARTESIAN_POINT ( 'NONE',  ( 1.975475456537005874E-15, 7.375000002731186832, 5.000000000000000000 ) ) ;
#10589=CARTESIAN_POINT ( 'NONE',  ( 9.457646018065525792E-16, -9.312499998634406140, 5.148502694627439702 ) ) ;
#10590=CARTESIAN_POINT ( 'NONE',  ( 4.458734124999999437, -47.06249999863440792, -5.460374474430324690E-16 ) ) ;
#10592=CARTESIAN_POINT ( 'NONE',  ( -3.152801135295367985, -145.8125000013655779, 3.152801135295367096 ) ) ;
#10595=ORIENTED_EDGE ( 'NONE', *, *, #3493, .F. ) ;
#10597=CARTESIAN_POINT ( 'NONE',  ( -4.458734124999999437, 28.35416666803226349, -2.574251347313719407 ) ) ;
#10599=CARTESIAN_POINT ( 'NONE',  ( 1.339745962155615144, -29.58034179853029499, 4.999999999999999112 ) ) ;
#10600=ORIENTED_EDGE ( 'NONE', *, *, #51497, .T. ) ;
#10607=CARTESIAN_POINT ( 'NONE',  ( 4.458734124999998549, -9.729166665301068662, -2.574251347313721627 ) ) ;
#10609=CARTESIAN_POINT ( 'NONE',  ( -4.458734124999999437, -90.43749999863440792, 0.000000000000000000 ) ) ;
#10610=CARTESIAN_POINT ( 'NONE',  ( 4.458734124999999437, -147.3750000013656063, -1.846868145590734978 ) ) ;
#10612=ORIENTED_EDGE ( 'NONE', *, *, #33487, .F. ) ;
#10617=CARTESIAN_POINT ( 'NONE',  ( 5.000000000000000000, -85.37499999726880162, -6.123233995736766282E-16 ) ) ;
#10623=CARTESIAN_POINT ( 'NONE',  ( -4.999999999999998224, -89.79166666393547303, 2.886751345948131764 ) ) ;
#10625=CARTESIAN_POINT ( 'NONE',  ( 4.458734124999998549, 12.27083333469892423, -2.574251347313721627 ) ) ;
#10628=CARTESIAN_POINT ( 'NONE',  ( 2.229367062500001939, -14.22916666530107221, 3.861377020970579999 ) ) ;
#10630=CARTESIAN_POINT ( 'NONE',  ( 4.458734125000000326, -163.3750000013656347, -1.846868145590734978 ) ) ;
#10634=EDGE_CURVE ( 'NONE', #50889, #46232, #13176, .T. ) ;
#10637=CARTESIAN_POINT ( 'NONE',  ( -6.972266317189433020E-16, -55.12499999726880873, -5.000000000000000000 ) ) ;
#10639=CYLINDRICAL_SURFACE ( 'NONE', #50267, 5.000000000000000000 ) ;
#10640=CARTESIAN_POINT ( 'NONE',  ( -4.458734124999999437, -154.1875000013656063, -5.460374474430324690E-16 ) ) ;
#10643=CARTESIAN_POINT ( 'NONE',  ( -6.972266317189433020E-16, -68.12499999726881583, -5.000000000000000000 ) ) ;
#10647=FACE_OUTER_BOUND ( 'NONE', #61401, .T. ) ;
#10648=CARTESIAN_POINT ( 'NONE',  ( -5.000000000000000000, -4.083333333333334814, -2.886751345948128211 ) ) ;
#10649=CARTESIAN_POINT ( 'NONE',  ( -4.458734124999999437, -65.39583333196773651, -2.574251347313719407 ) ) ;
#10652=CARTESIAN_POINT ( 'NONE',  ( -5.000000000000000000, -6.874999997268812280, 0.000000000000000000 ) ) ;
#10653=CARTESIAN_POINT ( 'NONE',  ( -3.152548672688508926E-16, -32.56249999863440792, -5.148502694627439702 ) ) ;
#10657=VERTEX_POINT ( 'NONE', #22718 ) ;
#10659=CARTESIAN_POINT ( 'NONE',  ( -2.500000000000000444, -51.16666666666666430, -4.330127018922193649 ) ) ;
#10660=CARTESIAN_POINT ( 'NONE',  ( 1.339745962155612702, -46.16965819600732601, -5.000000000000000000 ) ) ;
#10662=CARTESIAN_POINT ( 'NONE',  ( 5.000000000000000000, -32.37499999726880873, -6.123233995736766282E-16 ) ) ;
#10663=CARTESIAN_POINT ( 'NONE',  ( -2.229367062500000163, -74.47916666530106511, -3.861377020970580443 ) ) ;
#10664=CARTESIAN_POINT ( 'NONE',  ( 1.846868145590736310, -145.8750000013656063, 4.458734124999999437 ) ) ;
#10665=CARTESIAN_POINT ( 'NONE',  ( -4.458734124999999437, -84.31249999863439371, 0.000000000000000000 ) ) ;
#10667=CARTESIAN_POINT ( 'NONE',  ( -4.458734124999999437, -29.64583333196773651, -2.574251347313719407 ) ) ;
#10672=DIRECTION ( 'NONE',  ( -0.000000000000000000, 1.000000000000000000, -0.000000000000000000 ) ) ;
#10673=ORIENTED_EDGE ( 'NONE', *, *, #49606, .T. ) ;
#10675=CARTESIAN_POINT ( 'NONE',  ( 1.339745962155615144, -21.70534180126147916, 4.999999999999999112 ) ) ;
#10676=EDGE_CURVE ( 'NONE', #17081, #48474, #21444, .T. ) ;
#10681=CARTESIAN_POINT ( 'NONE',  ( 4.458734125000001214, -62.14583333196774362, 2.574251347313718519 ) ) ;
#10684=ORIENTED_EDGE ( 'NONE', *, *, #893, .T. ) ;
#10690=CARTESIAN_POINT ( 'NONE',  ( -3.152548672688508926E-16, 12.43750000136559564, -5.148502694627439702 ) ) ;
#10693=CARTESIAN_POINT ( 'NONE',  ( 3.152801135295366208, -161.5625000013656063, 3.152801135295367985 ) ) ;
#10702=VECTOR ( 'NONE', #21226, 1000.000000000000000 ) ;
#10703=CARTESIAN_POINT ( 'NONE',  ( 2.500000000000002220, -36.66666666666666430, 4.330127018922192761 ) ) ;
#10706=CARTESIAN_POINT ( 'NONE',  ( -2.500000000000000444, -73.04166666393548724, -4.330127018922193649 ) ) ;
#10707=CARTESIAN_POINT ( 'NONE',  ( 2.499999999999998668, -78.20833333060214443, -4.330127018922193649 ) ) ;
#10712=CARTESIAN_POINT ( 'NONE',  ( -4.458734124999999437, 0.4375000013655955255, 0.000000000000000000 ) ) ;
#10713=CARTESIAN_POINT ( 'NONE',  ( -5.000000000000000000, -161.6250000027311842, -6.123233995736766282E-16 ) ) ;
#10715=CARTESIAN_POINT ( 'NONE',  ( -2.071067811865478170, -147.4375000027312410, 5.000000000000000000 ) ) ;
#10723=CARTESIAN_POINT ( 'NONE',  ( -4.458734124999999437, -164.2500000013656063, -1.846868145590735644 ) ) ;
#10725=CARTESIAN_POINT ( 'NONE',  ( -2.071067811865580754, -159.8125000027311842, -4.999999999999894307 ) ) ;
#10727=CARTESIAN_POINT ( 'NONE',  ( -4.458734125000001214, -144.8750000013655779, 1.846868145590734089 ) ) ;
#10729=CARTESIAN_POINT ( 'NONE',  ( 9.457646018065525792E-16, 21.68750000136559208, 5.148502694627439702 ) ) ;
#10731=CARTESIAN_POINT ( 'NONE',  ( -4.458734124999999437, -64.56249999863440792, 0.000000000000000000 ) ) ;
#10734=DIRECTION ( 'NONE',  ( 0.000000000000000000, 0.000000000000000000, 1.000000000000000000 ) ) ;
#10735=CARTESIAN_POINT ( 'NONE',  ( 5.000000000000000000, 12.50000000000000000, -6.123233995736766282E-16 ) ) ;
#10736=CARTESIAN_POINT ( 'NONE',  ( -4.458734124999997661, -51.22916666530107932, 2.574251347313722516 ) ) ;
#10737=CARTESIAN_POINT ( 'NONE',  ( -3.152548672688508926E-16, -9.562499998634406140, -5.148502694627439702 ) ) ;
#10738=CARTESIAN_POINT ( 'NONE',  ( 3.535533905932738197, -166.0000000027312126, -3.535533905932738197 ) ) ;
#10743=CARTESIAN_POINT ( 'NONE',  ( 6.123233995736766282E-16, -170.0000000000000000, -5.000000000000000000 ) ) ;
#10746=CARTESIAN_POINT ( 'NONE',  ( 4.458734125000001214, -58.89583333196773651, 2.574251347313718519 ) ) ;
#10747=CARTESIAN_POINT ( 'NONE',  ( 1.846868145590735200, -156.5000000013656347, -4.458734125000000326 ) ) ;
#10748=AXIS2_PLACEMENT_3D ( 'NONE', #23572, #28067, #32258 ) ;
#10749=CARTESIAN_POINT ( 'NONE',  ( -5.000000000000000000, -56.95833333060214443, -2.886751345948128211 ) ) ;
#10750=ORIENTED_EDGE ( 'NONE', *, *, #24396, .T. ) ;
#10752=CARTESIAN_POINT ( 'NONE',  ( 4.458734124999998549, 2.020833334698927786, -2.574251347313721627 ) ) ;
#10754=( BOUNDED_CURVE ( )  B_SPLINE_CURVE ( 2, ( #37870, #36922, #62643, #18562, #13106, #12472, #42998, #42366, #38185 ),
 .UNSPECIFIED., .F., .F. ) 
 B_SPLINE_CURVE_WITH_KNOTS ( ( 3, 2, 2, 2, 3 ),
 ( 0.2354166666666666630, 0.2361111111111111049, 0.2374999999999999889, 0.2388888888888889006, 0.2395833333333333426 ),
 .UNSPECIFIED. ) 
 CURVE ( )  GEOMETRIC_REPRESENTATION_ITEM ( )  RATIONAL_B_SPLINE_CURVE ( ( 0.9330127018922194093, 0.9330127018922194093, 1.000000000000000000, 0.8660254037844387076, 1.000000000000000000, 0.8660254037844387076, 1.000000000000000000, 0.9330127018922194093, 0.9330127018922194093 ) ) 
 REPRESENTATION_ITEM ( '' )  );
#10755=FACE_OUTER_BOUND ( 'NONE', #1056, .T. ) ;
#10757=CARTESIAN_POINT ( 'NONE',  ( 4.458734124999999437, -156.4375000013655779, 0.000000000000000000 ) ) ;
#10758=ORIENTED_EDGE ( 'NONE', *, *, #63339, .F. ) ;
#10760=CARTESIAN_POINT ( 'NONE',  ( -4.458734124999999437, -90.31249999863440792, 0.000000000000000000 ) ) ;
#10761=CARTESIAN_POINT ( 'NONE',  ( -4.458734124999999437, -43.56249999863440081, 0.000000000000000000 ) ) ;
#10763=CARTESIAN_POINT ( 'NONE',  ( -1.339745962155613812, -46.20534180126146850, -5.000000000000000000 ) ) ;
#10765=EDGE_CURVE ( 'NONE', #17081, #60982, #56311, .T. ) ;
#10766=CARTESIAN_POINT ( 'NONE',  ( -2.229367062500000163, 29.52083333469892779, -3.861377020970580443 ) ) ;
#10770=( BOUNDED_CURVE ( )  B_SPLINE_CURVE ( 2, ( #22530, #56939, #42126, #17696, #37310 ),
 .UNSPECIFIED., .F., .F. ) 
 B_SPLINE_CURVE_WITH_KNOTS ( ( 3, 2, 3 ),
 ( 0.000000000000000000, 0.001388888888888888942, 0.002083333333333333738 ),
 .UNSPECIFIED. ) 
 CURVE ( )  GEOMETRIC_REPRESENTATION_ITEM ( )  RATIONAL_B_SPLINE_CURVE ( ( 1.000000000000000000, 0.8660254037844387076, 1.000000000000000000, 0.9330127018922192983, 0.9330127018922194093 ) ) 
 REPRESENTATION_ITEM ( '' )  );
#10771=CARTESIAN_POINT ( 'NONE',  ( 6.123233995736766282E-16, -170.0000000000000000, -5.000000000000000000 ) ) ;
#10775=DIRECTION ( 'NONE',  ( -0.000000000000000000, 1.000000000000000000, -0.000000000000000000 ) ) ;
#10776=ADVANCED_FACE ( 'NONE', ( #165 ), #44841, .T. ) ;
#10777=CARTESIAN_POINT ( 'NONE',  ( -2.071067811865602071, -157.6874999999999716, -4.999999999999874767 ) ) ;
#10780=CARTESIAN_POINT ( 'NONE',  ( 1.339745962155615144, -42.58034179853029144, 4.999999999999999112 ) ) ;
#10782=CARTESIAN_POINT ( 'NONE',  ( 2.229367062499998831, -89.89583333196773651, -3.861377020970580887 ) ) ;
#10788=CARTESIAN_POINT ( 'NONE',  ( -5.000000000000000888, -156.6875000027312126, -2.071067811865475949 ) ) ;
#10789=ORIENTED_EDGE ( 'NONE', *, *, #51676, .F. ) ;
#10797=CARTESIAN_POINT ( 'NONE',  ( 5.000000000000000888, -48.45833333060215153, 2.886751345948126879 ) ) ;
#10798=CARTESIAN_POINT ( 'NONE',  ( 2.229367062500001939, -18.97916666530106866, 3.861377020970579999 ) ) ;
#10799=CARTESIAN_POINT ( 'NONE',  ( -6.972266317189433020E-16, -75.25000000000000000, -5.000000000000000000 ) ) ;
#10800=CARTESIAN_POINT ( 'NONE',  ( 5.000000000000000000, -150.0625000000000000, 2.071067811865478614 ) ) ;
#10802=CARTESIAN_POINT ( 'NONE',  ( 1.846868145590735200, -154.2500000013656063, -4.458734125000000326 ) ) ;
#10803=ORIENTED_EDGE ( 'NONE', *, *, #23930, .T. ) ;
#10804=CARTESIAN_POINT ( 'NONE',  ( 4.458734124999998549, -45.97916666530106511, -2.574251347313721627 ) ) ;
#10805=CARTESIAN_POINT ( 'NONE',  ( 0.000000000000000000, -170.0000000000000000, 0.000000000000000000 ) ) ;
#10806=FACE_OUTER_BOUND ( 'NONE', #8324, .T. ) ;
#10807=CARTESIAN_POINT ( 'NONE',  ( 5.000000000000000000, 28.49999999999999645, -6.123233995736766282E-16 ) ) ;
#10808=CARTESIAN_POINT ( 'NONE',  ( -2.229367062499996610, 2.854166668032259935, 3.861377020970582219 ) ) ;
#10809=CARTESIAN_POINT ( 'NONE',  ( -4.999999999999998224, -43.91666666666665719, 2.886751345948131764 ) ) ;
#10810=CARTESIAN_POINT ( 'NONE',  ( 0.000000000000000000, -170.0000000000000000, 5.000000000000000000 ) ) ;
#10811=CARTESIAN_POINT ( 'NONE',  ( 5.000000000000000000, -17.41666666666666430, -2.886751345948130876 ) ) ;
#10812=CARTESIAN_POINT ( 'NONE',  ( -4.458734124999999437, 22.35416666803225638, -2.574251347313719407 ) ) ;
#10814=CARTESIAN_POINT ( 'NONE',  ( -2.500000000000000444, 5.958333336064519870, -4.330127018922193649 ) ) ;
#10815=ORIENTED_EDGE ( 'NONE', *, *, #62275, .T. ) ;
#10817=EDGE_LOOP ( 'NONE', ( #59567, #39206, #60006, #51564 ) ) ;
#10819=CARTESIAN_POINT ( 'NONE',  ( -4.458734124999998549, -37.22916666530107221, 2.574251347313722516 ) ) ;
#10821=CARTESIAN_POINT ( 'NONE',  ( 5.000000000000000888, -41.45833333060213732, 2.886751345948126879 ) ) ;
#10823=CARTESIAN_POINT ( 'NONE',  ( -4.458734124999998549, -13.22916666530107221, 2.574251347313722516 ) ) ;
#10825=CARTESIAN_POINT ( 'NONE',  ( -4.999999999999999112, -84.91666666666667140, 2.886751345948131764 ) ) ;
#10826=CARTESIAN_POINT ( 'NONE',  ( -1.846868145590737420, -168.7500000013656063, 4.458734124999999437 ) ) ;
#10827=CARTESIAN_POINT ( 'NONE',  ( 2.499999999999998668, -89.20833333060214443, -4.330127018922193649 ) ) ;
#10828=CARTESIAN_POINT ( 'NONE',  ( -5.000000000000000000, -32.00000000000000000, 0.000000000000000000 ) ) ;
#10829=ORIENTED_EDGE ( 'NONE', *, *, #29564, .T. ) ;
#10831=CARTESIAN_POINT ( 'NONE',  ( -4.458734124999999437, -26.56249999863440792, 0.000000000000000000 ) ) ;
#10834=VECTOR ( 'NONE', #32218, 1000.000000000000000 ) ;
#10835=CARTESIAN_POINT ( 'NONE',  ( -3.152801135295367096, -162.3125000013656063, -3.152801135295367541 ) ) ;
#10837=ORIENTED_EDGE ( 'NONE', *, *, #50029, .T. ) ;
#10839=CARTESIAN_POINT ( 'NONE',  ( -4.458734124999999437, -72.64583333196773651, -2.574251347313719407 ) ) ;
#10842=CARTESIAN_POINT ( 'NONE',  ( -1.846868145590737420, -142.0000000013655495, 4.458734124999997661 ) ) ;
#10847=( BOUNDED_CURVE ( )  B_SPLINE_CURVE ( 2, ( #59235, #29633, #5521, #29953, #10022, #14838, #33837, #38967, #38652 ),
 .UNSPECIFIED., .F., .F. ) 
 B_SPLINE_CURVE_WITH_KNOTS ( ( 3, 2, 2, 2, 3 ),
 ( 0.6395833333333332815, 0.6402777777777777235, 0.6416666666666667185, 0.6430555555555556024, 0.6437500000000000444 ),
 .UNSPECIFIED. ) 
 CURVE ( )  GEOMETRIC_REPRESENTATION_ITEM ( )  RATIONAL_B_SPLINE_CURVE ( ( 0.9330127018922194093, 0.9330127018922194093, 1.000000000000000000, 0.8660254037844387076, 1.000000000000000000, 0.8660254037844387076, 1.000000000000000000, 0.9330127018922194093, 0.9330127018922194093 ) ) 
 REPRESENTATION_ITEM ( '' )  );
#10849=CARTESIAN_POINT ( 'NONE',  ( -3.535533905932738641, -167.3750000000000284, 3.535533905932737309 ) ) ;
#10852=CYLINDRICAL_SURFACE ( 'NONE', #25298, 5.000000000000000000 ) ;
#10854=CARTESIAN_POINT ( 'NONE',  ( 4.458734124999998549, -74.97916666530106511, -2.574251347313721627 ) ) ;
#10855=CARTESIAN_POINT ( 'NONE',  ( -9.184850993605147944E-16, -166.2500000000000000, 5.000000000000000000 ) ) ;
#10856=CARTESIAN_POINT ( 'NONE',  ( -3.535533905932737309, -139.7500000027311842, -3.535533905932738197 ) ) ;
#10857=CARTESIAN_POINT ( 'NONE',  ( 5.000000000000000888, -68.58333333333332860, 2.886751345948126879 ) ) ;
#10859=ORIENTED_EDGE ( 'NONE', *, *, #30730, .T. ) ;
#10861=CARTESIAN_POINT ( 'NONE',  ( 1.339745962155615144, -15.70534180126148271, 4.999999999999999112 ) ) ;
#10866=CARTESIAN_POINT ( 'NONE',  ( 4.458734124999999437, 17.93750000136559208, -5.460374474430324690E-16 ) ) ;
#10873=CARTESIAN_POINT ( 'NONE',  ( 0.000000000000000000, -170.0000000000000000, 5.000000000000000000 ) ) ;
#10874=CARTESIAN_POINT ( 'NONE',  ( -3.152548672688508926E-16, -84.56249999863439371, -5.148502694627439702 ) ) ;
#10875=CARTESIAN_POINT ( 'NONE',  ( -3.152548672688508926E-16, -3.562499998634408360, -5.148502694627439702 ) ) ;
#10877=EDGE_LOOP ( 'NONE', ( #9449, #11141, #62579, #56399, #8926, #52924 ) ) ;
#10878=CARTESIAN_POINT ( 'NONE',  ( -3.152548672688508926E-16, -29.81249999863440436, -5.148502694627439702 ) ) ;
#10883=CARTESIAN_POINT ( 'NONE',  ( -2.229367062500000163, 24.52083333469892779, -3.861377020970580443 ) ) ;
#10885=CARTESIAN_POINT ( 'NONE',  ( -5.000000000000000888, -145.6875000027312126, -2.071067811865475949 ) ) ;
#10886=CARTESIAN_POINT ( 'NONE',  ( 2.229367062499998831, -78.89583333196773651, -3.861377020970580887 ) ) ;
#10889=CARTESIAN_POINT ( 'NONE',  ( -2.499999999999996447, 23.29166666939785202, 4.330127018922195425 ) ) ;
#10890=ORIENTED_EDGE ( 'NONE', *, *, #11000, .T. ) ;
#10893=CARTESIAN_POINT ( 'NONE',  ( 1.975475456537005874E-15, -57.74999999999999289, 5.000000000000000000 ) ) ;
#10894=CARTESIAN_POINT ( 'NONE',  ( 5.000000000000000000, -16.41666666666667140, -2.886751345948129988 ) ) ;
#10895=CARTESIAN_POINT ( 'NONE',  ( -4.458734124999999437, -20.39583333196774362, -2.574251347313719407 ) ) ;
#10896=CARTESIAN_POINT ( 'NONE',  ( 2.229367062499998831, -84.64583333196773651, -3.861377020970580887 ) ) ;
#10897=CARTESIAN_POINT ( 'NONE',  ( -4.999999999999999112, -24.79166666393548368, 2.886751345948131764 ) ) ;
#10898=CARTESIAN_POINT ( 'NONE',  ( 4.458734124999998549, -54.72916666530107932, -2.574251347313721627 ) ) ;
#10899=ORIENTED_EDGE ( 'NONE', *, *, #52386, .T. ) ;
#10902=CARTESIAN_POINT ( 'NONE',  ( -4.458734124999999437, -5.645833331967740953, -2.574251347313719407 ) ) ;
#10905=CARTESIAN_POINT ( 'NONE',  ( 1.060575238724906964E-15, -63.75000000000000000, 5.773502691896257311 ) ) ;
#10906=CARTESIAN_POINT ( 'NONE',  ( -4.458734125000000326, -154.2500000013656063, -1.846868145590735644 ) ) ;
#10908=CARTESIAN_POINT ( 'NONE',  ( -6.972266317189433020E-16, -81.12499999726881583, -5.000000000000000000 ) ) ;
#10909=CARTESIAN_POINT ( 'NONE',  ( 3.535533905932738197, -159.8750000000000284, -3.535533905932738197 ) ) ;
#10912=CARTESIAN_POINT ( 'NONE',  ( 9.457646018065525792E-16, -13.31249999863440259, 5.148502694627439702 ) ) ;
#10913=CARTESIAN_POINT ( 'NONE',  ( -2.229367062500000163, -50.72916666530107221, -3.861377020970580443 ) ) ;
#10915=CARTESIAN_POINT ( 'NONE',  ( 1.846868145590736310, -145.6250000013655779, 4.458734124999999437 ) ) ;
#10919=CARTESIAN_POINT ( 'NONE',  ( 4.458734124999999437, 27.93750000136559208, -5.460374474430324690E-16 ) ) ;
#10923=ORIENTED_EDGE ( 'NONE', *, *, #43376, .T. ) ;
#10926=CARTESIAN_POINT ( 'NONE',  ( -6.972266317189433020E-16, 7.875000002731185056, -5.000000000000000000 ) ) ;
#10928=CARTESIAN_POINT ( 'NONE',  ( -5.000000000000000000, 2.125000002731185056, 0.000000000000000000 ) ) ;
#10929=CARTESIAN_POINT ( 'NONE',  ( 2.229367062500001939, -6.979166665301073103, 3.861377020970579999 ) ) ;
#10931=CARTESIAN_POINT ( 'NONE',  ( 3.152801135295367541, -147.3125000013655779, -3.152801135295367541 ) ) ;
#10933=VERTEX_POINT ( 'NONE', #54175 ) ;
#10936=CARTESIAN_POINT ( 'NONE',  ( 1.339745962155615144, 1.419658201469705672, 4.999999999999999112 ) ) ;
#10940=CARTESIAN_POINT ( 'NONE',  ( 0.000000000000000000, 30.00000000000000000, 0.000000000000000000 ) ) ;
#10942=CARTESIAN_POINT ( 'NONE',  ( 4.458734124999998549, 10.27083333469892779, -2.574251347313721627 ) ) ;
#10944=VERTEX_POINT ( 'NONE', #10114 ) ;
#10945=CARTESIAN_POINT ( 'NONE',  ( -4.458734124999999437, -15.56249999863440436, 0.000000000000000000 ) ) ;
#10948=CARTESIAN_POINT ( 'NONE',  ( -4.458734125000001214, -163.8750000013655779, 1.846868145590734089 ) ) ;
#10954=DIRECTION ( 'NONE',  ( -0.000000000000000000, 1.000000000000000000, -0.000000000000000000 ) ) ;
#10955=CARTESIAN_POINT ( 'NONE',  ( -6.972266317189433020E-16, -38.25000000000000000, -5.000000000000000000 ) ) ;
#10958=CARTESIAN_POINT ( 'NONE',  ( 3.152801135295367541, -151.5625000013655779, -3.152801135295367541 ) ) ;
#10960=CARTESIAN_POINT ( 'NONE',  ( -2.500000000000000444, -58.04166666393548013, -4.330127018922193649 ) ) ;
#10967=CARTESIAN_POINT ( 'NONE',  ( 2.499999999999998668, -0.3333333333333348136, -4.330127018922193649 ) ) ;
#10970=CARTESIAN_POINT ( 'NONE',  ( -4.458734124999999437, -66.31249999863440792, 0.000000000000000000 ) ) ;
#10971=CARTESIAN_POINT ( 'NONE',  ( -3.535250795749689387E-16, -9.124999997268815832, -5.773502691896257311 ) ) ;
#10972=CARTESIAN_POINT ( 'NONE',  ( -2.229367062500000163, -32.47916666530106511, -3.861377020970580443 ) ) ;
#10973=VERTEX_POINT ( 'NONE', #6262 ) ;
#10974=CARTESIAN_POINT ( 'NONE',  ( -2.500000000000000444, -78.16666666666665719, -4.330127018922193649 ) ) ;
#10977=CARTESIAN_POINT ( 'NONE',  ( 4.458734125000001214, 13.85416666803226171, 2.574251347313718519 ) ) ;
#10980=CARTESIAN_POINT ( 'NONE',  ( 1.060575238724906964E-15, -51.75000000000000711, 5.773502691896257311 ) ) ;
#10982=CARTESIAN_POINT ( 'NONE',  ( -1.339745962155613812, 13.91965820146970678, -5.000000000000000000 ) ) ;
#10983=CARTESIAN_POINT ( 'NONE',  ( 4.458734124999999437, -74.81249999863440792, -5.460374474430324690E-16 ) ) ;
#10984=CARTESIAN_POINT ( 'NONE',  ( 4.458734124999999437, -141.7500000013655779, 1.846868145590737864 ) ) ;
#10985=CARTESIAN_POINT ( 'NONE',  ( -2.229367062500000163, -81.47916666530106511, -3.861377020970580443 ) ) ;
#10987=CARTESIAN_POINT ( 'NONE',  ( -4.458734124999998549, -31.47916666530107221, 2.574251347313722516 ) ) ;
#10990=ORIENTED_EDGE ( 'NONE', *, *, #16578, .T. ) ;
#10995=CARTESIAN_POINT ( 'NONE',  ( 5.000000000000000888, -12.58333333333333570, 2.886751345948126879 ) ) ;
#10996=CARTESIAN_POINT ( 'NONE',  ( 4.458734125000001214, -63.14583333196774362, 2.574251347313718519 ) ) ;
#11000=EDGE_CURVE ( 'NONE', #15736, #24591, #55145, .T. ) ;
#11002=CARTESIAN_POINT ( 'NONE',  ( -3.152548672688508926E-16, 6.437500001365592972, -5.148502694627439702 ) ) ;
#11004=CARTESIAN_POINT ( 'NONE',  ( -1.339745962155610925, -0.7946581987385198387, 5.000000000000000000 ) ) ;
#11005=CARTESIAN_POINT ( 'NONE',  ( -3.152801135295367985, -159.8125000013656063, 3.152801135295367096 ) ) ;
#11007=EDGE_LOOP ( 'NONE', ( #31175, #49595, #53543, #9615 ) ) ;
#11012=DIRECTION ( 'NONE',  ( 0.000000000000000000, 0.000000000000000000, 1.000000000000000000 ) ) ;
#11020=CARTESIAN_POINT ( 'NONE',  ( 5.000000000000000000, -82.29166666393547303, -2.886751345948130876 ) ) ;
#11023=CARTESIAN_POINT ( 'NONE',  ( -4.458734124999999437, 4.354166668032260823, -2.574251347313719407 ) ) ;
#11024=CARTESIAN_POINT ( 'NONE',  ( 2.071067811865560326, -145.9375000027311842, -4.999999999999914735 ) ) ;
#11026=CARTESIAN_POINT ( 'NONE',  ( -5.000000000000000000, -145.6250000027312126, -6.123233995736766282E-16 ) ) ;
#11030=CARTESIAN_POINT ( 'NONE',  ( -6.972266317189433020E-16, 5.749999999999999112, -5.000000000000000000 ) ) ;
#11035=CARTESIAN_POINT ( 'NONE',  ( -1.846868145590734756, -162.3750000013656063, -4.458734124999999437 ) ) ;
#11036=DIRECTION ( 'NONE',  ( -0.000000000000000000, 1.000000000000000000, -0.000000000000000000 ) ) ;
#11039=CARTESIAN_POINT ( 'NONE',  ( -1.846868145590737420, -140.7500000013655779, 4.458734124999999437 ) ) ;
#11041=CARTESIAN_POINT ( 'NONE',  ( -3.152548672688508926E-16, 25.18750000136558853, -5.148502694627439702 ) ) ;
#11042=ORIENTED_EDGE ( 'NONE', *, *, #37761, .T. ) ;
#11043=CARTESIAN_POINT ( 'NONE',  ( 2.229367062499998831, -62.89583333196774362, -3.861377020970580887 ) ) ;
#11045=CARTESIAN_POINT ( 'NONE',  ( -1.339745962155610925, -2.669658196007334450, 5.000000000000000000 ) ) ;
#11046=CARTESIAN_POINT ( 'NONE',  ( 2.499999999999998668, 15.66666666666666607, -4.330127018922193649 ) ) ;
#11048=CARTESIAN_POINT ( 'NONE',  ( -4.458734124999997661, -49.22916666530106511, 2.574251347313722516 ) ) ;
#11049=CARTESIAN_POINT ( 'NONE',  ( 9.457646018065525792E-16, -9.062499998634406140, 5.148502694627439702 ) ) ;
#11050=( BOUNDED_CURVE ( )  B_SPLINE_CURVE ( 2, ( #17828, #13000, #60960, #52246, #18139, #3365, #8187, #57398, #26858 ),
 .UNSPECIFIED., .F., .F. ) 
 B_SPLINE_CURVE_WITH_KNOTS ( ( 3, 2, 2, 2, 3 ),
 ( 0.2104166666666666685, 0.2111111111111111105, 0.2124999999999999944, 0.2138888888888888784, 0.2145833333333333481 ),
 .UNSPECIFIED. ) 
 CURVE ( )  GEOMETRIC_REPRESENTATION_ITEM ( )  RATIONAL_B_SPLINE_CURVE ( ( 0.9330127018922194093, 0.9330127018922194093, 1.000000000000000000, 0.8660254037844387076, 1.000000000000000000, 0.8660254037844387076, 1.000000000000000000, 0.9330127018922180770, 0.9330127018922194093 ) ) 
 REPRESENTATION_ITEM ( '' )  );
#11053=CARTESIAN_POINT ( 'NONE',  ( -6.972266317189433020E-16, -37.25000000000000000, -5.000000000000000000 ) ) ;
#11057=CARTESIAN_POINT ( 'NONE',  ( -5.000000000000000000, -34.00000000000000000, 0.000000000000000000 ) ) ;
#11060=CARTESIAN_POINT ( 'NONE',  ( -1.339745962155613812, -32.08034179853029855, -5.000000000000000000 ) ) ;
#11061=CARTESIAN_POINT ( 'NONE',  ( -4.458734124999999437, -59.31249999863440081, 0.000000000000000000 ) ) ;
#11062=CARTESIAN_POINT ( 'NONE',  ( 1.846868145590735200, -152.5000000013656347, -4.458734125000000326 ) ) ;
#11063=CARTESIAN_POINT ( 'NONE',  ( -4.458734124999999437, -68.39583333196773651, -2.574251347313719407 ) ) ;
#11065=CARTESIAN_POINT ( 'NONE',  ( -5.000000000000000000, -53.87499999726880162, 0.000000000000000000 ) ) ;
#11068=CARTESIAN_POINT ( 'NONE',  ( 2.229367062499998831, 0.1041666680322607397, -3.861377020970580887 ) ) ;
#11071=CARTESIAN_POINT ( 'NONE',  ( 0.000000000000000000, -170.0000000000000000, 5.000000000000000000 ) ) ;
#11072=CARTESIAN_POINT ( 'NONE',  ( 4.458734124999999437, -155.5000000013655779, 1.846868145590737864 ) ) ;
#11073=ORIENTED_EDGE ( 'NONE', *, *, #36719, .T. ) ;
#11074=DIRECTION ( 'NONE',  ( 0.000000000000000000, 0.000000000000000000, 1.000000000000000000 ) ) ;
#11077=CARTESIAN_POINT ( 'NONE',  ( 2.229367062499998831, -48.89583333196772941, -3.861377020970580887 ) ) ;
#11078=VERTEX_POINT ( 'NONE', #10955 ) ;
#11081=CARTESIAN_POINT ( 'NONE',  ( 2.229367062499998831, 23.35416666803225993, -3.861377020970580887 ) ) ;
#11086=CARTESIAN_POINT ( 'NONE',  ( -5.000000000000000000, 1.000000000000000888, 0.000000000000000000 ) ) ;
#11088=CARTESIAN_POINT ( 'NONE',  ( -5.000000000000000000, -78.87499999726881583, 0.000000000000000000 ) ) ;
#11089=CARTESIAN_POINT ( 'NONE',  ( -5.000000000000000000, -1.958333330602145983, -2.886751345948128211 ) ) ;
#11094=CARTESIAN_POINT ( 'NONE',  ( -4.458734124999999437, -90.56249999863440792, 0.000000000000000000 ) ) ;
#11095=CARTESIAN_POINT ( 'NONE',  ( 1.975475456537005874E-15, 8.375000002731187720, 5.000000000000000000 ) ) ;
#11097=( BOUNDED_CURVE ( )  B_SPLINE_CURVE ( 2, ( #27413, #12624, #36436, #16502, #56066, #22287, #31929, #51557, #36124 ),
 .UNSPECIFIED., .F., .F. ) 
 B_SPLINE_CURVE_WITH_KNOTS ( ( 3, 2, 2, 2, 3 ),
 ( 0.4354166666666666741, 0.4361111111111111160, 0.4375000000000000000, 0.4388888888888888840, 0.4395833333333333259 ),
 .UNSPECIFIED. ) 
 CURVE ( )  GEOMETRIC_REPRESENTATION_ITEM ( )  RATIONAL_B_SPLINE_CURVE ( ( 0.9330127018922194093, 0.9330127018922194093, 1.000000000000000000, 0.8660254037844387076, 1.000000000000000000, 0.8660254037844387076, 1.000000000000000000, 0.9330127018922194093, 0.9330127018922194093 ) ) 
 REPRESENTATION_ITEM ( '' )  );
#11098=ORIENTED_EDGE ( 'NONE', *, *, #34361, .T. ) ;
#11101=CARTESIAN_POINT ( 'NONE',  ( -3.535533905932738641, -158.5000000027312126, 3.535533905932737309 ) ) ;
#11102=VERTEX_POINT ( 'NONE', #15151 ) ;
#11108=EDGE_CURVE ( 'NONE', #15348, #20078, #57154, .T. ) ;
#11112=CARTESIAN_POINT ( 'NONE',  ( 4.458734124999998549, -20.72916666530107221, -2.574251347313721627 ) ) ;
#11113=CARTESIAN_POINT ( 'NONE',  ( -2.071067811865478170, -149.3125000000000000, 5.000000000000000000 ) ) ;
#11115=CARTESIAN_POINT ( 'NONE',  ( 1.846868145590736310, -152.6250000013655495, 4.458734124999999437 ) ) ;
#11116=ORIENTED_EDGE ( 'NONE', *, *, #4211, .F. ) ;
#11117=CARTESIAN_POINT ( 'NONE',  ( 4.458734124999998549, -43.97916666530106511, -2.574251347313721627 ) ) ;
#11119=CARTESIAN_POINT ( 'NONE',  ( 1.975475456537005874E-15, -41.62499999726880162, 5.000000000000000000 ) ) ;
#11120=CARTESIAN_POINT ( 'NONE',  ( -4.458734124999999437, -89.39583333196773651, -2.574251347313719407 ) ) ;
#11121=AXIS2_PLACEMENT_3D ( 'NONE', #1157, #34909, #15926 ) ;
#11122=CARTESIAN_POINT ( 'NONE',  ( 4.458734124999999437, 6.187500001365593860, -5.460374474430324690E-16 ) ) ;
#11123=CARTESIAN_POINT ( 'NONE',  ( -4.999999999999998224, -73.79166666393547303, 2.886751345948131764 ) ) ;
#11126=CARTESIAN_POINT ( 'NONE',  ( 4.458734125000001214, 13.85416666803226171, 2.574251347313718519 ) ) ;
#11128=CARTESIAN_POINT ( 'NONE',  ( -5.000000000000000000, 9.125000002731184168, 0.000000000000000000 ) ) ;
#11130=ORIENTED_EDGE ( 'NONE', *, *, #45236, .T. ) ;
#11131=CARTESIAN_POINT ( 'NONE',  ( -1.339745962155610925, 8.205341801261479162, 5.000000000000000000 ) ) ;
#11132=VERTEX_POINT ( 'NONE', #10002 ) ;
#11134=CARTESIAN_POINT ( 'NONE',  ( -4.458734124999999437, -42.39583333196773651, -2.574251347313719407 ) ) ;
#11135=EDGE_CURVE ( 'NONE', #2325, #1738, #29936, .T. ) ;
#11136=CARTESIAN_POINT ( 'NONE',  ( 2.500000000000002220, -59.54166666393546592, 4.330127018922192761 ) ) ;
#11138=CARTESIAN_POINT ( 'NONE',  ( 5.000000000000000888, -40.45833333060214443, 2.886751345948126879 ) ) ;
#11140=CARTESIAN_POINT ( 'NONE',  ( -3.152548672688508926E-16, -20.56249999863440081, -5.148502694627439702 ) ) ;
#11141=ORIENTED_EDGE ( 'NONE', *, *, #28767, .T. ) ;
#11142=CARTESIAN_POINT ( 'NONE',  ( -5.000000000000000000, -85.08333333333332860, -2.886751345948128211 ) ) ;
#11143=CARTESIAN_POINT ( 'NONE',  ( -1.846868145590734756, -169.1250000013656347, -4.458734125000000326 ) ) ;
#11146=CARTESIAN_POINT ( 'NONE',  ( -2.500000000000000444, -89.04166666393547303, -4.330127018922193649 ) ) ;
#11147=CARTESIAN_POINT ( 'NONE',  ( -4.999999999999998224, -34.79166666393547303, 2.886751345948131764 ) ) ;
#11148=ORIENTED_EDGE ( 'NONE', *, *, #57913, .F. ) ;
#11151=CARTESIAN_POINT ( 'NONE',  ( 9.457646018065525792E-16, -32.31249999863440792, 5.148502694627439702 ) ) ;
#11152=CARTESIAN_POINT ( 'NONE',  ( 5.000000000000000888, -5.458333330602148870, 2.886751345948126879 ) ) ;
#11157=CARTESIAN_POINT ( 'NONE',  ( 1.975475456537005874E-15, -44.74999999999999289, 5.000000000000000000 ) ) ;
#11159=CARTESIAN_POINT ( 'NONE',  ( 1.975475456537005874E-15, -25.75000000000000355, 5.000000000000000000 ) ) ;
#11161=CARTESIAN_POINT ( 'NONE',  ( 4.458734125000001214, -77.14583333196775072, 2.574251347313718519 ) ) ;
#11164=CARTESIAN_POINT ( 'NONE',  ( -8.190561711645485556E-16, -142.9375000013656063, 4.458734124999999437 ) ) ;
#11166=CARTESIAN_POINT ( 'NONE',  ( -4.458734124999999437, -47.31249999863440792, 0.000000000000000000 ) ) ;
#11170=CARTESIAN_POINT ( 'NONE',  ( -1.846868145590737420, -141.0000000013656063, 4.458734124999999437 ) ) ;
#11175=CARTESIAN_POINT ( 'NONE',  ( 2.229367062499998831, -71.89583333196773651, -3.861377020970580887 ) ) ;
#11176=DIRECTION ( 'NONE',  ( -0.000000000000000000, 1.000000000000000000, -0.000000000000000000 ) ) ;
#11186=CARTESIAN_POINT ( 'NONE',  ( 2.229367062499998831, 18.10416666803225993, -3.861377020970580887 ) ) ;
#11189=EDGE_CURVE ( 'NONE', #57597, #15422, #49562, .T. ) ;
#11194=CARTESIAN_POINT ( 'NONE',  ( -4.458734124999999437, -83.31249999863439371, 0.000000000000000000 ) ) ;
#11195=CARTESIAN_POINT ( 'NONE',  ( 2.229367062499998831, -1.645833331967737401, -3.861377020970580887 ) ) ;
#11196=CARTESIAN_POINT ( 'NONE',  ( 6.123233995736766282E-16, -170.0000000000000000, -5.000000000000000000 ) ) ;
#11198=CARTESIAN_POINT ( 'NONE',  ( 9.457646018065525792E-16, -28.31249999863440081, 5.148502694627439702 ) ) ;
#11199=AXIS2_PLACEMENT_3D ( 'NONE', #28140, #18497, #47757 ) ;
#11204=CARTESIAN_POINT ( 'NONE',  ( 2.229367062499998831, 18.35416666803225993, -3.861377020970580887 ) ) ;
#11207=CARTESIAN_POINT ( 'NONE',  ( -2.229367062500000163, -76.72916666530106511, -3.861377020970580443 ) ) ;
#11209=CARTESIAN_POINT ( 'NONE',  ( 2.500000000000002220, 23.45833333606451632, 4.330127018922192761 ) ) ;
#11212=CARTESIAN_POINT ( 'NONE',  ( 6.123233995736766282E-16, -170.0000000000000000, -5.000000000000000000 ) ) ;
#11213=CARTESIAN_POINT ( 'NONE',  ( -9.184850993605147944E-16, -140.2500000000000000, 5.000000000000000000 ) ) ;
#11214=CARTESIAN_POINT ( 'NONE',  ( 1.060575238724906964E-15, -25.75000000000000000, 5.773502691896257311 ) ) ;
#11215=CARTESIAN_POINT ( 'NONE',  ( -2.229367062500000163, -25.47916666530106866, -3.861377020970580443 ) ) ;
#11216=CARTESIAN_POINT ( 'NONE',  ( -2.229367062500000163, -87.47916666530107932, -3.861377020970580443 ) ) ;
#11217=CARTESIAN_POINT ( 'NONE',  ( 5.000000000000000888, -22.45833333060214088, 2.886751345948126879 ) ) ;
#11218=CARTESIAN_POINT ( 'NONE',  ( 2.229367062500001939, -53.97916666530107221, 3.861377020970579999 ) ) ;
#11219=ORIENTED_EDGE ( 'NONE', *, *, #17824, .T. ) ;
#11220=CARTESIAN_POINT ( 'NONE',  ( 5.000000000000000000, -49.50000000000000000, -6.123233995736766282E-16 ) ) ;
#11222=CARTESIAN_POINT ( 'NONE',  ( -2.229367062499996610, -2.395833331967737845, 3.861377020970582219 ) ) ;
#11224=CARTESIAN_POINT ( 'NONE',  ( -4.999999999999999112, -63.91666666666666430, 2.886751345948131764 ) ) ;
#11225=CARTESIAN_POINT ( 'NONE',  ( -3.152801135295367096, -150.3125000013655779, -3.152801135295367541 ) ) ;
#11228=CARTESIAN_POINT ( 'NONE',  ( -2.071067811865478170, -157.3125000000000000, 5.000000000000000000 ) ) ;
#11229=CARTESIAN_POINT ( 'NONE',  ( -6.972266317189433020E-16, -10.12499999726881406, -5.000000000000000000 ) ) ;
#11231=CARTESIAN_POINT ( 'NONE',  ( -2.229367062500000163, -13.72916666530107221, -3.861377020970580443 ) ) ;
#11232=CARTESIAN_POINT ( 'NONE',  ( -2.229367062500000163, -52.72916666530107221, -3.861377020970580443 ) ) ;
#11233=( BOUNDED_CURVE ( )  B_SPLINE_CURVE ( 2, ( #15450, #15764, #49531, #26052, #45666, #30543, #50167, #6443, #6122 ),
 .UNSPECIFIED., .F., .F. ) 
 B_SPLINE_CURVE_WITH_KNOTS ( ( 3, 2, 2, 2, 3 ),
 ( 0.1437499999999999889, 0.1444444444444444309, 0.1458333333333333426, 0.1472222222222222265, 0.1479166666666666685 ),
 .UNSPECIFIED. ) 
 CURVE ( )  GEOMETRIC_REPRESENTATION_ITEM ( )  RATIONAL_B_SPLINE_CURVE ( ( 0.9330127018922194093, 0.9330127018922194093, 1.000000000000000000, 0.8660254037844387076, 1.000000000000000000, 0.8660254037844387076, 1.000000000000000000, 0.9330127018922194093, 0.9330127018922194093 ) ) 
 REPRESENTATION_ITEM ( '' )  );
#11234=CARTESIAN_POINT ( 'NONE',  ( 5.275681513340003914E-14, 10.74999999999999645, -5.000000000000000000 ) ) ;
#11235=CARTESIAN_POINT ( 'NONE',  ( 4.458734125000000326, -144.3750000013656063, -1.846868145590734978 ) ) ;
#11238=ORIENTED_EDGE ( 'NONE', *, *, #5883, .F. ) ;
#11240=CARTESIAN_POINT ( 'NONE',  ( -3.152548672688508926E-16, 27.18750000136559564, -5.148502694627439702 ) ) ;
#11242=COLOUR_RGB ( '',0.8941176470588234615, 0.8941176470588234615, 0.8941176470588234615 ) ;
#11243=CARTESIAN_POINT ( 'NONE',  ( -6.972266317189433020E-16, -50.24999999999999289, -5.000000000000000000 ) ) ;
#11244=ORIENTED_EDGE ( 'NONE', *, *, #54759, .F. ) ;
#11246=CARTESIAN_POINT ( 'NONE',  ( 2.499999999999998668, -19.33333333333333570, -4.330127018922193649 ) ) ;
#11248=CARTESIAN_POINT ( 'NONE',  ( -2.500000000000000444, 8.833333333333332149, -4.330127018922193649 ) ) ;
#11249=CARTESIAN_POINT ( 'NONE',  ( 2.229367062500001939, -5.979166665301072214, 3.861377020970579999 ) ) ;
#11251=CARTESIAN_POINT ( 'NONE',  ( -1.846868145590737420, -148.7500000013656063, 4.458734124999997661 ) ) ;
#11254=CARTESIAN_POINT ( 'NONE',  ( -5.000000000000000000, -26.87499999726881583, 0.000000000000000000 ) ) ;
#11257=CARTESIAN_POINT ( 'NONE',  ( 1.339745962155612702, -25.16965819600734022, -5.000000000000000000 ) ) ;
#11258=CARTESIAN_POINT ( 'NONE',  ( 5.000000000000000000, 1.625000002731184834, -6.123233995736766282E-16 ) ) ;
#11261=DIRECTION ( 'NONE',  ( -0.000000000000000000, 1.000000000000000000, -0.000000000000000000 ) ) ;
#11265=CARTESIAN_POINT ( 'NONE',  ( 2.229367062499998831, 10.35416666803225993, -3.861377020970580887 ) ) ;
#11267=CARTESIAN_POINT ( 'NONE',  ( 2.229367062499998831, -14.89583333196773474, -3.861377020970580887 ) ) ;
#11269=CARTESIAN_POINT ( 'NONE',  ( -8.190561711645485556E-16, -165.6875000013655779, 4.458734124999999437 ) ) ;
#11270=CARTESIAN_POINT ( 'NONE',  ( 2.499999999999998668, 23.66666666666666430, -4.330127018922193649 ) ) ;
#11276=CARTESIAN_POINT ( 'NONE',  ( -4.458734124999997661, -35.22916666530107221, 2.574251347313722516 ) ) ;
#11279=CARTESIAN_POINT ( 'NONE',  ( -1.339745962155610925, -57.66965819600732601, 5.000000000000000000 ) ) ;
#11285=CARTESIAN_POINT ( 'NONE',  ( -3.535250795749689387E-16, -0.2500000000000002220, -5.773502691896257311 ) ) ;
#11286=CARTESIAN_POINT ( 'NONE',  ( 4.458734124999999437, -72.81249999863439371, -5.460374474430324690E-16 ) ) ;
#11287=CARTESIAN_POINT ( 'NONE',  ( 1.339745962155612702, -22.16965819600733312, -5.000000000000000000 ) ) ;
#11288=CARTESIAN_POINT ( 'NONE',  ( -2.500000000000000444, -7.041666663935481907, -4.330127018922193649 ) ) ;
#11289=CARTESIAN_POINT ( 'NONE',  ( -2.229367062499996610, -41.14583333196773651, 3.861377020970582219 ) ) ;
#11292=CARTESIAN_POINT ( 'NONE',  ( -3.152548672688508926E-16, 11.18750000136559564, -5.148502694627439702 ) ) ;
#11293=VERTEX_POINT ( 'NONE', #50198 ) ;
#11295=CARTESIAN_POINT ( 'NONE',  ( -5.000000000000000000, -52.99999999999999289, 0.000000000000000000 ) ) ;
#11298=CARTESIAN_POINT ( 'NONE',  ( 9.457646018065525792E-16, -76.06249999863440792, 5.148502694627439702 ) ) ;
#11299=( BOUNDED_CURVE ( )  B_SPLINE_CURVE ( 2, ( #43069, #62707, #13800, #33421, #18932, #33733, #53351, #9286, #44323 ),
 .UNSPECIFIED., .F., .F. ) 
 B_SPLINE_CURVE_WITH_KNOTS ( ( 3, 2, 2, 2, 3 ),
 ( 0.9187499999999999556, 0.9194444444444443976, 0.9208333333333332815, 0.9222222222222222765, 0.9229166666666667185 ),
 .UNSPECIFIED. ) 
 CURVE ( )  GEOMETRIC_REPRESENTATION_ITEM ( )  RATIONAL_B_SPLINE_CURVE ( ( 0.9330127018922194093, 0.9330127018922194093, 1.000000000000000000, 0.8660254037844387076, 1.000000000000000000, 0.8660254037844387076, 1.000000000000000000, 0.9330127018922194093, 0.9330127018922194093 ) ) 
 REPRESENTATION_ITEM ( '' )  );
#11300=CARTESIAN_POINT ( 'NONE',  ( -4.458734125000000326, -141.2500000013656063, -1.846868145590735644 ) ) ;
#11301=CARTESIAN_POINT ( 'NONE',  ( 9.457646018065525792E-16, -80.06249999863439371, 5.148502694627439702 ) ) ;
#11303=CARTESIAN_POINT ( 'NONE',  ( -4.458734124999999437, -35.56249999863440792, 0.000000000000000000 ) ) ;
#11304=VERTEX_POINT ( 'NONE', #29287 ) ;
#11305=CARTESIAN_POINT ( 'NONE',  ( 1.975475456537005874E-15, -16.62499999726881583, 5.000000000000000000 ) ) ;
#11310=LINE ( 'NONE', #30292, #43932 ) ;
#11312=CARTESIAN_POINT ( 'NONE',  ( -4.458734124999998549, -63.47916666530106511, 2.574251347313722516 ) ) ;
#11316=CARTESIAN_POINT ( 'NONE',  ( 1.339745962155590275, 3.419658201469704562, 5.000000000000013323 ) ) ;
#11318=ORIENTED_EDGE ( 'NONE', *, *, #10316, .F. ) ;
#11320=CARTESIAN_POINT ( 'NONE',  ( -2.229367062499996610, 5.854166668032262599, 3.861377020970582219 ) ) ;
#11322=CARTESIAN_POINT ( 'NONE',  ( 4.458734124999999437, -160.3750000013655779, -1.846868145590734978 ) ) ;
#11329=CARTESIAN_POINT ( 'NONE',  ( -2.498395430326213474E-14, 15.25000000000000000, 5.000000000000000000 ) ) ;
#11330=EDGE_CURVE ( 'NONE', #46232, #51312, #23879, .T. ) ;
#11331=CARTESIAN_POINT ( 'NONE',  ( 5.000000000000000888, 4.541666669397852019, 2.886751345948126879 ) ) ;
#11338=CARTESIAN_POINT ( 'NONE',  ( -3.152548672688508926E-16, 26.43750000136559564, -5.148502694627439702 ) ) ;
#11341=CARTESIAN_POINT ( 'NONE',  ( -4.458734124999997661, 1.520833334698927564, 2.574251347313722516 ) ) ;
#11342=CARTESIAN_POINT ( 'NONE',  ( -5.000000000000000888, -149.5625000027311842, 2.071067811865474617 ) ) ;
#11344=CARTESIAN_POINT ( 'NONE',  ( -2.071067811865478170, -146.4375000027311842, 5.000000000000000000 ) ) ;
#11348=EDGE_CURVE ( 'NONE', #897, #42031, #19358, .T. ) ;
#11350=DIRECTION ( 'NONE',  ( 0.000000000000000000, 0.000000000000000000, 1.000000000000000000 ) ) ;
#11351=DIRECTION ( 'NONE',  ( -0.000000000000000000, 1.000000000000000000, -0.000000000000000000 ) ) ;
#11353=CARTESIAN_POINT ( 'NONE',  ( -4.458734124999999437, -161.2500000013655779, -1.846868145590735644 ) ) ;
#11355=CARTESIAN_POINT ( 'NONE',  ( -1.846868145590734756, -141.1250000013655779, -4.458734125000000326 ) ) ;
#11356=ORIENTED_EDGE ( 'NONE', *, *, #23548, .T. ) ;
#11357=CARTESIAN_POINT ( 'NONE',  ( 4.458734125000001214, 23.85416666803225993, 2.574251347313718519 ) ) ;
#11358=VERTEX_POINT ( 'NONE', #26717 ) ;
#11360=CARTESIAN_POINT ( 'NONE',  ( 1.339745962155615144, 2.294658198738519950, 4.999999999999999112 ) ) ;
#11361=CARTESIAN_POINT ( 'NONE',  ( 5.000000000000000000, 11.58333333333333570, -2.886751345948129988 ) ) ;
#11362=CARTESIAN_POINT ( 'NONE',  ( -4.458734124999997661, -52.22916666530107932, 2.574251347313722516 ) ) ;
#11363=CARTESIAN_POINT ( 'NONE',  ( 4.458734124999998549, -13.72916666530107399, -2.574251347313721627 ) ) ;
#11365=EDGE_CURVE ( 'NONE', #46520, #56134, #51170, .T. ) ;
#11367=CARTESIAN_POINT ( 'NONE',  ( 0.000000000000000000, -170.0000000000000000, 5.000000000000000000 ) ) ;
#11368=CARTESIAN_POINT ( 'NONE',  ( -1.339745962155613812, -37.20534180126147561, -5.000000000000000000 ) ) ;
#11370=CARTESIAN_POINT ( 'NONE',  ( 5.000000000000000000, -35.50000000000000711, -6.123233995736766282E-16 ) ) ;
#11373=CARTESIAN_POINT ( 'NONE',  ( 5.000000000000000000, 21.62500000273118417, -6.123233995736766282E-16 ) ) ;
#11375=DIRECTION ( 'NONE',  ( -0.000000000000000000, 1.000000000000000000, -0.000000000000000000 ) ) ;
#11376=CARTESIAN_POINT ( 'NONE',  ( 2.229367062500001939, -56.97916666530107932, 3.861377020970579999 ) ) ;
#11377=CARTESIAN_POINT ( 'NONE',  ( 4.458734125000000326, -153.6250000013655779, -1.846868145590734978 ) ) ;
#11378=VECTOR ( 'NONE', #24735, 1000.000000000000000 ) ;
#11379=CARTESIAN_POINT ( 'NONE',  ( -4.458734124999999437, -65.31249999863440792, 0.000000000000000000 ) ) ;
#11381=CARTESIAN_POINT ( 'NONE',  ( 2.500000000000002220, -57.54166666393548013, 4.330127018922192761 ) ) ;
#11382=ORIENTED_EDGE ( 'NONE', *, *, #22011, .F. ) ;
#11385=CARTESIAN_POINT ( 'NONE',  ( 0.000000000000000000, -170.0000000000000000, 0.000000000000000000 ) ) ;
#11387=CARTESIAN_POINT ( 'NONE',  ( 1.846868145590735200, -154.2500000013656063, -4.458734125000000326 ) ) ;
#11388=ORIENTED_EDGE ( 'NONE', *, *, #38099, .F. ) ;
#11389=CARTESIAN_POINT ( 'NONE',  ( -6.972266317189433020E-16, -54.24999999999999289, -5.000000000000000000 ) ) ;
#11392=CARTESIAN_POINT ( 'NONE',  ( 4.458734125000001214, -48.14583333196773651, 2.574251347313718519 ) ) ;
#11394=VERTEX_POINT ( 'NONE', #21253 ) ;
#11395=EDGE_CURVE ( 'NONE', #1059, #20760, #35733, .T. ) ;
#11397=CARTESIAN_POINT ( 'NONE',  ( -6.972266317189433020E-16, 16.87500000273118417, -5.000000000000000000 ) ) ;
#11399=CARTESIAN_POINT ( 'NONE',  ( -3.152548672688508926E-16, 25.43750000136559208, -5.148502694627439702 ) ) ;
#11402=CARTESIAN_POINT ( 'NONE',  ( 0.000000000000000000, -170.0000000000000000, 5.000000000000000000 ) ) ;
#11406=( BOUNDED_CURVE ( )  B_SPLINE_CURVE ( 2, ( #55901, #16341, #40134, #1882, #21487, #1250, #50440, #51070, #20208 ),
 .UNSPECIFIED., .F., .F. ) 
 B_SPLINE_CURVE_WITH_KNOTS ( ( 3, 2, 2, 2, 3 ),
 ( 0.8854166666666666297, 0.8861111111111110716, 0.8874999999999999556, 0.8888888888888888395, 0.8895833333333332815 ),
 .UNSPECIFIED. ) 
 CURVE ( )  GEOMETRIC_REPRESENTATION_ITEM ( )  RATIONAL_B_SPLINE_CURVE ( ( 0.9330127018922194093, 0.9330127018922194093, 1.000000000000000000, 0.8660254037844387076, 1.000000000000000000, 0.8660254037844387076, 1.000000000000000000, 0.9330127018922194093, 0.9330127018922194093 ) ) 
 REPRESENTATION_ITEM ( '' )  );
#11407=CARTESIAN_POINT ( 'NONE',  ( 1.975475456537005874E-15, -63.74999999999998579, 5.000000000000000000 ) ) ;
#11408=CARTESIAN_POINT ( 'NONE',  ( -6.972266317189433020E-16, -2.124999997268814056, -5.000000000000000000 ) ) ;
#11411=FACE_OUTER_BOUND ( 'NONE', #33468, .T. ) ;
#11412=EDGE_CURVE ( 'NONE', #8866, #61326, #32724, .T. ) ;
#11413=CYLINDRICAL_SURFACE ( 'NONE', #11121, 5.000000000000000000 ) ;
#11418=CARTESIAN_POINT ( 'NONE',  ( -9.184850993605147944E-16, -143.3750000027312126, 5.000000000000000000 ) ) ;
#11420=CARTESIAN_POINT ( 'NONE',  ( -5.000000000000000888, -155.6875000027312126, -2.071067811865475949 ) ) ;
#11423=AXIS2_PLACEMENT_3D ( 'NONE', #58441, #15246, #57199 ) ;
#11431=CARTESIAN_POINT ( 'NONE',  ( 1.975475456537005874E-15, -89.74999999999998579, 5.000000000000000000 ) ) ;
#11432=CARTESIAN_POINT ( 'NONE',  ( -2.229367062499996610, -21.14583333196774007, 3.861377020970582219 ) ) ;
#11434=CARTESIAN_POINT ( 'NONE',  ( 2.071067811865476394, -151.1875000000000000, 5.000000000000000000 ) ) ;
#11436=CARTESIAN_POINT ( 'NONE',  ( 1.846868145590736310, -151.6250000013656063, 4.458734124999999437 ) ) ;
#11437=ORIENTED_EDGE ( 'NONE', *, *, #16894, .F. ) ;
#11438=CARTESIAN_POINT ( 'NONE',  ( -4.458734124999999437, -43.64583333196773651, -2.574251347313719407 ) ) ;
#11441=CARTESIAN_POINT ( 'NONE',  ( 1.060575238724906964E-15, 29.25000000000000000, 5.773502691896257311 ) ) ;
#11442=CARTESIAN_POINT ( 'NONE',  ( 4.458734124999998549, 3.270833334698929118, -2.574251347313721627 ) ) ;
#11443=CARTESIAN_POINT ( 'NONE',  ( -9.184850993605147944E-16, -160.3750000027311842, 5.000000000000000000 ) ) ;
#11444=CARTESIAN_POINT ( 'NONE',  ( 2.499999999999998668, -11.20833333060214798, -4.330127018922193649 ) ) ;
#11446=CARTESIAN_POINT ( 'NONE',  ( 4.458734124999999437, 15.93750000136559564, -5.460374474430324690E-16 ) ) ;
#11448=CARTESIAN_POINT ( 'NONE',  ( 5.000000000000000000, 7.625000002731186832, -6.123233995736766282E-16 ) ) ;
#11449=ORIENTED_EDGE ( 'NONE', *, *, #57018, .F. ) ;
#11450=CARTESIAN_POINT ( 'NONE',  ( 1.975475456537005874E-15, 4.375000002731185056, 5.000000000000000000 ) ) ;
#11453=CARTESIAN_POINT ( 'NONE',  ( 4.458734124999999437, -45.81249999863440081, -5.460374474430324690E-16 ) ) ;
#11454=CARTESIAN_POINT ( 'NONE',  ( 4.458734125000000326, -164.6250000013655779, -1.846868145590734978 ) ) ;
#11455=CARTESIAN_POINT ( 'NONE',  ( 2.499999999999998668, -42.20833333060214443, -4.330127018922193649 ) ) ;
#11457=CARTESIAN_POINT ( 'NONE',  ( 4.458734124999999437, -16.81249999863440436, -5.460374474430324690E-16 ) ) ;
#11459=CARTESIAN_POINT ( 'NONE',  ( 2.500000000000002220, -87.66666666666667140, 4.330127018922192761 ) ) ;
#11460=CARTESIAN_POINT ( 'NONE',  ( -4.458734124999999437, -162.9375000013655779, -5.460374474430324690E-16 ) ) ;
#11461=CARTESIAN_POINT ( 'NONE',  ( 2.500000000000002220, -87.54166666393547303, 4.330127018922192761 ) ) ;
#11462=CARTESIAN_POINT ( 'NONE',  ( -1.049326080737009628E-13, -20.62499999726881583, 5.000000000000000000 ) ) ;
#11466=CARTESIAN_POINT ( 'NONE',  ( -4.458734124999998549, -32.47916666530107221, 2.574251347313722516 ) ) ;
#11468=EDGE_LOOP ( 'NONE', ( #24641, #38954, #55862, #10859 ) ) ;
#11476=CARTESIAN_POINT ( 'NONE',  ( -1.339745962155613812, -26.20534180126147916, -5.000000000000000000 ) ) ;
#11478=CARTESIAN_POINT ( 'NONE',  ( -2.229367062499996610, -79.39583333196773651, 3.861377020970582219 ) ) ;
#11481=CARTESIAN_POINT ( 'NONE',  ( 1.846868145590736310, -141.8750000013656063, 4.458734124999997661 ) ) ;
#11482=( BOUNDED_CURVE ( )  B_SPLINE_CURVE ( 2, ( #425, #29670, #9115, #24865, #28723, #9422, #19391, #20030, #18758 ),
 .UNSPECIFIED., .F., .F. ) 
 B_SPLINE_CURVE_WITH_KNOTS ( ( 3, 2, 2, 2, 3 ),
 ( 0.5770833333333332815, 0.5777777777777777235, 0.5791666666666667185, 0.5805555555555556024, 0.5812500000000000444 ),
 .UNSPECIFIED. ) 
 CURVE ( )  GEOMETRIC_REPRESENTATION_ITEM ( )  RATIONAL_B_SPLINE_CURVE ( ( 0.9330127018922194093, 0.9330127018922194093, 1.000000000000000000, 0.8660254037844387076, 1.000000000000000000, 0.8660254037844387076, 1.000000000000000000, 0.9330127018922194093, 0.9330127018922194093 ) ) 
 REPRESENTATION_ITEM ( '' )  );
#11483=CARTESIAN_POINT ( 'NONE',  ( 1.339745962155612702, 20.70534180126147916, -5.000000000000000000 ) ) ;
#11485=CARTESIAN_POINT ( 'NONE',  ( 4.458734125000000326, -45.89583333196774362, 2.574251347313718519 ) ) ;
#11486=CARTESIAN_POINT ( 'NONE',  ( -2.500000000000000444, 27.83333333333333215, -4.330127018922193649 ) ) ;
#11487=EDGE_CURVE ( 'NONE', #16047, #8105, #21829, .T. ) ;
#11491=CYLINDRICAL_SURFACE ( 'NONE', #37114, 5.000000000000000000 ) ;
#11496=CARTESIAN_POINT ( 'NONE',  ( -2.229367062500000163, -79.72916666530106511, -3.861377020970580443 ) ) ;
#11501=EDGE_LOOP ( 'NONE', ( #13916, #15968, #13102, #17732 ) ) ;
#11505=DIRECTION ( 'NONE',  ( -0.000000000000000000, 1.000000000000000000, -0.000000000000000000 ) ) ;
#11507=CARTESIAN_POINT ( 'NONE',  ( 2.229367062499998831, 20.10416666803225993, -3.861377020970580887 ) ) ;
#11514=CARTESIAN_POINT ( 'NONE',  ( -4.458734124999999437, -84.31249999863439371, 0.000000000000000000 ) ) ;
#11515=CARTESIAN_POINT ( 'NONE',  ( 2.229367062500001939, -2.979166665301069550, 3.861377020970579999 ) ) ;
#11517=ORIENTED_EDGE ( 'NONE', *, *, #28268, .T. ) ;
#11518=CARTESIAN_POINT ( 'NONE',  ( 2.229367062500001939, -32.22916666530106511, 3.861377020970579999 ) ) ;
#11522=CARTESIAN_POINT ( 'NONE',  ( 4.458734125000001214, 20.10416666803225993, 2.574251347313718519 ) ) ;
#11524=CARTESIAN_POINT ( 'NONE',  ( 5.000000000000000888, -28.58333333333333570, 2.886751345948126879 ) ) ;
#11525=CARTESIAN_POINT ( 'NONE',  ( -4.458734124999999437, -79.56249999863440792, 0.000000000000000000 ) ) ;
#11528=CARTESIAN_POINT ( 'NONE',  ( -2.499999999999996447, 24.29166666939785202, 4.330127018922195425 ) ) ;
#11531=( BOUNDED_CURVE ( )  B_SPLINE_CURVE ( 2, ( #122, #39325, #4603, #43832, #63478, #45118, #31270, #26459, #5892 ),
 .UNSPECIFIED., .F., .F. ) 
 B_SPLINE_CURVE_WITH_KNOTS ( ( 3, 2, 2, 2, 3 ),
 ( 0.7354166666666667185, 0.7361111111111111605, 0.7375000000000000444, 0.7388888888888889284, 0.7395833333333333703 ),
 .UNSPECIFIED. ) 
 CURVE ( )  GEOMETRIC_REPRESENTATION_ITEM ( )  RATIONAL_B_SPLINE_CURVE ( ( 0.9330127018922194093, 0.9330127018922194093, 1.000000000000000000, 0.8660254037844387076, 1.000000000000000000, 0.8660254037844387076, 1.000000000000000000, 0.9330127018922194093, 0.9330127018922194093 ) ) 
 REPRESENTATION_ITEM ( '' )  );
#11532=CARTESIAN_POINT ( 'NONE',  ( 5.000000000000000000, -139.5625000013656063, 0.000000000000000000 ) ) ;
#11533=CARTESIAN_POINT ( 'NONE',  ( -2.499999999999996447, -24.83333333333333215, 4.330127018922195425 ) ) ;
#11534=CARTESIAN_POINT ( 'NONE',  ( -3.152548672688508926E-16, -26.56249999863440792, -5.148502694627439702 ) ) ;
#11535=CARTESIAN_POINT ( 'NONE',  ( -4.458734124999999437, -88.39583333196773651, -2.574251347313719407 ) ) ;
#11536=CARTESIAN_POINT ( 'NONE',  ( 2.499999999999998668, -21.20833333060214798, -4.330127018922193649 ) ) ;
#11537=CARTESIAN_POINT ( 'NONE',  ( -4.458734124999999437, -54.31249999863440081, 0.000000000000000000 ) ) ;
#11540=CARTESIAN_POINT ( 'NONE',  ( 0.000000000000000000, -170.0000000000000000, 5.000000000000000000 ) ) ;
#11541=CARTESIAN_POINT ( 'NONE',  ( 9.457646018065525792E-16, -5.312499998634402587, 5.148502694627439702 ) ) ;
#11542=VERTEX_POINT ( 'NONE', #58739 ) ;
#11543=CARTESIAN_POINT ( 'NONE',  ( -4.999999999999999112, -69.91666666666667140, 2.886751345948131764 ) ) ;
#11544=CARTESIAN_POINT ( 'NONE',  ( 4.458734124999999437, -152.7500000013656063, 1.846868145590737864 ) ) ;
#11547=CARTESIAN_POINT ( 'NONE',  ( -9.184850993605147944E-16, -157.2500000000000000, 5.000000000000000000 ) ) ;
#11548=CARTESIAN_POINT ( 'NONE',  ( -2.500000000000000444, -71.04166666393547303, -4.330127018922193649 ) ) ;
#11551=CARTESIAN_POINT ( 'NONE',  ( 2.229367062500001939, -16.22916666530107577, 3.861377020970579999 ) ) ;
#11552=CARTESIAN_POINT ( 'NONE',  ( -3.152548672688508926E-16, -49.81249999863440081, -5.148502694627439702 ) ) ;
#11554=CARTESIAN_POINT ( 'NONE',  ( -8.190561711645485556E-16, -145.6875000013656063, 4.458734124999999437 ) ) ;
#11559=CARTESIAN_POINT ( 'NONE',  ( 4.458734125000001214, 24.85416666803225993, 2.574251347313718519 ) ) ;
#11567=CARTESIAN_POINT ( 'NONE',  ( 4.458734125000001214, -8.895833331967736513, 2.574251347313718519 ) ) ;
#11568=CARTESIAN_POINT ( 'NONE',  ( 1.975475456537005874E-15, 6.375000002731185944, 5.000000000000000000 ) ) ;
#11569=CARTESIAN_POINT ( 'NONE',  ( -4.458734125000000326, -143.8750000013656063, 1.846868145590734089 ) ) ;
#11571=VERTEX_POINT ( 'NONE', #38480 ) ;
#11576=CARTESIAN_POINT ( 'NONE',  ( 1.339745962155612702, -85.16965819600733312, -5.000000000000000000 ) ) ;
#11577=CARTESIAN_POINT ( 'NONE',  ( 5.000000000000000000, -88.37499999726880162, -6.123233995736766282E-16 ) ) ;
#11579=ADVANCED_FACE ( 'NONE', ( #14356 ), #14036, .T. ) ;
#11583=DIRECTION ( 'NONE',  ( 0.000000000000000000, 1.000000000000000000, 0.000000000000000000 ) ) ;
#11585=CARTESIAN_POINT ( 'NONE',  ( -4.458734124999999437, 12.68750000136559564, 0.000000000000000000 ) ) ;
#11587=CARTESIAN_POINT ( 'NONE',  ( 4.458734124999999437, -12.06249999863440081, -5.460374474430324690E-16 ) ) ;
#11589=CARTESIAN_POINT ( 'NONE',  ( 2.730187237215162345E-16, -162.1875000013655779, -4.458734124999999437 ) ) ;
#11594=CARTESIAN_POINT ( 'NONE',  ( 4.458734125000000326, -34.89583333196772941, 2.574251347313718519 ) ) ;
#11603=CARTESIAN_POINT ( 'NONE',  ( 5.000000000000000000, -7.416666666666667851, -2.886751345948129988 ) ) ;
#11604=CARTESIAN_POINT ( 'NONE',  ( -4.458734124999999437, -71.39583333196773651, -2.574251347313719407 ) ) ;
#11607=CARTESIAN_POINT ( 'NONE',  ( 5.000000000000000000, -8.374999997268814056, -6.123233995736766282E-16 ) ) ;
#11608=CARTESIAN_POINT ( 'NONE',  ( -4.458734124999998549, -39.22916666530107221, 2.574251347313722516 ) ) ;
#11610=FACE_OUTER_BOUND ( 'NONE', #49438, .T. ) ;
#11611=CARTESIAN_POINT ( 'NONE',  ( 2.229367062499998831, 11.10416666803225993, -3.861377020970580887 ) ) ;
#11612=ORIENTED_EDGE ( 'NONE', *, *, #50396, .F. ) ;
#11614=CARTESIAN_POINT ( 'NONE',  ( 2.499999999999998668, -57.33333333333333570, -4.330127018922193649 ) ) ;
#11616=CARTESIAN_POINT ( 'NONE',  ( 5.000000000000000000, -145.0624999999999716, 2.071067811865478614 ) ) ;
#11617=CARTESIAN_POINT ( 'NONE',  ( -4.458734124999998549, -76.22916666530107932, 2.574251347313722516 ) ) ;
#11618=CARTESIAN_POINT ( 'NONE',  ( 5.000000000000000000, -169.0000000000000000, 0.000000000000000000 ) ) ;
#11619=CARTESIAN_POINT ( 'NONE',  ( -3.152548672688508926E-16, -86.56249999863440792, -5.148502694627439702 ) ) ;
#11621=CARTESIAN_POINT ( 'NONE',  ( 4.458734124999998549, -33.97916666530107221, -2.574251347313721627 ) ) ;
#11627=PLANE ( 'NONE',  #48078 ) ;
#11629=CARTESIAN_POINT ( 'NONE',  ( 4.458734124999998549, -65.97916666530106511, -2.574251347313721627 ) ) ;
#11631=ORIENTED_EDGE ( 'NONE', *, *, #20143, .T. ) ;
#11632=CARTESIAN_POINT ( 'NONE',  ( -5.000000000000000888, -156.6875000027312126, -2.071067811865475949 ) ) ;
#11636=CARTESIAN_POINT ( 'NONE',  ( 2.229367062499998831, 8.354166668032261711, -3.861377020970580887 ) ) ;
#11638=CARTESIAN_POINT ( 'NONE',  ( 1.846868145590735200, -161.2500000013655779, -4.458734124999999437 ) ) ;
#11644=CARTESIAN_POINT ( 'NONE',  ( 5.000000000000000000, 25.62500000273118417, -6.123233995736766282E-16 ) ) ;
#11646=CARTESIAN_POINT ( 'NONE',  ( 5.000000000000000000, -78.41666666666667140, -2.886751345948130876 ) ) ;
#11648=CARTESIAN_POINT ( 'NONE',  ( -6.972266317189433020E-16, -79.24999999999998579, -5.000000000000000000 ) ) ;
#11650=CARTESIAN_POINT ( 'NONE',  ( -4.458734124999997661, 25.77083333469893134, 2.574251347313722516 ) ) ;
#11653=CARTESIAN_POINT ( 'NONE',  ( 4.458734125000000326, 1.854166668032262599, 2.574251347313718519 ) ) ;
#11654=CARTESIAN_POINT ( 'NONE',  ( -5.000000000000000888, -149.6875000027312126, -2.071067811865475949 ) ) ;
#11656=CARTESIAN_POINT ( 'NONE',  ( -2.071067811865478170, -144.4375000027312126, 5.000000000000000000 ) ) ;
#11663=LINE ( 'NONE', #56705, #19268 ) ;
#11665=CARTESIAN_POINT ( 'NONE',  ( 3.152801135295367541, -160.5625000013656063, -3.152801135295367541 ) ) ;
#11668=CARTESIAN_POINT ( 'NONE',  ( -1.846868145590734756, -140.1250000013655779, -4.458734125000000326 ) ) ;
#11670=CARTESIAN_POINT ( 'NONE',  ( 4.458734124999998549, 23.02083333469892423, -2.574251347313721627 ) ) ;
#11671=VERTEX_POINT ( 'NONE', #34286 ) ;
#11676=CARTESIAN_POINT ( 'NONE',  ( -5.000000000000000000, 9.999999999999998224, 0.000000000000000000 ) ) ;
#11678=CARTESIAN_POINT ( 'NONE',  ( -4.458734124999999437, -56.39583333196773651, -2.574251347313719407 ) ) ;
#11679=CARTESIAN_POINT ( 'NONE',  ( -4.458734124999998549, -11.22916666530106866, 2.574251347313722516 ) ) ;
#11685=CARTESIAN_POINT ( 'NONE',  ( 2.499999999999998668, -33.33333333333332860, -4.330127018922193649 ) ) ;
#11690=CARTESIAN_POINT ( 'NONE',  ( -4.458734124999998549, -60.22916666530106511, 2.574251347313722516 ) ) ;
#11691=CARTESIAN_POINT ( 'NONE',  ( -8.190561711645485556E-16, -150.9375000013656063, 4.458734124999999437 ) ) ;
#11692=CARTESIAN_POINT ( 'NONE',  ( 9.457646018065525792E-16, -70.06249999863439371, 5.148502694627439702 ) ) ;
#11694=CARTESIAN_POINT ( 'NONE',  ( -3.152548672688508926E-16, -21.81249999863440436, -5.148502694627439702 ) ) ;
#11695=CARTESIAN_POINT ( 'NONE',  ( -2.499999999999996447, -58.70833333060214443, 4.330127018922195425 ) ) ;
#11696=ORIENTED_EDGE ( 'NONE', *, *, #40815, .T. ) ;
#11697=CARTESIAN_POINT ( 'NONE',  ( 5.000000000000000000, -31.29166666393548724, -2.886751345948130876 ) ) ;
#11698=ORIENTED_EDGE ( 'NONE', *, *, #35825, .F. ) ;
#11700=CARTESIAN_POINT ( 'NONE',  ( -5.000000000000000000, -157.6250000027311842, -6.123233995736766282E-16 ) ) ;
#11702=CARTESIAN_POINT ( 'NONE',  ( -3.152801135295367096, -154.0625000013656063, -3.152801135295367541 ) ) ;
#11703=EDGE_LOOP ( 'NONE', ( #45885, #21974, #54800, #32668 ) ) ;
#11704=( BOUNDED_CURVE ( )  B_SPLINE_CURVE ( 2, ( #57387, #39001, #62212, #48028, #37755, #43195, #38679, #53175, #38376 ),
 .UNSPECIFIED., .F., .F. ) 
 B_SPLINE_CURVE_WITH_KNOTS ( ( 3, 2, 2, 2, 3 ),
 ( 0.2645833333333333370, 0.2652777777777777790, 0.2666666666666666630, 0.2680555555555555469, 0.2687499999999999889 ),
 .UNSPECIFIED. ) 
 CURVE ( )  GEOMETRIC_REPRESENTATION_ITEM ( )  RATIONAL_B_SPLINE_CURVE ( ( 0.9330127018922194093, 0.9330127018922194093, 1.000000000000000000, 0.8660254037844387076, 1.000000000000000000, 0.8660254037844387076, 1.000000000000000000, 0.9330127018922194093, 0.9330127018922194093 ) ) 
 REPRESENTATION_ITEM ( '' )  );
#11707=CARTESIAN_POINT ( 'NONE',  ( -2.499999999999996447, -74.70833333060214443, 4.330127018922195425 ) ) ;
#11708=CARTESIAN_POINT ( 'NONE',  ( 2.229367062499998831, -45.89583333196774362, -3.861377020970580887 ) ) ;
#11711=CARTESIAN_POINT ( 'NONE',  ( 5.000000000000000000, 10.70833333606451987, -2.886751345948130876 ) ) ;
#11713=CARTESIAN_POINT ( 'NONE',  ( 4.458734124999999437, 23.18750000136559564, -5.460374474430324690E-16 ) ) ;
#11716=CARTESIAN_POINT ( 'NONE',  ( 2.500000000000002220, -61.54166666393547303, 4.330127018922192761 ) ) ;
#11726=CYLINDRICAL_SURFACE ( 'NONE', #32646, 5.000000000000000000 ) ;
#11729=CARTESIAN_POINT ( 'NONE',  ( -1.049326080737009628E-13, -18.62499999726881583, 5.000000000000000000 ) ) ;
#11731=CARTESIAN_POINT ( 'NONE',  ( 5.000000000000000000, -157.1250000027311842, 0.000000000000000000 ) ) ;
#11741=CARTESIAN_POINT ( 'NONE',  ( -2.229367062500000163, -25.47916666530106866, -3.861377020970580443 ) ) ;
#11743=CARTESIAN_POINT ( 'NONE',  ( -2.071067811865475061, -151.6875000000000000, -5.000000000000000888 ) ) ;
#11745=CARTESIAN_POINT ( 'NONE',  ( -4.458734125000001214, -149.8750000013655779, 1.846868145590734089 ) ) ;
#11746=ORIENTED_EDGE ( 'NONE', *, *, #56301, .F. ) ;
#11747=CARTESIAN_POINT ( 'NONE',  ( 2.229367062500001939, -50.22916666530107221, 3.861377020970579999 ) ) ;
#11748=CARTESIAN_POINT ( 'NONE',  ( 2.499999999999998668, -2.333333333333333037, -4.330127018922193649 ) ) ;
#11750=CARTESIAN_POINT ( 'NONE',  ( 5.000000000000000888, 28.41666666666666430, 2.886751345948126879 ) ) ;
#11754=CARTESIAN_POINT ( 'NONE',  ( -4.458734124999999437, 4.604166668032261711, -2.574251347313719407 ) ) ;
#11755=CARTESIAN_POINT ( 'NONE',  ( -5.000000000000000000, -73.95833333060214443, -2.886751345948128211 ) ) ;
#11757=CARTESIAN_POINT ( 'NONE',  ( 0.000000000000000000, -170.0000000000000000, 0.000000000000000000 ) ) ;
#11758=CARTESIAN_POINT ( 'NONE',  ( 9.457646018065525792E-16, 15.68750000136559386, 5.148502694627439702 ) ) ;
#11759=CARTESIAN_POINT ( 'NONE',  ( -2.500000000000000444, 0.9583333360645186483, -4.330127018922193649 ) ) ;
#11760=VERTEX_POINT ( 'NONE', #44252 ) ;
#11761=CYLINDRICAL_SURFACE ( 'NONE', #55154, 5.000000000000000000 ) ;
#11764=CARTESIAN_POINT ( 'NONE',  ( 2.229367062499998831, -45.64583333196774362, -3.861377020970580887 ) ) ;
#11765=CARTESIAN_POINT ( 'NONE',  ( -1.846868145590737420, -166.0000000013656063, 4.458734124999999437 ) ) ;
#11766=EDGE_CURVE ( 'NONE', #24077, #26556, #14843, .T. ) ;
#11767=CARTESIAN_POINT ( 'NONE',  ( -3.535250795749689387E-16, -43.12499999726880162, -5.773502691896257311 ) ) ;
#11769=CARTESIAN_POINT ( 'NONE',  ( 4.458734125000001214, -18.89583333196773651, 2.574251347313718519 ) ) ;
#11771=ORIENTED_EDGE ( 'NONE', *, *, #57099, .F. ) ;
#11772=CARTESIAN_POINT ( 'NONE',  ( -2.500000000000000444, -88.16666666666665719, -4.330127018922193649 ) ) ;
#11773=CARTESIAN_POINT ( 'NONE',  ( -3.152801135295367985, -163.8125000013656063, 3.152801135295367096 ) ) ;
#11775=ORIENTED_EDGE ( 'NONE', *, *, #1126, .F. ) ;
#11777=CARTESIAN_POINT ( 'NONE',  ( -2.229367062499996610, -32.39583333196773651, 3.861377020970582219 ) ) ;
#11779=ORIENTED_EDGE ( 'NONE', *, *, #57738, .T. ) ;
#11780=( BOUNDED_CURVE ( )  B_SPLINE_CURVE ( 2, ( #39139, #53629, #44600, #20493, #34967, #14696, #9867, #560, #54582 ),
 .UNSPECIFIED., .F., .F. ) 
 B_SPLINE_CURVE_WITH_KNOTS ( ( 3, 2, 2, 2, 3 ),
 ( 0.3979166666666666963, 0.3986111111111111382, 0.4000000000000000222, 0.4013888888888889062, 0.4020833333333333481 ),
 .UNSPECIFIED. ) 
 CURVE ( )  GEOMETRIC_REPRESENTATION_ITEM ( )  RATIONAL_B_SPLINE_CURVE ( ( 0.9330127018922194093, 0.9330127018922220739, 1.000000000000000000, 0.8660254037844387076, 1.000000000000000000, 0.8660254037844387076, 1.000000000000000000, 0.9330127018922194093, 0.9330127018922194093 ) ) 
 REPRESENTATION_ITEM ( '' )  );
#11787=CARTESIAN_POINT ( 'NONE',  ( 2.229367062499998831, -81.89583333196773651, -3.861377020970580887 ) ) ;
#11789=CARTESIAN_POINT ( 'NONE',  ( 2.499999999999998668, 22.66666666666666430, -4.330127018922193649 ) ) ;
#11790=CARTESIAN_POINT ( 'NONE',  ( -4.458734124999999437, -143.2500000013655779, -1.846868145590735644 ) ) ;
#11791=CARTESIAN_POINT ( 'NONE',  ( 5.000000000000000888, -84.45833333060214443, 2.886751345948126879 ) ) ;
#11793=CARTESIAN_POINT ( 'NONE',  ( -4.458734124999999437, -45.39583333196773651, -2.574251347313719407 ) ) ;
#11797=VECTOR ( 'NONE', #10577, 1000.000000000000000 ) ;
#11798=( BOUNDED_CURVE ( )  B_SPLINE_CURVE ( 2, ( #57406, #62854, #58018, #23300, #47421, #13946, #43214, #9126, #43523 ),
 .UNSPECIFIED., .F., .F. ) 
 B_SPLINE_CURVE_WITH_KNOTS ( ( 3, 2, 2, 2, 3 ),
 ( 0.1520833333333333481, 0.1527777777777777901, 0.1541666666666666741, 0.1555555555555555580, 0.1562500000000000000 ),
 .UNSPECIFIED. ) 
 CURVE ( )  GEOMETRIC_REPRESENTATION_ITEM ( )  RATIONAL_B_SPLINE_CURVE ( ( 0.9330127018922194093, 0.9330127018922207416, 1.000000000000000000, 0.8660254037844387076, 1.000000000000000000, 0.8660254037844387076, 1.000000000000000000, 0.9330127018922194093, 0.9330127018922194093 ) ) 
 REPRESENTATION_ITEM ( '' )  );
#11799=CARTESIAN_POINT ( 'NONE',  ( 5.000000000000000000, -159.1875000027312126, 2.071067811865478614 ) ) ;
#11802=LINE ( 'NONE', #3438, #5787 ) ;
#11804=CARTESIAN_POINT ( 'NONE',  ( 9.457646018065525792E-16, -77.31249999863440792, 5.148502694627439702 ) ) ;
#11807=VERTEX_POINT ( 'NONE', #32737 ) ;
#11809=DIRECTION ( 'NONE',  ( -0.000000000000000000, 1.000000000000000000, -0.000000000000000000 ) ) ;
#11812=CARTESIAN_POINT ( 'NONE',  ( -4.458734124999999437, 12.43750000136559564, 0.000000000000000000 ) ) ;
#11813=LINE ( 'NONE', #20851, #30484 ) ;
#11818=CARTESIAN_POINT ( 'NONE',  ( 1.975475456537005874E-15, -27.74999999999999645, 5.000000000000000000 ) ) ;
#11819=CARTESIAN_POINT ( 'NONE',  ( 4.458734125000001214, -83.89583333196773651, 2.574251347313718519 ) ) ;
#11820=CARTESIAN_POINT ( 'NONE',  ( -2.229367062500000163, -5.479166665301072214, -3.861377020970580443 ) ) ;
#11823=CARTESIAN_POINT ( 'NONE',  ( -4.458734124999999437, -36.64583333196773651, -2.574251347313719407 ) ) ;
#11827=CARTESIAN_POINT ( 'NONE',  ( -4.458734124999999437, 21.68750000136559208, 0.000000000000000000 ) ) ;
#11831=CARTESIAN_POINT ( 'NONE',  ( -9.184850993605147944E-16, -145.3750000027312126, 5.000000000000000000 ) ) ;
#11832=CARTESIAN_POINT ( 'NONE',  ( -2.229367062499996610, -78.39583333196773651, 3.861377020970582219 ) ) ;
#11834=ADVANCED_FACE ( 'NONE', ( #56564 ), #42066, .T. ) ;
#11836=CARTESIAN_POINT ( 'NONE',  ( -2.499999999999996447, 20.29166666939784847, 4.330127018922195425 ) ) ;
#11837=ORIENTED_EDGE ( 'NONE', *, *, #62117, .F. ) ;
#11840=CARTESIAN_POINT ( 'NONE',  ( -5.000000000000000888, -149.5625000000000568, -2.071067811865475949 ) ) ;
#11841=CARTESIAN_POINT ( 'NONE',  ( 5.000000000000000000, -24.50000000000000000, -6.123233995736766282E-16 ) ) ;
#11842=CARTESIAN_POINT ( 'NONE',  ( -4.458734124999998549, -25.22916666530106866, 2.574251347313722516 ) ) ;
#11843=CARTESIAN_POINT ( 'NONE',  ( 4.458734124999998549, -88.72916666530106511, -2.574251347313721627 ) ) ;
#11845=CARTESIAN_POINT ( 'NONE',  ( -5.000000000000000000, -25.95833333060214798, -2.886751345948128211 ) ) ;
#11846=CARTESIAN_POINT ( 'NONE',  ( -2.229367062500000163, -54.47916666530107221, -3.861377020970580443 ) ) ;
#11849=EDGE_CURVE ( 'NONE', #62091, #33038, #37043, .T. ) ;
#11850=CARTESIAN_POINT ( 'NONE',  ( -2.229367062500000163, -3.729166665301070438, -3.861377020970580443 ) ) ;
#11852=CARTESIAN_POINT ( 'NONE',  ( -2.499999999999996447, -72.83333333333332860, 4.330127018922195425 ) ) ;
#11856=( BOUNDED_CURVE ( )  B_SPLINE_CURVE ( 2, ( #3768, #47200, #51713, #3144, #33035, #23069, #52651, #46884, #8586 ),
 .UNSPECIFIED., .F., .F. ) 
 B_SPLINE_CURVE_WITH_KNOTS ( ( 3, 2, 2, 2, 3 ),
 ( 0.5750000000000005107, 0.5791666666666672736, 0.5833333333333339255, 0.5875000000000004663, 0.5916666666666671182 ),
 .UNSPECIFIED. ) 
 CURVE ( )  GEOMETRIC_REPRESENTATION_ITEM ( )  RATIONAL_B_SPLINE_CURVE ( ( 0.9999999999999898970, 0.9238795325112968415, 1.000000000000000000, 0.9238795325112867385, 1.000000000000000000, 0.9238795325112867385, 1.000000000000000000, 0.9238795325112786339, 1.000000000000008216 ) ) 
 REPRESENTATION_ITEM ( '' )  );
#11858=CARTESIAN_POINT ( 'NONE',  ( -3.535250795749689387E-16, -69.12499999726880162, -5.773502691896257311 ) ) ;
#11861=CARTESIAN_POINT ( 'NONE',  ( 2.229367062499998831, -15.89583333196773651, -3.861377020970580887 ) ) ;
#11862=CARTESIAN_POINT ( 'NONE',  ( 2.229367062500001939, -51.22916666530107221, 3.861377020970579999 ) ) ;
#11864=CARTESIAN_POINT ( 'NONE',  ( 3.152801135295367541, -142.3125000013655779, -3.152801135295367541 ) ) ;
#11866=CARTESIAN_POINT ( 'NONE',  ( 5.000000000000000000, -8.291666663935481907, -2.886751345948130876 ) ) ;
#11869=CARTESIAN_POINT ( 'NONE',  ( 2.229367062499998831, 24.10416666803225993, -3.861377020970580887 ) ) ;
#11874=CARTESIAN_POINT ( 'NONE',  ( 4.458734124999999437, -148.6875000013656063, 0.000000000000000000 ) ) ;
#11876=CARTESIAN_POINT ( 'NONE',  ( 2.229367062500001939, -63.22916666530106511, 3.861377020970579999 ) ) ;
#11877=CARTESIAN_POINT ( 'NONE',  ( -1.339745962155610925, -83.66965819600733312, 5.000000000000000000 ) ) ;
#11878=CARTESIAN_POINT ( 'NONE',  ( -2.229367062500000163, -9.479166665301068662, -3.861377020970580443 ) ) ;
#11880=CARTESIAN_POINT ( 'NONE',  ( -4.458734125000000326, -146.8750000013656063, 1.846868145590734089 ) ) ;
#11888=CARTESIAN_POINT ( 'NONE',  ( 2.229367062500001939, 25.77083333469892779, 3.861377020970579999 ) ) ;
#11889=CARTESIAN_POINT ( 'NONE',  ( -6.972266317189433020E-16, 1.875000002731185722, -5.000000000000000000 ) ) ;
#11890=AXIS2_PLACEMENT_3D ( 'NONE', #18294, #37917, #46305 ) ;
#11898=CARTESIAN_POINT ( 'NONE',  ( -2.229367062500000163, 11.52083333469892601, -3.861377020970580443 ) ) ;
#11900=CARTESIAN_POINT ( 'NONE',  ( 4.458734125000000326, -16.14583333196773651, 2.574251347313718519 ) ) ;
#11901=( BOUNDED_CURVE ( )  B_SPLINE_CURVE ( 2, ( #28896, #34678, #19880, #14102, #28582, #58801, #39176, #9281, #14732 ),
 .UNSPECIFIED., .F., .F. ) 
 B_SPLINE_CURVE_WITH_KNOTS ( ( 3, 2, 2, 2, 3 ),
 ( 0.4020833333333333481, 0.4027777777777777901, 0.4041666666666666741, 0.4055555555555555580, 0.4062500000000000000 ),
 .UNSPECIFIED. ) 
 CURVE ( )  GEOMETRIC_REPRESENTATION_ITEM ( )  RATIONAL_B_SPLINE_CURVE ( ( 0.9330127018922194093, 0.9330127018922194093, 1.000000000000000000, 0.8660254037844387076, 1.000000000000000000, 0.8660254037844387076, 1.000000000000000000, 0.9330127018922194093, 0.9330127018922194093 ) ) 
 REPRESENTATION_ITEM ( '' )  );
#11903=CARTESIAN_POINT ( 'NONE',  ( -8.190561711645485556E-16, -159.6875000013655779, 4.458734124999999437 ) ) ;
#11907=CARTESIAN_POINT ( 'NONE',  ( -5.000000000000000000, 9.999999999999998224, 0.000000000000000000 ) ) ;
#11909=CARTESIAN_POINT ( 'NONE',  ( 4.458734125000000326, -37.89583333196773651, 2.574251347313718519 ) ) ;
#11911=DIRECTION ( 'NONE',  ( -0.000000000000000000, 1.000000000000000000, -0.000000000000000000 ) ) ;
#11914=DIRECTION ( 'NONE',  ( -0.000000000000000000, 1.000000000000000000, -0.000000000000000000 ) ) ;
#11915=VERTEX_POINT ( 'NONE', #18576 ) ;
#11918=CARTESIAN_POINT ( 'NONE',  ( -2.499999999999996447, -6.833333333333330373, 4.330127018922195425 ) ) ;
#11919=CARTESIAN_POINT ( 'NONE',  ( -4.458734124999999437, -74.39583333196775072, -2.574251347313719407 ) ) ;
#11920=FACE_OUTER_BOUND ( 'NONE', #44522, .T. ) ;
#11921=CARTESIAN_POINT ( 'NONE',  ( 5.000000000000000888, -9.458333330602144429, 2.886751345948126879 ) ) ;
#11922=CARTESIAN_POINT ( 'NONE',  ( 2.229367062499998831, -37.64583333196773651, -3.861377020970580887 ) ) ;
#11924=CARTESIAN_POINT ( 'NONE',  ( -4.458734124999999437, 13.35416666803225993, -2.574251347313719407 ) ) ;
#11927=CARTESIAN_POINT ( 'NONE',  ( 1.060575238724906964E-15, -53.74999999999998579, 5.773502691896257311 ) ) ;
#11928=ADVANCED_FACE ( 'NONE', ( #13744 ), #46588, .T. ) ;
#11929=CARTESIAN_POINT ( 'NONE',  ( -1.846868145590737420, -162.0000000013655779, 4.458734124999999437 ) ) ;
#11932=CARTESIAN_POINT ( 'NONE',  ( 9.457646018065525792E-16, -73.06249999863440792, 5.148502694627439702 ) ) ;
#11933=VECTOR ( 'NONE', #46910, 1000.000000000000000 ) ;
#11934=CARTESIAN_POINT ( 'NONE',  ( -5.000000000000000000, -168.5000000000000000, -6.123233995736766282E-16 ) ) ;
#11936=CARTESIAN_POINT ( 'NONE',  ( -4.458734124999999437, -88.39583333196773651, -2.574251347313719407 ) ) ;
#11940=CARTESIAN_POINT ( 'NONE',  ( -4.458734124999999437, -33.56249999863440792, 0.000000000000000000 ) ) ;
#11945=VERTEX_POINT ( 'NONE', #5041 ) ;
#11948=CARTESIAN_POINT ( 'NONE',  ( -2.229367062499996610, -66.39583333196773651, 3.861377020970582219 ) ) ;
#11953=VERTEX_POINT ( 'NONE', #43322 ) ;
#11956=CARTESIAN_POINT ( 'NONE',  ( 2.229367062499998831, 10.35416666803225993, -3.861377020970580887 ) ) ;
#11957=CARTESIAN_POINT ( 'NONE',  ( 0.000000000000000000, -170.0000000000000000, 0.000000000000000000 ) ) ;
#11958=CARTESIAN_POINT ( 'NONE',  ( -3.152801135295367985, -155.8125000013656063, 3.152801135295367096 ) ) ;
#11959=LINE ( 'NONE', #25813, #35820 ) ;
#11966=CARTESIAN_POINT ( 'NONE',  ( 1.339745962155615144, -78.70534180126148271, 4.999999999999999112 ) ) ;
#11969=CARTESIAN_POINT ( 'NONE',  ( 2.499999999999998668, -82.20833333060214443, -4.330127018922193649 ) ) ;
#11972=CARTESIAN_POINT ( 'NONE',  ( 4.458734125000000326, 0.8541666680322613781, 2.574251347313718519 ) ) ;
#11973=AXIS2_PLACEMENT_3D ( 'NONE', #52493, #33182, #61517 ) ;
#11976=CARTESIAN_POINT ( 'NONE',  ( 2.071067811865476394, -146.3125000027312410, 5.000000000000000000 ) ) ;
#11980=VECTOR ( 'NONE', #36781, 1000.000000000000000 ) ;
#11984=EDGE_CURVE ( 'NONE', #39875, #56335, #39125, .T. ) ;
#11987=CARTESIAN_POINT ( 'NONE',  ( 1.846868145590736310, -159.8750000013655779, 4.458734124999997661 ) ) ;
#11990=CARTESIAN_POINT ( 'NONE',  ( -2.499999999999996447, -90.70833333060214443, 4.330127018922195425 ) ) ;
#11992=CARTESIAN_POINT ( 'NONE',  ( -2.229367062499996610, 23.60416666803225993, 3.861377020970582219 ) ) ;
#11998=CARTESIAN_POINT ( 'NONE',  ( 5.000000000000000888, 9.416666666666666075, 2.886751345948126879 ) ) ;
#11999=CARTESIAN_POINT ( 'NONE',  ( 9.457646018065525792E-16, -56.06249999863440792, 5.148502694627439702 ) ) ;
#12002=DIRECTION ( 'NONE',  ( -0.000000000000000000, 1.000000000000000000, -0.000000000000000000 ) ) ;
#12005=CARTESIAN_POINT ( 'NONE',  ( 2.500000000000002220, -41.66666666666667140, 4.330127018922192761 ) ) ;
#12007=CARTESIAN_POINT ( 'NONE',  ( -1.339745962155610925, -44.79465819873851018, 5.000000000000000000 ) ) ;
#12010=CARTESIAN_POINT ( 'NONE',  ( -4.458734124999998549, -62.22916666530106511, 2.574251347313722516 ) ) ;
#12011=CARTESIAN_POINT ( 'NONE',  ( 1.846868145590735200, -151.5000000013655779, -4.458734125000000326 ) ) ;
#12012=CARTESIAN_POINT ( 'NONE',  ( 2.229367062499998831, -69.64583333196773651, -3.861377020970580887 ) ) ;
#12014=CARTESIAN_POINT ( 'NONE',  ( 4.458734124999999437, -18.06249999863440792, -5.460374474430324690E-16 ) ) ;
#12015=CARTESIAN_POINT ( 'NONE',  ( 5.000000000000000000, -63.37499999726880873, -6.123233995736766282E-16 ) ) ;
#12017=CARTESIAN_POINT ( 'NONE',  ( -5.000000000000000888, -150.5625000000000284, -2.071067811865475949 ) ) ;
#12022=CARTESIAN_POINT ( 'NONE',  ( -3.152801135295367985, -153.8125000013656063, 3.152801135295367096 ) ) ;
#12023=ORIENTED_EDGE ( 'NONE', *, *, #35372, .F. ) ;
#12024=AXIS2_PLACEMENT_3D ( 'NONE', #52735, #17384, #32156 ) ;
#12025=CARTESIAN_POINT ( 'NONE',  ( 5.000000000000000000, 25.58333333333333215, -2.886751345948130876 ) ) ;
#12028=CARTESIAN_POINT ( 'NONE',  ( -4.458734124999999437, -46.56249999863440792, 0.000000000000000000 ) ) ;
#12030=AXIS2_PLACEMENT_3D ( 'NONE', #21556, #15770, #55006 ) ;
#12031=CARTESIAN_POINT ( 'NONE',  ( -5.000000000000000000, 17.04166666939785202, -2.886751345948128211 ) ) ;
#12035=CARTESIAN_POINT ( 'NONE',  ( -4.458734124999998549, 25.77083333469892779, 2.574251347313722516 ) ) ;
#12038=CARTESIAN_POINT ( 'NONE',  ( 1.846868145590735200, -167.2500000013655779, -4.458734124999999437 ) ) ;
#12043=ADVANCED_FACE ( 'NONE', ( #58751 ), #14680, .T. ) ;
#12049=CARTESIAN_POINT ( 'NONE',  ( 3.061616997868383141E-16, -139.8750000027312126, -5.000000000000000000 ) ) ;
#12055=CARTESIAN_POINT ( 'NONE',  ( 5.000000000000000888, -159.0625000027312126, -2.071067811865475505 ) ) ;
#12061=CARTESIAN_POINT ( 'NONE',  ( -5.000000000000000888, -147.4375000000000000, 2.071067811865474617 ) ) ;
#12065=CARTESIAN_POINT ( 'NONE',  ( -3.152548672688508926E-16, -27.56249999863440081, -5.148502694627439702 ) ) ;
#12066=CARTESIAN_POINT ( 'NONE',  ( -6.972266317189433020E-16, 14.74999999999999822, -5.000000000000000000 ) ) ;
#12067=CARTESIAN_POINT ( 'NONE',  ( 5.000000000000000000, -151.0625000000000000, 2.071067811865478614 ) ) ;
#12069=CARTESIAN_POINT ( 'NONE',  ( -4.458734125000001214, -150.8750000013655779, 1.846868145590734089 ) ) ;
#12071=CARTESIAN_POINT ( 'NONE',  ( 5.000000000000000888, -149.9375000000000000, -2.071067811865475505 ) ) ;
#12072=CARTESIAN_POINT ( 'NONE',  ( 4.458734124999998549, -48.97916666530107221, -2.574251347313721627 ) ) ;
#12073=AXIS2_PLACEMENT_3D ( 'NONE', #11957, #1701, #7155 ) ;
#12076=CARTESIAN_POINT ( 'NONE',  ( -2.499999999999996447, 25.16666666666666430, 4.330127018922195425 ) ) ;
#12077=AXIS2_PLACEMENT_3D ( 'NONE', #31454, #55289, #16361 ) ;
#12080=CARTESIAN_POINT ( 'NONE',  ( -4.458734124999998549, 5.770833334698927786, 2.574251347313722516 ) ) ;
#12081=CARTESIAN_POINT ( 'NONE',  ( 1.339745962155612702, 19.70534180126147561, -5.000000000000000000 ) ) ;
#12082=CARTESIAN_POINT ( 'NONE',  ( 5.000000000000000000, -41.29166666393548013, -2.886751345948130876 ) ) ;
#12083=CARTESIAN_POINT ( 'NONE',  ( 5.000000000000000000, -7.416666666666667851, -2.886751345948130876 ) ) ;
#12084=CARTESIAN_POINT ( 'NONE',  ( -2.229367062500000163, 16.27083333469892779, -3.861377020970580443 ) ) ;
#12085=CARTESIAN_POINT ( 'NONE',  ( 2.500000000000002220, 4.458333336064518093, 4.330127018922192761 ) ) ;
#12090=CARTESIAN_POINT ( 'NONE',  ( -2.499999999999996447, -70.83333333333332860, 4.330127018922195425 ) ) ;
#12091=CARTESIAN_POINT ( 'NONE',  ( 4.458734125000001214, -41.89583333196773651, 2.574251347313718519 ) ) ;
#12092=CARTESIAN_POINT ( 'NONE',  ( 1.846868145590735200, -164.5000000013655779, -4.458734125000000326 ) ) ;
#12093=CARTESIAN_POINT ( 'NONE',  ( 5.000000000000000888, -42.45833333060214443, 2.886751345948126879 ) ) ;
#12094=ORIENTED_EDGE ( 'NONE', *, *, #33473, .F. ) ;
#12095=CARTESIAN_POINT ( 'NONE',  ( -3.152548672688508926E-16, -19.56249999863440081, -5.148502694627439702 ) ) ;
#12097=CARTESIAN_POINT ( 'NONE',  ( -5.000000000000000000, -90.00000000000000000, 0.000000000000000000 ) ) ;
#12098=CARTESIAN_POINT ( 'NONE',  ( 1.846868145590735200, -163.2500000013655495, -4.458734125000000326 ) ) ;
#12099=CARTESIAN_POINT ( 'NONE',  ( -5.000000000000000000, -60.87499999726880873, 0.000000000000000000 ) ) ;
#12102=CARTESIAN_POINT ( 'NONE',  ( 2.229367062500001939, -30.22916666530107221, 3.861377020970579999 ) ) ;
#12103=ORIENTED_EDGE ( 'NONE', *, *, #748, .F. ) ;
#12106=CARTESIAN_POINT ( 'NONE',  ( -4.999999999999998224, -28.79166666393548013, 2.886751345948131764 ) ) ;
#12107=EDGE_LOOP ( 'NONE', ( #13612, #5695, #61672, #29094 ) ) ;
#12110=CARTESIAN_POINT ( 'NONE',  ( -2.229367062500000163, -79.72916666530106511, -3.861377020970580443 ) ) ;
#12113=CARTESIAN_POINT ( 'NONE',  ( 3.152801135295366208, -143.8125000013655779, 3.152801135295367985 ) ) ;
#12115=CARTESIAN_POINT ( 'NONE',  ( 1.339745962155615144, 20.29465819873851729, 4.999999999999999112 ) ) ;
#12117=CARTESIAN_POINT ( 'NONE',  ( -4.458734124999999437, -47.39583333196774362, -2.574251347313719407 ) ) ;
#12122=CARTESIAN_POINT ( 'NONE',  ( 5.000000000000000000, -3.416666666666665186, -2.886751345948130876 ) ) ;
#12125=CARTESIAN_POINT ( 'NONE',  ( -1.339745962155610925, -72.79465819873850307, 5.000000000000000000 ) ) ;
#12127=CARTESIAN_POINT ( 'NONE',  ( -2.229367062499996610, -77.39583333196773651, 3.861377020970582219 ) ) ;
#12132=CARTESIAN_POINT ( 'NONE',  ( 1.975475456537005874E-15, -77.62499999726881583, 5.000000000000000000 ) ) ;
#12133=CARTESIAN_POINT ( 'NONE',  ( -6.972266317189433020E-16, -47.24999999999999289, -5.000000000000000000 ) ) ;
#12135=CARTESIAN_POINT ( 'NONE',  ( -9.184850993605147944E-16, -168.3750000027312126, 5.000000000000000000 ) ) ;
#12137=CARTESIAN_POINT ( 'NONE',  ( 4.458734124999998549, 10.02083333469892779, -2.574251347313721627 ) ) ;
#12138=CARTESIAN_POINT ( 'NONE',  ( 1.975475456537005874E-15, -15.75000000000000000, 5.000000000000000000 ) ) ;
#12141=EDGE_CURVE ( 'NONE', #12417, #54676, #28381, .T. ) ;
#12147=CARTESIAN_POINT ( 'NONE',  ( -4.458734124999999437, -86.31249999863439371, 0.000000000000000000 ) ) ;
#12148=CARTESIAN_POINT ( 'NONE',  ( -2.229367062500000163, -8.479166665301073991, -3.861377020970580443 ) ) ;
#12150=ORIENTED_EDGE ( 'NONE', *, *, #6001, .T. ) ;
#12151=CARTESIAN_POINT ( 'NONE',  ( 4.458734124999998549, -34.97916666530107221, -2.574251347313721627 ) ) ;
#12155=ADVANCED_FACE ( 'NONE', ( #38803 ), #58442, .T. ) ;
#12156=CARTESIAN_POINT ( 'NONE',  ( 4.458734124999999437, -149.6250000013655779, -1.846868145590734978 ) ) ;
#12157=CARTESIAN_POINT ( 'NONE',  ( 2.229367062499998831, 22.35416666803225993, -3.861377020970580887 ) ) ;
#12158=CARTESIAN_POINT ( 'NONE',  ( 1.975475456537005874E-15, -53.74999999999999289, 5.000000000000000000 ) ) ;
#12159=CARTESIAN_POINT ( 'NONE',  ( -3.535533905932738641, -145.5000000027311842, 3.535533905932737309 ) ) ;
#12160=CARTESIAN_POINT ( 'NONE',  ( -3.152548672688508926E-16, -84.81249999863439371, -5.148502694627439702 ) ) ;
#12162=CARTESIAN_POINT ( 'NONE',  ( 5.000000000000000888, -72.45833333060213022, 2.886751345948126879 ) ) ;
#12163=CARTESIAN_POINT ( 'NONE',  ( -4.999999999999999112, 17.20833333606451987, 2.886751345948131764 ) ) ;
#12164=VERTEX_POINT ( 'NONE', #48154 ) ;
#12166=AXIS2_PLACEMENT_3D ( 'NONE', #9106, #54442, #53482 ) ;
#12169=CARTESIAN_POINT ( 'NONE',  ( 2.499999999999998668, -21.33333333333333570, -4.330127018922193649 ) ) ;
#12170=CARTESIAN_POINT ( 'NONE',  ( -3.152548672688508926E-16, -29.56249999863440436, -5.148502694627439702 ) ) ;
#12172=CARTESIAN_POINT ( 'NONE',  ( 2.229367062499998831, -85.64583333196773651, -3.861377020970580887 ) ) ;
#12174=CARTESIAN_POINT ( 'NONE',  ( -5.000000000000000000, -30.95833333060214443, -2.886751345948128211 ) ) ;
#12175=ADVANCED_FACE ( 'NONE', ( #33992 ), #53613, .T. ) ;
#12176=CARTESIAN_POINT ( 'NONE',  ( -2.229367062499996610, -54.14583333196773651, 3.861377020970582219 ) ) ;
#12178=DIRECTION ( 'NONE',  ( -0.000000000000000000, 1.000000000000000000, -0.000000000000000000 ) ) ;
#12180=CARTESIAN_POINT ( 'NONE',  ( -3.152548672688508926E-16, -5.812499998634404363, -5.148502694627439702 ) ) ;
#12181=VERTEX_POINT ( 'NONE', #4717 ) ;
#12182=CARTESIAN_POINT ( 'NONE',  ( -2.499999999999996447, -73.83333333333332860, 4.330127018922195425 ) ) ;
#12186=CARTESIAN_POINT ( 'NONE',  ( -2.499999999999996447, -75.70833333060214443, 4.330127018922195425 ) ) ;
#12187=CARTESIAN_POINT ( 'NONE',  ( 1.975475456537005874E-15, -53.62499999726880162, 5.000000000000000000 ) ) ;
#12189=CARTESIAN_POINT ( 'NONE',  ( -2.229367062499996610, -18.39583333196774007, 3.861377020970582219 ) ) ;
#12190=CARTESIAN_POINT ( 'NONE',  ( 4.458734124999999437, -50.06249999863440792, -5.460374474430324690E-16 ) ) ;
#12193=CARTESIAN_POINT ( 'NONE',  ( -3.152801135295367985, -140.8125000013655779, 3.152801135295367096 ) ) ;
#12195=ORIENTED_EDGE ( 'NONE', *, *, #15269, .T. ) ;
#12198=CARTESIAN_POINT ( 'NONE',  ( -6.972266317189433020E-16, 18.74999999999999645, -5.000000000000000000 ) ) ;
#12204=CARTESIAN_POINT ( 'NONE',  ( -4.458734125000001214, -147.1250000013656063, 1.846868145590734089 ) ) ;
#12208=CARTESIAN_POINT ( 'NONE',  ( 2.229367062499998831, -60.89583333196774362, -3.861377020970580887 ) ) ;
#12209=CARTESIAN_POINT ( 'NONE',  ( 1.975475456537005874E-15, -83.62499999726878741, 5.000000000000000000 ) ) ;
#12211=CARTESIAN_POINT ( 'NONE',  ( 3.152801135295366208, -143.5625000013655779, 3.152801135295367985 ) ) ;
#12216=CARTESIAN_POINT ( 'NONE',  ( -3.535533905932738641, -144.3750000000000000, 3.535533905932737309 ) ) ;
#12219=AXIS2_PLACEMENT_3D ( 'NONE', #37660, #29251, #53085 ) ;
#12220=CYLINDRICAL_SURFACE ( 'NONE', #62235, 5.000000000000000000 ) ;
#12221=ADVANCED_FACE ( 'NONE', ( #1198 ), #25619, .T. ) ;
#12227=CARTESIAN_POINT ( 'NONE',  ( 2.500000000000002220, -56.54166666393548013, 4.330127018922192761 ) ) ;
#12229=CARTESIAN_POINT ( 'NONE',  ( 1.339745962155602488, 21.29465819873852084, 5.000000000000007105 ) ) ;
#12230=CARTESIAN_POINT ( 'NONE',  ( -4.458734124999999437, 7.687500001365594748, 0.000000000000000000 ) ) ;
#12232=CARTESIAN_POINT ( 'NONE',  ( 2.229367062499998831, -20.89583333196774007, -3.861377020970580887 ) ) ;
#12234=CARTESIAN_POINT ( 'NONE',  ( -1.846868145590734756, -161.1250000013656063, -4.458734125000000326 ) ) ;
#12235=CARTESIAN_POINT ( 'NONE',  ( 1.975475456537005874E-15, -85.75000000000000000, 5.000000000000000000 ) ) ;
#12238=VECTOR ( 'NONE', #9138, 1000.000000000000000 ) ;
#12240=CARTESIAN_POINT ( 'NONE',  ( 4.458734124999998549, -35.72916666530107221, -2.574251347313721627 ) ) ;
#12241=CARTESIAN_POINT ( 'NONE',  ( 5.000000000000000000, -51.29166666393547303, -2.886751345948130876 ) ) ;
#12242=CARTESIAN_POINT ( 'NONE',  ( -3.152548672688508926E-16, -65.81249999863440792, -5.148502694627439702 ) ) ;
#12244=CARTESIAN_POINT ( 'NONE',  ( -6.972266317189433020E-16, -41.24999999999998579, -5.000000000000000000 ) ) ;
#12246=VERTEX_POINT ( 'NONE', #31071 ) ;
#12250=CARTESIAN_POINT ( 'NONE',  ( 1.060575238724906964E-15, -9.750000000000001776, 5.773502691896257311 ) ) ;
#12251=CARTESIAN_POINT ( 'NONE',  ( 4.458734124999999437, -69.81249999863439371, -5.460374474430324690E-16 ) ) ;
#12253=CARTESIAN_POINT ( 'NONE',  ( 1.060575238724906964E-15, -11.62499999726881761, 5.773502691896257311 ) ) ;
#12254=CARTESIAN_POINT ( 'NONE',  ( 2.229367062500001939, -40.97916666530107221, 3.861377020970579999 ) ) ;
#12256=CARTESIAN_POINT ( 'NONE',  ( -5.000000000000000000, 29.91666666666666430, -2.886751345948128211 ) ) ;
#12257=CARTESIAN_POINT ( 'NONE',  ( -2.229367062500000163, 11.27083333469892601, -3.861377020970580443 ) ) ;
#12260=CARTESIAN_POINT ( 'NONE',  ( -5.000000000000000000, -54.99999999999999289, 0.000000000000000000 ) ) ;
#12261=CARTESIAN_POINT ( 'NONE',  ( 4.458734124999999437, -161.7500000013655495, 1.846868145590737864 ) ) ;
#12264=CARTESIAN_POINT ( 'NONE',  ( -5.000000000000000000, -35.00000000000000000, 0.000000000000000000 ) ) ;
#12265=CARTESIAN_POINT ( 'NONE',  ( -2.229367062500000163, -78.47916666530106511, -3.861377020970580443 ) ) ;
#12266=CARTESIAN_POINT ( 'NONE',  ( -5.000000000000000888, -169.4375000000000284, 2.071067811865474617 ) ) ;
#12267=CARTESIAN_POINT ( 'NONE',  ( 9.457646018065525792E-16, -86.06249999863439371, 5.148502694627439702 ) ) ;
#12270=CARTESIAN_POINT ( 'NONE',  ( 2.229367062500001939, -0.2291666653010705768, 3.861377020970579999 ) ) ;
#12271=CARTESIAN_POINT ( 'NONE',  ( -4.458734124999998549, -36.47916666530107221, 2.574251347313722516 ) ) ;
#12272=CARTESIAN_POINT ( 'NONE',  ( 1.339745962155615144, -16.58034179853029499, 4.999999999999999112 ) ) ;
#12277=CARTESIAN_POINT ( 'NONE',  ( 3.535533905932738197, -151.8750000000000000, -3.535533905932738197 ) ) ;
#12278=CARTESIAN_POINT ( 'NONE',  ( -4.458734124999998549, -71.47916666530107932, 2.574251347313722516 ) ) ;
#12281=LINE ( 'NONE', #62126, #16356 ) ;
#12286=CARTESIAN_POINT ( 'NONE',  ( -4.458734124999999437, 7.604166668032259935, -2.574251347313719407 ) ) ;
#12287=CARTESIAN_POINT ( 'NONE',  ( 1.975475456537005874E-15, -75.74999999999998579, 5.000000000000000000 ) ) ;
#12288=CARTESIAN_POINT ( 'NONE',  ( 1.846868145590736310, -156.6250000013655779, 4.458734124999997661 ) ) ;
#12301=CARTESIAN_POINT ( 'NONE',  ( 2.500000000000002220, -82.54166666393547303, 4.330127018922192761 ) ) ;
#12302=EDGE_CURVE ( 'NONE', #7607, #24077, #54688, .T. ) ;
#12305=CARTESIAN_POINT ( 'NONE',  ( 4.458734124999998549, -0.9791666653010712151, -2.574251347313721627 ) ) ;
#12307=CARTESIAN_POINT ( 'NONE',  ( 5.000000000000000888, -160.0625000027312410, -2.071067811865475505 ) ) ;
#12310=CARTESIAN_POINT ( 'NONE',  ( -3.535533905932737309, -141.7500000027311842, -3.535533905932738197 ) ) ;
#12311=LINE ( 'NONE', #16496, #38727 ) ;
#12316=DIRECTION ( 'NONE',  ( 0.000000000000000000, 0.000000000000000000, 1.000000000000000000 ) ) ;
#12317=EDGE_CURVE ( 'NONE', #40520, #49284, #4165, .T. ) ;
#12318=CARTESIAN_POINT ( 'NONE',  ( -2.499999999999996447, -87.83333333333332860, 4.330127018922195425 ) ) ;
#12320=CARTESIAN_POINT ( 'NONE',  ( 3.152801135295366208, -159.8125000013656063, 3.152801135295367985 ) ) ;
#12322=CARTESIAN_POINT ( 'NONE',  ( -3.152801135295367985, -141.8125000013655779, 3.152801135295367096 ) ) ;
#12324=CARTESIAN_POINT ( 'NONE',  ( -4.458734124999998549, 19.52083333469893134, 2.574251347313722516 ) ) ;
#12329=CARTESIAN_POINT ( 'NONE',  ( 5.000000000000000000, -16.41666666666667140, -2.886751345948130876 ) ) ;
#12330=CARTESIAN_POINT ( 'NONE',  ( 2.500000000000002220, 9.333333333333332149, 4.330127018922192761 ) ) ;
#12331=CARTESIAN_POINT ( 'NONE',  ( -3.152548672688508926E-16, -54.56249999863439371, -5.148502694627439702 ) ) ;
#12336=CARTESIAN_POINT ( 'NONE',  ( -4.999999999999998224, -24.79166666393548368, 2.886751345948131764 ) ) ;
#12337=CARTESIAN_POINT ( 'NONE',  ( 2.499999999999998668, -38.33333333333332860, -4.330127018922193649 ) ) ;
#12341=CARTESIAN_POINT ( 'NONE',  ( 4.458734124999998549, -66.72916666530106511, -2.574251347313721627 ) ) ;
#12342=CARTESIAN_POINT ( 'NONE',  ( -3.152801135295367096, -152.3125000013655779, -3.152801135295367541 ) ) ;
#12343=CARTESIAN_POINT ( 'NONE',  ( -4.458734124999998549, -69.22916666530107932, 2.574251347313722516 ) ) ;
#12345=CARTESIAN_POINT ( 'NONE',  ( -4.458734124999998549, -19.47916666530107221, 2.574251347313722516 ) ) ;
#12346=CARTESIAN_POINT ( 'NONE',  ( -2.500000000000000444, -60.04166666393547303, -4.330127018922193649 ) ) ;
#12349=ORIENTED_EDGE ( 'NONE', *, *, #36892, .F. ) ;
#12351=CARTESIAN_POINT ( 'NONE',  ( 2.071067811865349828, -149.3125000027311842, 5.000000000000126121 ) ) ;
#12352=CARTESIAN_POINT ( 'NONE',  ( -3.152801135295367985, -151.8125000013655779, 3.152801135295367096 ) ) ;
#12357=CARTESIAN_POINT ( 'NONE',  ( 2.229367062499998831, -50.89583333196772941, -3.861377020970580887 ) ) ;
#12358=ORIENTED_EDGE ( 'NONE', *, *, #25126, .F. ) ;
#12359=AXIS2_PLACEMENT_3D ( 'NONE', #38319, #13868, #33491 ) ;
#12361=CARTESIAN_POINT ( 'NONE',  ( -4.458734124999999437, 25.60416666803225993, -2.574251347313719407 ) ) ;
#12364=CARTESIAN_POINT ( 'NONE',  ( 1.846868145590735200, -169.2500000013655779, -4.458734124999999437 ) ) ;
#12367=CARTESIAN_POINT ( 'NONE',  ( 3.061616997868383141E-16, -148.8750000027312126, -5.000000000000000000 ) ) ;
#12370=( BOUNDED_CURVE ( )  B_SPLINE_CURVE ( 2, ( #60625, #15266, #1139, #24920, #1454, #35851, #10119, #40017, #15594 ),
 .UNSPECIFIED., .F., .F. ) 
 B_SPLINE_CURVE_WITH_KNOTS ( ( 3, 2, 2, 2, 3 ),
 ( 0.2583333333333335813, 0.2625000000000002331, 0.2666666666666668850, 0.2708333333333335369, 0.2750000000000002442 ),
 .UNSPECIFIED. ) 
 CURVE ( )  GEOMETRIC_REPRESENTATION_ITEM ( )  RATIONAL_B_SPLINE_CURVE ( ( 0.9999999999999958922, 0.9238795325112908463, 1.000000000000000000, 0.9238795325112867385, 1.000000000000000000, 0.9238795325112867385, 1.000000000000000000, 0.9238795325112826307, 1.000000000000003997 ) ) 
 REPRESENTATION_ITEM ( '' )  );
#12371=LINE ( 'NONE', #28196, #17224 ) ;
#12375=CARTESIAN_POINT ( 'NONE',  ( 5.000000000000000888, -160.9375000000000000, -2.071067811865475505 ) ) ;
#12376=CARTESIAN_POINT ( 'NONE',  ( 1.975475456537005874E-15, -38.75000000000000000, 5.000000000000000000 ) ) ;
#12380=CARTESIAN_POINT ( 'NONE',  ( -6.972266317189433020E-16, 17.87500000273118417, -5.000000000000000000 ) ) ;
#12382=CARTESIAN_POINT ( 'NONE',  ( 2.071067811865476394, -155.3125000027311842, 5.000000000000000000 ) ) ;
#12388=CARTESIAN_POINT ( 'NONE',  ( 5.000000000000000000, -146.0000000000000284, 0.000000000000000000 ) ) ;
#12392=CARTESIAN_POINT ( 'NONE',  ( -2.229367062500000163, -22.47916666530107221, -3.861377020970580443 ) ) ;
#12395=CARTESIAN_POINT ( 'NONE',  ( 4.458734124999999437, -153.5000000013656063, 1.846868145590737864 ) ) ;
#12398=CARTESIAN_POINT ( 'NONE',  ( 2.071067811865349828, -150.1875000000000284, 5.000000000000126121 ) ) ;
#12399=CARTESIAN_POINT ( 'NONE',  ( 9.457646018065525792E-16, -53.31249999863440792, 5.148502694627439702 ) ) ;
#12400=CARTESIAN_POINT ( 'NONE',  ( 2.500000000000002220, -58.54166666393548013, 4.330127018922192761 ) ) ;
#12402=CARTESIAN_POINT ( 'NONE',  ( -3.535250795749689387E-16, 22.75000000000000000, -5.773502691896257311 ) ) ;
#12405=CARTESIAN_POINT ( 'NONE',  ( -2.229367062499996610, -1.145833331967736957, 3.861377020970582219 ) ) ;
#12406=CARTESIAN_POINT ( 'NONE',  ( -5.000000000000000888, -160.6875000027311842, -2.071067811865475949 ) ) ;
#12408=CARTESIAN_POINT ( 'NONE',  ( -2.229367062500000163, 15.27083333469892779, -3.861377020970580443 ) ) ;
#12409=CARTESIAN_POINT ( 'NONE',  ( 2.500000000000002220, 0.4583333360645182042, 4.330127018922192761 ) ) ;
#12411=CARTESIAN_POINT ( 'NONE',  ( 1.339745962155612702, -42.29465819873851729, -5.000000000000000000 ) ) ;
#12413=CARTESIAN_POINT ( 'NONE',  ( -1.510657702057710340E-15, 27.37500000273118417, 5.000000000000000000 ) ) ;
#12414=CARTESIAN_POINT ( 'NONE',  ( 4.458734124999999437, -41.81249999863440081, -5.460374474430324690E-16 ) ) ;
#12415=CARTESIAN_POINT ( 'NONE',  ( -4.458734124999999437, -164.1875000013655779, -5.460374474430324690E-16 ) ) ;
#12416=CARTESIAN_POINT ( 'NONE',  ( -3.535250795749689387E-16, -45.12499999726880162, -5.773502691896257311 ) ) ;
#12417=VERTEX_POINT ( 'NONE', #57127 ) ;
#12418=CARTESIAN_POINT ( 'NONE',  ( -4.458734124999998549, -20.22916666530107221, 2.574251347313722516 ) ) ;
#12419=ORIENTED_EDGE ( 'NONE', *, *, #14240, .T. ) ;
#12421=CARTESIAN_POINT ( 'NONE',  ( 5.000000000000000000, -86.50000000000000000, -6.123233995736766282E-16 ) ) ;
#12422=CARTESIAN_POINT ( 'NONE',  ( 3.152801135295367541, -166.3125000013656063, -3.152801135295367541 ) ) ;
#12426=CARTESIAN_POINT ( 'NONE',  ( 4.458734125000001214, -34.14583333196772941, 2.574251347313718519 ) ) ;
#12427=CARTESIAN_POINT ( 'NONE',  ( -2.071067811865604735, -147.4375000027312410, 4.999999999999872990 ) ) ;
#12428=ORIENTED_EDGE ( 'NONE', *, *, #47647, .F. ) ;
#12432=VERTEX_POINT ( 'NONE', #3717 ) ;
#12434=CARTESIAN_POINT ( 'NONE',  ( 4.458734124999999437, -79.06249999863440792, -5.460374474430324690E-16 ) ) ;
#12436=CARTESIAN_POINT ( 'NONE',  ( -6.972266317189433020E-16, 22.74999999999999645, -5.000000000000000000 ) ) ;
#12437=CARTESIAN_POINT ( 'NONE',  ( -5.000000000000000888, -158.5625000027312126, 2.071067811865474617 ) ) ;
#12438=CARTESIAN_POINT ( 'NONE',  ( -1.127183054612291972E-14, 24.25000000000000000, 4.999999999999999112 ) ) ;
#12440=CARTESIAN_POINT ( 'NONE',  ( -4.458734124999999437, -44.31249999863440081, 0.000000000000000000 ) ) ;
#12441=CARTESIAN_POINT ( 'NONE',  ( -5.000000000000000000, 27.91666666666666430, -2.886751345948128211 ) ) ;
#12443=CARTESIAN_POINT ( 'NONE',  ( 3.535533905932738197, -154.0000000027312126, -3.535533905932738197 ) ) ;
#12446=CARTESIAN_POINT ( 'NONE',  ( 1.339745962155615144, 16.41965820146970501, 4.999999999999999112 ) ) ;
#12449=CARTESIAN_POINT ( 'NONE',  ( 2.229367062500001939, -78.22916666530106511, 3.861377020970579999 ) ) ;
#12450=DIRECTION ( 'NONE',  ( 0.000000000000000000, 0.000000000000000000, 1.000000000000000000 ) ) ;
#12453=ORIENTED_EDGE ( 'NONE', *, *, #57893, .F. ) ;
#12456=CARTESIAN_POINT ( 'NONE',  ( -3.535533905932737309, -168.7500000027312126, -3.535533905932738197 ) ) ;
#12458=CARTESIAN_POINT ( 'NONE',  ( 4.458734125000000326, 10.85416666803225993, 2.574251347313718519 ) ) ;
#12464=CARTESIAN_POINT ( 'NONE',  ( 2.499999999999998668, -38.20833333060213732, -4.330127018922193649 ) ) ;
#12466=CARTESIAN_POINT ( 'NONE',  ( 2.229367062499998831, -11.64583333196774007, -3.861377020970580887 ) ) ;
#12468=ORIENTED_EDGE ( 'NONE', *, *, #36971, .T. ) ;
#12469=CARTESIAN_POINT ( 'NONE',  ( 2.229367062499998831, -36.89583333196773651, -3.861377020970580887 ) ) ;
#12472=CARTESIAN_POINT ( 'NONE',  ( 5.000000000000000888, 0.5416666693978527958, 2.886751345948126879 ) ) ;
#12475=CARTESIAN_POINT ( 'NONE',  ( -1.846868145590737420, -149.0000000013656063, 4.458734124999997661 ) ) ;
#12476=CARTESIAN_POINT ( 'NONE',  ( -4.458734124999999437, 12.68750000136559564, 0.000000000000000000 ) ) ;
#12477=CARTESIAN_POINT ( 'NONE',  ( -6.972266317189433020E-16, -44.12499999726880162, -5.000000000000000000 ) ) ;
#12478=CARTESIAN_POINT ( 'NONE',  ( -2.229367062499996610, -85.39583333196773651, 3.861377020970582219 ) ) ;
#12480=CARTESIAN_POINT ( 'NONE',  ( 3.061616997868383141E-16, -140.7500000000000000, -5.000000000000000000 ) ) ;
#12481=CARTESIAN_POINT ( 'NONE',  ( 1.060575238724906964E-15, 20.37500000273119127, 5.773502691896257311 ) ) ;
#12482=VERTEX_POINT ( 'NONE', #62263 ) ;
#12483=CARTESIAN_POINT ( 'NONE',  ( 5.000000000000000888, -147.0625000027311842, -2.071067811865475505 ) ) ;
#12486=CARTESIAN_POINT ( 'NONE',  ( 5.000000000000000000, -25.41666666666666430, -2.886751345948129988 ) ) ;
#12487=CARTESIAN_POINT ( 'NONE',  ( -4.458734124999998549, -26.22916666530106866, 2.574251347313722516 ) ) ;
#12488=EDGE_CURVE ( 'NONE', #1596, #42874, #17312, .T. ) ;
#12489=CARTESIAN_POINT ( 'NONE',  ( 4.458734124999998549, -89.72916666530106511, -2.574251347313721627 ) ) ;
#12490=CARTESIAN_POINT ( 'NONE',  ( 5.000000000000000000, -29.37499999726881228, -6.123233995736766282E-16 ) ) ;
#12491=CARTESIAN_POINT ( 'NONE',  ( -4.458734124999999437, -58.39583333196774362, -2.574251347313719407 ) ) ;
#12493=CARTESIAN_POINT ( 'NONE',  ( 0.000000000000000000, -170.0000000000000000, 0.000000000000000000 ) ) ;
#12494=CARTESIAN_POINT ( 'NONE',  ( 9.457646018065525792E-16, -10.31249999863440614, 5.148502694627439702 ) ) ;
#12496=CARTESIAN_POINT ( 'NONE',  ( -5.000000000000000000, -74.08333333333332860, -2.886751345948128211 ) ) ;
#12499=CARTESIAN_POINT ( 'NONE',  ( 2.499999999999998668, -78.20833333060214443, -4.330127018922193649 ) ) ;
#12501=ORIENTED_EDGE ( 'NONE', *, *, #26313, .F. ) ;
#12503=CARTESIAN_POINT ( 'NONE',  ( -2.229367062500000163, -15.72916666530107399, -3.861377020970580443 ) ) ;
#12504=CARTESIAN_POINT ( 'NONE',  ( 4.458734124999999437, -58.06249999863440081, -5.460374474430324690E-16 ) ) ;
#12505=EDGE_CURVE ( 'NONE', #14472, #50070, #63335, .T. ) ;
#12507=CARTESIAN_POINT ( 'NONE',  ( 3.152801135295367541, -169.5625000013656063, -3.152801135295367541 ) ) ;
#12508=EDGE_CURVE ( 'NONE', #52130, #63378, #10348, .T. ) ;
#12511=ORIENTED_EDGE ( 'NONE', *, *, #12734, .T. ) ;
#12514=CARTESIAN_POINT ( 'NONE',  ( -5.000000000000000000, -12.87499999726881050, 0.000000000000000000 ) ) ;
#12517=CARTESIAN_POINT ( 'NONE',  ( -1.846868145590734756, -148.3750000013655779, -4.458734125000000326 ) ) ;
#12519=DIRECTION ( 'NONE',  ( -0.000000000000000000, 1.000000000000000000, -0.000000000000000000 ) ) ;
#12521=CARTESIAN_POINT ( 'NONE',  ( -3.152548672688508926E-16, -60.81249999863440081, -5.148502694627439702 ) ) ;
#12524=CARTESIAN_POINT ( 'NONE',  ( 1.846868145590736310, -145.6250000013655779, 4.458734124999997661 ) ) ;
#12528=DIRECTION ( 'NONE',  ( -0.000000000000000000, 1.000000000000000000, -0.000000000000000000 ) ) ;
#12531=CARTESIAN_POINT ( 'NONE',  ( 0.000000000000000000, -170.0000000000000000, 0.000000000000000000 ) ) ;
#12538=CARTESIAN_POINT ( 'NONE',  ( -4.458734124999999437, 8.604166668032261711, -2.574251347313719407 ) ) ;
#12540=CARTESIAN_POINT ( 'NONE',  ( 2.229367062500001939, -18.22916666530106866, 3.861377020970579999 ) ) ;
#12542=CARTESIAN_POINT ( 'NONE',  ( -4.458734124999999437, -158.9375000013655779, -5.460374474430324690E-16 ) ) ;
#12543=CARTESIAN_POINT ( 'NONE',  ( 5.000000000000000000, 23.50000000000000000, -6.123233995736766282E-16 ) ) ;
#12547=( BOUNDED_CURVE ( )  B_SPLINE_CURVE ( 2, ( #45001, #45640, #15420, #16049, #59812, #20240, #40802, #50785, #55305 ),
 .UNSPECIFIED., .F., .F. ) 
 B_SPLINE_CURVE_WITH_KNOTS ( ( 3, 2, 2, 2, 3 ),
 ( 0.8604166666666667185, 0.8611111111111111605, 0.8625000000000000444, 0.8638888888888889284, 0.8645833333333333703 ),
 .UNSPECIFIED. ) 
 CURVE ( )  GEOMETRIC_REPRESENTATION_ITEM ( )  RATIONAL_B_SPLINE_CURVE ( ( 0.9330127018922194093, 0.9330127018922194093, 1.000000000000000000, 0.8660254037844387076, 1.000000000000000000, 0.8660254037844387076, 1.000000000000000000, 0.9330127018922194093, 0.9330127018922194093 ) ) 
 REPRESENTATION_ITEM ( '' )  );
#12548=CARTESIAN_POINT ( 'NONE',  ( -1.339745962155610925, -35.79465819873851729, 5.000000000000000000 ) ) ;
#12549=CARTESIAN_POINT ( 'NONE',  ( 4.458734124999998549, -39.72916666530107221, -2.574251347313721627 ) ) ;
#12550=CARTESIAN_POINT ( 'NONE',  ( -6.972266317189433020E-16, 19.87500000273118417, -5.000000000000000000 ) ) ;
#12551=CARTESIAN_POINT ( 'NONE',  ( 4.458734124999998549, -66.97916666530106511, -2.574251347313721627 ) ) ;
#12557=CARTESIAN_POINT ( 'NONE',  ( -4.999999999999998224, -67.79166666393547303, 2.886751345948131764 ) ) ;
#12558=CARTESIAN_POINT ( 'NONE',  ( 5.000000000000000888, -8.583333333333330373, 2.886751345948126879 ) ) ;
#12560=CARTESIAN_POINT ( 'NONE',  ( 2.229367062499998831, -71.64583333196773651, -3.861377020970580887 ) ) ;
#12563=CARTESIAN_POINT ( 'NONE',  ( 2.499999999999998668, -13.20833333060214976, -4.330127018922193649 ) ) ;
#12564=CARTESIAN_POINT ( 'NONE',  ( 2.229367062499998831, -41.64583333196773651, -3.861377020970580887 ) ) ;
#12566=DIRECTION ( 'NONE',  ( -0.000000000000000000, 1.000000000000000000, -0.000000000000000000 ) ) ;
#12567=CARTESIAN_POINT ( 'NONE',  ( 2.229367062500001939, 8.770833334698927786, 3.861377020970579999 ) ) ;
#12569=CARTESIAN_POINT ( 'NONE',  ( -6.972266317189433020E-16, -34.12499999726881583, -5.000000000000000000 ) ) ;
#12570=CARTESIAN_POINT ( 'NONE',  ( -5.000000000000000000, -58.08333333333332860, -2.886751345948128211 ) ) ;
#12571=CARTESIAN_POINT ( 'NONE',  ( 4.458734124999999437, -160.6875000013655779, 0.000000000000000000 ) ) ;
#12574=CARTESIAN_POINT ( 'NONE',  ( -4.458734124999999437, -82.39583333196773651, -2.574251347313719407 ) ) ;
#12575=CARTESIAN_POINT ( 'NONE',  ( -2.071067811865475061, -164.6875000000000568, -5.000000000000000888 ) ) ;
#12577=CARTESIAN_POINT ( 'NONE',  ( 2.229367062500001939, -88.97916666530106511, 3.861377020970579999 ) ) ;
#12579=CARTESIAN_POINT ( 'NONE',  ( 2.229367062500001939, -1.229166665301071548, 3.861377020970579999 ) ) ;
#12580=CARTESIAN_POINT ( 'NONE',  ( -4.458734124999999437, -36.64583333196773651, -2.574251347313719407 ) ) ;
#12581=CARTESIAN_POINT ( 'NONE',  ( 5.000000000000000888, -72.58333333333332860, 2.886751345948126879 ) ) ;
#12588=CARTESIAN_POINT ( 'NONE',  ( -5.000000000000000000, -18.87499999726881583, 0.000000000000000000 ) ) ;
#12589=CARTESIAN_POINT ( 'NONE',  ( -2.229367062499996610, -69.39583333196773651, 3.861377020970582219 ) ) ;
#12592=ORIENTED_EDGE ( 'NONE', *, *, #5515, .F. ) ;
#12593=DIRECTION ( 'NONE',  ( -0.000000000000000000, 1.000000000000000000, -0.000000000000000000 ) ) ;
#12594=CARTESIAN_POINT ( 'NONE',  ( 6.123233995736766282E-16, -170.0000000000000000, -5.000000000000000000 ) ) ;
#12596=LINE ( 'NONE', #1147, #44577 ) ;
#12597=CARTESIAN_POINT ( 'NONE',  ( -4.458734124999998549, 4.770833334698926009, 2.574251347313722516 ) ) ;
#12598=CARTESIAN_POINT ( 'NONE',  ( -1.339745962155610925, -75.79465819873853150, 5.000000000000000000 ) ) ;
#12599=CARTESIAN_POINT ( 'NONE',  ( -1.846868145590737420, -156.7500000013656063, 4.458734124999997661 ) ) ;
#12601=ORIENTED_EDGE ( 'NONE', *, *, #34737, .T. ) ;
#12603=CARTESIAN_POINT ( 'NONE',  ( -2.499999999999996447, -24.83333333333333215, 4.330127018922195425 ) ) ;
#12605=EDGE_CURVE ( 'NONE', #15422, #50505, #19437, .T. ) ;
#12606=CARTESIAN_POINT ( 'NONE',  ( -9.184850993605147944E-16, -166.2500000000000000, 5.000000000000000000 ) ) ;
#12609=CARTESIAN_POINT ( 'NONE',  ( 1.975475456537005874E-15, 8.249999999999998224, 5.000000000000000000 ) ) ;
#12612=CARTESIAN_POINT ( 'NONE',  ( 4.458734124999998549, 25.27083333469892779, -2.574251347313721627 ) ) ;
#12614=CARTESIAN_POINT ( 'NONE',  ( 4.458734124999998549, -1.979166665301068662, -2.574251347313721627 ) ) ;
#12615=( BOUNDED_CURVE ( )  B_SPLINE_CURVE ( 2, ( #31069, #35907, #50693, #5680, #6636, #60039, #44917, #26244, #59393 ),
 .UNSPECIFIED., .F., .F. ) 
 B_SPLINE_CURVE_WITH_KNOTS ( ( 3, 2, 2, 2, 3 ),
 ( 0.2250000000000001998, 0.2291666666666668517, 0.2333333333333335313, 0.2375000000000001832, 0.2416666666666668628 ),
 .UNSPECIFIED. ) 
 CURVE ( )  GEOMETRIC_REPRESENTATION_ITEM ( )  RATIONAL_B_SPLINE_CURVE ( ( 0.9999999999999964473, 0.9238795325112902912, 1.000000000000000000, 0.9238795325112867385, 1.000000000000000000, 0.9238795325112867385, 1.000000000000000000, 0.9238795325112831858, 1.000000000000003553 ) ) 
 REPRESENTATION_ITEM ( '' )  );
#12618=CARTESIAN_POINT ( 'NONE',  ( -5.000000000000000888, -140.5625000027312410, 2.071067811865474617 ) ) ;
#12624=CARTESIAN_POINT ( 'NONE',  ( 1.339745962155612702, -22.29465819873851729, -5.000000000000000000 ) ) ;
#12626=CARTESIAN_POINT ( 'NONE',  ( -1.846868145590737420, -158.0000000013656063, 4.458734124999997661 ) ) ;
#12628=VERTEX_POINT ( 'NONE', #44509 ) ;
#12629=CARTESIAN_POINT ( 'NONE',  ( 4.458734124999998549, 18.02083333469892779, -2.574251347313721627 ) ) ;
#12630=ORIENTED_EDGE ( 'NONE', *, *, #54153, .T. ) ;
#12635=CARTESIAN_POINT ( 'NONE',  ( 5.000000000000000000, 7.500000000000000000, -6.123233995736766282E-16 ) ) ;
#12636=CARTESIAN_POINT ( 'NONE',  ( 9.457646018065525792E-16, -57.06249999863440081, 5.148502694627439702 ) ) ;
#12640=ADVANCED_FACE ( 'NONE', ( #63513 ), #58678, .T. ) ;
#12641=DIRECTION ( 'NONE',  ( -0.000000000000000000, 1.000000000000000000, -0.000000000000000000 ) ) ;
#12646=CARTESIAN_POINT ( 'NONE',  ( 5.000000000000000888, -37.58333333333332860, 2.886751345948126879 ) ) ;
#12647=DIRECTION ( 'NONE',  ( 0.000000000000000000, 0.000000000000000000, 1.000000000000000000 ) ) ;
#12650=CYLINDRICAL_SURFACE ( 'NONE', #41960, 5.000000000000000000 ) ;
#12651=CARTESIAN_POINT ( 'NONE',  ( 4.458734125000001214, -65.89583333196772230, 2.574251347313718519 ) ) ;
#12652=CARTESIAN_POINT ( 'NONE',  ( -4.458734125000000326, -149.2500000013655779, -1.846868145590735644 ) ) ;
#12653=CARTESIAN_POINT ( 'NONE',  ( -3.152548672688508926E-16, -73.56249999863440792, -5.148502694627439702 ) ) ;
#12656=CARTESIAN_POINT ( 'NONE',  ( -4.458734124999998549, -20.47916666530107577, 2.574251347313722516 ) ) ;
#12657=CARTESIAN_POINT ( 'NONE',  ( 1.060575238724906964E-15, -61.62499999726880873, 5.773502691896257311 ) ) ;
#12659=CARTESIAN_POINT ( 'NONE',  ( 3.061616997868383141E-16, -150.7500000000000284, -5.000000000000000000 ) ) ;
#12665=EDGE_CURVE ( 'NONE', #27072, #61565, #16211, .T. ) ;
#12666=ORIENTED_EDGE ( 'NONE', *, *, #22108, .T. ) ;
#12668=EDGE_CURVE ( 'NONE', #45244, #49104, #30059, .T. ) ;
#12671=CARTESIAN_POINT ( 'NONE',  ( -6.972266317189433020E-16, -75.12499999726880162, -5.000000000000000000 ) ) ;
#12672=CARTESIAN_POINT ( 'NONE',  ( -2.229367062499996610, -55.39583333196773651, 3.861377020970582219 ) ) ;
#12674=DIRECTION ( 'NONE',  ( -0.000000000000000000, 1.000000000000000000, -0.000000000000000000 ) ) ;
#12676=CARTESIAN_POINT ( 'NONE',  ( -2.229367062500000163, 18.52083333469892779, -3.861377020970580443 ) ) ;
#12679=CARTESIAN_POINT ( 'NONE',  ( -1.846868145590737420, -168.7500000013656063, 4.458734124999997661 ) ) ;
#12680=VERTEX_POINT ( 'NONE', #20725 ) ;
#12684=CARTESIAN_POINT ( 'NONE',  ( 3.061616997868383141E-16, -139.8750000027312126, -5.000000000000000000 ) ) ;
#12694=CARTESIAN_POINT ( 'NONE',  ( -6.972266317189433020E-16, -22.12499999726881228, -5.000000000000000000 ) ) ;
#12696=CARTESIAN_POINT ( 'NONE',  ( 3.535533905932738197, -153.0000000027312126, -3.535533905932738197 ) ) ;
#12702=CARTESIAN_POINT ( 'NONE',  ( -5.000000000000000888, -146.4375000000000000, 2.071067811865474617 ) ) ;
#12705=CARTESIAN_POINT ( 'NONE',  ( -4.458734124999999437, -24.39583333196773651, -2.574251347313719407 ) ) ;
#12706=CARTESIAN_POINT ( 'NONE',  ( 3.535533905932738197, -146.8750000000000000, -3.535533905932738197 ) ) ;
#12707=CARTESIAN_POINT ( 'NONE',  ( 2.500000000000002220, 18.45833333606451632, 4.330127018922192761 ) ) ;
#12709=CARTESIAN_POINT ( 'NONE',  ( 2.730187237215162345E-16, -148.1875000013656063, -4.458734124999999437 ) ) ;
#12712=CARTESIAN_POINT ( 'NONE',  ( -4.458734124999997661, -49.47916666530107221, 2.574251347313722516 ) ) ;
#12713=CARTESIAN_POINT ( 'NONE',  ( 2.500000000000002220, -2.666666666666664298, 4.330127018922192761 ) ) ;
#12715=CARTESIAN_POINT ( 'NONE',  ( -2.500000000000000444, 23.83333333333333215, -4.330127018922193649 ) ) ;
#12717=CARTESIAN_POINT ( 'NONE',  ( 4.458734125000001214, -1.895833331967737623, 2.574251347313718519 ) ) ;
#12720=CARTESIAN_POINT ( 'NONE',  ( -2.499999999999996447, -73.83333333333332860, 4.330127018922195425 ) ) ;
#12721=CARTESIAN_POINT ( 'NONE',  ( -4.458734124999999437, 8.437500001365595637, 0.000000000000000000 ) ) ;
#12724=ORIENTED_EDGE ( 'NONE', *, *, #15037, .F. ) ;
#12725=CARTESIAN_POINT ( 'NONE',  ( 2.499999999999998668, -7.208333330602150646, -4.330127018922193649 ) ) ;
#12726=CARTESIAN_POINT ( 'NONE',  ( 4.458734124999998549, -48.72916666530107221, -2.574251347313721627 ) ) ;
#12727=CARTESIAN_POINT ( 'NONE',  ( 4.458734124999999437, -162.7500000013655779, 1.846868145590737864 ) ) ;
#12728=CARTESIAN_POINT ( 'NONE',  ( -4.999999999999999112, -42.79166666393548013, 2.886751345948131764 ) ) ;
#12729=ORIENTED_EDGE ( 'NONE', *, *, #9096, .T. ) ;
#12730=CARTESIAN_POINT ( 'NONE',  ( 2.229367062499998831, -25.64583333196773651, -3.861377020970580887 ) ) ;
#12731=EDGE_LOOP ( 'NONE', ( #29648, #39121, #48947, #31792 ) ) ;
#12732=CARTESIAN_POINT ( 'NONE',  ( -2.071067811865432873, -142.8125000027312410, -5.000000000000041744 ) ) ;
#12733=CARTESIAN_POINT ( 'NONE',  ( -4.458734125000001214, -163.8750000013655779, 1.846868145590734089 ) ) ;
#12734=EDGE_CURVE ( 'NONE', #49021, #33297, #49796, .T. ) ;
#12735=FACE_OUTER_BOUND ( 'NONE', #4838, .T. ) ;
#12737=CARTESIAN_POINT ( 'NONE',  ( -4.458734124999999437, -39.64583333196774362, -2.574251347313719407 ) ) ;
#12738=CARTESIAN_POINT ( 'NONE',  ( 0.000000000000000000, -170.0000000000000000, 0.000000000000000000 ) ) ;
#12739=ORIENTED_EDGE ( 'NONE', *, *, #24396, .F. ) ;
#12744=CARTESIAN_POINT ( 'NONE',  ( 1.339745962155612702, -59.29465819873853150, -5.000000000000000000 ) ) ;
#12748=CARTESIAN_POINT ( 'NONE',  ( 4.458734125000001214, -78.14583333196775072, 2.574251347313718519 ) ) ;
#12750=FACE_OUTER_BOUND ( 'NONE', #50971, .T. ) ;
#12751=CARTESIAN_POINT ( 'NONE',  ( 3.061616997868383141E-16, -144.8750000027312126, -5.000000000000000000 ) ) ;
#12753=CARTESIAN_POINT ( 'NONE',  ( -5.000000000000000000, -71.95833333060214443, -2.886751345948128211 ) ) ;
#12756=CARTESIAN_POINT ( 'NONE',  ( -6.972266317189433020E-16, 3.749999999999999556, -5.000000000000000000 ) ) ;
#12759=CARTESIAN_POINT ( 'NONE',  ( 5.000000000000000888, 16.54166666939785202, 2.886751345948126879 ) ) ;
#12761=CARTESIAN_POINT ( 'NONE',  ( 2.229367062500001939, -81.22916666530106511, 3.861377020970579999 ) ) ;
#12764=ORIENTED_EDGE ( 'NONE', *, *, #56675, .T. ) ;
#12767=CARTESIAN_POINT ( 'NONE',  ( -3.535533905932737309, -164.7500000027312126, -3.535533905932738197 ) ) ;
#12769=CARTESIAN_POINT ( 'NONE',  ( 4.458734124999998549, 11.02083333469892956, -2.574251347313721627 ) ) ;
#12770=DIRECTION ( 'NONE',  ( 0.000000000000000000, 0.000000000000000000, 1.000000000000000000 ) ) ;
#12776=CARTESIAN_POINT ( 'NONE',  ( 5.000000000000000888, -38.45833333060213732, 2.886751345948126879 ) ) ;
#12777=DIRECTION ( 'NONE',  ( -0.000000000000000000, 1.000000000000000000, -0.000000000000000000 ) ) ;
#12778=CARTESIAN_POINT ( 'NONE',  ( 4.458734124999998549, -7.729166665301073991, -2.574251347313721627 ) ) ;
#12780=EDGE_LOOP ( 'NONE', ( #30929, #37777, #5056, #47392 ) ) ;
#12781=CARTESIAN_POINT ( 'NONE',  ( 9.457646018065525792E-16, -36.31249999863440792, 5.148502694627439702 ) ) ;
#12786=CARTESIAN_POINT ( 'NONE',  ( 4.458734124999999437, -149.6875000013656063, 0.000000000000000000 ) ) ;
#12787=CARTESIAN_POINT ( 'NONE',  ( 2.229367062499998831, 17.35416666803225993, -3.861377020970580887 ) ) ;
#12790=CYLINDRICAL_SURFACE ( 'NONE', #30706, 5.000000000000000000 ) ;
#12791=CARTESIAN_POINT ( 'NONE',  ( 9.457646018065525792E-16, -84.31249999863440792, 5.148502694627439702 ) ) ;
#12793=( BOUNDED_CURVE ( )  B_SPLINE_CURVE ( 2, ( #36073, #60530, #26104, #49584, #5526, #15818, #16454, #60211, #713 ),
 .UNSPECIFIED., .F., .F. ) 
 B_SPLINE_CURVE_WITH_KNOTS ( ( 3, 2, 2, 2, 3 ),
 ( 0.2854166666666666519, 0.2861111111111110938, 0.2874999999999999778, 0.2888888888888888618, 0.2895833333333333592 ),
 .UNSPECIFIED. ) 
 CURVE ( )  GEOMETRIC_REPRESENTATION_ITEM ( )  RATIONAL_B_SPLINE_CURVE ( ( 0.9330127018922194093, 0.9330127018922194093, 1.000000000000000000, 0.8660254037844387076, 1.000000000000000000, 0.8660254037844387076, 1.000000000000000000, 0.9330127018922167448, 0.9330127018922194093 ) ) 
 REPRESENTATION_ITEM ( '' )  );
#12794=CARTESIAN_POINT ( 'NONE',  ( -1.339745962155610925, -1.669658196007333784, 5.000000000000000000 ) ) ;
#12795=CARTESIAN_POINT ( 'NONE',  ( 2.500000000000002220, 18.45833333606451632, 4.330127018922192761 ) ) ;
#12799=FACE_OUTER_BOUND ( 'NONE', #2858, .T. ) ;
#12801=CARTESIAN_POINT ( 'NONE',  ( 1.060575238724906964E-15, -28.74999999999999645, 5.773502691896257311 ) ) ;
#12802=CARTESIAN_POINT ( 'NONE',  ( 4.458734124999999437, -33.81249999863440792, -5.460374474430324690E-16 ) ) ;
#12803=CARTESIAN_POINT ( 'NONE',  ( 6.123233995736766282E-16, -170.0000000000000000, -5.000000000000000000 ) ) ;
#12804=CARTESIAN_POINT ( 'NONE',  ( 1.060575238724906964E-15, -26.62499999726881228, 5.773502691896257311 ) ) ;
#12805=CARTESIAN_POINT ( 'NONE',  ( -3.152548672688508926E-16, -59.56249999863440081, -5.148502694627439702 ) ) ;
#12808=CARTESIAN_POINT ( 'NONE',  ( 4.458734125000001214, -11.14583333196774007, 2.574251347313718519 ) ) ;
#12810=CARTESIAN_POINT ( 'NONE',  ( 2.499999999999998668, -69.33333333333332860, -4.330127018922193649 ) ) ;
#12813=CARTESIAN_POINT ( 'NONE',  ( 5.000000000000000000, -79.37499999726881583, -6.123233995736766282E-16 ) ) ;
#12817=CARTESIAN_POINT ( 'NONE',  ( 4.458734125000001214, -16.14583333196773651, 2.574251347313718519 ) ) ;
#12818=CARTESIAN_POINT ( 'NONE',  ( -4.458734124999999437, -57.64583333196773651, -2.574251347313719407 ) ) ;
#12819=CARTESIAN_POINT ( 'NONE',  ( -6.972266317189433020E-16, -24.24999999999999645, -5.000000000000000000 ) ) ;
#12820=CARTESIAN_POINT ( 'NONE',  ( -3.152801135295367985, -139.8125000013655779, 3.152801135295367096 ) ) ;
#12822=DIRECTION ( 'NONE',  ( 0.000000000000000000, 0.000000000000000000, 1.000000000000000000 ) ) ;
#12823=( BOUNDED_CURVE ( )  B_SPLINE_CURVE ( 2, ( #29376, #44184, #39671, #786, #5595, #63194, #53839, #38721, #58362 ),
 .UNSPECIFIED., .F., .F. ) 
 B_SPLINE_CURVE_WITH_KNOTS ( ( 3, 2, 2, 2, 3 ),
 ( 0.04166666666666670599, 0.04583333333333337173, 0.05000000000000004441, 0.05416666666666671709, 0.05833333333333338283 ),
 .UNSPECIFIED. ) 
 CURVE ( )  GEOMETRIC_REPRESENTATION_ITEM ( )  RATIONAL_B_SPLINE_CURVE ( ( 0.9999999999999992228, 0.9238795325112875156, 1.000000000000000000, 0.9238795325112867385, 1.000000000000000000, 0.9238795325112867385, 1.000000000000000000, 0.9238795325112858503, 1.000000000000000888 ) ) 
 REPRESENTATION_ITEM ( '' )  );
#12827=FACE_OUTER_BOUND ( 'NONE', #5534, .T. ) ;
#12830=CARTESIAN_POINT ( 'NONE',  ( 2.730187237215162345E-16, -146.4375000013656063, -4.458734124999999437 ) ) ;
#12834=CARTESIAN_POINT ( 'NONE',  ( -2.229367062499996610, -64.39583333196773651, 3.861377020970582219 ) ) ;
#12837=CARTESIAN_POINT ( 'NONE',  ( 1.846868145590735200, -145.2500000013656347, -4.458734124999999437 ) ) ;
#12840=VERTEX_POINT ( 'NONE', #6249 ) ;
#12842=CARTESIAN_POINT ( 'NONE',  ( -9.184850993605147944E-16, -144.2500000000000284, 5.000000000000000000 ) ) ;
#12846=CARTESIAN_POINT ( 'NONE',  ( 1.975475456537005874E-15, -14.62499999726881228, 5.000000000000000000 ) ) ;
#12849=CARTESIAN_POINT ( 'NONE',  ( -2.229367062500000163, 27.27083333469892779, -3.861377020970580443 ) ) ;
#12853=DIRECTION ( 'NONE',  ( 0.000000000000000000, 0.000000000000000000, 1.000000000000000000 ) ) ;
#12855=CARTESIAN_POINT ( 'NONE',  ( -2.229367062500000163, 8.520833334698926009, -3.861377020970580443 ) ) ;
#12857=CARTESIAN_POINT ( 'NONE',  ( 4.458734125000000326, -18.14583333196773651, 2.574251347313718519 ) ) ;
#12859=CARTESIAN_POINT ( 'NONE',  ( -4.458734124999999437, -159.9375000013655779, -5.460374474430324690E-16 ) ) ;
#12860=CARTESIAN_POINT ( 'NONE',  ( 1.339745962155612702, 15.83034180399266511, -5.000000000000000000 ) ) ;
#12863=VECTOR ( 'NONE', #43753, 1000.000000000000000 ) ;
#12865=CARTESIAN_POINT ( 'NONE',  ( -4.458734124999999437, -42.39583333196773651, -2.574251347313719407 ) ) ;
#12867=CARTESIAN_POINT ( 'NONE',  ( 2.229367062499998831, -69.89583333196773651, -3.861377020970580887 ) ) ;
#12871=VERTEX_POINT ( 'NONE', #25538 ) ;
#12873=LINE ( 'NONE', #2929, #53477 ) ;
#12874=CARTESIAN_POINT ( 'NONE',  ( 5.000000000000000888, -7.583333333333330373, 2.886751345948126879 ) ) ;
#12875=CARTESIAN_POINT ( 'NONE',  ( 2.229367062499998831, -13.64583333196774184, -3.861377020970580887 ) ) ;
#12876=CARTESIAN_POINT ( 'NONE',  ( -4.458734124999999437, -76.31249999863440792, 0.000000000000000000 ) ) ;
#12878=CARTESIAN_POINT ( 'NONE',  ( 5.000000000000000000, -14.37499999726881228, -6.123233995736766282E-16 ) ) ;
#12879=CARTESIAN_POINT ( 'NONE',  ( -4.458734124999999437, -44.39583333196773651, -2.574251347313719407 ) ) ;
#12880=ORIENTED_EDGE ( 'NONE', *, *, #53981, .F. ) ;
#12882=CARTESIAN_POINT ( 'NONE',  ( -4.458734124999999437, 4.437500001365595637, 0.000000000000000000 ) ) ;
#12884=CARTESIAN_POINT ( 'NONE',  ( 2.500000000000002220, -34.54166666393547303, 4.330127018922192761 ) ) ;
#12885=CARTESIAN_POINT ( 'NONE',  ( -4.999999999999999112, -55.91666666666667140, 2.886751345948131764 ) ) ;
#12886=CARTESIAN_POINT ( 'NONE',  ( 1.846868145590735200, -158.5000000013656631, -4.458734125000000326 ) ) ;
#12888=CARTESIAN_POINT ( 'NONE',  ( -3.152548672688508926E-16, -80.56249999863440792, -5.148502694627439702 ) ) ;
#12889=CARTESIAN_POINT ( 'NONE',  ( -9.184850993605147944E-16, -166.2500000000000000, 5.000000000000000000 ) ) ;
#12890=CARTESIAN_POINT ( 'NONE',  ( 5.000000000000000000, 5.625000002731185056, -6.123233995736766282E-16 ) ) ;
#12892=CARTESIAN_POINT ( 'NONE',  ( 2.229367062500001939, 1.770833334698927786, 3.861377020970579999 ) ) ;
#12893=CARTESIAN_POINT ( 'NONE',  ( 4.458734125000001214, -42.14583333196773651, 2.574251347313718519 ) ) ;
#12895=CARTESIAN_POINT ( 'NONE',  ( 5.000000000000000000, -84.49999999999998579, -6.123233995736766282E-16 ) ) ;
#12898=CARTESIAN_POINT ( 'NONE',  ( -9.184850993605147944E-16, -152.2500000000000000, 5.000000000000000000 ) ) ;
#12899=CARTESIAN_POINT ( 'NONE',  ( -4.458734124999999437, -69.64583333196773651, -2.574251347313719407 ) ) ;
#12901=VERTEX_POINT ( 'NONE', #40329 ) ;
#12902=VECTOR ( 'NONE', #45431, 1000.000000000000000 ) ;
#12903=CARTESIAN_POINT ( 'NONE',  ( 3.535533905932736864, -164.1250000000000284, 3.535533905932738641 ) ) ;
#12904=CARTESIAN_POINT ( 'NONE',  ( -1.049326080737009628E-13, -3.624999997268818053, 5.000000000000000000 ) ) ;
#12907=CARTESIAN_POINT ( 'NONE',  ( -3.152548672688508926E-16, 0.4375000013655955255, -5.148502694627439702 ) ) ;
#12909=CARTESIAN_POINT ( 'NONE',  ( 1.846868145590736310, -158.6250000013655779, 4.458734124999997661 ) ) ;
#12913=CARTESIAN_POINT ( 'NONE',  ( -1.339745962155610925, -24.79465819873852439, 5.000000000000000000 ) ) ;
#12917=CARTESIAN_POINT ( 'NONE',  ( -6.972266317189433020E-16, 0.7499999999999996669, -5.000000000000000000 ) ) ;
#12921=CARTESIAN_POINT ( 'NONE',  ( 0.000000000000000000, -170.0000000000000000, 0.000000000000000000 ) ) ;
#12924=CARTESIAN_POINT ( 'NONE',  ( 9.457646018065525792E-16, 20.93750000136558853, 5.148502694627439702 ) ) ;
#12926=CARTESIAN_POINT ( 'NONE',  ( -2.229367062499996610, -1.395833331967737179, 3.861377020970582219 ) ) ;
#12929=CARTESIAN_POINT ( 'NONE',  ( 5.000000000000000888, -140.0625000027312126, -2.071067811865475505 ) ) ;
#12930=CARTESIAN_POINT ( 'NONE',  ( 1.975475456537005874E-15, -75.62499999726880162, 5.000000000000000000 ) ) ;
#12935=DIRECTION ( 'NONE',  ( -0.000000000000000000, 1.000000000000000000, -0.000000000000000000 ) ) ;
#12938=EDGE_CURVE ( 'NONE', #51592, #39751, #43213, .T. ) ;
#12940=CARTESIAN_POINT ( 'NONE',  ( -3.152801135295367096, -159.3125000013656063, -3.152801135295367541 ) ) ;
#12943=CARTESIAN_POINT ( 'NONE',  ( 9.457646018065525792E-16, 19.68750000136559208, 5.148502694627439702 ) ) ;
#12948=CARTESIAN_POINT ( 'NONE',  ( 2.500000000000002220, -16.66666666666666430, 4.330127018922192761 ) ) ;
#12949=CARTESIAN_POINT ( 'NONE',  ( -2.499999999999996447, 8.166666666666666075, 4.330127018922195425 ) ) ;
#12950=EDGE_CURVE ( 'NONE', #51146, #8450, #5850, .T. ) ;
#12951=CARTESIAN_POINT ( 'NONE',  ( -4.458734124999997661, -58.22916666530106511, 2.574251347313722516 ) ) ;
#12952=CARTESIAN_POINT ( 'NONE',  ( 1.975475456537005874E-15, -52.62499999726880873, 5.000000000000000000 ) ) ;
#12954=CARTESIAN_POINT ( 'NONE',  ( -2.229367062500000163, -28.47916666530107221, -3.861377020970580443 ) ) ;
#12956=CARTESIAN_POINT ( 'NONE',  ( -1.339745962155613812, -25.08034179853028789, -5.000000000000000000 ) ) ;
#12957=CARTESIAN_POINT ( 'NONE',  ( -5.000000000000000000, -39.99999999999999289, 0.000000000000000000 ) ) ;
#12958=DIRECTION ( 'NONE',  ( 0.000000000000000000, 0.000000000000000000, 1.000000000000000000 ) ) ;
#12959=CARTESIAN_POINT ( 'NONE',  ( -2.500000000000000444, 14.83333333333333215, -4.330127018922193649 ) ) ;
#12961=CARTESIAN_POINT ( 'NONE',  ( -5.000000000000000000, -143.5000000000000284, -6.123233995736766282E-16 ) ) ;
#12962=CARTESIAN_POINT ( 'NONE',  ( -4.458734124999998549, -67.22916666530106511, 2.574251347313722516 ) ) ;
#12963=CARTESIAN_POINT ( 'NONE',  ( -3.152801135295367096, -149.3125000013655779, -3.152801135295367541 ) ) ;
#12964=CARTESIAN_POINT ( 'NONE',  ( -2.229367062499996610, -73.14583333196773651, 3.861377020970582219 ) ) ;
#12966=CARTESIAN_POINT ( 'NONE',  ( -2.229367062500000163, -25.72916666530106866, -3.861377020970580443 ) ) ;
#12967=CARTESIAN_POINT ( 'NONE',  ( -5.000000000000000000, -62.95833333060214443, -2.886751345948128211 ) ) ;
#12969=ADVANCED_FACE ( 'NONE', ( #2077 ), #52209, .T. ) ;
#12978=CARTESIAN_POINT ( 'NONE',  ( -1.339745962155613812, -56.08034179853028434, -5.000000000000000000 ) ) ;
#12979=CARTESIAN_POINT ( 'NONE',  ( 4.458734124999998549, -55.97916666530107932, -2.574251347313721627 ) ) ;
#12983=CARTESIAN_POINT ( 'NONE',  ( 4.458734125000001214, 17.10416666803225993, 2.574251347313718519 ) ) ;
#12985=CARTESIAN_POINT ( 'NONE',  ( 2.499999999999998668, 20.79166666939784847, -4.330127018922193649 ) ) ;
#12987=( BOUNDED_CURVE ( )  B_SPLINE_CURVE ( 2, ( #33096, #62692, #18616, #38242, #25977, #10857, #34668, #34342, #49463 ),
 .UNSPECIFIED., .F., .F. ) 
 B_SPLINE_CURVE_WITH_KNOTS ( ( 3, 2, 2, 2, 3 ),
 ( 0.8187499999999999778, 0.8194444444444444198, 0.8208333333333333037, 0.8222222222222221877, 0.8229166666666666297 ),
 .UNSPECIFIED. ) 
 CURVE ( )  GEOMETRIC_REPRESENTATION_ITEM ( )  RATIONAL_B_SPLINE_CURVE ( ( 0.9330127018922194093, 0.9330127018922194093, 1.000000000000000000, 0.8660254037844387076, 1.000000000000000000, 0.8660254037844387076, 1.000000000000000000, 0.9330127018922194093, 0.9330127018922194093 ) ) 
 REPRESENTATION_ITEM ( '' )  );
#12988=AXIS2_PLACEMENT_3D ( 'NONE', #22055, #55834, #7271 ) ;
#12989=ORIENTED_EDGE ( 'NONE', *, *, #44521, .T. ) ;
#12993=AXIS2_PLACEMENT_3D ( 'NONE', #61760, #31842, #62073 ) ;
#12995=EDGE_CURVE ( 'NONE', #27115, #30305, #22312, .T. ) ;
#12996=DIRECTION ( 'NONE',  ( -0.000000000000000000, 1.000000000000000000, -0.000000000000000000 ) ) ;
#12997=ADVANCED_FACE ( 'NONE', ( #41586 ), #12650, .T. ) ;
#13000=CARTESIAN_POINT ( 'NONE',  ( 1.339745962155612702, 4.705341801261479162, -5.000000000000000000 ) ) ;
#13002=CARTESIAN_POINT ( 'NONE',  ( -1.049326080737009628E-13, -20.62499999726881583, 5.000000000000000000 ) ) ;
#13003=LINE ( 'NONE', #16882, #62452 ) ;
#13009=CARTESIAN_POINT ( 'NONE',  ( -3.535533905932737309, -153.7500000027312126, -3.535533905932738197 ) ) ;
#13016=CARTESIAN_POINT ( 'NONE',  ( -3.535533905932738641, -145.3750000000000000, 3.535533905932737309 ) ) ;
#13020=CARTESIAN_POINT ( 'NONE',  ( 4.458734124999997661, -168.7500000013656063, 1.846868145590737864 ) ) ;
#13021=CARTESIAN_POINT ( 'NONE',  ( 2.229367062500001939, -22.97916666530107221, 3.861377020970579999 ) ) ;
#13025=CARTESIAN_POINT ( 'NONE',  ( 4.458734124999999437, -148.4375000013656063, 0.000000000000000000 ) ) ;
#13028=CARTESIAN_POINT ( 'NONE',  ( 4.458734125000000326, -54.14583333196773651, 2.574251347313718519 ) ) ;
#13030=CARTESIAN_POINT ( 'NONE',  ( 0.000000000000000000, -170.0000000000000000, 5.000000000000000000 ) ) ;
#13032=CARTESIAN_POINT ( 'NONE',  ( 5.000000000000000000, 22.50000000000000000, -6.123233995736766282E-16 ) ) ;
#13033=DIRECTION ( 'NONE',  ( 0.000000000000000000, 0.000000000000000000, 1.000000000000000000 ) ) ;
#13034=CARTESIAN_POINT ( 'NONE',  ( 9.457646018065525792E-16, -3.062499998634407472, 5.148502694627439702 ) ) ;
#13037=CARTESIAN_POINT ( 'NONE',  ( 1.975475456537005874E-15, -61.62499999726880162, 5.000000000000000000 ) ) ;
#13038=CARTESIAN_POINT ( 'NONE',  ( 4.458734124999998549, 12.02083333469892601, -2.574251347313721627 ) ) ;
#13039=VERTEX_POINT ( 'NONE', #10027 ) ;
#13041=EDGE_LOOP ( 'NONE', ( #60524, #12428, #390, #62795 ) ) ;
#13042=AXIS2_PLACEMENT_3D ( 'NONE', #24851, #5548, #15195 ) ;
#13043=CARTESIAN_POINT ( 'NONE',  ( 2.500000000000002220, -7.541666663935481907, 4.330127018922192761 ) ) ;
#13044=CARTESIAN_POINT ( 'NONE',  ( 9.457646018065525792E-16, -50.06249999863440792, 5.148502694627439702 ) ) ;
#13045=CARTESIAN_POINT ( 'NONE',  ( -4.458734125000000326, -161.2500000013655779, -1.846868145590735644 ) ) ;
#13048=CARTESIAN_POINT ( 'NONE',  ( -2.499999999999996447, -46.70833333060214443, 4.330127018922195425 ) ) ;
#13049=EDGE_LOOP ( 'NONE', ( #57588, #10803, #15964, #3098 ) ) ;
#13050=CARTESIAN_POINT ( 'NONE',  ( -3.152548672688508926E-16, -23.56249999863440436, -5.148502694627439702 ) ) ;
#13051=ORIENTED_EDGE ( 'NONE', *, *, #36926, .T. ) ;
#13053=CARTESIAN_POINT ( 'NONE',  ( 4.458734125000000326, -162.3750000013655779, -1.846868145590734978 ) ) ;
#13056=CARTESIAN_POINT ( 'NONE',  ( -4.458734124999999437, -35.56249999863440792, 0.000000000000000000 ) ) ;
#13061=CARTESIAN_POINT ( 'NONE',  ( 2.499999999999998668, -59.33333333333333570, -4.330127018922193649 ) ) ;
#13062=EDGE_LOOP ( 'NONE', ( #13584, #24492, #53380, #7971 ) ) ;
#13063=CARTESIAN_POINT ( 'NONE',  ( -1.339745962155613812, -60.08034179853027723, -5.000000000000000000 ) ) ;
#13065=CARTESIAN_POINT ( 'NONE',  ( 2.229367062500001939, -88.22916666530107932, 3.861377020970579999 ) ) ;
#13068=CARTESIAN_POINT ( 'NONE',  ( -4.999999999999998224, -6.916666666666667851, 2.886751345948131764 ) ) ;
#13075=EDGE_CURVE ( 'NONE', #40991, #14611, #45665, .T. ) ;
#13078=CYLINDRICAL_SURFACE ( 'NONE', #13995, 5.000000000000000000 ) ;
#13080=CARTESIAN_POINT ( 'NONE',  ( 2.229367062499998831, -82.89583333196773651, -3.861377020970580887 ) ) ;
#13087=CARTESIAN_POINT ( 'NONE',  ( 3.535533905932736864, -166.2500000027312126, 3.535533905932738641 ) ) ;
#13089=CARTESIAN_POINT ( 'NONE',  ( -4.458734124999997661, 12.52083333469892601, 2.574251347313722516 ) ) ;
#13090=CARTESIAN_POINT ( 'NONE',  ( 0.000000000000000000, -170.0000000000000000, 0.000000000000000000 ) ) ;
#13093=AXIS2_PLACEMENT_3D ( 'NONE', #33255, #45592, #52875 ) ;
#13099=CARTESIAN_POINT ( 'NONE',  ( -2.229367062499996610, -10.14583333196773829, 3.861377020970582219 ) ) ;
#13102=ORIENTED_EDGE ( 'NONE', *, *, #2429, .T. ) ;
#13103=CARTESIAN_POINT ( 'NONE',  ( 9.457646018065525792E-16, -37.31249999863440792, 5.148502694627439702 ) ) ;
#13105=EDGE_CURVE ( 'NONE', #23654, #22858, #13602, .T. ) ;
#13106=CARTESIAN_POINT ( 'NONE',  ( 5.000000000000000000, 0.6250000027311873874, -6.123233995736766282E-16 ) ) ;
#13107=CARTESIAN_POINT ( 'NONE',  ( -4.999999999999998224, 10.08333333333333393, 2.886751345948131764 ) ) ;
#13110=CARTESIAN_POINT ( 'NONE',  ( 2.229367062500001939, 13.02083333469892779, 3.861377020970579999 ) ) ;
#13113=CARTESIAN_POINT ( 'NONE',  ( -4.458734124999999437, -81.56249999863440792, 0.000000000000000000 ) ) ;
#13115=CARTESIAN_POINT ( 'NONE',  ( 1.339745962155612702, -72.16965819600733312, -5.000000000000000000 ) ) ;
#13116=CARTESIAN_POINT ( 'NONE',  ( -2.499999999999996447, 19.29166666939785202, 4.330127018922195425 ) ) ;
#13117=ORIENTED_EDGE ( 'NONE', *, *, #23699, .F. ) ;
#13118=CARTESIAN_POINT ( 'NONE',  ( -2.500000000000000444, -66.16666666666667140, -4.330127018922193649 ) ) ;
#13121=CARTESIAN_POINT ( 'NONE',  ( -4.999999999999999112, -29.91666666666667140, 2.886751345948131764 ) ) ;
#13122=CARTESIAN_POINT ( 'NONE',  ( 9.457646018065525792E-16, -32.06249999863440792, 5.148502694627439702 ) ) ;
#13124=CARTESIAN_POINT ( 'NONE',  ( -5.000000000000000000, -29.87499999726881228, 0.000000000000000000 ) ) ;
#13125=CARTESIAN_POINT ( 'NONE',  ( 4.458734125000001214, -61.89583333196773651, 2.574251347313718519 ) ) ;
#13127=CARTESIAN_POINT ( 'NONE',  ( 2.500000000000002220, -62.54166666393547303, 4.330127018922192761 ) ) ;
#13128=CARTESIAN_POINT ( 'NONE',  ( -4.458734124999999437, -11.56249999863440792, 0.000000000000000000 ) ) ;
#13130=CARTESIAN_POINT ( 'NONE',  ( 1.060575238724906964E-15, -78.75000000000001421, 5.773502691896257311 ) ) ;
#13133=VECTOR ( 'NONE', #40021, 1000.000000000000000 ) ;
#13134=CARTESIAN_POINT ( 'NONE',  ( 5.000000000000000000, -75.29166666393547303, -2.886751345948129988 ) ) ;
#13136=VERTEX_POINT ( 'NONE', #38657 ) ;
#13138=CARTESIAN_POINT ( 'NONE',  ( 4.458734125000001214, -20.14583333196774007, 2.574251347313718519 ) ) ;
#13139=CARTESIAN_POINT ( 'NONE',  ( -4.458734124999998549, -56.47916666530107221, 2.574251347313722516 ) ) ;
#13142=CARTESIAN_POINT ( 'NONE',  ( 3.152801135295366208, -139.5625000013655779, 3.152801135295367985 ) ) ;
#13144=VERTEX_POINT ( 'NONE', #14529 ) ;
#13150=CARTESIAN_POINT ( 'NONE',  ( 2.730187237215162345E-16, -148.4375000013656063, -4.458734124999999437 ) ) ;
#13154=CARTESIAN_POINT ( 'NONE',  ( -3.152548672688508926E-16, -64.81249999863440792, -5.148502694627439702 ) ) ;
#13157=CARTESIAN_POINT ( 'NONE',  ( -3.152801135295367985, -140.8125000013655779, 3.152801135295367096 ) ) ;
#13159=ORIENTED_EDGE ( 'NONE', *, *, #15760, .T. ) ;
#13160=CARTESIAN_POINT ( 'NONE',  ( -2.071067811865415109, -164.4375000027311557, 5.000000000000062172 ) ) ;
#13161=CARTESIAN_POINT ( 'NONE',  ( -6.972266317189433020E-16, 16.74999999999999645, -5.000000000000000000 ) ) ;
#13166=CARTESIAN_POINT ( 'NONE',  ( 4.458734124999999437, 25.93750000136559564, -5.460374474430324690E-16 ) ) ;
#13167=DIRECTION ( 'NONE',  ( -0.000000000000000000, 1.000000000000000000, -0.000000000000000000 ) ) ;
#13172=CARTESIAN_POINT ( 'NONE',  ( 1.975475456537005874E-15, -43.62499999726880873, 5.000000000000000000 ) ) ;
#13173=CARTESIAN_POINT ( 'NONE',  ( 9.457646018065525792E-16, 6.937500001365595637, 5.148502694627439702 ) ) ;
#13175=CARTESIAN_POINT ( 'NONE',  ( 4.458734124999998549, -17.97916666530106866, -2.574251347313721627 ) ) ;
#13176=( BOUNDED_CURVE ( )  B_SPLINE_CURVE ( 2, ( #18196, #12732, #28471, #48398, #51978, #53233, #32669, #28155, #38132 ),
 .UNSPECIFIED., .F., .F. ) 
 B_SPLINE_CURVE_WITH_KNOTS ( ( 3, 2, 2, 2, 3 ),
 ( 0.8749999999999998890, 0.8791666666666665408, 0.8833333333333330817, 0.8874999999999997335, 0.8916666666666664964 ),
 .UNSPECIFIED. ) 
 CURVE ( )  GEOMETRIC_REPRESENTATION_ITEM ( )  RATIONAL_B_SPLINE_CURVE ( ( 1.000000000000001998, 0.9238795325112847401, 1.000000000000000000, 0.9238795325112867385, 1.000000000000000000, 0.9238795325112867385, 1.000000000000000000, 0.9238795325112908463, 0.9999999999999958922 ) ) 
 REPRESENTATION_ITEM ( '' )  );
#13179=CARTESIAN_POINT ( 'NONE',  ( -1.846868145590737420, -158.7500000013656063, 4.458734124999999437 ) ) ;
#13180=CARTESIAN_POINT ( 'NONE',  ( -2.498395430326213474E-14, 15.37500000273118239, 5.000000000000000000 ) ) ;
#13183=CARTESIAN_POINT ( 'NONE',  ( 4.458734124999998549, -38.72916666530106511, -2.574251347313721627 ) ) ;
#13186=CARTESIAN_POINT ( 'NONE',  ( -4.458734124999997661, -68.47916666530107932, 2.574251347313722516 ) ) ;
#13188=DIRECTION ( 'NONE',  ( -0.000000000000000000, 1.000000000000000000, -0.000000000000000000 ) ) ;
#13189=CARTESIAN_POINT ( 'NONE',  ( 2.500000000000002220, -36.54166666393547303, 4.330127018922192761 ) ) ;
#13190=VERTEX_POINT ( 'NONE', #63443 ) ;
#13191=CARTESIAN_POINT ( 'NONE',  ( -5.000000000000000000, 15.12500000273118417, 0.000000000000000000 ) ) ;
#13192=CARTESIAN_POINT ( 'NONE',  ( -6.972266317189433020E-16, -68.12499999726881583, -5.000000000000000000 ) ) ;
#13193=CARTESIAN_POINT ( 'NONE',  ( -2.500000000000000444, -11.16666666666666430, -4.330127018922193649 ) ) ;
#13194=CARTESIAN_POINT ( 'NONE',  ( -2.229367062500000163, -14.47916666530107221, -3.861377020970580443 ) ) ;
#13195=CARTESIAN_POINT ( 'NONE',  ( -4.458734124999997661, -75.22916666530106511, 2.574251347313722516 ) ) ;
#13197=CARTESIAN_POINT ( 'NONE',  ( 2.499999999999998668, -59.20833333060214443, -4.330127018922193649 ) ) ;
#13198=CARTESIAN_POINT ( 'NONE',  ( -2.500000000000000444, -12.04166666393547835, -4.330127018922193649 ) ) ;
#13199=CARTESIAN_POINT ( 'NONE',  ( -3.152548672688508926E-16, -45.56249999863439371, -5.148502694627439702 ) ) ;
#13202=CARTESIAN_POINT ( 'NONE',  ( 2.229367062499998831, 6.104166668032262599, -3.861377020970580887 ) ) ;
#13204=CARTESIAN_POINT ( 'NONE',  ( 5.000000000000000888, -81.58333333333332860, 2.886751345948126879 ) ) ;
#13205=CARTESIAN_POINT ( 'NONE',  ( 5.000000000000000000, -62.50000000000000000, -6.123233995736766282E-16 ) ) ;
#13206=CARTESIAN_POINT ( 'NONE',  ( -4.458734125000001214, -162.1250000013655779, 1.846868145590734089 ) ) ;
#13209=CARTESIAN_POINT ( 'NONE',  ( -2.229367062499996610, -79.14583333196773651, 3.861377020970582219 ) ) ;
#13210=CARTESIAN_POINT ( 'NONE',  ( -3.535533905932737309, -164.6250000000000284, -3.535533905932738197 ) ) ;
#13213=CARTESIAN_POINT ( 'NONE',  ( 2.229367062500001939, -4.229166665301070438, 3.861377020970579999 ) ) ;
#13214=CARTESIAN_POINT ( 'NONE',  ( -4.458734124999999437, -42.64583333196773651, -2.574251347313719407 ) ) ;
#13217=CARTESIAN_POINT ( 'NONE',  ( -2.499999999999996447, 16.29166666939785202, 4.330127018922195425 ) ) ;
#13218=VERTEX_POINT ( 'NONE', #63129 ) ;
#13220=( BOUNDED_CURVE ( )  B_SPLINE_CURVE ( 2, ( #6449, #26058, #50506, #20918, #21232, #55658, #16725, #30226, #40838 ),
 .UNSPECIFIED., .F., .F. ) 
 B_SPLINE_CURVE_WITH_KNOTS ( ( 3, 2, 2, 2, 3 ),
 ( 0.7645833333333332815, 0.7652777777777777235, 0.7666666666666667185, 0.7680555555555556024, 0.7687500000000000444 ),
 .UNSPECIFIED. ) 
 CURVE ( )  GEOMETRIC_REPRESENTATION_ITEM ( )  RATIONAL_B_SPLINE_CURVE ( ( 0.9330127018922194093, 0.9330127018922194093, 1.000000000000000000, 0.8660254037844387076, 1.000000000000000000, 0.8660254037844387076, 1.000000000000000000, 0.9330127018922194093, 0.9330127018922194093 ) ) 
 REPRESENTATION_ITEM ( '' )  );
#13221=FACE_OUTER_BOUND ( 'NONE', #21755, .T. ) ;
#13222=CARTESIAN_POINT ( 'NONE',  ( 4.458734124999999437, -69.06249999863439371, -5.460374474430324690E-16 ) ) ;
#13224=CARTESIAN_POINT ( 'NONE',  ( -3.152801135295367096, -145.3125000013655779, -3.152801135295367541 ) ) ;
#13225=ORIENTED_EDGE ( 'NONE', *, *, #3241, .F. ) ;
#13226=DIRECTION ( 'NONE',  ( -0.000000000000000000, 1.000000000000000000, -0.000000000000000000 ) ) ;
#13229=CARTESIAN_POINT ( 'NONE',  ( 4.458734124999999437, 1.187500001365596081, -5.460374474430324690E-16 ) ) ;
#13231=CARTESIAN_POINT ( 'NONE',  ( -8.190561711645485556E-16, -158.6875000013655779, 4.458734124999999437 ) ) ;
#13238=DIRECTION ( 'NONE',  ( -0.000000000000000000, 1.000000000000000000, -0.000000000000000000 ) ) ;
#13239=CARTESIAN_POINT ( 'NONE',  ( 1.975475456537005874E-15, -23.62499999726880873, 5.000000000000000000 ) ) ;
#13245=CARTESIAN_POINT ( 'NONE',  ( -4.458734124999999437, 21.68750000136559208, 0.000000000000000000 ) ) ;
#13247=CARTESIAN_POINT ( 'NONE',  ( 4.458734124999998549, -2.979166665301069106, -2.574251347313721627 ) ) ;
#13250=CARTESIAN_POINT ( 'NONE',  ( -2.071067811865478170, -140.4375000027312126, 5.000000000000000000 ) ) ;
#13255=CYLINDRICAL_SURFACE ( 'NONE', #50, 5.000000000000000000 ) ;
#13256=DIRECTION ( 'NONE',  ( 0.000000000000000000, 0.000000000000000000, 1.000000000000000000 ) ) ;
#13258=CARTESIAN_POINT ( 'NONE',  ( -4.458734124999999437, -158.2500000013656063, -1.846868145590735644 ) ) ;
#13260=CARTESIAN_POINT ( 'NONE',  ( -9.184850993605147944E-16, -147.2500000000000284, 5.000000000000000000 ) ) ;
#13262=CARTESIAN_POINT ( 'NONE',  ( 2.229367062499998831, 17.10416666803225993, -3.861377020970580887 ) ) ;
#13269=CARTESIAN_POINT ( 'NONE',  ( 5.000000000000000888, 3.416666666666665186, 2.886751345948126879 ) ) ;
#13271=CARTESIAN_POINT ( 'NONE',  ( -4.458734124999999437, -61.39583333196774362, -2.574251347313719407 ) ) ;
#13272=FACE_OUTER_BOUND ( 'NONE', #1938, .T. ) ;
#13274=CARTESIAN_POINT ( 'NONE',  ( -2.229367062500000163, -29.47916666530107221, -3.861377020970580443 ) ) ;
#13276=CARTESIAN_POINT ( 'NONE',  ( -4.999999999999998224, 26.20833333606451632, 2.886751345948131764 ) ) ;
#13278=CARTESIAN_POINT ( 'NONE',  ( 5.000000000000000000, -39.49999999999999289, -6.123233995736766282E-16 ) ) ;
#13279=CARTESIAN_POINT ( 'NONE',  ( 5.000000000000000000, -70.37499999726880162, -6.123233995736766282E-16 ) ) ;
#13283=CARTESIAN_POINT ( 'NONE',  ( 4.458734124999998549, -62.72916666530106511, -2.574251347313721627 ) ) ;
#13284=CARTESIAN_POINT ( 'NONE',  ( -1.846868145590734756, -147.3750000013656063, -4.458734125000000326 ) ) ;
#13285=CARTESIAN_POINT ( 'NONE',  ( 4.458734124999998549, -75.72916666530106511, -2.574251347313721627 ) ) ;
#13288=CARTESIAN_POINT ( 'NONE',  ( -3.152548672688508926E-16, -26.81249999863440436, -5.148502694627439702 ) ) ;
#13289=CARTESIAN_POINT ( 'NONE',  ( 2.499999999999998668, -64.20833333060213022, -4.330127018922193649 ) ) ;
#13290=ORIENTED_EDGE ( 'NONE', *, *, #36629, .F. ) ;
#13291=CARTESIAN_POINT ( 'NONE',  ( 1.975475456537005874E-15, -1.749999999999999334, 5.000000000000000000 ) ) ;
#13292=ORIENTED_EDGE ( 'NONE', *, *, #36817, .F. ) ;
#13294=CARTESIAN_POINT ( 'NONE',  ( 3.535533905932736864, -149.2500000027311842, 3.535533905932738641 ) ) ;
#13298=CARTESIAN_POINT ( 'NONE',  ( -1.339745962155613812, -78.08034179853028434, -5.000000000000000000 ) ) ;
#13299=CARTESIAN_POINT ( 'NONE',  ( -2.229367062500000163, -55.72916666530107221, -3.861377020970580443 ) ) ;
#13301=( BOUNDED_CURVE ( )  B_SPLINE_CURVE ( 2, ( #8872, #27856, #13386, #32373, #38149, #62606, #61658, #57155, #61973 ),
 .UNSPECIFIED., .F., .F. ) 
 B_SPLINE_CURVE_WITH_KNOTS ( ( 3, 2, 2, 2, 3 ),
 ( 0.6312499999999999778, 0.6319444444444444198, 0.6333333333333333037, 0.6347222222222221877, 0.6354166666666666297 ),
 .UNSPECIFIED. ) 
 CURVE ( )  GEOMETRIC_REPRESENTATION_ITEM ( )  RATIONAL_B_SPLINE_CURVE ( ( 0.9330127018922194093, 0.9330127018922194093, 1.000000000000000000, 0.8660254037844387076, 1.000000000000000000, 0.8660254037844387076, 1.000000000000000000, 0.9330127018922194093, 0.9330127018922194093 ) ) 
 REPRESENTATION_ITEM ( '' )  );
#13302=EDGE_CURVE ( 'NONE', #55786, #13440, #3785, .T. ) ;
#13306=CARTESIAN_POINT ( 'NONE',  ( -3.152548672688508926E-16, 16.43750000136559564, -5.148502694627439702 ) ) ;
#13309=CARTESIAN_POINT ( 'NONE',  ( 5.000000000000000000, -165.0625000000000000, 2.071067811865478614 ) ) ;
#13313=DIRECTION ( 'NONE',  ( 0.000000000000000000, 1.000000000000000000, 0.000000000000000000 ) ) ;
#13315=EDGE_CURVE ( 'NONE', #61278, #15327, #15226, .T. ) ;
#13316=CARTESIAN_POINT ( 'NONE',  ( 1.975475456537005874E-15, -59.74999999999999289, 5.000000000000000000 ) ) ;
#13320=CARTESIAN_POINT ( 'NONE',  ( 6.123233995736766282E-16, -170.0000000000000000, -5.000000000000000000 ) ) ;
#13321=LINE ( 'NONE', #8498, #751 ) ;
#13322=CARTESIAN_POINT ( 'NONE',  ( -6.972266317189433020E-16, -57.12499999726880162, -5.000000000000000000 ) ) ;
#13328=CARTESIAN_POINT ( 'NONE',  ( -2.071067811865478170, -152.4375000027311842, 5.000000000000000000 ) ) ;
#13334=CARTESIAN_POINT ( 'NONE',  ( -5.000000000000000888, -148.4375000000000284, 2.071067811865474617 ) ) ;
#13335=EDGE_CURVE ( 'NONE', #59584, #50115, #32132, .T. ) ;
#13338=CARTESIAN_POINT ( 'NONE',  ( -1.846868145590734756, -168.3750000013655779, -4.458734124999999437 ) ) ;
#13339=CARTESIAN_POINT ( 'NONE',  ( 4.458734125000000326, -27.89583333196774007, 2.574251347313718519 ) ) ;
#13341=CARTESIAN_POINT ( 'NONE',  ( -5.000000000000000000, 9.041666669397853795, -2.886751345948128211 ) ) ;
#13343=CARTESIAN_POINT ( 'NONE',  ( 1.846868145590736310, -149.6250000013655779, 4.458734124999999437 ) ) ;
#13344=ORIENTED_EDGE ( 'NONE', *, *, #35407, .T. ) ;
#13346=CARTESIAN_POINT ( 'NONE',  ( -4.458734124999997661, -58.47916666530106511, 2.574251347313722516 ) ) ;
#13348=DIRECTION ( 'NONE',  ( -0.000000000000000000, 1.000000000000000000, -0.000000000000000000 ) ) ;
#13349=CARTESIAN_POINT ( 'NONE',  ( 2.500000000000002220, 16.33333333333333215, 4.330127018922192761 ) ) ;
#13351=CARTESIAN_POINT ( 'NONE',  ( -4.458734124999999437, -1.312499998634406140, 0.000000000000000000 ) ) ;
#13352=CARTESIAN_POINT ( 'NONE',  ( 0.000000000000000000, -170.0000000000000000, 5.000000000000000000 ) ) ;
#13354=CARTESIAN_POINT ( 'NONE',  ( 4.458734124999999437, 11.93750000136559564, -5.460374474430324690E-16 ) ) ;
#13358=CARTESIAN_POINT ( 'NONE',  ( -5.000000000000000000, -23.87499999726881228, 0.000000000000000000 ) ) ;
#13359=CARTESIAN_POINT ( 'NONE',  ( -2.229367062500000163, -48.47916666530106511, -3.861377020970580443 ) ) ;
#13360=CARTESIAN_POINT ( 'NONE',  ( 4.458734124999999437, -161.7500000013655495, 1.846868145590737864 ) ) ;
#13361=AXIS2_PLACEMENT_3D ( 'NONE', #18249, #23081, #47213 ) ;
#13363=CARTESIAN_POINT ( 'NONE',  ( -5.000000000000000000, -49.87499999726881583, 0.000000000000000000 ) ) ;
#13364=EDGE_CURVE ( 'NONE', #57658, #38838, #12793, .T. ) ;
#13366=CARTESIAN_POINT ( 'NONE',  ( 4.458734124999999437, -24.81249999863440436, -5.460374474430324690E-16 ) ) ;
#13369=CARTESIAN_POINT ( 'NONE',  ( 3.535533905932738197, -169.8750000000000284, -3.535533905932738197 ) ) ;
#13370=CARTESIAN_POINT ( 'NONE',  ( -1.846868145590734756, -162.1250000013655779, -4.458734125000000326 ) ) ;
#13371=( BOUNDED_CURVE ( )  B_SPLINE_CURVE ( 2, ( #48055, #42913, #18777, #42287, #32958, #62865, #61927, #17846, #58027, #13956, #37469, #52268, #62561, #32638, #4312, #13020, #8205, #27808, #47433, #23002, #42603, #13338, #53202, #9136, #62240, #18159, #37787, #28744, #28124, #57417, #48370, #47742, #23932, #19416, #34201, #44810, #54140, #25195, #39030, #44486, #24563, #59294, #4940, #34854, #29360, #45133, #58657, #44168, #9753, #43845, #14273, #33892, #49642, #53514, #49321, #15225, #20053, #5579, #25515, #447, #48993, #39979, #49956, #772, #9443, #135, #53824, #29052, #20706, #19729, #1097, #39657, #10402, #15557, #14579, #30014, #48676, #4616, #58345, #20379, #59625, #35177, #54795, #39342, #58973, #63491, #5265, #10723, #54475, #14900, #24241, #24885, #30330, #5908, #34509, #10079, #29690, #7184, #46723, #7498, #36764, #36126, #2668, #51249, #17140, #21335, #15872, #40935, #50919, #21018, #2050, #16186, #31613, #30658, #27110, #59949, #55110, #11035, #35813, #56392, #6861, #60268, #6225, #45453, #26792, #16505, #25837, #46412, #1419, #21658, #40625, #55437, #2361, #55748, #21970, #11353, #26476, #6541, #30975, #50599, #41249, #26154, #40311, #45773, #1731, #60585, #11665, #35492, #50280, #41563, #31284, #46090, #60895, #16819, #61214, #36438, #56068, #11987, #12320, #31931, #51559, #17467, #27733, #61854, #37089, #48292, #12940, #9062, #3620, #38023, #43150, #42208, #57655, #41889, #56707, #28672, #8753, #47979, #47361, #33200, #52815, #22613, #27415, #13258, #18709, #42841, #32563, #12626, #32882, #23552, #23227, #3309, #22930, #22290, #28358, #61535, #53130, #38334, #17771, #13884, #3933, #62790, #42524, #32242, #62161, #52510, #2996, #47668, #37390, #13581, #51871, #18402, #8445, #28048, #57963, #18081, #7813, #37704, #62484, #33512, #47046, #57025, #52185, #8130, #57342, #63108, #24487, #59221, #19019, #38632, #54398, #49247, #23859, #43774, #58894, #24170, #59548, #30253, #4868, #14823, #34437, #54720, #34774, #10327, #28983, #15483, #35102, #5502, #10640, #5190, #44410, #63420, #29938, #29289, #371, #24806, #4244, #15153, #19976, #14506, #39584, #58275, #14194, #49564, #9372, #48606, #39903, #20302, #33819, #25118, #19338, #48919, #44730, #54066, #44093, #43462, #53439, #57, #690, #4545, #38950, #9682, #58588, #34128, #53749, #19654, #39266, #10005, #29617, #22455, #10958, #56554, #5825, #1026, #52038, #27269, #46896, #40549, #32087, #51722, #42053, #15796, #7349, #17626, #61378, #1345, #20631, #26959, #61696, #17299, #60190, #16987, #7978, #7663, #49876, #25440, #56868, #25768, #32408, #37243, #12786, #12156, #40237, #31775, #2519, #50201, #36927, #45380, #2837, #45060, #59874, #12475, #35413, #55034, #30580, #6152, #20947, #36602, #56234, #51406, #46577, #22135, #41730, #8409, #23191, #14708, #42804, #20184, #28011, #44295, #15358, #62445, #34983, #59106, #18365, #37987, #57619, #257, #34327, #54598, #5390, #13546, #15033, #47628, #3584, #10520, #59429, #57307, #44615, #33167, #23515, #10213, #53952, #63618, #30134, #42485, #43972, #25005, #49763, #29816, #37664, #62124, #39469, #19539, #18041, #49448, #52781, #575, #5709, #9883, #13224, #5067, #8710, #39782, #32845, #52473, #28324, #47941, #3894, #39153, #58778, #29489, #49125, #24687, #19855, #34649, #54273, #40744, #25324, #6666, #46217, #51370, #21139, #15676, #12113, #60710, #60391, #16317, #31739, #36251, #2180, #56193, #55566, #11790, #30458, #6040, #35938, #51046, #11164, #21463, #35295, #36562, #16630, #40427, #35616, #55878, #902, #54915, #20826, #26273, #31408, #25645, #21785, #10842, #45261, #11481, #1227, #41377, #50083, #45895, #61023, #60067, #16949, #41063, #15991, #55242, #30786, #1857, #31101, #44944, #6989, #50409, #20509, #50722, #26601, #40108, #59751, #6357, #25961, #45578, #1534, #8557, #18528, #8254, #47475, #27230, #33006, #32371, #3429, #52319, #7311 ),
 .UNSPECIFIED., .F., .F. ) 
 B_SPLINE_CURVE_WITH_KNOTS ( ( 3, 2, 2, 2, 2, 2, 2, 2, 2, 2, 2, 2, 2, 2, 2, 2, 2, 2, 2, 2, 2, 2, 2, 2, 2, 2, 2, 2, 2, 2, 2, 2, 2, 2, 2, 2, 2, 2, 2, 2, 2, 2, 2, 2, 2, 2, 2, 2, 2, 2, 2, 2, 2, 2, 2, 2, 2, 2, 2, 2, 2, 2, 2, 2, 2, 2, 2, 2, 2, 2, 2, 2, 2, 2, 2, 2, 2, 2, 2, 2, 2, 2, 2, 2, 2, 2, 2, 2, 2, 2, 2, 2, 2, 2, 2, 2, 2, 2, 2, 2, 2, 2, 2, 2, 2, 2, 2, 2, 2, 2, 2, 2, 2, 2, 2, 2, 2, 2, 2, 2, 2, 2, 2, 2, 2, 2, 2, 2, 2, 2, 2, 2, 2, 2, 2, 2, 2, 2, 2, 2, 2, 2, 2, 2, 2, 2, 2, 2, 2, 2, 2, 2, 2, 2, 2, 2, 2, 2, 2, 2, 2, 2, 2, 2, 2, 2, 2, 2, 2, 2, 2, 2, 2, 2, 2, 2, 2, 2, 2, 2, 2, 2, 2, 2, 2, 2, 2, 2, 2, 2, 2, 2, 2, 2, 2, 2, 2, 2, 2, 2, 2, 2, 2, 2, 2, 2, 2, 2, 2, 2, 2, 2, 2, 2, 2, 2, 2, 2, 2, 2, 2, 2, 2, 2, 2, 2, 2, 2, 2, 2, 2, 2, 2, 2, 2, 2, 2, 2, 2, 2, 3 ),
 ( 0.000000000000000000, 0.004166666666666666609, 0.008333333333333333218, 0.01250000000000000069, 0.01666666666666666644, 0.02083333333333333218, 0.02500000000000000139, 0.02916666666666666713, 0.03333333333333333287, 0.03749999999999999861, 0.04166666666666666435, 0.04583333333333333010, 0.05000000000000000278, 0.05416666666666666852, 0.05833333333333333426, 0.06250000000000000000, 0.06666666666666666574, 0.07083333333333333148, 0.07499999999999999722, 0.07916666666666666297, 0.08333333333333332871, 0.08749999999999999445, 0.09166666666666666019, 0.09583333333333333981, 0.1000000000000000056, 0.1041666666666666713, 0.1083333333333333370, 0.1125000000000000028, 0.1166666666666666685, 0.1208333333333333343, 0.1250000000000000000, 0.1291666666666666796, 0.1333333333333333315, 0.1375000000000000111, 0.1416666666666666630, 0.1458333333333333426, 0.1499999999999999944, 0.1541666666666666741, 0.1583333333333333259, 0.1625000000000000056, 0.1666666666666666574, 0.1708333333333333370, 0.1749999999999999889, 0.1791666666666666685, 0.1833333333333333204, 0.1875000000000000000, 0.1916666666666666796, 0.1958333333333333315, 0.2000000000000000111, 0.2041666666666666630, 0.2083333333333333426, 0.2124999999999999944, 0.2166666666666666741, 0.2208333333333333259, 0.2250000000000000056, 0.2291666666666666574, 0.2333333333333333370, 0.2374999999999999889, 0.2416666666666666685, 0.2458333333333333204, 0.2500000000000000000, 0.2541666666666666519, 0.2583333333333333592, 0.2625000000000000111, 0.2666666666666666630, 0.2708333333333333148, 0.2750000000000000222, 0.2791666666666666741, 0.2833333333333333259, 0.2874999999999999778, 0.2916666666666666852, 0.2958333333333333370, 0.2999999999999999889, 0.3041666666666666408, 0.3083333333333333481, 0.3125000000000000000, 0.3166666666666666519, 0.3208333333333333592, 0.3250000000000000111, 0.3291666666666666630, 0.3333333333333333148, 0.3375000000000000222, 0.3416666666666666741, 0.3458333333333333259, 0.3499999999999999778, 0.3541666666666666852, 0.3583333333333333370, 0.3624999999999999889, 0.3666666666666666408, 0.3708333333333333481, 0.3750000000000000000, 0.3791666666666666519, 0.3833333333333333592, 0.3875000000000000111, 0.3916666666666666630, 0.3958333333333333148, 0.4000000000000000222, 0.4041666666666666741, 0.4083333333333333259, 0.4124999999999999778, 0.4166666666666666852, 0.4208333333333333370, 0.4249999999999999889, 0.4291666666666666408, 0.4333333333333333481, 0.4375000000000000000, 0.4416666666666666519, 0.4458333333333333592, 0.4500000000000000111, 0.4541666666666666630, 0.4583333333333333148, 0.4625000000000000222, 0.4666666666666666741, 0.4708333333333333259, 0.4749999999999999778, 0.4791666666666666852, 0.4833333333333333370, 0.4874999999999999889, 0.4916666666666666408, 0.4958333333333333481, 0.5000000000000000000, 0.5041666666666666519, 0.5083333333333333037, 0.5124999999999999556, 0.5166666666666667185, 0.5208333333333333703, 0.5250000000000000222, 0.5291666666666666741, 0.5333333333333333259, 0.5374999999999999778, 0.5416666666666666297, 0.5458333333333332815, 0.5500000000000000444, 0.5541666666666666963, 0.5583333333333333481, 0.5625000000000000000, 0.5666666666666666519, 0.5708333333333333037, 0.5749999999999999556, 0.5791666666666667185, 0.5833333333333333703, 0.5875000000000000222, 0.5916666666666666741, 0.5958333333333333259, 0.5999999999999999778, 0.6041666666666666297, 0.6083333333333332815, 0.6125000000000000444, 0.6166666666666666963, 0.6208333333333333481, 0.6250000000000000000, 0.6291666666666666519, 0.6333333333333333037, 0.6374999999999999556, 0.6416666666666667185, 0.6458333333333333703, 0.6500000000000000222, 0.6541666666666666741, 0.6583333333333333259, 0.6624999999999999778, 0.6666666666666666297, 0.6708333333333332815, 0.6750000000000000444, 0.6791666666666666963, 0.6833333333333333481, 0.6875000000000000000, 0.6916666666666666519, 0.6958333333333333037, 0.6999999999999999556, 0.7041666666666667185, 0.7083333333333333703, 0.7125000000000000222, 0.7166666666666666741, 0.7208333333333333259, 0.7249999999999999778, 0.7291666666666666297, 0.7333333333333332815, 0.7375000000000000444, 0.7416666666666666963, 0.7458333333333333481, 0.7500000000000000000, 0.7541666666666666519, 0.7583333333333333037, 0.7624999999999999556, 0.7666666666666667185, 0.7708333333333333703, 0.7750000000000000222, 0.7791666666666666741, 0.7833333333333333259, 0.7874999999999999778, 0.7916666666666666297, 0.7958333333333332815, 0.8000000000000000444, 0.8041666666666666963, 0.8083333333333333481, 0.8125000000000000000, 0.8166666666666666519, 0.8208333333333333037, 0.8249999999999999556, 0.8291666666666667185, 0.8333333333333333703, 0.8375000000000000222, 0.8416666666666666741, 0.8458333333333333259, 0.8499999999999999778, 0.8541666666666666297, 0.8583333333333332815, 0.8625000000000000444, 0.8666666666666666963, 0.8708333333333333481, 0.8750000000000000000, 0.8791666666666666519, 0.8833333333333333037, 0.8874999999999999556, 0.8916666666666667185, 0.8958333333333333703, 0.9000000000000000222, 0.9041666666666666741, 0.9083333333333333259, 0.9124999999999999778, 0.9166666666666666297, 0.9208333333333332815, 0.9250000000000000444, 0.9291666666666666963, 0.9333333333333333481, 0.9375000000000000000, 0.9416666666666666519, 0.9458333333333333037, 0.9499999999999999556, 0.9541666666666667185, 0.9583333333333333703, 0.9625000000000000222, 0.9666666666666666741, 0.9708333333333333259, 0.9749999999999999778, 0.9791666666666666297, 0.9833333333333332815, 0.9875000000000000444, 0.9916666666666666963, 0.9958333333333333481, 1.000000000000000000 ),
 .UNSPECIFIED. ) 
 CURVE ( )  GEOMETRIC_REPRESENTATION_ITEM ( )  RATIONAL_B_SPLINE_CURVE ( ( 1.000000000000000000, 0.9238795325112867385, 1.000000000000000000, 0.9238795325112867385, 1.000000000000000000, 0.9238795325112867385, 1.000000000000000000, 0.9238795325112867385, 1.000000000000000000, 0.9238795325112867385, 1.000000000000000000, 0.9238795325112867385, 1.000000000000000000, 0.9238795325112867385, 1.000000000000000000, 0.9238795325112867385, 1.000000000000000000, 0.9238795325112867385, 1.000000000000000000, 0.9238795325112867385, 1.000000000000000000, 0.9238795325112867385, 1.000000000000000000, 0.9238795325112867385, 1.000000000000000000, 0.9238795325112867385, 1.000000000000000000, 0.9238795325112867385, 1.000000000000000000, 0.9238795325112867385, 1.000000000000000000, 0.9238795325112867385, 1.000000000000000000, 0.9238795325112867385, 1.000000000000000000, 0.9238795325112867385, 1.000000000000000000, 0.9238795325112867385, 1.000000000000000000, 0.9238795325112867385, 1.000000000000000000, 0.9238795325112867385, 1.000000000000000000, 0.9238795325112867385, 1.000000000000000000, 0.9238795325112867385, 1.000000000000000000, 0.9238795325112867385, 1.000000000000000000, 0.9238795325112867385, 1.000000000000000000, 0.9238795325112867385, 1.000000000000000000, 0.9238795325112867385, 1.000000000000000000, 0.9238795325112867385, 1.000000000000000000, 0.9238795325112867385, 1.000000000000000000, 0.9238795325112867385, 1.000000000000000000, 0.9238795325112867385, 1.000000000000000000, 0.9238795325112867385, 1.000000000000000000, 0.9238795325112867385, 1.000000000000000000, 0.9238795325112867385, 1.000000000000000000, 0.9238795325112867385, 1.000000000000000000, 0.9238795325112867385, 1.000000000000000000, 0.9238795325112867385, 1.000000000000000000, 0.9238795325112867385, 1.000000000000000000, 0.9238795325112867385, 1.000000000000000000, 0.9238795325112867385, 1.000000000000000000, 0.9238795325112867385, 1.000000000000000000, 0.9238795325112867385, 1.000000000000000000, 0.9238795325112867385, 1.000000000000000000, 0.9238795325112867385, 1.000000000000000000, 0.9238795325112867385, 1.000000000000000000, 0.9238795325112867385, 1.000000000000000000, 0.9238795325112867385, 1.000000000000000000, 0.9238795325112867385, 1.000000000000000000, 0.9238795325112867385, 1.000000000000000000, 0.9238795325112867385, 1.000000000000000000, 0.9238795325112867385, 1.000000000000000000, 0.9238795325112867385, 1.000000000000000000, 0.9238795325112867385, 1.000000000000000000, 0.9238795325112867385, 1.000000000000000000, 0.9238795325112867385, 1.000000000000000000, 0.9238795325112867385, 1.000000000000000000, 0.9238795325112867385, 1.000000000000000000, 0.9238795325112867385, 1.000000000000000000, 0.9238795325112867385, 1.000000000000000000, 0.9238795325112867385, 1.000000000000000000, 0.9238795325112867385, 1.000000000000000000, 0.9238795325112867385, 1.000000000000000000, 0.9238795325112867385, 1.000000000000000000, 0.9238795325112867385, 1.000000000000000000, 0.9238795325112867385, 1.000000000000000000, 0.9238795325112867385, 1.000000000000000000, 0.9238795325112867385, 1.000000000000000000, 0.9238795325112867385, 1.000000000000000000, 0.9238795325112867385, 1.000000000000000000, 0.9238795325112867385, 1.000000000000000000, 0.9238795325112867385, 1.000000000000000000, 0.9238795325112867385, 1.000000000000000000, 0.9238795325112867385, 1.000000000000000000, 0.9238795325112867385, 1.000000000000000000, 0.9238795325112867385, 1.000000000000000000, 0.9238795325112867385, 1.000000000000000000, 0.9238795325112867385, 1.000000000000000000, 0.9238795325112867385, 1.000000000000000000, 0.9238795325112867385, 1.000000000000000000, 0.9238795325112867385, 1.000000000000000000, 0.9238795325112867385, 1.000000000000000000, 0.9238795325112867385, 1.000000000000000000, 0.9238795325112867385, 1.000000000000000000, 0.9238795325112867385, 1.000000000000000000, 0.9238795325112867385, 1.000000000000000000, 0.9238795325112867385, 1.000000000000000000, 0.9238795325112867385, 1.000000000000000000, 0.9238795325112867385, 1.000000000000000000, 0.9238795325112867385, 1.000000000000000000, 0.9238795325112867385, 1.000000000000000000, 0.9238795325112867385, 1.000000000000000000, 0.9238795325112867385, 1.000000000000000000, 0.9238795325112867385, 1.000000000000000000, 0.9238795325112867385, 1.000000000000000000, 0.9238795325112867385, 1.000000000000000000, 0.9238795325112867385, 1.000000000000000000, 0.9238795325112867385, 1.000000000000000000, 0.9238795325112867385, 1.000000000000000000, 0.9238795325112867385, 1.000000000000000000, 0.9238795325112867385, 1.000000000000000000, 0.9238795325112867385, 1.000000000000000000, 0.9238795325112867385, 1.000000000000000000, 0.9238795325112867385, 1.000000000000000000, 0.9238795325112867385, 1.000000000000000000, 0.9238795325112867385, 1.000000000000000000, 0.9238795325112867385, 1.000000000000000000, 0.9238795325112867385, 1.000000000000000000, 0.9238795325112867385, 1.000000000000000000, 0.9238795325112867385, 1.000000000000000000, 0.9238795325112867385, 1.000000000000000000, 0.9238795325112867385, 1.000000000000000000, 0.9238795325112867385, 1.000000000000000000, 0.9238795325112867385, 1.000000000000000000, 0.9238795325112867385, 1.000000000000000000, 0.9238795325112867385, 1.000000000000000000, 0.9238795325112867385, 1.000000000000000000, 0.9238795325112867385, 1.000000000000000000, 0.9238795325112867385, 1.000000000000000000, 0.9238795325112867385, 1.000000000000000000, 0.9238795325112867385, 1.000000000000000000, 0.9238795325112867385, 1.000000000000000000, 0.9238795325112867385, 1.000000000000000000, 0.9238795325112867385, 1.000000000000000000, 0.9238795325112867385, 1.000000000000000000, 0.9238795325112867385, 1.000000000000000000, 0.9238795325112867385, 1.000000000000000000, 0.9238795325112867385, 1.000000000000000000, 0.9238795325112867385, 1.000000000000000000, 0.9238795325112867385, 1.000000000000000000, 0.9238795325112867385, 1.000000000000000000, 0.9238795325112867385, 1.000000000000000000, 0.9238795325112867385, 1.000000000000000000, 0.9238795325112867385, 1.000000000000000000, 0.9238795325112867385, 1.000000000000000000, 0.9238795325112867385, 1.000000000000000000, 0.9238795325112867385, 1.000000000000000000, 0.9238795325112867385, 1.000000000000000000, 0.9238795325112867385, 1.000000000000000000, 0.9238795325112867385, 1.000000000000000000, 0.9238795325112867385, 1.000000000000000000, 0.9238795325112867385, 1.000000000000000000, 0.9238795325112867385, 1.000000000000000000, 0.9238795325112867385, 1.000000000000000000, 0.9238795325112867385, 1.000000000000000000, 0.9238795325112867385, 1.000000000000000000, 0.9238795325112867385, 1.000000000000000000, 0.9238795325112867385, 1.000000000000000000, 0.9238795325112867385, 1.000000000000000000, 0.9238795325112867385, 1.000000000000000000, 0.9238795325112867385, 1.000000000000000000, 0.9238795325112867385, 1.000000000000000000, 0.9238795325112867385, 1.000000000000000000, 0.9238795325112867385, 1.000000000000000000, 0.9238795325112867385, 1.000000000000000000, 0.9238795325112867385, 1.000000000000000000, 0.9238795325112867385, 1.000000000000000000, 0.9238795325112867385, 1.000000000000000000, 0.9238795325112867385, 1.000000000000000000, 0.9238795325112867385, 1.000000000000000000, 0.9238795325112867385, 1.000000000000000000, 0.9238795325112867385, 1.000000000000000000, 0.9238795325112867385, 1.000000000000000000, 0.9238795325112867385, 1.000000000000000000, 0.9238795325112867385, 1.000000000000000000, 0.9238795325112867385, 1.000000000000000000, 0.9238795325112867385, 1.000000000000000000, 0.9238795325112867385, 1.000000000000000000, 0.9238795325112867385, 1.000000000000000000, 0.9238795325112867385, 1.000000000000000000, 0.9238795325112867385, 1.000000000000000000, 0.9238795325112867385, 1.000000000000000000, 0.9238795325112867385, 1.000000000000000000, 0.9238795325112867385, 1.000000000000000000, 0.9238795325112867385, 1.000000000000000000, 0.9238795325112867385, 1.000000000000000000, 0.9238795325112867385, 1.000000000000000000, 0.9238795325112867385, 1.000000000000000000, 0.9238795325112867385, 1.000000000000000000, 0.9238795325112867385, 1.000000000000000000, 0.9238795325112867385, 1.000000000000000000, 0.9238795325112867385, 1.000000000000000000, 0.9238795325112867385, 1.000000000000000000, 0.9238795325112867385, 1.000000000000000000, 0.9238795325112867385, 1.000000000000000000, 0.9238795325112867385, 1.000000000000000000, 0.9238795325112867385, 1.000000000000000000, 0.9238795325112867385, 1.000000000000000000, 0.9238795325112867385, 1.000000000000000000, 0.9238795325112867385, 1.000000000000000000, 0.9238795325112867385, 1.000000000000000000, 0.9238795325112867385, 1.000000000000000000, 0.9238795325112867385, 1.000000000000000000, 0.9238795325112867385, 1.000000000000000000, 0.9238795325112867385, 1.000000000000000000, 0.9238795325112867385, 1.000000000000000000, 0.9238795325112867385, 1.000000000000000000, 0.9238795325112867385, 1.000000000000000000, 0.9238795325112867385, 1.000000000000000000, 0.9238795325112867385, 1.000000000000000000, 0.9238795325112867385, 1.000000000000000000, 0.9238795325112867385, 1.000000000000000000, 0.9238795325112867385, 1.000000000000000000, 0.9238795325112867385, 1.000000000000000000, 0.9238795325112867385, 1.000000000000000000, 0.9238795325112867385, 1.000000000000000000, 0.9238795325112867385, 1.000000000000000000, 0.9238795325112867385, 1.000000000000000000, 0.9238795325112867385, 1.000000000000000000, 0.9238795325112867385, 1.000000000000000000, 0.9238795325112867385, 1.000000000000000000, 0.9238795325112867385, 1.000000000000000000, 0.9238795325112867385, 1.000000000000000000, 0.9238795325112867385, 1.000000000000000000, 0.9238795325112867385, 1.000000000000000000, 0.9238795325112867385, 1.000000000000000000, 0.9238795325112867385, 1.000000000000000000, 0.9238795325112867385, 1.000000000000000000, 0.9238795325112867385, 1.000000000000000000, 0.9238795325112867385, 1.000000000000000000, 0.9238795325112867385, 1.000000000000000000, 0.9238795325112867385, 1.000000000000000000, 0.9238795325112867385, 1.000000000000000000, 0.9238795325112867385, 1.000000000000000000, 0.9238795325112867385, 1.000000000000000000, 0.9238795325112867385, 1.000000000000000000, 0.9238795325112867385, 1.000000000000000000, 0.9238795325112867385, 1.000000000000000000, 0.9238795325112867385, 1.000000000000000000, 0.9238795325112867385, 1.000000000000000000, 0.9238795325112867385, 1.000000000000000000, 0.9238795325112867385, 1.000000000000000000, 0.9238795325112867385, 1.000000000000000000, 0.9238795325112867385, 1.000000000000000000, 0.9238795325112867385, 1.000000000000000000, 0.9238795325112867385, 1.000000000000000000, 0.9238795325112867385, 1.000000000000000000, 0.9238795325112867385, 1.000000000000000000, 0.9238795325112867385, 1.000000000000000000, 0.9238795325112867385, 1.000000000000000000, 0.9238795325112867385, 1.000000000000000000 ) ) 
 REPRESENTATION_ITEM ( '' )  );
#13374=CARTESIAN_POINT ( 'NONE',  ( 4.458734124999999437, -40.06249999863440081, -5.460374474430324690E-16 ) ) ;
#13377=EDGE_CURVE ( 'NONE', #33297, #36444, #48096, .T. ) ;
#13380=ORIENTED_EDGE ( 'NONE', *, *, #63339, .T. ) ;
#13382=CARTESIAN_POINT ( 'NONE',  ( 2.229367062499998831, -85.89583333196773651, -3.861377020970580887 ) ) ;
#13385=CARTESIAN_POINT ( 'NONE',  ( 1.975475456537005874E-15, -6.749999999999999112, 5.000000000000000000 ) ) ;
#13386=CARTESIAN_POINT ( 'NONE',  ( -2.499999999999996447, -46.70833333060214443, 4.330127018922195425 ) ) ;
#13388=CARTESIAN_POINT ( 'NONE',  ( -2.499999999999996447, -84.70833333060214443, 4.330127018922195425 ) ) ;
#13394=DIRECTION ( 'NONE',  ( -0.000000000000000000, 1.000000000000000000, -0.000000000000000000 ) ) ;
#13396=CARTESIAN_POINT ( 'NONE',  ( 4.458734124999998549, -86.97916666530106511, -2.574251347313721627 ) ) ;
#13399=( BOUNDED_CURVE ( )  B_SPLINE_CURVE ( 2, ( #33879, #4300, #33568, #47725, #23296, #13636, #28729, #42896, #18464 ),
 .UNSPECIFIED., .F., .F. ) 
 B_SPLINE_CURVE_WITH_KNOTS ( ( 3, 2, 2, 2, 3 ),
 ( 0.4416666666666670404, 0.4458333333333337478, 0.4500000000000003997, 0.4541666666666671071, 0.4583333333333337589 ),
 .UNSPECIFIED. ) 
 CURVE ( )  GEOMETRIC_REPRESENTATION_ITEM ( )  RATIONAL_B_SPLINE_CURVE ( ( 0.9999999999999928946, 0.9238795325112938439, 1.000000000000000000, 0.9238795325112867385, 1.000000000000000000, 0.9238795325112867385, 1.000000000000000000, 0.9238795325112786339, 1.000000000000008216 ) ) 
 REPRESENTATION_ITEM ( '' )  );
#13402=CARTESIAN_POINT ( 'NONE',  ( -6.972266317189433020E-16, -81.24999999999998579, -5.000000000000000000 ) ) ;
#13404=CARTESIAN_POINT ( 'NONE',  ( -2.071067811865475061, -165.8125000027311842, -5.000000000000000888 ) ) ;
#13406=VECTOR ( 'NONE', #27670, 1000.000000000000000 ) ;
#13408=CARTESIAN_POINT ( 'NONE',  ( 1.975475456537005874E-15, -29.74999999999999645, 5.000000000000000000 ) ) ;
#13413=CARTESIAN_POINT ( 'NONE',  ( 0.000000000000000000, -170.0000000000000000, 5.000000000000000000 ) ) ;
#13414=CARTESIAN_POINT ( 'NONE',  ( -4.458734124999997661, -9.229166665301068662, 2.574251347313722516 ) ) ;
#13415=CARTESIAN_POINT ( 'NONE',  ( 0.000000000000000000, -170.0000000000000000, 0.000000000000000000 ) ) ;
#13416=VERTEX_POINT ( 'NONE', #1676 ) ;
#13417=CARTESIAN_POINT ( 'NONE',  ( 9.457646018065525792E-16, -38.31249999863440792, 5.148502694627439702 ) ) ;
#13423=CARTESIAN_POINT ( 'NONE',  ( -4.458734124999999437, 17.68750000136559208, 0.000000000000000000 ) ) ;
#13424=CARTESIAN_POINT ( 'NONE',  ( -6.972266317189433020E-16, -34.12499999726881583, -5.000000000000000000 ) ) ;
#13425=CARTESIAN_POINT ( 'NONE',  ( 1.339745962155615144, -55.70534180126148271, 4.999999999999999112 ) ) ;
#13426=CARTESIAN_POINT ( 'NONE',  ( 2.229367062499998831, -81.89583333196773651, -3.861377020970580887 ) ) ;
#13428=CARTESIAN_POINT ( 'NONE',  ( 2.500000000000002220, 14.45833333606451809, 4.330127018922192761 ) ) ;
#13431=CARTESIAN_POINT ( 'NONE',  ( -9.184850993605147944E-16, -149.3750000027312126, 5.000000000000000000 ) ) ;
#13433=CARTESIAN_POINT ( 'NONE',  ( 2.499999999999998668, -31.33333333333333215, -4.330127018922193649 ) ) ;
#13434=CARTESIAN_POINT ( 'NONE',  ( -2.229367062500000163, -31.47916666530107577, -3.861377020970580443 ) ) ;
#13436=EDGE_CURVE ( 'NONE', #3491, #57658, #10345, .T. ) ;
#13437=CARTESIAN_POINT ( 'NONE',  ( 5.000000000000000000, -30.37499999726881228, -6.123233995736766282E-16 ) ) ;
#13438=EDGE_CURVE ( 'NONE', #21932, #56335, #1732, .T. ) ;
#13439=CARTESIAN_POINT ( 'NONE',  ( 2.229367062499998831, -60.64583333196774362, -3.861377020970580887 ) ) ;
#13440=VERTEX_POINT ( 'NONE', #54741 ) ;
#13442=CARTESIAN_POINT ( 'NONE',  ( -3.152548672688508926E-16, -8.812499998634406140, -5.148502694627439702 ) ) ;
#13445=CARTESIAN_POINT ( 'NONE',  ( -2.499999999999996447, -74.83333333333332860, 4.330127018922195425 ) ) ;
#13447=VECTOR ( 'NONE', #9052, 1000.000000000000000 ) ;
#13450=CARTESIAN_POINT ( 'NONE',  ( 2.500000000000002220, -74.54166666393547303, 4.330127018922192761 ) ) ;
#13452=ORIENTED_EDGE ( 'NONE', *, *, #51863, .F. ) ;
#13453=AXIS2_PLACEMENT_3D ( 'NONE', #49653, #54805, #10734 ) ;
#13455=EDGE_CURVE ( 'NONE', #46822, #42419, #23507, .T. ) ;
#13456=CARTESIAN_POINT ( 'NONE',  ( 2.229367062500001939, -19.22916666530106866, 3.861377020970579999 ) ) ;
#13457=EDGE_CURVE ( 'NONE', #43823, #11304, #46359, .T. ) ;
#13458=CARTESIAN_POINT ( 'NONE',  ( 2.229367062499998831, -54.89583333196773651, -3.861377020970580887 ) ) ;
#13461=CARTESIAN_POINT ( 'NONE',  ( 3.152801135295367541, -166.5625000013656063, -3.152801135295367541 ) ) ;
#13463=CARTESIAN_POINT ( 'NONE',  ( -6.972266317189433020E-16, 17.75000000000000355, -5.000000000000000000 ) ) ;
#13465=EDGE_CURVE ( 'NONE', #15263, #61537, #45289, .T. ) ;
#13473=CARTESIAN_POINT ( 'NONE',  ( 2.730187237215162345E-16, -145.4375000013656063, -4.458734124999999437 ) ) ;
#13475=CARTESIAN_POINT ( 'NONE',  ( -6.972266317189433020E-16, -70.25000000000000000, -5.000000000000000000 ) ) ;
#13477=CARTESIAN_POINT ( 'NONE',  ( -2.229367062499996610, -70.39583333196773651, 3.861377020970582219 ) ) ;
#13480=CARTESIAN_POINT ( 'NONE',  ( 4.458734124999999437, -139.4375000013656063, 0.000000000000000000 ) ) ;
#13489=CARTESIAN_POINT ( 'NONE',  ( -4.458734124999999437, 25.35416666803225993, -2.574251347313719407 ) ) ;
#13490=CARTESIAN_POINT ( 'NONE',  ( -9.184850993605147944E-16, -157.3750000027311842, 5.000000000000000000 ) ) ;
#13491=( BOUNDED_CURVE ( )  B_SPLINE_CURVE ( 2, ( #29745, #45189, #831, #50012, #30717, #54200, #189, #10780, #31031 ),
 .UNSPECIFIED., .F., .F. ) 
 B_SPLINE_CURVE_WITH_KNOTS ( ( 3, 2, 2, 2, 3 ),
 ( 0.5937500000000000000, 0.5944444444444444420, 0.5958333333333333259, 0.5972222222222222099, 0.5979166666666666519 ),
 .UNSPECIFIED. ) 
 CURVE ( )  GEOMETRIC_REPRESENTATION_ITEM ( )  RATIONAL_B_SPLINE_CURVE ( ( 0.9330127018922194093, 0.9330127018922194093, 1.000000000000000000, 0.8660254037844387076, 1.000000000000000000, 0.8660254037844387076, 1.000000000000000000, 0.9330127018922194093, 0.9330127018922194093 ) ) 
 REPRESENTATION_ITEM ( '' )  );
#13496=CARTESIAN_POINT ( 'NONE',  ( 5.000000000000000000, -43.29166666393548013, -2.886751345948130876 ) ) ;
#13497=CARTESIAN_POINT ( 'NONE',  ( -4.458734124999999437, 4.687500001365595637, 0.000000000000000000 ) ) ;
#13499=CARTESIAN_POINT ( 'NONE',  ( 9.457646018065525792E-16, -21.31249999863440081, 5.148502694627439702 ) ) ;
#13501=CARTESIAN_POINT ( 'NONE',  ( -4.458734125000000326, -157.0000000013655779, -1.846868145590735644 ) ) ;
#13502=CARTESIAN_POINT ( 'NONE',  ( 5.000000000000000888, 23.41666666666666430, 2.886751345948126879 ) ) ;
#13508=CARTESIAN_POINT ( 'NONE',  ( -3.152548672688508926E-16, -40.56249999863440081, -5.148502694627439702 ) ) ;
#13511=CARTESIAN_POINT ( 'NONE',  ( 4.458734124999998549, -68.97916666530107932, -2.574251347313721627 ) ) ;
#13515=ORIENTED_EDGE ( 'NONE', *, *, #41414, .F. ) ;
#13518=CARTESIAN_POINT ( 'NONE',  ( 1.339745962155590275, 2.419658201469706782, 5.000000000000013323 ) ) ;
#13519=CARTESIAN_POINT ( 'NONE',  ( -3.535250795749689387E-16, -15.25000000000000000, -5.773502691896257311 ) ) ;
#13520=CARTESIAN_POINT ( 'NONE',  ( -3.152548672688508926E-16, -15.56249999863440614, -5.148502694627439702 ) ) ;
#13521=CARTESIAN_POINT ( 'NONE',  ( -4.458734124999999437, -75.31249999863440792, 0.000000000000000000 ) ) ;
#13523=CARTESIAN_POINT ( 'NONE',  ( -5.000000000000000000, -12.87499999726881050, 0.000000000000000000 ) ) ;
#13524=CARTESIAN_POINT ( 'NONE',  ( 2.229367062499998831, -46.64583333196774362, -3.861377020970580887 ) ) ;
#13525=ORIENTED_EDGE ( 'NONE', *, *, #58924, .T. ) ;
#13526=CARTESIAN_POINT ( 'NONE',  ( -2.229367062499996610, 7.604166668032260823, 3.861377020970582219 ) ) ;
#13527=ORIENTED_EDGE ( 'NONE', *, *, #14502, .T. ) ;
#13529=CARTESIAN_POINT ( 'NONE',  ( 2.500000000000002220, -58.66666666666665719, 4.330127018922192761 ) ) ;
#13530=CARTESIAN_POINT ( 'NONE',  ( -4.458734125000001214, -158.1250000013656063, 1.846868145590734089 ) ) ;
#13532=CARTESIAN_POINT ( 'NONE',  ( -1.339745962155610925, -64.79465819873851729, 5.000000000000000000 ) ) ;
#13533=CARTESIAN_POINT ( 'NONE',  ( -3.535533905932738641, -168.3750000000000284, 3.535533905932737309 ) ) ;
#13534=DIRECTION ( 'NONE',  ( -0.000000000000000000, 1.000000000000000000, -0.000000000000000000 ) ) ;
#13536=CARTESIAN_POINT ( 'NONE',  ( 9.457646018065525792E-16, -6.312499998634404363, 5.148502694627439702 ) ) ;
#13537=CARTESIAN_POINT ( 'NONE',  ( 2.229367062500001939, -40.22916666530107221, 3.861377020970579999 ) ) ;
#13539=CARTESIAN_POINT ( 'NONE',  ( 1.846868145590736310, -153.6250000013655779, 4.458734124999999437 ) ) ;
#13543=CARTESIAN_POINT ( 'NONE',  ( -2.071067811865562991, -141.3124999999999716, 4.999999999999913847 ) ) ;
#13544=CARTESIAN_POINT ( 'NONE',  ( 1.339745962155615144, -2.580341798530292774, 4.999999999999999112 ) ) ;
#13545=CARTESIAN_POINT ( 'NONE',  ( 4.458734124999999437, -70.06249999863439371, -5.460374474430324690E-16 ) ) ;
#13546=CARTESIAN_POINT ( 'NONE',  ( -4.458734125000000326, -147.1250000013656063, 1.846868145590734089 ) ) ;
#13552=CARTESIAN_POINT ( 'NONE',  ( 4.458734125000001214, 3.104166668032260379, 2.574251347313718519 ) ) ;
#13553=CARTESIAN_POINT ( 'NONE',  ( -6.972266317189433020E-16, -80.24999999999998579, -5.000000000000000000 ) ) ;
#13554=CARTESIAN_POINT ( 'NONE',  ( 1.846868145590735200, -153.2500000013656063, -4.458734124999999437 ) ) ;
#13555=( BOUNDED_CURVE ( )  B_SPLINE_CURVE ( 2, ( #35545, #44865, #26208, #6284, #50009, #51305, #7243, #31669, #828 ),
 .UNSPECIFIED., .F., .F. ) 
 B_SPLINE_CURVE_WITH_KNOTS ( ( 3, 2, 2, 2, 3 ),
 ( 0.3916666666666669960, 0.3958333333333336479, 0.4000000000000003553, 0.4041666666666670071, 0.4083333333333336590 ),
 .UNSPECIFIED. ) 
 CURVE ( )  GEOMETRIC_REPRESENTATION_ITEM ( )  RATIONAL_B_SPLINE_CURVE ( ( 0.9999999999999938938, 0.9238795325112928447, 1.000000000000000000, 0.9238795325112867385, 1.000000000000000000, 0.9238795325112867385, 1.000000000000000000, 0.9238795325112806323, 1.000000000000005995 ) ) 
 REPRESENTATION_ITEM ( '' )  );
#13564=CARTESIAN_POINT ( 'NONE',  ( 1.339745962155615144, -87.70534180126146850, 4.999999999999999112 ) ) ;
#13569=CARTESIAN_POINT ( 'NONE',  ( -2.229367062500000163, 22.52083333469892423, -3.861377020970580443 ) ) ;
#13571=CARTESIAN_POINT ( 'NONE',  ( -2.229367062500000163, -2.729166665301069550, -3.861377020970580443 ) ) ;
#13572=DIRECTION ( 'NONE',  ( -0.000000000000000000, 1.000000000000000000, -0.000000000000000000 ) ) ;
#13574=CARTESIAN_POINT ( 'NONE',  ( -3.535533905932738641, -139.5000000027311842, 3.535533905932737309 ) ) ;
#13575=CARTESIAN_POINT ( 'NONE',  ( 2.500000000000002220, -75.54166666393547303, 4.330127018922192761 ) ) ;
#13581=CARTESIAN_POINT ( 'NONE',  ( 4.458734124999999437, -156.6250000013655779, -1.846868145590734978 ) ) ;
#13584=ORIENTED_EDGE ( 'NONE', *, *, #49083, .T. ) ;
#13585=CARTESIAN_POINT ( 'NONE',  ( -2.229367062500000163, 19.27083333469892779, -3.861377020970580443 ) ) ;
#13590=CARTESIAN_POINT ( 'NONE',  ( 3.535533905932736864, -162.1250000000000284, 3.535533905932738641 ) ) ;
#13591=CARTESIAN_POINT ( 'NONE',  ( -2.500000000000000444, 4.833333333333332149, -4.330127018922193649 ) ) ;
#13592=CARTESIAN_POINT ( 'NONE',  ( 9.457646018065525792E-16, -60.06249999863440081, 5.148502694627439702 ) ) ;
#13594=CARTESIAN_POINT ( 'NONE',  ( 2.500000000000002220, 3.458333336064517205, 4.330127018922192761 ) ) ;
#13595=CARTESIAN_POINT ( 'NONE',  ( -4.458734124999999437, -27.31249999863440081, 0.000000000000000000 ) ) ;
#13598=CARTESIAN_POINT ( 'NONE',  ( -2.500000000000000444, -25.04166666393547658, -4.330127018922193649 ) ) ;
#13599=CARTESIAN_POINT ( 'NONE',  ( -5.000000000000000000, -45.00000000000000000, 0.000000000000000000 ) ) ;
#13602=LINE ( 'NONE', #62812, #60485 ) ;
#13603=CARTESIAN_POINT ( 'NONE',  ( 2.229367062500001939, -64.97916666530106511, 3.861377020970579999 ) ) ;
#13604=( BOUNDED_CURVE ( )  B_SPLINE_CURVE ( 2, ( #28958, #43750, #19312, #48896, #49538, #45355, #1631, #49851, #16086 ),
 .UNSPECIFIED., .F., .F. ) 
 B_SPLINE_CURVE_WITH_KNOTS ( ( 3, 2, 2, 2, 3 ),
 ( 0.7083333333333329263, 0.7124999999999995781, 0.7166666666666663410, 0.7208333333333329929, 0.7249999999999996447 ),
 .UNSPECIFIED. ) 
 CURVE ( )  GEOMETRIC_REPRESENTATION_ITEM ( )  RATIONAL_B_SPLINE_CURVE ( ( 1.000000000000008216, 0.9238795325112786339, 1.000000000000000000, 0.9238795325112867385, 1.000000000000000000, 0.9238795325112867385, 1.000000000000000000, 0.9238795325112928447, 0.9999999999999938938 ) ) 
 REPRESENTATION_ITEM ( '' )  );
#13605=CARTESIAN_POINT ( 'NONE',  ( 2.730187237215162345E-16, -146.4375000013656063, -4.458734124999999437 ) ) ;
#13606=CARTESIAN_POINT ( 'NONE',  ( 4.458734124999999437, -75.81249999863440792, -5.460374474430324690E-16 ) ) ;
#13608=CARTESIAN_POINT ( 'NONE',  ( -3.152548672688508926E-16, -25.81249999863440792, -5.148502694627439702 ) ) ;
#13609=CARTESIAN_POINT ( 'NONE',  ( -2.499999999999996447, -64.70833333060213022, 4.330127018922195425 ) ) ;
#13612=ORIENTED_EDGE ( 'NONE', *, *, #9177, .F. ) ;
#13614=CARTESIAN_POINT ( 'NONE',  ( 0.000000000000000000, -170.0000000000000000, 5.000000000000000000 ) ) ;
#13616=VERTEX_POINT ( 'NONE', #56018 ) ;
#13617=LINE ( 'NONE', #28399, #33249 ) ;
#13618=CARTESIAN_POINT ( 'NONE',  ( 4.458734124999999437, -52.06249999863440792, -5.460374474430324690E-16 ) ) ;
#13620=ORIENTED_EDGE ( 'NONE', *, *, #7436, .F. ) ;
#13623=CARTESIAN_POINT ( 'NONE',  ( -2.229367062499996610, 16.85416666803225993, 3.861377020970582219 ) ) ;
#13625=CARTESIAN_POINT ( 'NONE',  ( 2.626220312808019583E-14, 20.87500000273118062, -5.000000000000000000 ) ) ;
#13626=CARTESIAN_POINT ( 'NONE',  ( -4.458734124999999437, -164.9375000013655779, -5.460374474430324690E-16 ) ) ;
#13627=ORIENTED_EDGE ( 'NONE', *, *, #10235, .F. ) ;
#13631=DIRECTION ( 'NONE',  ( 0.000000000000000000, 0.000000000000000000, 1.000000000000000000 ) ) ;
#13635=CARTESIAN_POINT ( 'NONE',  ( -6.972266317189433020E-16, -73.25000000000000000, -5.000000000000000000 ) ) ;
#13636=CARTESIAN_POINT ( 'NONE',  ( -5.000000000000000888, -156.4374999999999716, 2.071067811865474617 ) ) ;
#13640=DIRECTION ( 'NONE',  ( 0.000000000000000000, 0.000000000000000000, 1.000000000000000000 ) ) ;
#13642=CARTESIAN_POINT ( 'NONE',  ( 3.061616997868383141E-16, -151.8750000027311842, -5.000000000000000000 ) ) ;
#13645=EDGE_CURVE ( 'NONE', #59659, #54895, #56343, .T. ) ;
#13649=CARTESIAN_POINT ( 'NONE',  ( 5.000000000000000000, -142.0000000000000284, 0.000000000000000000 ) ) ;
#13652=CARTESIAN_POINT ( 'NONE',  ( -5.000000000000000000, -54.99999999999999289, 0.000000000000000000 ) ) ;
#13653=CARTESIAN_POINT ( 'NONE',  ( 4.458734124999999437, -28.81249999863440436, -5.460374474430324690E-16 ) ) ;
#13657=CARTESIAN_POINT ( 'NONE',  ( -4.458734125000001214, -148.8750000013655495, 1.846868145590734089 ) ) ;
#13660=CARTESIAN_POINT ( 'NONE',  ( 2.229367062500001939, -59.22916666530106511, 3.861377020970579999 ) ) ;
#13663=CARTESIAN_POINT ( 'NONE',  ( 5.000000000000000000, 19.58333333333333215, -2.886751345948129988 ) ) ;
#13664=CYLINDRICAL_SURFACE ( 'NONE', #45867, 5.000000000000000000 ) ;
#13665=CARTESIAN_POINT ( 'NONE',  ( 2.229367062500001939, 1.020833334698927120, 3.861377020970579999 ) ) ;
#13667=CARTESIAN_POINT ( 'NONE',  ( -5.147856630858197489E-14, 4.249999999999996447, 5.000000000000000000 ) ) ;
#13668=CARTESIAN_POINT ( 'NONE',  ( 4.458734124999999437, 8.937500001365592084, -5.460374474430324690E-16 ) ) ;
#13669=CARTESIAN_POINT ( 'NONE',  ( 6.123233995736766282E-16, -170.0000000000000000, -5.000000000000000000 ) ) ;
#13672=CARTESIAN_POINT ( 'NONE',  ( 4.458734125000001214, -49.89583333196772941, 2.574251347313718519 ) ) ;
#13673=CARTESIAN_POINT ( 'NONE',  ( -1.846868145590737420, -160.0000000013656063, 4.458734124999999437 ) ) ;
#13674=( BOUNDED_CURVE ( )  B_SPLINE_CURVE ( 2, ( #37051, #41534, #62129, #18047, #51838, #27384, #42492, #22582, #2329 ),
 .UNSPECIFIED., .F., .F. ) 
 B_SPLINE_CURVE_WITH_KNOTS ( ( 3, 2, 2, 2, 3 ),
 ( 0.2229166666666666796, 0.2236111111111111216, 0.2250000000000000056, 0.2263888888888888895, 0.2270833333333333315 ),
 .UNSPECIFIED. ) 
 CURVE ( )  GEOMETRIC_REPRESENTATION_ITEM ( )  RATIONAL_B_SPLINE_CURVE ( ( 0.9330127018922194093, 0.9330127018922207416, 1.000000000000000000, 0.8660254037844387076, 1.000000000000000000, 0.8660254037844387076, 1.000000000000000000, 0.9330127018922194093, 0.9330127018922194093 ) ) 
 REPRESENTATION_ITEM ( '' )  );
#13675=CARTESIAN_POINT ( 'NONE',  ( -3.535250795749689387E-16, -52.12499999726881583, -5.773502691896257311 ) ) ;
#13676=ORIENTED_EDGE ( 'NONE', *, *, #59964, .T. ) ;
#13677=CARTESIAN_POINT ( 'NONE',  ( -2.229367062500000163, -21.47916666530107221, -3.861377020970580443 ) ) ;
#13678=VERTEX_POINT ( 'NONE', #6810 ) ;
#13680=CARTESIAN_POINT ( 'NONE',  ( 5.000000000000000888, -169.9375000000000284, -2.071067811865475505 ) ) ;
#13681=CARTESIAN_POINT ( 'NONE',  ( -3.152801135295367096, -161.0625000013656063, -3.152801135295367541 ) ) ;
#13683=CARTESIAN_POINT ( 'NONE',  ( -6.972266317189433020E-16, -35.25000000000000000, -5.000000000000000000 ) ) ;
#13685=CARTESIAN_POINT ( 'NONE',  ( -2.229367062499996610, -38.39583333196773651, 3.861377020970582219 ) ) ;
#13689=CARTESIAN_POINT ( 'NONE',  ( 5.000000000000000888, -24.45833333060214798, 2.886751345948126879 ) ) ;
#13692=CARTESIAN_POINT ( 'NONE',  ( -2.229367062500000163, -86.72916666530107932, -3.861377020970580443 ) ) ;
#13704=CARTESIAN_POINT ( 'NONE',  ( -4.999999999999998224, -60.91666666666666430, 2.886751345948131764 ) ) ;
#13705=CARTESIAN_POINT ( 'NONE',  ( -4.458734124999998549, -85.47916666530106511, 2.574251347313722516 ) ) ;
#13710=CARTESIAN_POINT ( 'NONE',  ( 5.000000000000000000, -167.1875000027312410, 2.071067811865478614 ) ) ;
#13714=CARTESIAN_POINT ( 'NONE',  ( -4.999999999999998224, -29.91666666666667140, 2.886751345948131764 ) ) ;
#13721=CARTESIAN_POINT ( 'NONE',  ( 1.339745962155612702, -86.16965819600731891, -5.000000000000000000 ) ) ;
#13723=CARTESIAN_POINT ( 'NONE',  ( -4.458734124999997661, -15.22916666530107754, 2.574251347313722516 ) ) ;
#13724=FACE_OUTER_BOUND ( 'NONE', #19735, .T. ) ;
#13726=CARTESIAN_POINT ( 'NONE',  ( 2.229367062500001939, -42.22916666530107932, 3.861377020970579999 ) ) ;
#13734=CARTESIAN_POINT ( 'NONE',  ( 2.229367062500001939, 16.02083333469892779, 3.861377020970579999 ) ) ;
#13736=EDGE_CURVE ( 'NONE', #14611, #38431, #54682, .T. ) ;
#13737=CARTESIAN_POINT ( 'NONE',  ( -1.339745962155613812, -65.08034179853029855, -5.000000000000000000 ) ) ;
#13738=CARTESIAN_POINT ( 'NONE',  ( 9.457646018065525792E-16, -90.31249999863439371, 5.148502694627439702 ) ) ;
#13740=CARTESIAN_POINT ( 'NONE',  ( 2.499999999999998668, 11.79166666939785202, -4.330127018922193649 ) ) ;
#13742=CARTESIAN_POINT ( 'NONE',  ( 5.000000000000000000, -79.50000000000000000, -6.123233995736766282E-16 ) ) ;
#13744=FACE_OUTER_BOUND ( 'NONE', #54736, .T. ) ;
#13745=CARTESIAN_POINT ( 'NONE',  ( -5.000000000000000000, -27.99999999999999645, 0.000000000000000000 ) ) ;
#13746=CARTESIAN_POINT ( 'NONE',  ( -2.229367062500000163, -32.47916666530106511, -3.861377020970580443 ) ) ;
#13747=CARTESIAN_POINT ( 'NONE',  ( 1.060575238724906964E-15, -35.62499999726881583, 5.773502691896257311 ) ) ;
#13748=CARTESIAN_POINT ( 'NONE',  ( -3.152548672688508926E-16, -61.56249999863440792, -5.148502694627439702 ) ) ;
#13749=ORIENTED_EDGE ( 'NONE', *, *, #56664, .T. ) ;
#13751=CARTESIAN_POINT ( 'NONE',  ( 4.458734124999998549, -7.979166665301073991, -2.574251347313721627 ) ) ;
#13752=ORIENTED_EDGE ( 'NONE', *, *, #49381, .F. ) ;
#13753=CARTESIAN_POINT ( 'NONE',  ( 5.000000000000000888, -78.58333333333334281, 2.886751345948126879 ) ) ;
#13756=CARTESIAN_POINT ( 'NONE',  ( 5.000000000000000000, -83.29166666393547303, -2.886751345948129988 ) ) ;
#13757=CARTESIAN_POINT ( 'NONE',  ( 0.000000000000000000, -170.0000000000000000, 0.000000000000000000 ) ) ;
#13760=CARTESIAN_POINT ( 'NONE',  ( -2.229367062500000163, -20.72916666530107221, -3.861377020970580443 ) ) ;
#13761=CARTESIAN_POINT ( 'NONE',  ( -4.458734124999999437, -56.56249999863440081, 0.000000000000000000 ) ) ;
#13762=ORIENTED_EDGE ( 'NONE', *, *, #6329, .F. ) ;
#13764=CARTESIAN_POINT ( 'NONE',  ( -3.152801135295367096, -165.3125000013656063, -3.152801135295367541 ) ) ;
#13772=CARTESIAN_POINT ( 'NONE',  ( -9.184850993605147944E-16, -153.3750000027311842, 5.000000000000000000 ) ) ;
#13775=VECTOR ( 'NONE', #39470, 1000.000000000000000 ) ;
#13776=CARTESIAN_POINT ( 'NONE',  ( -1.846868145590737420, -143.0000000013655779, 4.458734124999999437 ) ) ;
#13778=CARTESIAN_POINT ( 'NONE',  ( 2.499999999999998668, -70.33333333333332860, -4.330127018922193649 ) ) ;
#13780=CARTESIAN_POINT ( 'NONE',  ( -2.229367062500000163, -66.72916666530106511, -3.861377020970580443 ) ) ;
#13781=CARTESIAN_POINT ( 'NONE',  ( -6.972266317189433020E-16, -73.12499999726878741, -5.000000000000000000 ) ) ;
#13783=CARTESIAN_POINT ( 'NONE',  ( -3.152801135295367096, -143.0625000013655779, -3.152801135295367541 ) ) ;
#13785=VERTEX_POINT ( 'NONE', #29241 ) ;
#13786=CARTESIAN_POINT ( 'NONE',  ( 5.000000000000000888, -159.9375000000000000, -2.071067811865475505 ) ) ;
#13789=CARTESIAN_POINT ( 'NONE',  ( 2.499999999999998668, -14.20833333060214976, -4.330127018922193649 ) ) ;
#13791=CARTESIAN_POINT ( 'NONE',  ( -3.152548672688508926E-16, 22.18750000136559564, -5.148502694627439702 ) ) ;
#13793=CARTESIAN_POINT ( 'NONE',  ( -1.339745962155617365, 23.33034180399266333, 4.999999999999998224 ) ) ;
#13795=EDGE_CURVE ( 'NONE', #23803, #47078, #32901, .T. ) ;
#13800=CARTESIAN_POINT ( 'NONE',  ( 2.499999999999998668, -80.33333333333332860, -4.330127018922193649 ) ) ;
#13801=EDGE_CURVE ( 'NONE', #592, #51356, #16928, .T. ) ;
#13802=CARTESIAN_POINT ( 'NONE',  ( -2.229367062500000163, 3.520833334698929118, -3.861377020970580443 ) ) ;
#13803=CARTESIAN_POINT ( 'NONE',  ( 9.457646018065525792E-16, -24.31249999863440436, 5.148502694627439702 ) ) ;
#13804=CARTESIAN_POINT ( 'NONE',  ( -4.458734125000001214, -155.8750000013655779, 1.846868145590734089 ) ) ;
#13808=CARTESIAN_POINT ( 'NONE',  ( 1.339745962155602488, 15.29465819873851729, 5.000000000000007105 ) ) ;
#13812=CARTESIAN_POINT ( 'NONE',  ( -4.458734124999997661, -75.47916666530106511, 2.574251347313722516 ) ) ;
#13814=CARTESIAN_POINT ( 'NONE',  ( 1.339745962155612702, -73.29465819873851729, -5.000000000000000000 ) ) ;
#13815=CARTESIAN_POINT ( 'NONE',  ( 3.535533905932738197, -156.0000000027312126, -3.535533905932738197 ) ) ;
#13818=CARTESIAN_POINT ( 'NONE',  ( -6.972266317189433020E-16, 11.87500000273118594, -5.000000000000000000 ) ) ;
#13819=CARTESIAN_POINT ( 'NONE',  ( -5.000000000000000000, -13.08333333333333570, -2.886751345948128211 ) ) ;
#13820=CARTESIAN_POINT ( 'NONE',  ( 4.458734124999999437, -17.81249999863440792, -5.460374474430324690E-16 ) ) ;
#13822=CARTESIAN_POINT ( 'NONE',  ( 4.458734125000000326, -76.89583333196773651, 2.574251347313718519 ) ) ;
#13823=CARTESIAN_POINT ( 'NONE',  ( -3.152801135295367985, -167.0625000013656063, 3.152801135295367096 ) ) ;
#13824=CARTESIAN_POINT ( 'NONE',  ( 5.000000000000000000, -19.37499999726881583, -6.123233995736766282E-16 ) ) ;
#13825=CARTESIAN_POINT ( 'NONE',  ( -4.458734124999999437, -42.39583333196773651, -2.574251347313719407 ) ) ;
#13828=CARTESIAN_POINT ( 'NONE',  ( 2.229367062499998831, 7.104166668032259935, -3.861377020970580887 ) ) ;
#13831=CARTESIAN_POINT ( 'NONE',  ( 5.000000000000000888, -61.58333333333334281, 2.886751345948126879 ) ) ;
#13832=CARTESIAN_POINT ( 'NONE',  ( 2.730187237215162345E-16, -157.4375000013655779, -4.458734124999999437 ) ) ;
#13834=CARTESIAN_POINT ( 'NONE',  ( 2.071067811865476394, -167.1875000000000284, 5.000000000000000000 ) ) ;
#13835=CARTESIAN_POINT ( 'NONE',  ( 1.339745962155612702, 5.830341803992665106, -5.000000000000000000 ) ) ;
#13837=CARTESIAN_POINT ( 'NONE',  ( 9.457646018065525792E-16, -4.312499998634408804, 5.148502694627439702 ) ) ;
#13838=CARTESIAN_POINT ( 'NONE',  ( -2.229367062499996610, -40.39583333196773651, 3.861377020970582219 ) ) ;
#13840=CARTESIAN_POINT ( 'NONE',  ( -4.458734124999999437, -147.9375000013656063, -5.460374474430324690E-16 ) ) ;
#13842=CARTESIAN_POINT ( 'NONE',  ( -6.972266317189433020E-16, 8.750000000000000000, -5.000000000000000000 ) ) ;
#13846=CARTESIAN_POINT ( 'NONE',  ( 2.229367062500001939, -76.22916666530106511, 3.861377020970579999 ) ) ;
#13848=( BOUNDED_CURVE ( )  B_SPLINE_CURVE ( 2, ( #42708, #37575, #62034, #27918, #43029, #52994, #3490, #47238, #22485 ),
 .UNSPECIFIED., .F., .F. ) 
 B_SPLINE_CURVE_WITH_KNOTS ( ( 3, 2, 2, 2, 3 ),
 ( 0.7854166666666666519, 0.7861111111111110938, 0.7874999999999999778, 0.7888888888888888618, 0.7895833333333333037 ),
 .UNSPECIFIED. ) 
 CURVE ( )  GEOMETRIC_REPRESENTATION_ITEM ( )  RATIONAL_B_SPLINE_CURVE ( ( 0.9330127018922194093, 0.9330127018922194093, 1.000000000000000000, 0.8660254037844387076, 1.000000000000000000, 0.8660254037844387076, 1.000000000000000000, 0.9330127018922194093, 0.9330127018922194093 ) ) 
 REPRESENTATION_ITEM ( '' )  );
#13849=CARTESIAN_POINT ( 'NONE',  ( 0.000000000000000000, -170.0000000000000000, 0.000000000000000000 ) ) ;
#13851=CARTESIAN_POINT ( 'NONE',  ( 5.000000000000000000, -79.37499999726881583, -6.123233995736766282E-16 ) ) ;
#13852=CARTESIAN_POINT ( 'NONE',  ( 2.229367062499998831, 0.3541666680322609340, -3.861377020970580887 ) ) ;
#13853=CARTESIAN_POINT ( 'NONE',  ( -4.999999999999998224, -79.91666666666667140, 2.886751345948131764 ) ) ;
#13854=CARTESIAN_POINT ( 'NONE',  ( -4.458734124999999437, -155.0000000013656063, -1.846868145590735644 ) ) ;
#13861=CARTESIAN_POINT ( 'NONE',  ( 1.975475456537005874E-15, -69.62499999726880162, 5.000000000000000000 ) ) ;
#13863=AXIS2_PLACEMENT_3D ( 'NONE', #5055, #19204, #19841 ) ;
#13864=( BOUNDED_CURVE ( )  B_SPLINE_CURVE ( 2, ( #51691, #56523, #22742, #11799, #32379, #47178, #26280, #56839, #3121 ),
 .UNSPECIFIED., .F., .F. ) 
 B_SPLINE_CURVE_WITH_KNOTS ( ( 3, 2, 2, 2, 3 ),
 ( 0.3250000000000002887, 0.3291666666666669405, 0.3333333333333335924, 0.3375000000000002998, 0.3416666666666669516 ),
 .UNSPECIFIED. ) 
 CURVE ( )  GEOMETRIC_REPRESENTATION_ITEM ( )  RATIONAL_B_SPLINE_CURVE ( ( 0.9999999999999948930, 0.9238795325112918455, 1.000000000000000000, 0.9238795325112867385, 1.000000000000000000, 0.9238795325112867385, 1.000000000000000000, 0.9238795325112816315, 1.000000000000005107 ) ) 
 REPRESENTATION_ITEM ( '' )  );
#13866=EDGE_CURVE ( 'NONE', #9036, #3130, #28377, .T. ) ;
#13868=DIRECTION ( 'NONE',  ( -0.000000000000000000, 1.000000000000000000, -0.000000000000000000 ) ) ;
#13870=CARTESIAN_POINT ( 'NONE',  ( -5.000000000000000000, -72.08333333333332860, -2.886751345948128211 ) ) ;
#13871=CARTESIAN_POINT ( 'NONE',  ( 4.458734124999999437, 25.18750000136559208, -5.460374474430324690E-16 ) ) ;
#13873=CARTESIAN_POINT ( 'NONE',  ( 9.457646018065525792E-16, -11.31249999863440792, 5.148502694627439702 ) ) ;
#13874=LINE ( 'NONE', #48278, #13447 ) ;
#13876=CARTESIAN_POINT ( 'NONE',  ( -1.846868145590737420, -168.7500000013656063, 4.458734124999999437 ) ) ;
#13884=CARTESIAN_POINT ( 'NONE',  ( -4.458734124999999437, -157.2500000013656063, -1.846868145590735644 ) ) ;
#13889=ORIENTED_EDGE ( 'NONE', *, *, #53458, .F. ) ;
#13895=CARTESIAN_POINT ( 'NONE',  ( -2.499999999999996447, 5.166666666666666963, 4.330127018922195425 ) ) ;
#13896=CARTESIAN_POINT ( 'NONE',  ( -3.152548672688508926E-16, -60.56249999863440792, -5.148502694627439702 ) ) ;
#13898=EDGE_CURVE ( 'NONE', #44027, #57843, #56393, .T. ) ;
#13899=CARTESIAN_POINT ( 'NONE',  ( 5.000000000000000000, 2.708333336064520314, -2.886751345948129988 ) ) ;
#13900=CARTESIAN_POINT ( 'NONE',  ( -2.229367062499996610, -30.14583333196773651, 3.861377020970582219 ) ) ;
#13903=CARTESIAN_POINT ( 'NONE',  ( -5.000000000000000000, -46.00000000000000000, 0.000000000000000000 ) ) ;
#13906=CARTESIAN_POINT ( 'NONE',  ( 3.061616997868383141E-16, -154.7500000000000000, -5.000000000000000000 ) ) ;
#13907=CARTESIAN_POINT ( 'NONE',  ( 2.229367062500001939, -68.97916666530107932, 3.861377020970579999 ) ) ;
#13908=CARTESIAN_POINT ( 'NONE',  ( -3.152801135295367985, -149.0625000013655779, 3.152801135295367096 ) ) ;
#13909=CARTESIAN_POINT ( 'NONE',  ( -2.229367062500000163, -77.47916666530106511, -3.861377020970580443 ) ) ;
#13911=AXIS2_PLACEMENT_3D ( 'NONE', #37064, #8423, #61515 ) ;
#13912=CARTESIAN_POINT ( 'NONE',  ( -3.152548672688508926E-16, -22.81249999863440436, -5.148502694627439702 ) ) ;
#13913=CARTESIAN_POINT ( 'NONE',  ( -5.000000000000000000, -65.87499999726881583, 0.000000000000000000 ) ) ;
#13916=ORIENTED_EDGE ( 'NONE', *, *, #29545, .F. ) ;
#13919=DIRECTION ( 'NONE',  ( 1.000000000000000000, 0.000000000000000000, 0.000000000000000000 ) ) ;
#13922=CYLINDRICAL_SURFACE ( 'NONE', #1414, 5.000000000000000000 ) ;
#13923=CARTESIAN_POINT ( 'NONE',  ( -2.229367062500000163, -54.72916666530107221, -3.861377020970580443 ) ) ;
#13927=CARTESIAN_POINT ( 'NONE',  ( -3.152548672688508926E-16, 19.43750000136559208, -5.148502694627439702 ) ) ;
#13929=CARTESIAN_POINT ( 'NONE',  ( -2.498395430326213474E-14, 20.37500000273118062, 5.000000000000000000 ) ) ;
#13930=CARTESIAN_POINT ( 'NONE',  ( 3.152801135295366208, -163.5625000013656063, 3.152801135295367985 ) ) ;
#13933=CARTESIAN_POINT ( 'NONE',  ( -6.972266317189433020E-16, -52.12499999726880873, -5.000000000000000000 ) ) ;
#13936=CARTESIAN_POINT ( 'NONE',  ( 6.123233995736766282E-16, -170.0000000000000000, -5.000000000000000000 ) ) ;
#13946=CARTESIAN_POINT ( 'NONE',  ( 5.000000000000000888, 11.41666666666666607, 2.886751345948126879 ) ) ;
#13948=CARTESIAN_POINT ( 'NONE',  ( 5.000000000000000000, -148.1875000027312126, 2.071067811865478614 ) ) ;
#13954=CARTESIAN_POINT ( 'NONE',  ( 2.071067811865476394, -144.1875000000000000, 5.000000000000000000 ) ) ;
#13956=CARTESIAN_POINT ( 'NONE',  ( -4.458734125000000326, -169.1250000013656063, 1.846868145590734089 ) ) ;
#13957=CARTESIAN_POINT ( 'NONE',  ( 2.229367062500001939, -32.97916666530106511, 3.861377020970579999 ) ) ;
#13959=DIRECTION ( 'NONE',  ( -0.000000000000000000, 1.000000000000000000, -0.000000000000000000 ) ) ;
#13961=CARTESIAN_POINT ( 'NONE',  ( 4.458734124999999437, -149.5000000013655779, 1.846868145590737864 ) ) ;
#13962=ORIENTED_EDGE ( 'NONE', *, *, #14942, .F. ) ;
#13963=CARTESIAN_POINT ( 'NONE',  ( 4.458734124999998549, 29.02083333469893134, -2.574251347313721627 ) ) ;
#13965=CARTESIAN_POINT ( 'NONE',  ( -4.458734124999999437, -55.56249999863440081, 0.000000000000000000 ) ) ;
#13967=( BOUNDED_CURVE ( )  B_SPLINE_CURVE ( 2, ( #32219, #37681, #18690, #26211, #61832, #57323, #23207, #17754, #13239 ),
 .UNSPECIFIED., .F., .F. ) 
 B_SPLINE_CURVE_WITH_KNOTS ( ( 3, 2, 2, 2, 3 ),
 ( 0.4354166666666666741, 0.4361111111111111160, 0.4375000000000000000, 0.4388888888888888840, 0.4395833333333333259 ),
 .UNSPECIFIED. ) 
 CURVE ( )  GEOMETRIC_REPRESENTATION_ITEM ( )  RATIONAL_B_SPLINE_CURVE ( ( 0.9330127018922194093, 0.9330127018922194093, 1.000000000000000000, 0.8660254037844387076, 1.000000000000000000, 0.8660254037844387076, 1.000000000000000000, 0.9330127018922194093, 0.9330127018922194093 ) ) 
 REPRESENTATION_ITEM ( '' )  );
#13969=CARTESIAN_POINT ( 'NONE',  ( 1.060575238724906964E-15, 18.24999999999999645, 5.773502691896257311 ) ) ;
#13970=CARTESIAN_POINT ( 'NONE',  ( 0.000000000000000000, -170.0000000000000000, 0.000000000000000000 ) ) ;
#13971=CARTESIAN_POINT ( 'NONE',  ( -4.458734124999998549, -8.229166665301073991, 2.574251347313722516 ) ) ;
#13972=CARTESIAN_POINT ( 'NONE',  ( -5.000000000000000000, -154.5000000000000284, -6.123233995736766282E-16 ) ) ;
#13973=CARTESIAN_POINT ( 'NONE',  ( 5.000000000000000000, -165.1875000027312126, 2.071067811865478614 ) ) ;
#13974=CARTESIAN_POINT ( 'NONE',  ( 4.458734124999999437, 10.93750000136559386, -5.460374474430324690E-16 ) ) ;
#13978=CARTESIAN_POINT ( 'NONE',  ( -4.458734124999999437, -50.39583333196773651, -2.574251347313719407 ) ) ;
#13979=CARTESIAN_POINT ( 'NONE',  ( -4.458734125000001214, -161.1250000013656063, 1.846868145590734089 ) ) ;
#13980=CARTESIAN_POINT ( 'NONE',  ( 1.060575238724906964E-15, -52.62499999726881583, 5.773502691896257311 ) ) ;
#13981=ORIENTED_EDGE ( 'NONE', *, *, #45977, .F. ) ;
#13982=CARTESIAN_POINT ( 'NONE',  ( -2.229367062499996610, 2.604166668032259491, 3.861377020970582219 ) ) ;
#13983=ORIENTED_EDGE ( 'NONE', *, *, #28401, .T. ) ;
#13986=CARTESIAN_POINT ( 'NONE',  ( -3.152801135295367985, -158.8125000013656063, 3.152801135295367096 ) ) ;
#13987=ORIENTED_EDGE ( 'NONE', *, *, #42115, .F. ) ;
#13989=CARTESIAN_POINT ( 'NONE',  ( 1.339745962155615144, -83.70534180126149693, 4.999999999999999112 ) ) ;
#13991=EDGE_CURVE ( 'NONE', #35553, #60346, #45008, .T. ) ;
#13993=CARTESIAN_POINT ( 'NONE',  ( -4.458734124999999437, -37.56249999863440792, 0.000000000000000000 ) ) ;
#13994=ORIENTED_EDGE ( 'NONE', *, *, #7853, .T. ) ;
#13995=AXIS2_PLACEMENT_3D ( 'NONE', #61667, #8263, #36571 ) ;
#13998=CARTESIAN_POINT ( 'NONE',  ( 1.339745962155612702, -24.16965819600733312, -5.000000000000000000 ) ) ;
#14000=CARTESIAN_POINT ( 'NONE',  ( -4.458734124999999437, -87.64583333196773651, -2.574251347313719407 ) ) ;
#14006=CARTESIAN_POINT ( 'NONE',  ( -5.000000000000000000, -84.95833333060213022, -2.886751345948128211 ) ) ;
#14009=CARTESIAN_POINT ( 'NONE',  ( -2.499999999999996447, -81.83333333333332860, 4.330127018922195425 ) ) ;
#14014=CARTESIAN_POINT ( 'NONE',  ( -2.229367062499996610, -84.39583333196773651, 3.861377020970582219 ) ) ;
#14018=CARTESIAN_POINT ( 'NONE',  ( -1.339745962155613812, -17.08034179853029144, -5.000000000000000000 ) ) ;
#14020=CARTESIAN_POINT ( 'NONE',  ( -5.000000000000000000, -165.6250000027312126, -6.123233995736766282E-16 ) ) ;
#14023=CARTESIAN_POINT ( 'NONE',  ( 3.061616997868383141E-16, -148.7500000000000284, -5.000000000000000000 ) ) ;
#14030=CARTESIAN_POINT ( 'NONE',  ( -2.229367062500000163, -15.47916666530107399, -3.861377020970580443 ) ) ;
#14032=VERTEX_POINT ( 'NONE', #1604 ) ;
#14033=CARTESIAN_POINT ( 'NONE',  ( -4.458734124999997661, -43.47916666530106511, 2.574251347313722516 ) ) ;
#14034=CARTESIAN_POINT ( 'NONE',  ( 2.499999999999998668, -77.33333333333334281, -4.330127018922193649 ) ) ;
#14036=CYLINDRICAL_SURFACE ( 'NONE', #18322, 5.000000000000000000 ) ;
#14041=( BOUNDED_CURVE ( )  B_SPLINE_CURVE ( 2, ( #62448, #47945, #43431, #58234, #13851, #62759, #4215, #9030, #18370 ),
 .UNSPECIFIED., .F., .F. ) 
 B_SPLINE_CURVE_WITH_KNOTS ( ( 3, 2, 2, 2, 3 ),
 ( 0.9020833333333333481, 0.9027777777777777901, 0.9041666666666666741, 0.9055555555555555580, 0.9062500000000000000 ),
 .UNSPECIFIED. ) 
 CURVE ( )  GEOMETRIC_REPRESENTATION_ITEM ( )  RATIONAL_B_SPLINE_CURVE ( ( 0.9330127018922194093, 0.9330127018922194093, 1.000000000000000000, 0.8660254037844387076, 1.000000000000000000, 0.8660254037844387076, 1.000000000000000000, 0.9330127018922194093, 0.9330127018922194093 ) ) 
 REPRESENTATION_ITEM ( '' )  );
#14042=CARTESIAN_POINT ( 'NONE',  ( 9.457646018065525792E-16, 11.93750000136559386, 5.148502694627439702 ) ) ;
#14045=CARTESIAN_POINT ( 'NONE',  ( 3.061616997868383141E-16, -144.7500000000000284, -5.000000000000000000 ) ) ;
#14048=CARTESIAN_POINT ( 'NONE',  ( 5.000000000000000000, 15.70833333606451809, -2.886751345948129988 ) ) ;
#14051=VERTEX_POINT ( 'NONE', #26031 ) ;
#14052=CARTESIAN_POINT ( 'NONE',  ( 2.071067811865443975, -166.8125000000000000, -5.000000000000031974 ) ) ;
#14053=DIRECTION ( 'NONE',  ( -0.000000000000000000, 1.000000000000000000, -0.000000000000000000 ) ) ;
#14054=CARTESIAN_POINT ( 'NONE',  ( 5.000000000000000000, -28.49999999999999645, -6.123233995736766282E-16 ) ) ;
#14055=CARTESIAN_POINT ( 'NONE',  ( -3.152548672688508926E-16, -30.56249999863440436, -5.148502694627439702 ) ) ;
#14056=CARTESIAN_POINT ( 'NONE',  ( 5.000000000000000888, -36.45833333060214443, 2.886751345948126879 ) ) ;
#14057=CARTESIAN_POINT ( 'NONE',  ( 2.229367062499998831, -68.64583333196773651, -3.861377020970580887 ) ) ;
#14060=CARTESIAN_POINT ( 'NONE',  ( -4.458734124999999437, -15.64583333196773474, -2.574251347313719407 ) ) ;
#14061=ORIENTED_EDGE ( 'NONE', *, *, #60875, .F. ) ;
#14062=CARTESIAN_POINT ( 'NONE',  ( 5.000000000000000000, -76.50000000000000000, -6.123233995736766282E-16 ) ) ;
#14065=CARTESIAN_POINT ( 'NONE',  ( 1.060575238724906964E-15, -82.62499999726880162, 5.773502691896257311 ) ) ;
#14069=CARTESIAN_POINT ( 'NONE',  ( -4.458734124999999437, -23.64583333196773651, -2.574251347313719407 ) ) ;
#14070=CARTESIAN_POINT ( 'NONE',  ( 2.229367062499998831, -59.89583333196774362, -3.861377020970580887 ) ) ;
#14071=VERTEX_POINT ( 'NONE', #10584 ) ;
#14072=CARTESIAN_POINT ( 'NONE',  ( -8.190561711645485556E-16, -164.9375000013655779, 4.458734124999999437 ) ) ;
#14078=CARTESIAN_POINT ( 'NONE',  ( 5.000000000000000888, 18.41666666666666430, 2.886751345948126879 ) ) ;
#14079=VECTOR ( 'NONE', #4293, 1000.000000000000000 ) ;
#14081=VECTOR ( 'NONE', #593, 1000.000000000000000 ) ;
#14083=EDGE_CURVE ( 'NONE', #45777, #14700, #46047, .T. ) ;
#14084=CARTESIAN_POINT ( 'NONE',  ( 4.458734124999999437, -142.6875000013656063, 0.000000000000000000 ) ) ;
#14088=FACE_OUTER_BOUND ( 'NONE', #40344, .T. ) ;
#14091=CARTESIAN_POINT ( 'NONE',  ( 9.457646018065525792E-16, -71.31249999863439371, 5.148502694627439702 ) ) ;
#14092=CARTESIAN_POINT ( 'NONE',  ( 1.846868145590736310, -140.6250000013656063, 4.458734124999997661 ) ) ;
#14101=CARTESIAN_POINT ( 'NONE',  ( 2.229367062500001939, 21.77083333469892779, 3.861377020970579999 ) ) ;
#14102=CARTESIAN_POINT ( 'NONE',  ( 5.000000000000000000, -18.41666666666666430, -2.886751345948130876 ) ) ;
#14109=CARTESIAN_POINT ( 'NONE',  ( 4.458734124999998549, -0.7291666653010709931, -2.574251347313721627 ) ) ;
#14110=CARTESIAN_POINT ( 'NONE',  ( -2.229367062499996610, -26.39583333196774007, 3.861377020970582219 ) ) ;
#14111=CARTESIAN_POINT ( 'NONE',  ( -1.846868145590737420, -154.7500000013656063, 4.458734124999999437 ) ) ;
#14115=LINE ( 'NONE', #39824, #7177 ) ;
#14118=CARTESIAN_POINT ( 'NONE',  ( 4.458734125000000326, -73.14583333196772230, 2.574251347313718519 ) ) ;
#14121=CARTESIAN_POINT ( 'NONE',  ( -1.339745962155564296, -11.08034179853029677, -5.000000000000028422 ) ) ;
#14122=ORIENTED_EDGE ( 'NONE', *, *, #25938, .T. ) ;
#14123=CARTESIAN_POINT ( 'NONE',  ( 5.000000000000000000, 6.499999999999999112, -6.123233995736766282E-16 ) ) ;
#14125=CARTESIAN_POINT ( 'NONE',  ( 2.499999999999998668, -14.33333333333333037, -4.330127018922193649 ) ) ;
#14126=CARTESIAN_POINT ( 'NONE',  ( -2.229367062499996610, -17.14583333196773651, 3.861377020970582219 ) ) ;
#14127=CARTESIAN_POINT ( 'NONE',  ( 4.458734124999999437, -77.81249999863440792, -5.460374474430324690E-16 ) ) ;
#14128=CARTESIAN_POINT ( 'NONE',  ( -3.152801135295367985, -169.0625000013656063, 3.152801135295367096 ) ) ;
#14129=CARTESIAN_POINT ( 'NONE',  ( -4.999999999999999112, -20.79166666393548013, 2.886751345948131764 ) ) ;
#14130=CARTESIAN_POINT ( 'NONE',  ( -4.458734124999998549, -45.22916666530106511, 2.574251347313722516 ) ) ;
#14133=CARTESIAN_POINT ( 'NONE',  ( -4.458734124999998549, 0.5208333346989265644, 2.574251347313722516 ) ) ;
#14136=CARTESIAN_POINT ( 'NONE',  ( -4.999999999999999112, -59.91666666666665719, 2.886751345948131764 ) ) ;
#14137=CARTESIAN_POINT ( 'NONE',  ( -8.190561711645485556E-16, -157.9375000013655779, 4.458734124999999437 ) ) ;
#14140=( BOUNDED_CURVE ( )  B_SPLINE_CURVE ( 2, ( #26859, #2417, #33566, #42894, #58327, #29036, #39015, #42584, #38387 ),
 .UNSPECIFIED., .F., .F. ) 
 B_SPLINE_CURVE_WITH_KNOTS ( ( 3, 2, 2, 2, 3 ),
 ( 0.6270833333333333259, 0.6277777777777777679, 0.6291666666666666519, 0.6305555555555555358, 0.6312499999999999778 ),
 .UNSPECIFIED. ) 
 CURVE ( )  GEOMETRIC_REPRESENTATION_ITEM ( )  RATIONAL_B_SPLINE_CURVE ( ( 0.9330127018922194093, 0.9330127018922194093, 1.000000000000000000, 0.8660254037844387076, 1.000000000000000000, 0.8660254037844387076, 1.000000000000000000, 0.9330127018922194093, 0.9330127018922194093 ) ) 
 REPRESENTATION_ITEM ( '' )  );
#14141=CARTESIAN_POINT ( 'NONE',  ( 5.000000000000000888, -160.9375000000000284, -2.071067811865475505 ) ) ;
#14142=CYLINDRICAL_SURFACE ( 'NONE', #24111, 5.000000000000000000 ) ;
#14145=CARTESIAN_POINT ( 'NONE',  ( 2.229367062499998831, -6.895833331967741842, -3.861377020970580887 ) ) ;
#14146=CARTESIAN_POINT ( 'NONE',  ( 2.229367062500001939, -43.22916666530107932, 3.861377020970579999 ) ) ;
#14147=EDGE_CURVE ( 'NONE', #29588, #21097, #57445, .T. ) ;
#14148=ADVANCED_FACE ( 'NONE', ( #7051 ), #50793, .T. ) ;
#14150=CARTESIAN_POINT ( 'NONE',  ( 3.152801135295366208, -147.5625000013655779, 3.152801135295367985 ) ) ;
#14162=CARTESIAN_POINT ( 'NONE',  ( 4.458734124999998549, -3.729166665301070438, -2.574251347313721627 ) ) ;
#14163=CARTESIAN_POINT ( 'NONE',  ( -4.999999999999998224, -42.91666666666665719, 2.886751345948131764 ) ) ;
#14164=CARTESIAN_POINT ( 'NONE',  ( -3.152801135295367985, -152.8125000013656063, 3.152801135295367096 ) ) ;
#14169=CARTESIAN_POINT ( 'NONE',  ( -1.339745962155613812, -75.20534180126148271, -5.000000000000000000 ) ) ;
#14180=CARTESIAN_POINT ( 'NONE',  ( -2.229367062500000163, 16.52083333469892779, -3.861377020970580443 ) ) ;
#14182=CARTESIAN_POINT ( 'NONE',  ( -4.458734124999997661, -7.479166665301073991, 2.574251347313722516 ) ) ;
#14185=CARTESIAN_POINT ( 'NONE',  ( -1.846868145590734756, -166.1250000013655779, -4.458734125000000326 ) ) ;
#14194=CARTESIAN_POINT ( 'NONE',  ( -3.152801135295367096, -153.3125000013656063, -3.152801135295367541 ) ) ;
#14197=DIRECTION ( 'NONE',  ( 0.000000000000000000, 0.000000000000000000, 1.000000000000000000 ) ) ;
#14202=CARTESIAN_POINT ( 'NONE',  ( 5.000000000000000888, -161.9374999999999716, -2.071067811865475505 ) ) ;
#14203=CARTESIAN_POINT ( 'NONE',  ( 1.060575238724906964E-15, 3.249999999999999556, 5.773502691896257311 ) ) ;
#14204=CARTESIAN_POINT ( 'NONE',  ( 9.457646018065525792E-16, -62.06249999863440792, 5.148502694627439702 ) ) ;
#14205=CARTESIAN_POINT ( 'NONE',  ( 1.975475456537005874E-15, -30.62499999726881583, 5.000000000000000000 ) ) ;
#14206=CARTESIAN_POINT ( 'NONE',  ( -4.999999999999999112, -4.791666663935479242, 2.886751345948131764 ) ) ;
#14207=CARTESIAN_POINT ( 'NONE',  ( 2.229367062500001939, -26.97916666530106866, 3.861377020970579999 ) ) ;
#14208=CARTESIAN_POINT ( 'NONE',  ( 2.788906526875773208E-15, 28.75000000000000000, -5.000000000000000000 ) ) ;
#14211=CARTESIAN_POINT ( 'NONE',  ( 5.000000000000000000, -44.50000000000000000, -6.123233995736766282E-16 ) ) ;
#14216=CARTESIAN_POINT ( 'NONE',  ( 9.457646018065525792E-16, -69.06249999863439371, 5.148502694627439702 ) ) ;
#14217=CARTESIAN_POINT ( 'NONE',  ( 4.458734124999999437, -143.6875000013656063, 0.000000000000000000 ) ) ;
#14218=CARTESIAN_POINT ( 'NONE',  ( 2.229367062500001939, -76.97916666530106511, 3.861377020970579999 ) ) ;
#14221=CARTESIAN_POINT ( 'NONE',  ( -2.229367062499996610, -24.39583333196773651, 3.861377020970582219 ) ) ;
#14222=CARTESIAN_POINT ( 'NONE',  ( -2.500000000000000444, -67.04166666393547303, -4.330127018922193649 ) ) ;
#14224=ORIENTED_EDGE ( 'NONE', *, *, #52664, .T. ) ;
#14228=CARTESIAN_POINT ( 'NONE',  ( 5.000000000000000000, 28.49999999999999645, -6.123233995736766282E-16 ) ) ;
#14231=EDGE_CURVE ( 'NONE', #25897, #27694, #31163, .T. ) ;
#14232=CARTESIAN_POINT ( 'NONE',  ( -5.000000000000000000, -77.87499999726881583, 0.000000000000000000 ) ) ;
#14233=CARTESIAN_POINT ( 'NONE',  ( -2.229367062500000163, -56.72916666530107221, -3.861377020970580443 ) ) ;
#14238=( BOUNDED_CURVE ( )  B_SPLINE_CURVE ( 2, ( #21079, #49701, #14967, #54853, #44230, #59357, #55504, #840, #24624 ),
 .UNSPECIFIED., .F., .F. ) 
 B_SPLINE_CURVE_WITH_KNOTS ( ( 3, 2, 2, 2, 3 ),
 ( 0.008333333333333340157, 0.01250000000000001110, 0.01666666666666668031, 0.02083333333333334952, 0.02500000000000002220 ),
 .UNSPECIFIED. ) 
 CURVE ( )  GEOMETRIC_REPRESENTATION_ITEM ( )  RATIONAL_B_SPLINE_CURVE ( ( 0.9999999999999998890, 0.9238795325112868495, 1.000000000000000000, 0.9238795325112867385, 1.000000000000000000, 0.9238795325112867385, 1.000000000000000000, 0.9238795325112864054, 1.000000000000000444 ) ) 
 REPRESENTATION_ITEM ( '' )  );
#14240=EDGE_CURVE ( 'NONE', #39148, #39239, #6731, .T. ) ;
#14241=CARTESIAN_POINT ( 'NONE',  ( -2.229367062500000163, 13.52083333469892779, -3.861377020970580443 ) ) ;
#14244=CARTESIAN_POINT ( 'NONE',  ( 4.458734124999999437, -165.3750000013656347, -1.846868145590734978 ) ) ;
#14245=VERTEX_POINT ( 'NONE', #43562 ) ;
#14260=CARTESIAN_POINT ( 'NONE',  ( -2.229367062499996610, 8.604166668032261711, 3.861377020970582219 ) ) ;
#14261=AXIS2_PLACEMENT_3D ( 'NONE', #50937, #15887, #54809 ) ;
#14265=CARTESIAN_POINT ( 'NONE',  ( 2.071067811865475505, -149.9375000027312126, -5.000000000000000888 ) ) ;
#14266=CARTESIAN_POINT ( 'NONE',  ( -4.999999999999998224, 29.08333333333333215, 2.886751345948131764 ) ) ;
#14271=CARTESIAN_POINT ( 'NONE',  ( -2.071067811865478170, -141.3125000000000000, 5.000000000000000000 ) ) ;
#14273=CARTESIAN_POINT ( 'NONE',  ( 3.152801135295367541, -166.5625000013656063, -3.152801135295367541 ) ) ;
#14274=CARTESIAN_POINT ( 'NONE',  ( -2.229367062500000163, -28.47916666530107221, -3.861377020970580443 ) ) ;
#14278=CARTESIAN_POINT ( 'NONE',  ( -3.152801135295367985, -145.8125000013655779, 3.152801135295367096 ) ) ;
#14280=CARTESIAN_POINT ( 'NONE',  ( 2.499999999999998668, -90.20833333060214443, -4.330127018922193649 ) ) ;
#14282=CARTESIAN_POINT ( 'NONE',  ( -3.152548672688508926E-16, -57.81249999863440081, -5.148502694627439702 ) ) ;
#14284=CARTESIAN_POINT ( 'NONE',  ( -6.972266317189433020E-16, -90.12499999726880162, -5.000000000000000000 ) ) ;
#14285=CARTESIAN_POINT ( 'NONE',  ( 5.000000000000000000, 17.50000000000000000, -6.123233995736766282E-16 ) ) ;
#14286=CARTESIAN_POINT ( 'NONE',  ( -6.972266317189433020E-16, -37.12499999726881583, -5.000000000000000000 ) ) ;
#14287=CARTESIAN_POINT ( 'NONE',  ( 9.457646018065525792E-16, -4.062499998634408804, 5.148502694627439702 ) ) ;
#14288=FACE_OUTER_BOUND ( 'NONE', #12731, .T. ) ;
#14290=CARTESIAN_POINT ( 'NONE',  ( 0.000000000000000000, -170.0000000000000000, 0.000000000000000000 ) ) ;
#14295=CARTESIAN_POINT ( 'NONE',  ( 2.229367062500001939, -53.97916666530107221, 3.861377020970579999 ) ) ;
#14296=CARTESIAN_POINT ( 'NONE',  ( 1.846868145590736310, -158.8750000013655779, 4.458734124999999437 ) ) ;
#14297=CARTESIAN_POINT ( 'NONE',  ( 1.060575238724906964E-15, -48.62499999726881583, 5.773502691896257311 ) ) ;
#14298=ORIENTED_EDGE ( 'NONE', *, *, #49083, .F. ) ;
#14299=CARTESIAN_POINT ( 'NONE',  ( -4.458734124999999437, 5.354166668032262599, -2.574251347313719407 ) ) ;
#14303=CARTESIAN_POINT ( 'NONE',  ( 4.458734124999999437, -162.5000000013655779, 1.846868145590737864 ) ) ;
#14304=ORIENTED_EDGE ( 'NONE', *, *, #9380, .F. ) ;
#14308=LINE ( 'NONE', #46926, #48016 ) ;
#14309=AXIS2_PLACEMENT_3D ( 'NONE', #44171, #4943, #138 ) ;
#14310=CARTESIAN_POINT ( 'NONE',  ( 9.457646018065525792E-16, -42.31249999863440081, 5.148502694627439702 ) ) ;
#14314=CARTESIAN_POINT ( 'NONE',  ( 1.339745962155615144, -59.70534180126147561, 4.999999999999999112 ) ) ;
#14316=CARTESIAN_POINT ( 'NONE',  ( 4.458734124999999437, -88.06249999863439371, -5.460374474430324690E-16 ) ) ;
#14318=CARTESIAN_POINT ( 'NONE',  ( 5.000000000000000000, -35.29166666393547303, -2.886751345948130876 ) ) ;
#14323=CARTESIAN_POINT ( 'NONE',  ( -1.339745962155613812, -62.08034179853028434, -5.000000000000000000 ) ) ;
#14330=DIRECTION ( 'NONE',  ( -0.000000000000000000, 1.000000000000000000, -0.000000000000000000 ) ) ;
#14332=CARTESIAN_POINT ( 'NONE',  ( 4.458734124999998549, -85.97916666530107932, -2.574251347313721627 ) ) ;
#14335=ORIENTED_EDGE ( 'NONE', *, *, #54703, .F. ) ;
#14336=CARTESIAN_POINT ( 'NONE',  ( -3.535533905932737309, -155.7500000027312126, -3.535533905932738197 ) ) ;
#14338=CARTESIAN_POINT ( 'NONE',  ( 3.535533905932736864, -163.2500000027312126, 3.535533905932738641 ) ) ;
#14340=CARTESIAN_POINT ( 'NONE',  ( 2.626220312808019583E-14, 21.75000000000000000, -5.000000000000000000 ) ) ;
#14348=CARTESIAN_POINT ( 'NONE',  ( -5.000000000000000000, -20.08333333333333925, -2.886751345948128211 ) ) ;
#14349=CARTESIAN_POINT ( 'NONE',  ( 2.229367062499998831, -14.64583333196773474, -3.861377020970580887 ) ) ;
#14351=CARTESIAN_POINT ( 'NONE',  ( -5.000000000000000888, -153.5625000000000568, -2.071067811865475949 ) ) ;
#14352=ORIENTED_EDGE ( 'NONE', *, *, #37764, .T. ) ;
#14353=CARTESIAN_POINT ( 'NONE',  ( 2.229367062500001939, -40.22916666530107221, 3.861377020970579999 ) ) ;
#14356=FACE_OUTER_BOUND ( 'NONE', #42846, .T. ) ;
#14360=CARTESIAN_POINT ( 'NONE',  ( 4.458734124999998549, 8.270833334698926009, -2.574251347313721627 ) ) ;
#14361=FACE_OUTER_BOUND ( 'NONE', #30765, .T. ) ;
#14362=CARTESIAN_POINT ( 'NONE',  ( -2.229367062499996610, -90.39583333196773651, 3.861377020970582219 ) ) ;
#14364=CARTESIAN_POINT ( 'NONE',  ( 5.000000000000000000, 14.70833333606451987, -2.886751345948129988 ) ) ;
#14368=CARTESIAN_POINT ( 'NONE',  ( 0.000000000000000000, -170.0000000000000000, 0.000000000000000000 ) ) ;
#14369=CARTESIAN_POINT ( 'NONE',  ( 2.499999999999998668, -32.33333333333332860, -4.330127018922193649 ) ) ;
#14370=CARTESIAN_POINT ( 'NONE',  ( 4.458734125000001214, -35.89583333196773651, 2.574251347313718519 ) ) ;
#14371=CARTESIAN_POINT ( 'NONE',  ( -4.999999999999999112, -36.79166666393548013, 2.886751345948131764 ) ) ;
#14372=CARTESIAN_POINT ( 'NONE',  ( 4.458734124999998549, -64.72916666530106511, -2.574251347313721627 ) ) ;
#14373=VERTEX_POINT ( 'NONE', #9164 ) ;
#14375=CARTESIAN_POINT ( 'NONE',  ( 2.229367062499998831, -14.64583333196773474, -3.861377020970580887 ) ) ;
#14376=CARTESIAN_POINT ( 'NONE',  ( 4.458734124999999437, -16.06249999863440436, -5.460374474430324690E-16 ) ) ;
#14377=ORIENTED_EDGE ( 'NONE', *, *, #61491, .F. ) ;
#14378=CARTESIAN_POINT ( 'NONE',  ( -5.000000000000000000, -76.00000000000000000, 0.000000000000000000 ) ) ;
#14381=CARTESIAN_POINT ( 'NONE',  ( -3.535250795749689387E-16, -81.12499999726881583, -5.773502691896257311 ) ) ;
#14385=CARTESIAN_POINT ( 'NONE',  ( -4.458734124999998549, -21.47916666530107221, 2.574251347313722516 ) ) ;
#14388=CARTESIAN_POINT ( 'NONE',  ( 4.458734125000000326, -166.6250000013656063, -1.846868145590734978 ) ) ;
#14390=CARTESIAN_POINT ( 'NONE',  ( -5.000000000000000888, -167.5625000027312126, 2.071067811865474617 ) ) ;
#14402=CARTESIAN_POINT ( 'NONE',  ( -1.846868145590734756, -142.3750000013656063, -4.458734125000000326 ) ) ;
#14406=CARTESIAN_POINT ( 'NONE',  ( 4.458734124999998549, -67.97916666530107932, -2.574251347313721627 ) ) ;
#14407=CARTESIAN_POINT ( 'NONE',  ( 1.339745962155612702, -43.29465819873851729, -5.000000000000000000 ) ) ;
#14409=CARTESIAN_POINT ( 'NONE',  ( 1.846868145590736310, -142.6250000013656063, 4.458734124999997661 ) ) ;
#14417=CARTESIAN_POINT ( 'NONE',  ( -4.458734124999999437, 24.43750000136559208, 0.000000000000000000 ) ) ;
#14418=CYLINDRICAL_SURFACE ( 'NONE', #34550, 5.000000000000000000 ) ;
#14419=( BOUNDED_CURVE ( )  B_SPLINE_CURVE ( 2, ( #39939, #29014, #48640, #43810, #59585, #35139, #14858, #63456, #19375 ),
 .UNSPECIFIED., .F., .F. ) 
 B_SPLINE_CURVE_WITH_KNOTS ( ( 3, 2, 2, 2, 3 ),
 ( 0.01874999999999999931, 0.01944444444444444475, 0.02083333333333333218, 0.02222222222222222307, 0.02291666666666666852 ),
 .UNSPECIFIED. ) 
 CURVE ( )  GEOMETRIC_REPRESENTATION_ITEM ( )  RATIONAL_B_SPLINE_CURVE ( ( 0.9330127018922194093, 0.9330127018922194093, 1.000000000000000000, 0.8660254037844387076, 1.000000000000000000, 0.8660254037844387076, 1.000000000000000000, 0.9330127018922191873, 0.9330127018922194093 ) ) 
 REPRESENTATION_ITEM ( '' )  );
#14425=CARTESIAN_POINT ( 'NONE',  ( 9.457646018065525792E-16, -0.06249999863440491854, 5.148502694627439702 ) ) ;
#14426=CARTESIAN_POINT ( 'NONE',  ( -4.458734124999999437, -23.56249999863440436, 0.000000000000000000 ) ) ;
#14430=CARTESIAN_POINT ( 'NONE',  ( -3.152548672688508926E-16, 27.43750000136559564, -5.148502694627439702 ) ) ;
#14433=CARTESIAN_POINT ( 'NONE',  ( -2.229367062499996610, -73.39583333196773651, 3.861377020970582219 ) ) ;
#14435=CARTESIAN_POINT ( 'NONE',  ( 6.123233995736766282E-16, -170.0000000000000000, -5.000000000000000000 ) ) ;
#14440=CARTESIAN_POINT ( 'NONE',  ( 5.000000000000000000, -17.50000000000000000, -6.123233995736766282E-16 ) ) ;
#14441=CARTESIAN_POINT ( 'NONE',  ( 2.229367062500001939, -22.97916666530107221, 3.861377020970579999 ) ) ;
#14442=AXIS2_PLACEMENT_3D ( 'NONE', #22699, #13348, #3708 ) ;
#14443=CARTESIAN_POINT ( 'NONE',  ( -4.458734124999997661, -82.22916666530106511, 2.574251347313722516 ) ) ;
#14444=CARTESIAN_POINT ( 'NONE',  ( -4.458734125000001214, -167.1250000013656063, 1.846868145590734089 ) ) ;
#14446=CARTESIAN_POINT ( 'NONE',  ( 5.000000000000000000, -16.29166666393548368, -2.886751345948129988 ) ) ;
#14447=CARTESIAN_POINT ( 'NONE',  ( -4.458734124999999437, -52.39583333196773651, -2.574251347313719407 ) ) ;
#14450=CARTESIAN_POINT ( 'NONE',  ( 2.229367062499998831, 4.104166668032260823, -3.861377020970580887 ) ) ;
#14451=ORIENTED_EDGE ( 'NONE', *, *, #16209, .T. ) ;
#14453=CARTESIAN_POINT ( 'NONE',  ( 5.000000000000000000, -60.50000000000000000, -6.123233995736766282E-16 ) ) ;
#14454=CARTESIAN_POINT ( 'NONE',  ( -4.458734125000001214, -156.1250000013655779, 1.846868145590734089 ) ) ;
#14456=CARTESIAN_POINT ( 'NONE',  ( -5.000000000000000000, -55.99999999999999289, 0.000000000000000000 ) ) ;
#14457=CARTESIAN_POINT ( 'NONE',  ( 2.071067811865476394, -163.1875000000000284, 5.000000000000000000 ) ) ;
#14460=CARTESIAN_POINT ( 'NONE',  ( -4.458734124999999437, -6.562499998634403475, 0.000000000000000000 ) ) ;
#14461=CARTESIAN_POINT ( 'NONE',  ( 2.229367062500001939, -48.22916666530106511, 3.861377020970579999 ) ) ;
#14463=CARTESIAN_POINT ( 'NONE',  ( 1.846868145590735200, -149.2500000013655779, -4.458734125000000326 ) ) ;
#14465=CARTESIAN_POINT ( 'NONE',  ( 5.000000000000000000, 8.583333333333332149, -2.886751345948130876 ) ) ;
#14466=( BOUNDED_CURVE ( )  B_SPLINE_CURVE ( 2, ( #39346, #39981, #21659, #41250, #45455, #1420, #25838, #40936, #60897 ),
 .UNSPECIFIED., .F., .F. ) 
 B_SPLINE_CURVE_WITH_KNOTS ( ( 3, 2, 2, 2, 3 ),
 ( 0.1854166666666666741, 0.1861111111111111160, 0.1875000000000000000, 0.1888888888888888840, 0.1895833333333333259 ),
 .UNSPECIFIED. ) 
 CURVE ( )  GEOMETRIC_REPRESENTATION_ITEM ( )  RATIONAL_B_SPLINE_CURVE ( ( 0.9330127018922194093, 0.9330127018922194093, 1.000000000000000000, 0.8660254037844387076, 1.000000000000000000, 0.8660254037844387076, 1.000000000000000000, 0.9330127018922194093, 0.9330127018922194093 ) ) 
 REPRESENTATION_ITEM ( '' )  );
#14469=CARTESIAN_POINT ( 'NONE',  ( -6.972266317189433020E-16, -6.124999997268813168, -5.000000000000000000 ) ) ;
#14472=VERTEX_POINT ( 'NONE', #19761 ) ;
#14475=CARTESIAN_POINT ( 'NONE',  ( 2.229367062500001939, -0.9791666653010712151, 3.861377020970579999 ) ) ;
#14477=CARTESIAN_POINT ( 'NONE',  ( 3.152801135295367541, -153.3125000013656063, -3.152801135295367541 ) ) ;
#14479=VERTEX_POINT ( 'NONE', #14614 ) ;
#14482=FACE_OUTER_BOUND ( 'NONE', #1221, .T. ) ;
#14489=CARTESIAN_POINT ( 'NONE',  ( 2.500000000000002220, -64.54166666393547303, 4.330127018922192761 ) ) ;
#14492=EDGE_LOOP ( 'NONE', ( #38427, #22355, #44815, #61750 ) ) ;
#14493=CARTESIAN_POINT ( 'NONE',  ( 4.458734124999998549, 19.27083333469893134, -2.574251347313721627 ) ) ;
#14495=CARTESIAN_POINT ( 'NONE',  ( 4.458734124999998549, -6.979166665301073103, -2.574251347313721627 ) ) ;
#14498=CARTESIAN_POINT ( 'NONE',  ( 5.000000000000000000, -139.1250000027312126, 0.000000000000000000 ) ) ;
#14502=EDGE_CURVE ( 'NONE', #47078, #39600, #26320, .T. ) ;
#14504=CARTESIAN_POINT ( 'NONE',  ( -1.339745962155613812, -55.08034179853029144, -5.000000000000000000 ) ) ;
#14505=DIRECTION ( 'NONE',  ( 0.000000000000000000, 0.000000000000000000, 1.000000000000000000 ) ) ;
#14506=CARTESIAN_POINT ( 'NONE',  ( 1.846868145590735200, -153.5000000013656063, -4.458734124999999437 ) ) ;
#14509=DIRECTION ( 'NONE',  ( -0.000000000000000000, 1.000000000000000000, -0.000000000000000000 ) ) ;
#14510=ORIENTED_EDGE ( 'NONE', *, *, #50324, .T. ) ;
#14514=CARTESIAN_POINT ( 'NONE',  ( 5.000000000000000000, 12.50000000000000000, -6.123233995736766282E-16 ) ) ;
#14515=CARTESIAN_POINT ( 'NONE',  ( 1.060575238724906964E-15, 5.250000000000000888, 5.773502691896257311 ) ) ;
#14516=ADVANCED_FACE ( 'NONE', ( #29390 ), #14931, .T. ) ;
#14517=CARTESIAN_POINT ( 'NONE',  ( 9.457646018065525792E-16, -59.06249999863440792, 5.148502694627439702 ) ) ;
#14519=CARTESIAN_POINT ( 'NONE',  ( 5.000000000000000888, -2.458333330602146205, 2.886751345948126879 ) ) ;
#14520=CARTESIAN_POINT ( 'NONE',  ( 4.458734124999999437, -31.81249999863440436, -5.460374474430324690E-16 ) ) ;
#14522=CARTESIAN_POINT ( 'NONE',  ( 2.499999999999998668, 17.79166666939785557, -4.330127018922193649 ) ) ;
#14523=CARTESIAN_POINT ( 'NONE',  ( 3.061616997868383141E-16, -156.7500000000000000, -5.000000000000000000 ) ) ;
#14526=CARTESIAN_POINT ( 'NONE',  ( 5.000000000000000000, -44.41666666666665719, -2.886751345948129988 ) ) ;
#14527=ADVANCED_FACE ( 'NONE', ( #26187 ), #45164, .T. ) ;
#14529=CARTESIAN_POINT ( 'NONE',  ( 1.975475456537005874E-15, -1.624999997268813834, 5.000000000000000000 ) ) ;
#14530=CARTESIAN_POINT ( 'NONE',  ( 4.458734124999998549, -67.72916666530107932, -2.574251347313721627 ) ) ;
#14531=CARTESIAN_POINT ( 'NONE',  ( 3.152801135295366208, -144.8125000013655779, 3.152801135295367985 ) ) ;
#14533=CARTESIAN_POINT ( 'NONE',  ( 2.229367062499998831, -75.64583333196773651, -3.861377020970580887 ) ) ;
#14535=CARTESIAN_POINT ( 'NONE',  ( 4.458734124999999437, -32.06249999863440792, -5.460374474430324690E-16 ) ) ;
#14536=CARTESIAN_POINT ( 'NONE',  ( -2.499999999999996447, -68.70833333060214443, 4.330127018922195425 ) ) ;
#14541=CARTESIAN_POINT ( 'NONE',  ( -1.339745962155610925, 8.330341803992665106, 5.000000000000000000 ) ) ;
#14543=AXIS2_PLACEMENT_3D ( 'NONE', #87, #10672, #54749 ) ;
#14544=CARTESIAN_POINT ( 'NONE',  ( -2.499999999999996447, -77.70833333060214443, 4.330127018922195425 ) ) ;
#14545=EDGE_CURVE ( 'NONE', #29728, #46916, #34961, .T. ) ;
#14546=CARTESIAN_POINT ( 'NONE',  ( 4.458734125000001214, -61.14583333196773651, 2.574251347313718519 ) ) ;
#14548=ORIENTED_EDGE ( 'NONE', *, *, #52476, .F. ) ;
#14549=CARTESIAN_POINT ( 'NONE',  ( 2.071067811865392461, -142.1875000000000284, 5.000000000000084377 ) ) ;
#14550=CARTESIAN_POINT ( 'NONE',  ( -4.999999999999998224, -59.79166666393547303, 2.886751345948131764 ) ) ;
#14551=CARTESIAN_POINT ( 'NONE',  ( -4.458734124999998549, 12.77083333469892601, 2.574251347313722516 ) ) ;
#14553=CARTESIAN_POINT ( 'NONE',  ( 2.499999999999998668, -24.33333333333333215, -4.330127018922193649 ) ) ;
#14554=CARTESIAN_POINT ( 'NONE',  ( -4.458734124999999437, -164.0000000013656063, -1.846868145590735644 ) ) ;
#14564=DIRECTION ( 'NONE',  ( 0.000000000000000000, 0.000000000000000000, 1.000000000000000000 ) ) ;
#14568=CARTESIAN_POINT ( 'NONE',  ( 4.458734125000000326, 4.854166668032262599, 2.574251347313718519 ) ) ;
#14571=CARTESIAN_POINT ( 'NONE',  ( -5.000000000000000888, -147.5625000027311842, 2.071067811865474617 ) ) ;
#14575=CARTESIAN_POINT ( 'NONE',  ( 3.061616997868383141E-16, -141.7500000000000284, -5.000000000000000000 ) ) ;
#14579=CARTESIAN_POINT ( 'NONE',  ( -3.152801135295367985, -165.0625000013656063, 3.152801135295367096 ) ) ;
#14580=CARTESIAN_POINT ( 'NONE',  ( 2.229367062500001939, -31.97916666530106866, 3.861377020970579999 ) ) ;
#14585=CARTESIAN_POINT ( 'NONE',  ( -1.846868145590737420, -145.7500000013655779, 4.458734124999999437 ) ) ;
#14587=CARTESIAN_POINT ( 'NONE',  ( 2.500000000000002220, -89.54166666393547303, 4.330127018922192761 ) ) ;
#14588=CARTESIAN_POINT ( 'NONE',  ( 2.229367062499998831, -57.89583333196773651, -3.861377020970580887 ) ) ;
#14590=CARTESIAN_POINT ( 'NONE',  ( -6.972266317189433020E-16, 13.87500000273118594, -5.000000000000000000 ) ) ;
#14591=CARTESIAN_POINT ( 'NONE',  ( -4.999999999999999112, 21.08333333333333215, 2.886751345948131764 ) ) ;
#14595=CARTESIAN_POINT ( 'NONE',  ( 6.123233995736766282E-16, -170.0000000000000000, -5.000000000000000000 ) ) ;
#14596=CARTESIAN_POINT ( 'NONE',  ( -4.458734124999998549, -5.229166665301072214, 2.574251347313722516 ) ) ;
#14597=CARTESIAN_POINT ( 'NONE',  ( 0.000000000000000000, -170.0000000000000000, 5.000000000000000000 ) ) ;
#14598=CARTESIAN_POINT ( 'NONE',  ( -9.184850993605147944E-16, -165.3750000027312126, 5.000000000000000000 ) ) ;
#14599=CARTESIAN_POINT ( 'NONE',  ( 2.071067811865370256, -157.9375000027312126, -5.000000000000105693 ) ) ;
#14601=ADVANCED_FACE ( 'NONE', ( #10755 ), #55469, .T. ) ;
#14602=DIRECTION ( 'NONE',  ( -0.000000000000000000, 1.000000000000000000, -0.000000000000000000 ) ) ;
#14603=CARTESIAN_POINT ( 'NONE',  ( 0.000000000000000000, -170.0000000000000000, 5.000000000000000000 ) ) ;
#14606=CARTESIAN_POINT ( 'NONE',  ( -2.229367062499996610, -56.14583333196773651, 3.861377020970582219 ) ) ;
#14607=CARTESIAN_POINT ( 'NONE',  ( -4.458734125000000326, -154.2500000013656063, -1.846868145590735644 ) ) ;
#14608=EDGE_CURVE ( 'NONE', #55393, #3859, #41144, .T. ) ;
#14610=CARTESIAN_POINT ( 'NONE',  ( 5.000000000000000000, -48.29166666393547303, -2.886751345948129988 ) ) ;
#14611=VERTEX_POINT ( 'NONE', #22004 ) ;
#14612=CARTESIAN_POINT ( 'NONE',  ( 2.229367062500001939, 3.770833334698926009, 3.861377020970579999 ) ) ;
#14614=CARTESIAN_POINT ( 'NONE',  ( -6.972266317189433020E-16, -3.124999997268813612, -5.000000000000000000 ) ) ;
#14616=CARTESIAN_POINT ( 'NONE',  ( 4.458734124999999437, -158.5000000013656631, 1.846868145590737864 ) ) ;
#14617=ORIENTED_EDGE ( 'NONE', *, *, #13991, .F. ) ;
#14621=CARTESIAN_POINT ( 'NONE',  ( 1.975475456537005874E-15, -58.62499999726879452, 5.000000000000000000 ) ) ;
#14622=CARTESIAN_POINT ( 'NONE',  ( 4.458734124999998549, -43.97916666530105800, -2.574251347313721627 ) ) ;
#14626=DIRECTION ( 'NONE',  ( -0.000000000000000000, 1.000000000000000000, -0.000000000000000000 ) ) ;
#14628=CARTESIAN_POINT ( 'NONE',  ( -4.458734124999999437, 26.68750000136559564, 0.000000000000000000 ) ) ;
#14633=CARTESIAN_POINT ( 'NONE',  ( -6.972266317189433020E-16, -62.12499999726880162, -5.000000000000000000 ) ) ;
#14635=CARTESIAN_POINT ( 'NONE',  ( -1.339745962155610925, 7.205341801261477386, 5.000000000000000000 ) ) ;
#14638=DIRECTION ( 'NONE',  ( 0.000000000000000000, 0.000000000000000000, 1.000000000000000000 ) ) ;
#14639=CARTESIAN_POINT ( 'NONE',  ( 0.000000000000000000, -170.0000000000000000, 5.000000000000000000 ) ) ;
#14640=DIRECTION ( 'NONE',  ( -0.000000000000000000, 1.000000000000000000, -0.000000000000000000 ) ) ;
#14643=ORIENTED_EDGE ( 'NONE', *, *, #27594, .T. ) ;
#14644=CARTESIAN_POINT ( 'NONE',  ( 5.000000000000000888, -9.458333330602146205, 2.886751345948126879 ) ) ;
#14646=CARTESIAN_POINT ( 'NONE',  ( 3.535533905932736864, -160.2500000027312126, 3.535533905932738641 ) ) ;
#14648=CARTESIAN_POINT ( 'NONE',  ( 2.071067811865540342, -163.3125000027312126, 4.999999999999936051 ) ) ;
#14656=CARTESIAN_POINT ( 'NONE',  ( -1.339745962155613812, -54.20534180126147561, -5.000000000000000000 ) ) ;
#14657=CARTESIAN_POINT ( 'NONE',  ( -4.458734124999999437, -13.31249999863440259, 0.000000000000000000 ) ) ;
#14659=CARTESIAN_POINT ( 'NONE',  ( 3.535533905932736864, -154.1250000000000000, 3.535533905932738641 ) ) ;
#14662=CARTESIAN_POINT ( 'NONE',  ( 2.229367062499998831, -41.89583333196773651, -3.861377020970580887 ) ) ;
#14663=( BOUNDED_CURVE ( )  B_SPLINE_CURVE ( 2, ( #58412, #39093, #30401, #10462, #58722, #25263, #19479, #19797, #5333 ),
 .UNSPECIFIED., .F., .F. ) 
 B_SPLINE_CURVE_WITH_KNOTS ( ( 3, 2, 2, 2, 3 ),
 ( 0.6520833333333333481, 0.6527777777777777901, 0.6541666666666666741, 0.6555555555555555580, 0.6562500000000000000 ),
 .UNSPECIFIED. ) 
 CURVE ( )  GEOMETRIC_REPRESENTATION_ITEM ( )  RATIONAL_B_SPLINE_CURVE ( ( 0.9330127018922194093, 0.9330127018922194093, 1.000000000000000000, 0.8660254037844387076, 1.000000000000000000, 0.8660254037844387076, 1.000000000000000000, 0.9330127018922194093, 0.9330127018922194093 ) ) 
 REPRESENTATION_ITEM ( '' )  );
#14665=CARTESIAN_POINT ( 'NONE',  ( -2.500000000000000444, -12.16666666666666607, -4.330127018922193649 ) ) ;
#14669=CARTESIAN_POINT ( 'NONE',  ( 4.458734124999999437, 9.187500001365592084, -5.460374474430324690E-16 ) ) ;
#14671=CARTESIAN_POINT ( 'NONE',  ( -2.071067811865435981, -165.4375000027311557, 5.000000000000041744 ) ) ;
#14672=CARTESIAN_POINT ( 'NONE',  ( -4.458734124999999437, -89.56249999863440792, 0.000000000000000000 ) ) ;
#14673=CARTESIAN_POINT ( 'NONE',  ( 4.458734124999998549, 23.02083333469892423, -2.574251347313721627 ) ) ;
#14675=CARTESIAN_POINT ( 'NONE',  ( -2.500000000000000444, 15.95833333606451809, -4.330127018922193649 ) ) ;
#14678=CARTESIAN_POINT ( 'NONE',  ( -2.500000000000000444, -7.041666663935481907, -4.330127018922193649 ) ) ;
#14680=CYLINDRICAL_SURFACE ( 'NONE', #30619, 5.000000000000000000 ) ;
#14681=CARTESIAN_POINT ( 'NONE',  ( -2.500000000000000444, -35.16666666666666430, -4.330127018922193649 ) ) ;
#14682=CARTESIAN_POINT ( 'NONE',  ( -2.229367062499996610, -39.14583333196773651, 3.861377020970582219 ) ) ;
#14684=ADVANCED_FACE ( 'NONE', ( #22323 ), #51597, .T. ) ;
#14685=CARTESIAN_POINT ( 'NONE',  ( 5.000000000000000000, -34.29166666393547303, -2.886751345948129988 ) ) ;
#14686=CARTESIAN_POINT ( 'NONE',  ( -4.458734124999998549, -65.22916666530106511, 2.574251347313722516 ) ) ;
#14687=ORIENTED_EDGE ( 'NONE', *, *, #445, .T. ) ;
#14689=CARTESIAN_POINT ( 'NONE',  ( 4.458734124999998549, -14.72916666530107399, -2.574251347313721627 ) ) ;
#14690=CARTESIAN_POINT ( 'NONE',  ( 2.229367062500001939, -15.22916666530107399, 3.861377020970579999 ) ) ;
#14692=CARTESIAN_POINT ( 'NONE',  ( 5.000000000000000000, -82.50000000000000000, -6.123233995736766282E-16 ) ) ;
#14695=CARTESIAN_POINT ( 'NONE',  ( -3.535250795749689387E-16, -82.12499999726883004, -5.773502691896257311 ) ) ;
#14696=CARTESIAN_POINT ( 'NONE',  ( -5.000000000000000000, -18.08333333333333215, -2.886751345948128211 ) ) ;
#14699=CARTESIAN_POINT ( 'NONE',  ( 2.229367062500001939, -29.22916666530107221, 3.861377020970579999 ) ) ;
#14700=VERTEX_POINT ( 'NONE', #47082 ) ;
#14701=CARTESIAN_POINT ( 'NONE',  ( 3.152801135295367541, -168.5625000013656063, -3.152801135295367541 ) ) ;
#14703=CARTESIAN_POINT ( 'NONE',  ( -6.972266317189433020E-16, -55.12499999726880873, -5.000000000000000000 ) ) ;
#14708=CARTESIAN_POINT ( 'NONE',  ( -4.458734125000000326, -148.1250000013655779, 1.846868145590734089 ) ) ;
#14710=CARTESIAN_POINT ( 'NONE',  ( -2.499999999999996447, 0.1666666666666656582, 4.330127018922195425 ) ) ;
#14714=CARTESIAN_POINT ( 'NONE',  ( -4.458734124999999437, -146.1875000013656063, -5.460374474430324690E-16 ) ) ;
#14719=CARTESIAN_POINT ( 'NONE',  ( -4.458734124999998549, -73.47916666530106511, 2.574251347313722516 ) ) ;
#14721=CARTESIAN_POINT ( 'NONE',  ( 1.339745962155612702, -54.16965819600732601, -5.000000000000000000 ) ) ;
#14725=DIRECTION ( 'NONE',  ( -0.000000000000000000, 1.000000000000000000, -0.000000000000000000 ) ) ;
#14731=CARTESIAN_POINT ( 'NONE',  ( 4.458734125000000326, 23.85416666803225993, 2.574251347313718519 ) ) ;
#14732=CARTESIAN_POINT ( 'NONE',  ( 1.975475456537005874E-15, -18.74999999999999645, 5.000000000000000000 ) ) ;
#14733=AXIS2_PLACEMENT_3D ( 'NONE', #8478, #37746, #48641 ) ;
#14738=CARTESIAN_POINT ( 'NONE',  ( -6.972266317189433020E-16, -51.12499999726880873, -5.000000000000000000 ) ) ;
#14739=CARTESIAN_POINT ( 'NONE',  ( -4.458734124999999437, -0.3124999986344051406, 0.000000000000000000 ) ) ;
#14741=CARTESIAN_POINT ( 'NONE',  ( -2.229367062500000163, -24.72916666530106866, -3.861377020970580443 ) ) ;
#14744=CARTESIAN_POINT ( 'NONE',  ( -2.229367062499996610, 24.85416666803225993, 3.861377020970582219 ) ) ;
#14747=CARTESIAN_POINT ( 'NONE',  ( 2.229367062500001939, -72.22916666530107932, 3.861377020970579999 ) ) ;
#14749=CARTESIAN_POINT ( 'NONE',  ( 2.500000000000002220, -73.66666666666665719, 4.330127018922192761 ) ) ;
#14750=CARTESIAN_POINT ( 'NONE',  ( 5.000000000000000000, -156.1250000027311842, 0.000000000000000000 ) ) ;
#14751=VERTEX_POINT ( 'NONE', #36797 ) ;
#14753=CARTESIAN_POINT ( 'NONE',  ( -6.972266317189433020E-16, 2.875000002731185500, -5.000000000000000000 ) ) ;
#14754=CARTESIAN_POINT ( 'NONE',  ( 5.000000000000000000, -20.41666666666666430, -2.886751345948129988 ) ) ;
#14755=CARTESIAN_POINT ( 'NONE',  ( -2.229367062500000163, -20.47916666530107221, -3.861377020970580443 ) ) ;
#14756=CARTESIAN_POINT ( 'NONE',  ( 9.457646018065525792E-16, -85.06249999863440792, 5.148502694627439702 ) ) ;
#14757=CARTESIAN_POINT ( 'NONE',  ( 3.152801135295367541, -166.5625000013656063, -3.152801135295367541 ) ) ;
#14758=CARTESIAN_POINT ( 'NONE',  ( 1.060575238724906964E-15, -18.62499999726881583, 5.773502691896257311 ) ) ;
#14759=CARTESIAN_POINT ( 'NONE',  ( 2.229367062500001939, -48.97916666530107221, 3.861377020970579999 ) ) ;
#14762=CARTESIAN_POINT ( 'NONE',  ( 1.062108568985190270E-13, -28.12499999726880873, -4.999999999999999112 ) ) ;
#14763=CARTESIAN_POINT ( 'NONE',  ( -4.458734124999999437, 0.4375000013655955255, 0.000000000000000000 ) ) ;
#14764=ORIENTED_EDGE ( 'NONE', *, *, #61736, .T. ) ;
#14766=CARTESIAN_POINT ( 'NONE',  ( 1.060575238724906964E-15, -67.75000000000000000, 5.773502691896257311 ) ) ;
#14767=CARTESIAN_POINT ( 'NONE',  ( -8.190561711645485556E-16, -156.9375000013655779, 4.458734124999999437 ) ) ;
#14770=CARTESIAN_POINT ( 'NONE',  ( -2.071067811865478170, -162.3125000000000284, 5.000000000000000000 ) ) ;
#14773=CARTESIAN_POINT ( 'NONE',  ( 2.229367062499998831, -8.895833331967736513, -3.861377020970580887 ) ) ;
#14774=CARTESIAN_POINT ( 'NONE',  ( -4.458734124999999437, -48.64583333196773651, -2.574251347313719407 ) ) ;
#14775=VECTOR ( 'NONE', #58790, 1000.000000000000000 ) ;
#14776=CARTESIAN_POINT ( 'NONE',  ( -1.339745962155613812, -8.080341798530294994, -5.000000000000000000 ) ) ;
#14777=CARTESIAN_POINT ( 'NONE',  ( -1.846868145590737420, -146.7500000013656063, 4.458734124999999437 ) ) ;
#14779=CARTESIAN_POINT ( 'NONE',  ( 3.535533905932736864, -167.2500000027312126, 3.535533905932738641 ) ) ;
#14780=EDGE_LOOP ( 'NONE', ( #33898, #20820, #59954, #16927 ) ) ;
#14782=CARTESIAN_POINT ( 'NONE',  ( 6.123233995736766282E-16, -170.0000000000000000, -5.000000000000000000 ) ) ;
#14785=CARTESIAN_POINT ( 'NONE',  ( -1.339745962155610925, -61.79465819873851729, 5.000000000000000000 ) ) ;
#14792=CARTESIAN_POINT ( 'NONE',  ( -6.972266317189433020E-16, 1.875000002731185722, -5.000000000000000000 ) ) ;
#14793=CARTESIAN_POINT ( 'NONE',  ( 4.458734125000001214, -0.8958333319677401763, 2.574251347313718519 ) ) ;
#14795=CARTESIAN_POINT ( 'NONE',  ( -3.152801135295367096, -154.0625000013656063, -3.152801135295367541 ) ) ;
#14801=CARTESIAN_POINT ( 'NONE',  ( 1.975475456537005874E-15, -33.62499999726880873, 5.000000000000000000 ) ) ;
#14802=CARTESIAN_POINT ( 'NONE',  ( 5.000000000000000888, 29.41666666666666785, 2.886751345948126879 ) ) ;
#14805=LINE ( 'NONE', #50182, #6568 ) ;
#14809=CARTESIAN_POINT ( 'NONE',  ( 2.229367062500001939, 16.02083333469892779, 3.861377020970579999 ) ) ;
#14811=ORIENTED_EDGE ( 'NONE', *, *, #29103, .T. ) ;
#14812=CARTESIAN_POINT ( 'NONE',  ( -3.152548672688508926E-16, -10.81249999863440792, -5.148502694627439702 ) ) ;
#14815=CARTESIAN_POINT ( 'NONE',  ( -3.152801135295367096, -168.0625000013656063, -3.152801135295367541 ) ) ;
#14816=CARTESIAN_POINT ( 'NONE',  ( 5.000000000000000888, -63.45833333060215153, 2.886751345948126879 ) ) ;
#14820=CARTESIAN_POINT ( 'NONE',  ( -1.339745962155610925, -76.79465819873853150, 5.000000000000000000 ) ) ;
#14821=CARTESIAN_POINT ( 'NONE',  ( 3.535533905932736864, -142.2500000027311842, 3.535533905932738641 ) ) ;
#14822=LINE ( 'NONE', #25766, #10044 ) ;
#14823=CARTESIAN_POINT ( 'NONE',  ( 4.458734124999997661, -154.7500000013656063, 1.846868145590737864 ) ) ;
#14831=CARTESIAN_POINT ( 'NONE',  ( 2.500000000000002220, -3.666666666666665186, 4.330127018922192761 ) ) ;
#14832=CARTESIAN_POINT ( 'NONE',  ( -2.229367062499996610, -69.14583333196773651, 3.861377020970582219 ) ) ;
#14834=CARTESIAN_POINT ( 'NONE',  ( -4.999999999999999112, -1.791666663935480353, 2.886751345948131764 ) ) ;
#14835=CARTESIAN_POINT ( 'NONE',  ( 9.457646018065525792E-16, -33.06249999863440792, 5.148502694627439702 ) ) ;
#14836=EDGE_LOOP ( 'NONE', ( #31588, #21110, #31381, #54750 ) ) ;
#14838=CARTESIAN_POINT ( 'NONE',  ( -5.000000000000000000, -47.95833333060215153, -2.886751345948128211 ) ) ;
#14839=( BOUNDED_CURVE ( )  B_SPLINE_CURVE ( 2, ( #647, #6110, #59501, #10285, #983, #59829, #40820, #25725, #1305 ),
 .UNSPECIFIED., .F., .F. ) 
 B_SPLINE_CURVE_WITH_KNOTS ( ( 3, 2, 2, 2, 3 ),
 ( 0.06458333333333333981, 0.06527777777777778179, 0.06666666666666666574, 0.06805555555555554970, 0.06875000000000000555 ),
 .UNSPECIFIED. ) 
 CURVE ( )  GEOMETRIC_REPRESENTATION_ITEM ( )  RATIONAL_B_SPLINE_CURVE ( ( 0.9330127018922194093, 0.9330127018922200755, 1.000000000000000000, 0.8660254037844387076, 1.000000000000000000, 0.8660254037844387076, 1.000000000000000000, 0.9330127018922187432, 0.9330127018922194093 ) ) 
 REPRESENTATION_ITEM ( '' )  );
#14841=CARTESIAN_POINT ( 'NONE',  ( -5.000000000000000000, -46.08333333333333570, -2.886751345948128211 ) ) ;
#14842=CARTESIAN_POINT ( 'NONE',  ( 0.000000000000000000, -170.0000000000000000, 0.000000000000000000 ) ) ;
#14843=( BOUNDED_CURVE ( )  B_SPLINE_CURVE ( 2, ( #34599, #10168, #29772, #4393, #48139, #24012, #3775, #18563, #38186 ),
 .UNSPECIFIED., .F., .F. ) 
 B_SPLINE_CURVE_WITH_KNOTS ( ( 3, 2, 2, 2, 3 ),
 ( 0.01458333333333333356, 0.01527777777777777728, 0.01666666666666666644, 0.01805555555555555386, 0.01874999999999999931 ),
 .UNSPECIFIED. ) 
 CURVE ( )  GEOMETRIC_REPRESENTATION_ITEM ( )  RATIONAL_B_SPLINE_CURVE ( ( 0.9330127018922192983, 0.9330127018922194093, 1.000000000000000000, 0.8660254037844387076, 1.000000000000000000, 0.8660254037844387076, 1.000000000000000000, 0.9330127018922194093, 0.9330127018922194093 ) ) 
 REPRESENTATION_ITEM ( '' )  );
#14845=CARTESIAN_POINT ( 'NONE',  ( 2.071067811865645591, -155.1875000000000000, 4.999999999999830358 ) ) ;
#14846=CARTESIAN_POINT ( 'NONE',  ( -4.458734124999999437, -68.31249999863439371, 0.000000000000000000 ) ) ;
#14847=CARTESIAN_POINT ( 'NONE',  ( -3.152801135295367985, -143.0625000013655779, 3.152801135295367096 ) ) ;
#14848=CARTESIAN_POINT ( 'NONE',  ( -3.152548672688508926E-16, -82.56249999863442213, -5.148502694627439702 ) ) ;
#14850=CARTESIAN_POINT ( 'NONE',  ( 4.458734124999998549, -32.97916666530106511, -2.574251347313721627 ) ) ;
#14851=CARTESIAN_POINT ( 'NONE',  ( -2.499999999999996447, -73.70833333060214443, 4.330127018922195425 ) ) ;
#14852=VERTEX_POINT ( 'NONE', #32278 ) ;
#14853=CARTESIAN_POINT ( 'NONE',  ( 0.000000000000000000, -170.0000000000000000, 5.000000000000000000 ) ) ;
#14854=ORIENTED_EDGE ( 'NONE', *, *, #55946, .F. ) ;
#14858=CARTESIAN_POINT ( 'NONE',  ( 2.500000000000002220, 27.33333333333333215, 4.330127018922192761 ) ) ;
#14859=CARTESIAN_POINT ( 'NONE',  ( 2.500000000000002220, -12.66666666666666607, 4.330127018922192761 ) ) ;
#14860=CARTESIAN_POINT ( 'NONE',  ( -3.152548672688508926E-16, -59.81249999863440792, -5.148502694627439702 ) ) ;
#14861=EDGE_CURVE ( 'NONE', #30862, #13218, #7846, .T. ) ;
#14863=ORIENTED_EDGE ( 'NONE', *, *, #41328, .T. ) ;
#14864=VECTOR ( 'NONE', #47533, 1000.000000000000000 ) ;
#14865=FACE_OUTER_BOUND ( 'NONE', #9176, .T. ) ;
#14867=( BOUNDED_CURVE ( )  B_SPLINE_CURVE ( 2, ( #54489, #29705, #10417, #4633, #30028, #49657, #10738, #45148, #21348 ),
 .UNSPECIFIED., .F., .F. ) 
 B_SPLINE_CURVE_WITH_KNOTS ( ( 3, 2, 2, 2, 3 ),
 ( 0.09166666666666674346, 0.09583333333333342308, 0.1000000000000000888, 0.1041666666666667546, 0.1083333333333334203 ),
 .UNSPECIFIED. ) 
 CURVE ( )  GEOMETRIC_REPRESENTATION_ITEM ( )  RATIONAL_B_SPLINE_CURVE ( ( 0.9999999999999984457, 0.9238795325112882928, 1.000000000000000000, 0.9238795325112867385, 1.000000000000000000, 0.9238795325112867385, 1.000000000000000000, 0.9238795325112851842, 1.000000000000001554 ) ) 
 REPRESENTATION_ITEM ( '' )  );
#14868=CARTESIAN_POINT ( 'NONE',  ( -4.458734124999999437, 12.68750000136559564, 0.000000000000000000 ) ) ;
#14870=CARTESIAN_POINT ( 'NONE',  ( 5.000000000000000888, -27.45833333060214798, 2.886751345948126879 ) ) ;
#14871=CARTESIAN_POINT ( 'NONE',  ( 1.846868145590736310, -163.6250000013656063, 4.458734124999997661 ) ) ;
#14872=ORIENTED_EDGE ( 'NONE', *, *, #56312, .T. ) ;
#14874=CARTESIAN_POINT ( 'NONE',  ( 2.499999999999998668, -39.33333333333332860, -4.330127018922193649 ) ) ;
#14877=EDGE_CURVE ( 'NONE', #23954, #48784, #4161, .T. ) ;
#14883=CARTESIAN_POINT ( 'NONE',  ( 5.000000000000000000, -61.50000000000000000, -6.123233995736766282E-16 ) ) ;
#14887=CARTESIAN_POINT ( 'NONE',  ( -2.229367062499996610, 9.604166668032261711, 3.861377020970582219 ) ) ;
#14889=CARTESIAN_POINT ( 'NONE',  ( 0.000000000000000000, -170.0000000000000000, 0.000000000000000000 ) ) ;
#14891=CARTESIAN_POINT ( 'NONE',  ( -5.000000000000000888, -150.6875000027312126, -2.071067811865475949 ) ) ;
#14892=CARTESIAN_POINT ( 'NONE',  ( -1.339745962155612258, 29.20534180126147916, 5.000000000000000000 ) ) ;
#14897=CARTESIAN_POINT ( 'NONE',  ( 3.535533905932736864, -143.1250000000000000, 3.535533905932738641 ) ) ;
#14898=CARTESIAN_POINT ( 'NONE',  ( 3.535533905932738197, -141.0000000027311842, -3.535533905932738197 ) ) ;
#14900=CARTESIAN_POINT ( 'NONE',  ( -4.458734125000000326, -164.1250000013656063, 1.846868145590734089 ) ) ;
#14901=CARTESIAN_POINT ( 'NONE',  ( 4.458734124999998549, -33.72916666530107221, -2.574251347313721627 ) ) ;
#14905=CARTESIAN_POINT ( 'NONE',  ( -4.458734125000000326, -144.0000000013655779, -1.846868145590735644 ) ) ;
#14906=ORIENTED_EDGE ( 'NONE', *, *, #59057, .F. ) ;
#14908=CARTESIAN_POINT ( 'NONE',  ( 5.000000000000000000, -90.29166666393547303, -2.886751345948129988 ) ) ;
#14909=VERTEX_POINT ( 'NONE', #4577 ) ;
#14910=CARTESIAN_POINT ( 'NONE',  ( -2.229367062499996610, -60.39583333196774362, 3.861377020970582219 ) ) ;
#14912=CARTESIAN_POINT ( 'NONE',  ( -2.500000000000000444, 14.83333333333333215, -4.330127018922193649 ) ) ;
#14913=CARTESIAN_POINT ( 'NONE',  ( -2.229367062499996610, -53.14583333196773651, 3.861377020970582219 ) ) ;
#14915=CARTESIAN_POINT ( 'NONE',  ( 2.229367062499998831, -4.645833331967740065, -3.861377020970580887 ) ) ;
#14916=CARTESIAN_POINT ( 'NONE',  ( -4.999999999999998224, -22.91666666666666785, 2.886751345948131764 ) ) ;
#14917=EDGE_CURVE ( 'NONE', #62567, #27206, #23875, .T. ) ;
#14919=CARTESIAN_POINT ( 'NONE',  ( 2.071067811865582087, -158.3125000027312126, 4.999999999999894307 ) ) ;
#14924=CARTESIAN_POINT ( 'NONE',  ( -4.458734124999999437, -55.31249999863440081, 0.000000000000000000 ) ) ;
#14925=CARTESIAN_POINT ( 'NONE',  ( 1.846868145590735200, -155.5000000013655779, -4.458734125000000326 ) ) ;
#14926=CARTESIAN_POINT ( 'NONE',  ( -5.000000000000000000, -54.87499999726880162, 0.000000000000000000 ) ) ;
#14928=CARTESIAN_POINT ( 'NONE',  ( 5.000000000000000000, -26.49999999999999645, -6.123233995736766282E-16 ) ) ;
#14929=CARTESIAN_POINT ( 'NONE',  ( -2.229367062499996610, 6.604166668032259935, 3.861377020970582219 ) ) ;
#14931=CYLINDRICAL_SURFACE ( 'NONE', #37887, 5.000000000000000000 ) ;
#14933=CARTESIAN_POINT ( 'NONE',  ( -3.152801135295367985, -157.8125000013656063, 3.152801135295367096 ) ) ;
#14934=VERTEX_POINT ( 'NONE', #34468 ) ;
#14935=CARTESIAN_POINT ( 'NONE',  ( 2.500000000000002220, -87.54166666393547303, 4.330127018922192761 ) ) ;
#14937=CARTESIAN_POINT ( 'NONE',  ( -5.000000000000000000, -58.87499999726880873, 0.000000000000000000 ) ) ;
#14938=CARTESIAN_POINT ( 'NONE',  ( 2.229367062499998831, -42.89583333196773651, -3.861377020970580887 ) ) ;
#14942=EDGE_CURVE ( 'NONE', #56674, #28481, #8784, .T. ) ;
#14943=CARTESIAN_POINT ( 'NONE',  ( -2.071067811865391128, -145.6875000000000284, -5.000000000000086153 ) ) ;
#14947=CARTESIAN_POINT ( 'NONE',  ( -2.229367062499996610, 28.85416666803226349, 3.861377020970582219 ) ) ;
#14955=EDGE_CURVE ( 'NONE', #58407, #30540, #25940, .T. ) ;
#14960=CARTESIAN_POINT ( 'NONE',  ( 1.975475456537005874E-15, 5.250000000000000000, 5.000000000000000000 ) ) ;
#14961=EDGE_CURVE ( 'NONE', #43716, #62883, #59190, .T. ) ;
#14963=CARTESIAN_POINT ( 'NONE',  ( -2.229367062500000163, -87.72916666530107932, -3.861377020970580443 ) ) ;
#14966=ORIENTED_EDGE ( 'NONE', *, *, #31900, .F. ) ;
#14967=CARTESIAN_POINT ( 'NONE',  ( -3.535533905932737309, -169.6250000000000284, -3.535533905932738197 ) ) ;
#14969=CARTESIAN_POINT ( 'NONE',  ( 5.000000000000000888, -161.0625000027312126, -2.071067811865475505 ) ) ;
#14971=CARTESIAN_POINT ( 'NONE',  ( 2.499999999999998668, -19.20833333060214798, -4.330127018922193649 ) ) ;
#14981=CARTESIAN_POINT ( 'NONE',  ( 4.458734125000000326, -16.89583333196773651, 2.574251347313718519 ) ) ;
#14983=CARTESIAN_POINT ( 'NONE',  ( 5.000000000000000000, -153.0625000000000000, 2.071067811865478614 ) ) ;
#14986=CARTESIAN_POINT ( 'NONE',  ( 2.229367062499998831, -48.89583333196772941, -3.861377020970580887 ) ) ;
#14987=CARTESIAN_POINT ( 'NONE',  ( -2.499999999999996447, 26.16666666666666430, 4.330127018922195425 ) ) ;
#14992=CARTESIAN_POINT ( 'NONE',  ( -2.229367062500000163, 9.520833334698927786, -3.861377020970580443 ) ) ;
#14993=( BOUNDED_CURVE ( )  B_SPLINE_CURVE ( 2, ( #8605, #47829, #53296, #57821, #28215, #3790, #37883, #52363, #19189 ),
 .UNSPECIFIED., .F., .F. ) 
 B_SPLINE_CURVE_WITH_KNOTS ( ( 3, 2, 2, 2, 3 ),
 ( 0.1145833333333333426, 0.1152777777777777846, 0.1166666666666666685, 0.1180555555555555525, 0.1187500000000000083 ),
 .UNSPECIFIED. ) 
 CURVE ( )  GEOMETRIC_REPRESENTATION_ITEM ( )  RATIONAL_B_SPLINE_CURVE ( ( 0.9330127018922194093, 0.9330127018922200755, 1.000000000000000000, 0.8660254037844387076, 1.000000000000000000, 0.8660254037844387076, 1.000000000000000000, 0.9330127018922187432, 0.9330127018922194093 ) ) 
 REPRESENTATION_ITEM ( '' )  );
#14994=CARTESIAN_POINT ( 'NONE',  ( -2.500000000000000444, -44.16666666666665719, -4.330127018922193649 ) ) ;
#14995=CARTESIAN_POINT ( 'NONE',  ( -2.229367062500000163, -87.72916666530107932, -3.861377020970580443 ) ) ;
#14996=CARTESIAN_POINT ( 'NONE',  ( 4.458734125000001214, 19.85416666803226349, 2.574251347313718519 ) ) ;
#14998=CARTESIAN_POINT ( 'NONE',  ( -4.999999999999999112, 7.208333336064517205, 2.886751345948131764 ) ) ;
#15001=ORIENTED_EDGE ( 'NONE', *, *, #5119, .T. ) ;
#15004=CARTESIAN_POINT ( 'NONE',  ( -4.999999999999999112, -33.91666666666666430, 2.886751345948131764 ) ) ;
#15005=CARTESIAN_POINT ( 'NONE',  ( -3.152548672688508926E-16, -40.56249999863440081, -5.148502694627439702 ) ) ;
#15007=CARTESIAN_POINT ( 'NONE',  ( 5.000000000000000888, -33.45833333060215153, 2.886751345948126879 ) ) ;
#15008=ORIENTED_EDGE ( 'NONE', *, *, #44726, .T. ) ;
#15010=CARTESIAN_POINT ( 'NONE',  ( -4.458734124999999437, -11.39583333196774007, -2.574251347313719407 ) ) ;
#15011=CARTESIAN_POINT ( 'NONE',  ( -4.458734124999999437, -16.56249999863440436, 0.000000000000000000 ) ) ;
#15012=ORIENTED_EDGE ( 'NONE', *, *, #61486, .F. ) ;
#15013=CARTESIAN_POINT ( 'NONE',  ( -5.000000000000000000, -84.08333333333332860, -2.886751345948128211 ) ) ;
#15014=CARTESIAN_POINT ( 'NONE',  ( 4.458734125000000326, -169.3750000013656347, -1.846868145590734978 ) ) ;
#15016=CARTESIAN_POINT ( 'NONE',  ( 1.060575238724906964E-15, -83.62499999726881583, 5.773502691896257311 ) ) ;
#15017=DIRECTION ( 'NONE',  ( -0.000000000000000000, 1.000000000000000000, -0.000000000000000000 ) ) ;
#15018=EDGE_LOOP ( 'NONE', ( #39066, #19526, #59859, #56243 ) ) ;
#15020=CARTESIAN_POINT ( 'NONE',  ( -4.458734124999999437, -28.64583333196774007, -2.574251347313719407 ) ) ;
#15021=CARTESIAN_POINT ( 'NONE',  ( -2.499999999999996447, -49.83333333333332860, 4.330127018922195425 ) ) ;
#15022=ORIENTED_EDGE ( 'NONE', *, *, #62834, .F. ) ;
#15023=EDGE_CURVE ( 'NONE', #41751, #10933, #18977, .T. ) ;
#15025=CARTESIAN_POINT ( 'NONE',  ( -3.152801135295367096, -163.3125000013656063, -3.152801135295367541 ) ) ;
#15027=CARTESIAN_POINT ( 'NONE',  ( -6.972266317189433020E-16, -23.24999999999999645, -5.000000000000000000 ) ) ;
#15030=CARTESIAN_POINT ( 'NONE',  ( 9.457646018065525792E-16, -73.31249999863440792, 5.148502694627439702 ) ) ;
#15033=CARTESIAN_POINT ( 'NONE',  ( -3.152801135295367985, -147.0625000013655779, 3.152801135295367096 ) ) ;
#15035=CARTESIAN_POINT ( 'NONE',  ( 1.975475456537005874E-15, 6.375000002731185944, 5.000000000000000000 ) ) ;
#15036=CARTESIAN_POINT ( 'NONE',  ( -4.999999999999998224, 0.08333333333333454995, 2.886751345948131764 ) ) ;
#15037=EDGE_CURVE ( 'NONE', #5644, #29232, #43574, .T. ) ;
#15040=ORIENTED_EDGE ( 'NONE', *, *, #52830, .T. ) ;
#15044=CARTESIAN_POINT ( 'NONE',  ( -6.972266317189433020E-16, -86.12499999726880162, -5.000000000000000000 ) ) ;
#15046=CARTESIAN_POINT ( 'NONE',  ( -4.458734124999999437, -73.64583333196773651, -2.574251347313719407 ) ) ;
#15049=CARTESIAN_POINT ( 'NONE',  ( -6.972266317189433020E-16, -70.25000000000000000, -5.000000000000000000 ) ) ;
#15050=CYLINDRICAL_SURFACE ( 'NONE', #62423, 5.000000000000000000 ) ;
#15053=ORIENTED_EDGE ( 'NONE', *, *, #51137, .T. ) ;
#15054=AXIS2_PLACEMENT_3D ( 'NONE', #4476, #28290, #53052 ) ;
#15055=CARTESIAN_POINT ( 'NONE',  ( 2.071067811865560326, -145.8125000000000284, -4.999999999999914735 ) ) ;
#15063=CARTESIAN_POINT ( 'NONE',  ( -4.458734124999999437, 19.43750000136559208, 0.000000000000000000 ) ) ;
#15064=CARTESIAN_POINT ( 'NONE',  ( -2.499999999999996447, 27.16666666666666430, 4.330127018922195425 ) ) ;
#15065=VECTOR ( 'NONE', #23602, 1000.000000000000000 ) ;
#15071=CARTESIAN_POINT ( 'NONE',  ( -2.229367062499996610, 2.854166668032259935, 3.861377020970582219 ) ) ;
#15072=CARTESIAN_POINT ( 'NONE',  ( -2.229367062500000163, -22.72916666530107221, -3.861377020970580443 ) ) ;
#15075=CARTESIAN_POINT ( 'NONE',  ( 9.457646018065525792E-16, 24.93750000136559564, 5.148502694627439702 ) ) ;
#15078=CARTESIAN_POINT ( 'NONE',  ( -4.458734124999997661, -70.47916666530107932, 2.574251347313722516 ) ) ;
#15080=CARTESIAN_POINT ( 'NONE',  ( -2.499999999999996447, -65.70833333060213022, 4.330127018922195425 ) ) ;
#15081=CARTESIAN_POINT ( 'NONE',  ( 5.000000000000000000, 25.62500000273118417, -6.123233995736766282E-16 ) ) ;
#15083=CARTESIAN_POINT ( 'NONE',  ( 1.339745962155612702, 6.705341801261480050, -5.000000000000000000 ) ) ;
#15084=( BOUNDED_CURVE ( )  B_SPLINE_CURVE ( 2, ( #48717, #43571, #49681, #54184, #4658, #20091, #23968, #35214, #63215 ),
 .UNSPECIFIED., .F., .F. ) 
 B_SPLINE_CURVE_WITH_KNOTS ( ( 3, 2, 2, 2, 3 ),
 ( 0.8583333333333330595, 0.8624999999999998224, 0.8666666666666664742, 0.8708333333333332371, 0.8749999999999998890 ),
 .UNSPECIFIED. ) 
 CURVE ( )  GEOMETRIC_REPRESENTATION_ITEM ( )  RATIONAL_B_SPLINE_CURVE ( ( 1.000000000000003997, 0.9238795325112826307, 1.000000000000000000, 0.9238795325112867385, 1.000000000000000000, 0.9238795325112867385, 1.000000000000000000, 0.9238795325112887369, 0.9999999999999980016 ) ) 
 REPRESENTATION_ITEM ( '' )  );
#15086=CARTESIAN_POINT ( 'NONE',  ( 2.500000000000002220, -17.66666666666666430, 4.330127018922192761 ) ) ;
#15087=CARTESIAN_POINT ( 'NONE',  ( -4.458734124999999437, -24.31249999863440436, 0.000000000000000000 ) ) ;
#15088=CARTESIAN_POINT ( 'NONE',  ( 2.229367062500001939, -83.97916666530106511, 3.861377020970579999 ) ) ;
#15089=CARTESIAN_POINT ( 'NONE',  ( 3.152801135295366208, -166.8125000013656063, 3.152801135295367985 ) ) ;
#15090=CARTESIAN_POINT ( 'NONE',  ( 2.500000000000002220, -16.54166666393548368, 4.330127018922192761 ) ) ;
#15091=CARTESIAN_POINT ( 'NONE',  ( 4.458734124999998549, -50.72916666530107932, -2.574251347313721627 ) ) ;
#15094=CARTESIAN_POINT ( 'NONE',  ( 4.458734125000001214, -0.1458333319677394824, 2.574251347313718519 ) ) ;
#15097=CARTESIAN_POINT ( 'NONE',  ( 5.000000000000000000, -64.50000000000000000, -6.123233995736766282E-16 ) ) ;
#15098=CARTESIAN_POINT ( 'NONE',  ( 4.458734124999999437, -151.7500000013655779, 1.846868145590737864 ) ) ;
#15101=CARTESIAN_POINT ( 'NONE',  ( 2.071067811865475505, -162.8125000000000000, -5.000000000000000888 ) ) ;
#15105=CARTESIAN_POINT ( 'NONE',  ( 2.229367062500001939, -9.229166665301075767, 3.861377020970579999 ) ) ;
#15106=AXIS2_PLACEMENT_3D ( 'NONE', #57392, #13313, #52558 ) ;
#15107=CARTESIAN_POINT ( 'NONE',  ( 4.458734124999998549, -43.97916666530105800, -2.574251347313721627 ) ) ;
#15109=CARTESIAN_POINT ( 'NONE',  ( 3.152801135295367541, -148.3125000013655779, -3.152801135295367541 ) ) ;
#15112=ORIENTED_EDGE ( 'NONE', *, *, #11189, .T. ) ;
#15114=DIRECTION ( 'NONE',  ( 0.000000000000000000, 0.000000000000000000, 1.000000000000000000 ) ) ;
#15117=VERTEX_POINT ( 'NONE', #725 ) ;
#15122=CARTESIAN_POINT ( 'NONE',  ( -3.152548672688508926E-16, -4.562499998634401699, -5.148502694627439702 ) ) ;
#15123=CARTESIAN_POINT ( 'NONE',  ( 4.458734124999999437, -149.3750000013656063, -1.846868145590734978 ) ) ;
#15125=ORIENTED_EDGE ( 'NONE', *, *, #16199, .F. ) ;
#15127=CARTESIAN_POINT ( 'NONE',  ( -1.339745962155610925, -74.79465819873854571, 5.000000000000000000 ) ) ;
#15128=CYLINDRICAL_SURFACE ( 'NONE', #39185, 5.000000000000000000 ) ;
#15131=CARTESIAN_POINT ( 'NONE',  ( 1.975475456537005874E-15, -12.74999999999999822, 5.000000000000000000 ) ) ;
#15138=CARTESIAN_POINT ( 'NONE',  ( -4.458734124999999437, 19.60416666803225993, -2.574251347313719407 ) ) ;
#15141=CARTESIAN_POINT ( 'NONE',  ( 2.229367062500001939, -10.22916666530106866, 3.861377020970579999 ) ) ;
#15144=CARTESIAN_POINT ( 'NONE',  ( 3.152801135295366208, -167.5625000013656063, 3.152801135295367985 ) ) ;
#15151=CARTESIAN_POINT ( 'NONE',  ( -6.972266317189433020E-16, -75.12499999726880162, -5.000000000000000000 ) ) ;
#15153=CARTESIAN_POINT ( 'NONE',  ( 4.458734124999999437, -153.6250000013655779, -1.846868145590734978 ) ) ;
#15157=ORIENTED_EDGE ( 'NONE', *, *, #36172, .F. ) ;
#15161=CARTESIAN_POINT ( 'NONE',  ( 5.000000000000000888, -0.5833333333333350357, 2.886751345948126879 ) ) ;
#15162=CARTESIAN_POINT ( 'NONE',  ( -4.458734124999999437, -69.39583333196773651, -2.574251347313719407 ) ) ;
#15163=CARTESIAN_POINT ( 'NONE',  ( -1.339745962155610925, 20.20534180126147916, 5.000000000000000000 ) ) ;
#15164=CARTESIAN_POINT ( 'NONE',  ( -3.535250795749689387E-16, -2.124999997268814944, -5.773502691896257311 ) ) ;
#15165=CARTESIAN_POINT ( 'NONE',  ( 4.458734124999998549, -33.72916666530106511, -2.574251347313721627 ) ) ;
#15167=CARTESIAN_POINT ( 'NONE',  ( -5.000000000000000000, -78.00000000000000000, 0.000000000000000000 ) ) ;
#15168=CARTESIAN_POINT ( 'NONE',  ( -9.184850993605147944E-16, -157.2500000000000000, 5.000000000000000000 ) ) ;
#15169=ORIENTED_EDGE ( 'NONE', *, *, #18863, .T. ) ;
#15170=CARTESIAN_POINT ( 'NONE',  ( 2.500000000000002220, 5.333333333333332149, 4.330127018922192761 ) ) ;
#15171=CARTESIAN_POINT ( 'NONE',  ( -5.000000000000000000, -52.00000000000000711, 0.000000000000000000 ) ) ;
#15172=CARTESIAN_POINT ( 'NONE',  ( 1.975475456537005874E-15, -26.62499999726881228, 5.000000000000000000 ) ) ;
#15174=CARTESIAN_POINT ( 'NONE',  ( 4.458734125000001214, -71.89583333196773651, 2.574251347313718519 ) ) ;
#15175=CARTESIAN_POINT ( 'NONE',  ( -8.190561711645485556E-16, -144.9375000013656063, 4.458734124999999437 ) ) ;
#15176=CARTESIAN_POINT ( 'NONE',  ( 4.458734124999998549, -83.72916666530107932, -2.574251347313721627 ) ) ;
#15178=CARTESIAN_POINT ( 'NONE',  ( -4.458734124999999437, -28.56249999863440081, 0.000000000000000000 ) ) ;
#15179=( BOUNDED_CURVE ( )  B_SPLINE_CURVE ( 2, ( #50450, #39573, #58577, #24796, #30818 ),
 .UNSPECIFIED., .F., .F. ) 
 B_SPLINE_CURVE_WITH_KNOTS ( ( 3, 2, 3 ),
 ( 0.000000000000000000, 0.004166666666666670078, 0.008333333333333340157 ),
 .UNSPECIFIED. ) 
 CURVE ( )  GEOMETRIC_REPRESENTATION_ITEM ( )  RATIONAL_B_SPLINE_CURVE ( ( 1.000000000000000000, 0.9238795325112867385, 1.000000000000000000, 0.9238795325112866275, 1.000000000000000222 ) ) 
 REPRESENTATION_ITEM ( '' )  );
#15180=CARTESIAN_POINT ( 'NONE',  ( -3.535250795749689387E-16, -74.12499999726880162, -5.773502691896257311 ) ) ;
#15181=EDGE_LOOP ( 'NONE', ( #39686, #12419, #29485, #56570 ) ) ;
#15183=EDGE_LOOP ( 'NONE', ( #5144, #9199, #22867, #9142 ) ) ;
#15185=CARTESIAN_POINT ( 'NONE',  ( 2.500000000000002220, -21.66666666666666785, 4.330127018922192761 ) ) ;
#15187=CARTESIAN_POINT ( 'NONE',  ( -2.500000000000000444, 16.83333333333333215, -4.330127018922193649 ) ) ;
#15190=CARTESIAN_POINT ( 'NONE',  ( 2.229367062499998831, -57.89583333196773651, -3.861377020970580887 ) ) ;
#15194=CARTESIAN_POINT ( 'NONE',  ( 3.535533905932738197, -141.8750000000000000, -3.535533905932738197 ) ) ;
#15195=DIRECTION ( 'NONE',  ( 0.000000000000000000, 0.000000000000000000, 1.000000000000000000 ) ) ;
#15196=CARTESIAN_POINT ( 'NONE',  ( -4.458734124999998549, 15.77083333469892601, 2.574251347313722516 ) ) ;
#15198=CARTESIAN_POINT ( 'NONE',  ( 1.339745962155615144, -32.70534180126148271, 4.999999999999999112 ) ) ;
#15199=CARTESIAN_POINT ( 'NONE',  ( 4.458734124999999437, -162.3750000013656063, -1.846868145590734978 ) ) ;
#15202=CARTESIAN_POINT ( 'NONE',  ( -1.339745962155613812, -70.08034179853029855, -5.000000000000000000 ) ) ;
#15205=CARTESIAN_POINT ( 'NONE',  ( -9.184850993605147944E-16, -162.3750000027311842, 5.000000000000000000 ) ) ;
#15208=CARTESIAN_POINT ( 'NONE',  ( -5.000000000000000000, -29.08333333333332860, -2.886751345948128211 ) ) ;
#15214=CARTESIAN_POINT ( 'NONE',  ( 9.457646018065525792E-16, 4.687500001365595637, 5.148502694627439702 ) ) ;
#15215=CARTESIAN_POINT ( 'NONE',  ( -1.339745962155613812, -10.08034179853029144, -5.000000000000000000 ) ) ;
#15217=CARTESIAN_POINT ( 'NONE',  ( 5.000000000000000000, -149.1875000027312410, 2.071067811865478614 ) ) ;
#15225=CARTESIAN_POINT ( 'NONE',  ( -4.458734124999999437, -166.2500000013656063, -1.846868145590735644 ) ) ;
#15226=( BOUNDED_CURVE ( )  B_SPLINE_CURVE ( 2, ( #58916, #14845, #38355, #57981, #43172, #42861, #62506, #57676, #13906 ),
 .UNSPECIFIED., .F., .F. ) 
 B_SPLINE_CURVE_WITH_KNOTS ( ( 3, 2, 2, 2, 3 ),
 ( 0.4916666666666670849, 0.4958333333333337922, 0.5000000000000004441, 0.5041666666666670960, 0.5083333333333337478 ),
 .UNSPECIFIED. ) 
 CURVE ( )  GEOMETRIC_REPRESENTATION_ITEM ( )  RATIONAL_B_SPLINE_CURVE ( ( 0.9999999999999918954, 0.9238795325112948431, 1.000000000000000000, 0.9238795325112867385, 1.000000000000000000, 0.9238795325112867385, 1.000000000000000000, 0.9238795325112786339, 1.000000000000008216 ) ) 
 REPRESENTATION_ITEM ( '' )  );
#15227=CARTESIAN_POINT ( 'NONE',  ( -2.071067811865580754, -160.6875000000000284, -4.999999999999894307 ) ) ;
#15230=CARTESIAN_POINT ( 'NONE',  ( -8.190561711645485556E-16, -144.6875000013656063, 4.458734124999999437 ) ) ;
#15232=CARTESIAN_POINT ( 'NONE',  ( 4.458734125000001214, 27.85416666803225993, 2.574251347313718519 ) ) ;
#15234=CARTESIAN_POINT ( 'NONE',  ( -3.152548672688508926E-16, -59.81249999863440792, -5.148502694627439702 ) ) ;
#15237=CARTESIAN_POINT ( 'NONE',  ( 1.975475456537005874E-15, -90.62499999726880162, 5.000000000000000000 ) ) ;
#15238=CARTESIAN_POINT ( 'NONE',  ( 5.000000000000000000, 14.49999999999999822, -6.123233995736766282E-16 ) ) ;
#15240=AXIS2_PLACEMENT_3D ( 'NONE', #45868, #54889, #51020 ) ;
#15241=CARTESIAN_POINT ( 'NONE',  ( 2.229367062500001939, -50.97916666530107221, 3.861377020970579999 ) ) ;
#15242=CARTESIAN_POINT ( 'NONE',  ( 4.458734124999999437, -7.812499998634405252, -5.460374474430324690E-16 ) ) ;
#15246=DIRECTION ( 'NONE',  ( -0.000000000000000000, 1.000000000000000000, -0.000000000000000000 ) ) ;
#15251=CARTESIAN_POINT ( 'NONE',  ( 4.458734124999999437, -55.81249999863440081, -5.460374474430324690E-16 ) ) ;
#15252=CARTESIAN_POINT ( 'NONE',  ( -3.152801135295367096, -156.3125000013656063, -3.152801135295367541 ) ) ;
#15254=CARTESIAN_POINT ( 'NONE',  ( -5.000000000000000000, -55.95833333060215153, -2.886751345948128211 ) ) ;
#15255=ORIENTED_EDGE ( 'NONE', *, *, #41745, .T. ) ;
#15257=CARTESIAN_POINT ( 'NONE',  ( -3.152548672688508926E-16, 3.187500001365594748, -5.148502694627439702 ) ) ;
#15258=EDGE_CURVE ( 'NONE', #38746, #55791, #34555, .T. ) ;
#15262=CARTESIAN_POINT ( 'NONE',  ( 3.152801135295367541, -158.3125000013656063, -3.152801135295367541 ) ) ;
#15263=VERTEX_POINT ( 'NONE', #41846 ) ;
#15266=CARTESIAN_POINT ( 'NONE',  ( 2.071067811865561215, -161.3125000027312126, 4.999999999999913847 ) ) ;
#15267=CARTESIAN_POINT ( 'NONE',  ( -2.229367062500000163, -43.72916666530106511, -3.861377020970580443 ) ) ;
#15269=EDGE_CURVE ( 'NONE', #25522, #35059, #36652, .T. ) ;
#15272=CARTESIAN_POINT ( 'NONE',  ( 4.458734125000001214, 28.10416666803225993, 2.574251347313718519 ) ) ;
#15275=CARTESIAN_POINT ( 'NONE',  ( 6.123233995736766282E-16, -170.0000000000000000, -5.000000000000000000 ) ) ;
#15281=VECTOR ( 'NONE', #28084, 1000.000000000000000 ) ;
#15282=CARTESIAN_POINT ( 'NONE',  ( 1.339745962155615144, -33.70534180126148271, 4.999999999999999112 ) ) ;
#15288=CARTESIAN_POINT ( 'NONE',  ( -4.458734124999999437, -87.64583333196773651, -2.574251347313719407 ) ) ;
#15289=CARTESIAN_POINT ( 'NONE',  ( -5.000000000000000000, 11.04166666939785202, -2.886751345948128211 ) ) ;
#15291=ORIENTED_EDGE ( 'NONE', *, *, #24846, .T. ) ;
#15292=CARTESIAN_POINT ( 'NONE',  ( -2.071067811865415109, -163.4375000027311842, 5.000000000000062172 ) ) ;
#15294=CARTESIAN_POINT ( 'NONE',  ( -2.071067811865478170, -160.4375000027312126, 5.000000000000000000 ) ) ;
#15306=CARTESIAN_POINT ( 'NONE',  ( 9.457646018065525792E-16, -18.06249999863440792, 5.148502694627439702 ) ) ;
#15308=CARTESIAN_POINT ( 'NONE',  ( 5.000000000000000888, -154.9375000000000000, -2.071067811865475505 ) ) ;
#15310=CARTESIAN_POINT ( 'NONE',  ( -1.846868145590737420, -157.7500000013656063, 4.458734124999999437 ) ) ;
#15312=CARTESIAN_POINT ( 'NONE',  ( -2.229367062499996610, -47.39583333196774362, 3.861377020970582219 ) ) ;
#15313=CARTESIAN_POINT ( 'NONE',  ( 2.499999999999998668, -44.20833333060214443, -4.330127018922193649 ) ) ;
#15315=CARTESIAN_POINT ( 'NONE',  ( -5.000000000000000000, 30.00000000000000000, 0.000000000000000000 ) ) ;
#15319=CARTESIAN_POINT ( 'NONE',  ( 4.458734124999999437, 7.187500001365594748, -5.460374474430324690E-16 ) ) ;
#15320=CARTESIAN_POINT ( 'NONE',  ( 0.000000000000000000, -170.0000000000000000, 5.000000000000000000 ) ) ;
#15321=CARTESIAN_POINT ( 'NONE',  ( 2.500000000000002220, -17.66666666666666430, 4.330127018922192761 ) ) ;
#15322=CARTESIAN_POINT ( 'NONE',  ( 2.229367062500001939, 21.77083333469892779, 3.861377020970579999 ) ) ;
#15324=CARTESIAN_POINT ( 'NONE',  ( -5.000000000000000000, 10.04166666939785202, -2.886751345948128211 ) ) ;
#15326=CARTESIAN_POINT ( 'NONE',  ( -4.999999999999998224, 8.083333333333332149, 2.886751345948131764 ) ) ;
#15327=VERTEX_POINT ( 'NONE', #17731 ) ;
#15330=CARTESIAN_POINT ( 'NONE',  ( -4.458734124999999437, -38.39583333196773651, -2.574251347313719407 ) ) ;
#15331=VECTOR ( 'NONE', #47247, 1000.000000000000000 ) ;
#15332=CARTESIAN_POINT ( 'NONE',  ( -5.000000000000000000, -40.87499999726880162, 0.000000000000000000 ) ) ;
#15335=CARTESIAN_POINT ( 'NONE',  ( 2.229367062499998831, -11.64583333196774007, -3.861377020970580887 ) ) ;
#15336=EDGE_CURVE ( 'NONE', #54054, #31959, #56769, .T. ) ;
#15337=CARTESIAN_POINT ( 'NONE',  ( 9.457646018065525792E-16, -19.31249999863440792, 5.148502694627439702 ) ) ;
#15338=ORIENTED_EDGE ( 'NONE', *, *, #20124, .F. ) ;
#15339=CARTESIAN_POINT ( 'NONE',  ( 5.000000000000000000, -81.50000000000000000, -6.123233995736766282E-16 ) ) ;
#15340=CARTESIAN_POINT ( 'NONE',  ( -4.458734124999999437, -166.9375000013655779, -5.460374474430324690E-16 ) ) ;
#15342=CARTESIAN_POINT ( 'NONE',  ( 5.000000000000000888, -85.45833333060213022, 2.886751345948126879 ) ) ;
#15343=CARTESIAN_POINT ( 'NONE',  ( -4.999999999999998224, -31.91666666666666430, 2.886751345948131764 ) ) ;
#15344=ORIENTED_EDGE ( 'NONE', *, *, #23548, .F. ) ;
#15346=CARTESIAN_POINT ( 'NONE',  ( -2.229367062500000163, -29.72916666530107221, -3.861377020970580443 ) ) ;
#15347=CARTESIAN_POINT ( 'NONE',  ( -5.000000000000000000, -50.00000000000000000, 0.000000000000000000 ) ) ;
#15348=VERTEX_POINT ( 'NONE', #32198 ) ;
#15349=PRODUCT_CONTEXT ( 'NONE', #4731, 'mechanical' ) ;
#15350=CARTESIAN_POINT ( 'NONE',  ( -1.846868145590737420, -163.0000000013655779, 4.458734124999999437 ) ) ;
#15355=CARTESIAN_POINT ( 'NONE',  ( -2.229367062499996610, -73.39583333196773651, 3.861377020970582219 ) ) ;
#15358=CARTESIAN_POINT ( 'NONE',  ( 3.152801135295366208, -147.8125000013655779, 3.152801135295367985 ) ) ;
#15359=CARTESIAN_POINT ( 'NONE',  ( -1.339745962155617365, 23.20534180126148271, 4.999999999999998224 ) ) ;
#15364=( BOUNDED_CURVE ( )  B_SPLINE_CURVE ( 2, ( #12187, #17330, #46603, #36952, #55634, #55944, #31801, #51434, #56579 ),
 .UNSPECIFIED., .F., .F. ) 
 B_SPLINE_CURVE_WITH_KNOTS ( ( 3, 2, 2, 2, 3 ),
 ( 0.6895833333333333259, 0.6902777777777777679, 0.6916666666666666519, 0.6930555555555555358, 0.6937499999999999778 ),
 .UNSPECIFIED. ) 
 CURVE ( )  GEOMETRIC_REPRESENTATION_ITEM ( )  RATIONAL_B_SPLINE_CURVE ( ( 0.9330127018922194093, 0.9330127018922194093, 1.000000000000000000, 0.8660254037844387076, 1.000000000000000000, 0.8660254037844387076, 1.000000000000000000, 0.9330127018922194093, 0.9330127018922194093 ) ) 
 REPRESENTATION_ITEM ( '' )  );
#15366=CARTESIAN_POINT ( 'NONE',  ( 1.846868145590735200, -140.5000000013656347, -4.458734125000000326 ) ) ;
#15369=CARTESIAN_POINT ( 'NONE',  ( -1.339745962155610925, -52.79465819873851729, 5.000000000000000000 ) ) ;
#15371=CARTESIAN_POINT ( 'NONE',  ( 4.458734125000001214, -76.14583333196773651, 2.574251347313718519 ) ) ;
#15372=FACE_OUTER_BOUND ( 'NONE', #58463, .T. ) ;
#15373=CARTESIAN_POINT ( 'NONE',  ( 5.000000000000000888, -54.45833333060214443, 2.886751345948126879 ) ) ;
#15382=AXIS2_PLACEMENT_3D ( 'NONE', #60119, #40162, #54963 ) ;
#15383=CARTESIAN_POINT ( 'NONE',  ( -2.229367062500000163, 19.27083333469892779, -3.861377020970580443 ) ) ;
#15384=CYLINDRICAL_SURFACE ( 'NONE', #3779, 5.000000000000000000 ) ;
#15386=( BOUNDED_CURVE ( )  B_SPLINE_CURVE ( 2, ( #24967, #29135, #28831, #20142, #38478, #58107, #14665, #39739, #43614 ),
 .UNSPECIFIED., .F., .F. ) 
 B_SPLINE_CURVE_WITH_KNOTS ( ( 3, 2, 2, 2, 3 ),
 ( 0.3479166666666666519, 0.3486111111111110938, 0.3499999999999999778, 0.3513888888888888618, 0.3520833333333333592 ),
 .UNSPECIFIED. ) 
 CURVE ( )  GEOMETRIC_REPRESENTATION_ITEM ( )  RATIONAL_B_SPLINE_CURVE ( ( 0.9330127018922194093, 0.9330127018922194093, 1.000000000000000000, 0.8660254037844387076, 1.000000000000000000, 0.8660254037844387076, 1.000000000000000000, 0.9330127018922167448, 0.9330127018922194093 ) ) 
 REPRESENTATION_ITEM ( '' )  );
#15391=CARTESIAN_POINT ( 'NONE',  ( -3.152548672688508926E-16, -5.562499998634400811, -5.148502694627439702 ) ) ;
#15393=CARTESIAN_POINT ( 'NONE',  ( 4.458734124999999437, -28.06249999863440081, -5.460374474430324690E-16 ) ) ;
#15397=CARTESIAN_POINT ( 'NONE',  ( 2.229367062500001939, 27.02083333469892423, 3.861377020970579999 ) ) ;
#15398=ADVANCED_FACE ( 'NONE', ( #27066 ), #46682, .T. ) ;
#15399=ADVANCED_FACE ( 'NONE', ( #42480 ), #18037, .T. ) ;
#15400=CARTESIAN_POINT ( 'NONE',  ( 5.000000000000000000, 26.70833333606451632, -2.886751345948130876 ) ) ;
#15401=FACE_OUTER_BOUND ( 'NONE', #14836, .T. ) ;
#15402=CARTESIAN_POINT ( 'NONE',  ( -4.458734124999999437, -77.64583333196773651, -2.574251347313719407 ) ) ;
#15405=CARTESIAN_POINT ( 'NONE',  ( -9.184850993605147944E-16, -152.2500000000000000, 5.000000000000000000 ) ) ;
#15406=CARTESIAN_POINT ( 'NONE',  ( 5.000000000000000000, 25.70833333606452342, -2.886751345948129988 ) ) ;
#15408=LINE ( 'NONE', #48849, #35592 ) ;
#15410=LINE ( 'NONE', #29863, #36046 ) ;
#15411=CARTESIAN_POINT ( 'NONE',  ( -2.499999999999996447, -16.83333333333333215, 4.330127018922195425 ) ) ;
#15412=CARTESIAN_POINT ( 'NONE',  ( -4.458734124999999437, -21.31249999863440436, 0.000000000000000000 ) ) ;
#15414=CARTESIAN_POINT ( 'NONE',  ( -4.458734124999999437, -80.31249999863440792, 0.000000000000000000 ) ) ;
#15415=EDGE_CURVE ( 'NONE', #37124, #32095, #25560, .T. ) ;
#15416=CARTESIAN_POINT ( 'NONE',  ( -3.535250795749689387E-16, -21.12499999726881228, -5.773502691896257311 ) ) ;
#15417=CARTESIAN_POINT ( 'NONE',  ( -4.458734124999999437, -47.39583333196774362, -2.574251347313719407 ) ) ;
#15418=EDGE_LOOP ( 'NONE', ( #8211, #35666, #9468, #29698 ) ) ;
#15420=CARTESIAN_POINT ( 'NONE',  ( 2.499999999999998668, -74.20833333060214443, -4.330127018922193649 ) ) ;
#15421=CARTESIAN_POINT ( 'NONE',  ( -2.229367062499996610, 3.604166668032260379, 3.861377020970582219 ) ) ;
#15422=VERTEX_POINT ( 'NONE', #9021 ) ;
#15424=CARTESIAN_POINT ( 'NONE',  ( 5.000000000000000000, -65.50000000000000000, -6.123233995736766282E-16 ) ) ;
#15426=CARTESIAN_POINT ( 'NONE',  ( -1.846868145590734756, -152.3750000013655779, -4.458734125000000326 ) ) ;
#15429=CARTESIAN_POINT ( 'NONE',  ( 3.535533905932736864, -164.1250000000000284, 3.535533905932738641 ) ) ;
#15431=EDGE_CURVE ( 'NONE', #52288, #54333, #6226, .T. ) ;
#15433=VECTOR ( 'NONE', #45858, 1000.000000000000000 ) ;
#15435=CARTESIAN_POINT ( 'NONE',  ( -2.229367062499996610, -10.39583333196773829, 3.861377020970582219 ) ) ;
#15436=CARTESIAN_POINT ( 'NONE',  ( -2.229367062499996610, -47.39583333196774362, 3.861377020970582219 ) ) ;
#15438=CARTESIAN_POINT ( 'NONE',  ( 4.458734124999999437, -145.4375000013656063, 0.000000000000000000 ) ) ;
#15446=EDGE_LOOP ( 'NONE', ( #28783, #3998, #24341, #561 ) ) ;
#15448=CARTESIAN_POINT ( 'NONE',  ( 1.339745962155565406, -19.70534180126148271, 5.000000000000028422 ) ) ;
#15450=CARTESIAN_POINT ( 'NONE',  ( -6.972266317189433020E-16, 11.87500000273118594, -5.000000000000000000 ) ) ;
#15451=CARTESIAN_POINT ( 'NONE',  ( -2.229367062500000163, -5.479166665301072214, -3.861377020970580443 ) ) ;
#15453=CARTESIAN_POINT ( 'NONE',  ( -1.846868145590734756, -148.1250000013655779, -4.458734124999999437 ) ) ;
#15457=CARTESIAN_POINT ( 'NONE',  ( -5.000000000000000000, -26.95833333060214798, -2.886751345948128211 ) ) ;
#15459=CARTESIAN_POINT ( 'NONE',  ( 5.000000000000000888, -25.45833333060214443, 2.886751345948126879 ) ) ;
#15460=CARTESIAN_POINT ( 'NONE',  ( 1.975475456537005874E-15, -88.62499999726880162, 5.000000000000000000 ) ) ;
#15466=LINE ( 'NONE', #44396, #23342 ) ;
#15467=CARTESIAN_POINT ( 'NONE',  ( 4.458734125000000326, 13.10416666803226171, 2.574251347313718519 ) ) ;
#15471=CARTESIAN_POINT ( 'NONE',  ( -2.229367062499996610, -12.39583333196774007, 3.861377020970582219 ) ) ;
#15472=( BOUNDED_CURVE ( )  B_SPLINE_CURVE ( 2, ( #24973, #34607, #4398, #24651, #537, #24019, #33669, #44257, #29778 ),
 .UNSPECIFIED., .F., .F. ) 
 B_SPLINE_CURVE_WITH_KNOTS ( ( 3, 2, 2, 2, 3 ),
 ( 0.1479166666666666685, 0.1486111111111111105, 0.1499999999999999944, 0.1513888888888888784, 0.1520833333333333481 ),
 .UNSPECIFIED. ) 
 CURVE ( )  GEOMETRIC_REPRESENTATION_ITEM ( )  RATIONAL_B_SPLINE_CURVE ( ( 0.9330127018922194093, 0.9330127018922194093, 1.000000000000000000, 0.8660254037844387076, 1.000000000000000000, 0.8660254037844387076, 1.000000000000000000, 0.9330127018922180770, 0.9330127018922194093 ) ) 
 REPRESENTATION_ITEM ( '' )  );
#15474=CARTESIAN_POINT ( 'NONE',  ( -4.458734124999999437, -161.9375000013655779, -5.460374474430324690E-16 ) ) ;
#15475=CARTESIAN_POINT ( 'NONE',  ( 2.499999999999998668, -63.20833333060215153, -4.330127018922193649 ) ) ;
#15483=CARTESIAN_POINT ( 'NONE',  ( -1.846868145590734756, -154.3750000013655779, -4.458734124999999437 ) ) ;
#15485=CARTESIAN_POINT ( 'NONE',  ( -2.499999999999996447, -13.83333333333333570, 4.330127018922195425 ) ) ;
#15487=ORIENTED_EDGE ( 'NONE', *, *, #48630, .F. ) ;
#15491=CARTESIAN_POINT ( 'NONE',  ( -4.999999999999999112, -4.916666666666666075, 2.886751345948131764 ) ) ;
#15492=CARTESIAN_POINT ( 'NONE',  ( 9.457646018065525792E-16, -68.06249999863440792, 5.148502694627439702 ) ) ;
#15493=DIRECTION ( 'NONE',  ( -0.000000000000000000, 1.000000000000000000, -0.000000000000000000 ) ) ;
#15494=CARTESIAN_POINT ( 'NONE',  ( 2.500000000000002220, -8.541666663935483683, 4.330127018922192761 ) ) ;
#15495=CARTESIAN_POINT ( 'NONE',  ( 2.229367062499998831, -32.64583333196773651, -3.861377020970580887 ) ) ;
#15496=ORIENTED_EDGE ( 'NONE', *, *, #14147, .T. ) ;
#15499=EDGE_LOOP ( 'NONE', ( #60362, #58684, #13749, #40896 ) ) ;
#15501=CARTESIAN_POINT ( 'NONE',  ( 5.000000000000000888, -50.58333333333332860, 2.886751345948126879 ) ) ;
#15503=CARTESIAN_POINT ( 'NONE',  ( 1.339745962155615144, -46.58034179853028434, 4.999999999999999112 ) ) ;
#15505=CARTESIAN_POINT ( 'NONE',  ( -5.000000000000000000, -41.95833333060214443, -2.886751345948128211 ) ) ;
#15506=CARTESIAN_POINT ( 'NONE',  ( -4.458734124999999437, -77.39583333196772230, -2.574251347313719407 ) ) ;
#15507=CARTESIAN_POINT ( 'NONE',  ( 4.458734124999999437, -145.7500000013655779, 1.846868145590737864 ) ) ;
#15508=CARTESIAN_POINT ( 'NONE',  ( 9.457646018065525792E-16, -82.06249999863442213, 5.148502694627439702 ) ) ;
#15510=CARTESIAN_POINT ( 'NONE',  ( -4.458734124999999437, -30.64583333196774007, -2.574251347313719407 ) ) ;
#15511=CARTESIAN_POINT ( 'NONE',  ( -5.000000000000000000, -73.87499999726880162, 0.000000000000000000 ) ) ;
#15514=CARTESIAN_POINT ( 'NONE',  ( 2.500000000000002220, -51.66666666666666430, 4.330127018922192761 ) ) ;
#15517=CARTESIAN_POINT ( 'NONE',  ( 1.975475456537005874E-15, -21.75000000000000000, 5.000000000000000000 ) ) ;
#15522=CARTESIAN_POINT ( 'NONE',  ( 4.458734125000001214, -60.14583333196774362, 2.574251347313718519 ) ) ;
#15524=ORIENTED_EDGE ( 'NONE', *, *, #38979, .F. ) ;
#15525=DIRECTION ( 'NONE',  ( -0.000000000000000000, 1.000000000000000000, -0.000000000000000000 ) ) ;
#15526=CARTESIAN_POINT ( 'NONE',  ( 4.458734125000001214, 13.10416666803226171, 2.574251347313718519 ) ) ;
#15528=CARTESIAN_POINT ( 'NONE',  ( 1.339745962155612702, -27.16965819600733312, -5.000000000000000000 ) ) ;
#15529=CARTESIAN_POINT ( 'NONE',  ( -4.458734124999999437, -160.9375000013655779, -5.460374474430324690E-16 ) ) ;
#15530=FACE_OUTER_BOUND ( 'NONE', #23752, .T. ) ;
#15531=VERTEX_POINT ( 'NONE', #50156 ) ;
#15533=DIRECTION ( 'NONE',  ( -0.000000000000000000, 1.000000000000000000, -0.000000000000000000 ) ) ;
#15540=CARTESIAN_POINT ( 'NONE',  ( -2.499999999999996447, -72.70833333060214443, 4.330127018922195425 ) ) ;
#15545=CARTESIAN_POINT ( 'NONE',  ( -4.458734124999999437, 4.437500001365595637, 0.000000000000000000 ) ) ;
#15546=CARTESIAN_POINT ( 'NONE',  ( -2.071067811865548780, -161.8125000027312126, -4.999999999999926281 ) ) ;
#15548=CARTESIAN_POINT ( 'NONE',  ( 3.061616997868383141E-16, -143.8750000027312126, -5.000000000000000000 ) ) ;
#15557=CARTESIAN_POINT ( 'NONE',  ( -4.458734125000000326, -165.1250000013656347, 1.846868145590734089 ) ) ;
#15558=CARTESIAN_POINT ( 'NONE',  ( -2.500000000000000444, -33.16666666666666430, -4.330127018922193649 ) ) ;
#15561=CARTESIAN_POINT ( 'NONE',  ( -4.458734124999999437, -143.9375000013656063, -5.460374474430324690E-16 ) ) ;
#15563=CARTESIAN_POINT ( 'NONE',  ( -4.458734124999999437, 25.35416666803225993, -2.574251347313719407 ) ) ;
#15565=CARTESIAN_POINT ( 'NONE',  ( 2.229367062499998831, -59.89583333196774362, -3.861377020970580887 ) ) ;
#15568=CARTESIAN_POINT ( 'NONE',  ( -2.500000000000000444, 13.83333333333333215, -4.330127018922193649 ) ) ;
#15570=CARTESIAN_POINT ( 'NONE',  ( -4.458734124999999437, -50.31249999863440792, 0.000000000000000000 ) ) ;
#15571=CARTESIAN_POINT ( 'NONE',  ( 4.458734124999999437, -9.812499998634406140, -5.460374474430324690E-16 ) ) ;
#15572=( BOUNDED_CURVE ( )  B_SPLINE_CURVE ( 2, ( #25911, #45529, #24961, #1490, #44566, #524, #39733, #34929, #15632 ),
 .UNSPECIFIED., .F., .F. ) 
 B_SPLINE_CURVE_WITH_KNOTS ( ( 3, 2, 2, 2, 3 ),
 ( 0.9062500000000000000, 0.9069444444444444420, 0.9083333333333333259, 0.9097222222222222099, 0.9104166666666666519 ),
 .UNSPECIFIED. ) 
 CURVE ( )  GEOMETRIC_REPRESENTATION_ITEM ( )  RATIONAL_B_SPLINE_CURVE ( ( 0.9330127018922194093, 0.9330127018922194093, 1.000000000000000000, 0.8660254037844387076, 1.000000000000000000, 0.8660254037844387076, 1.000000000000000000, 0.9330127018922194093, 0.9330127018922194093 ) ) 
 REPRESENTATION_ITEM ( '' )  );
#15573=CARTESIAN_POINT ( 'NONE',  ( -5.000000000000000000, -23.08333333333333215, -2.886751345948128211 ) ) ;
#15574=CARTESIAN_POINT ( 'NONE',  ( -2.500000000000000444, -64.04166666393547303, -4.330127018922193649 ) ) ;
#15578=CARTESIAN_POINT ( 'NONE',  ( -1.339745962155623360, 15.20534180126147739, 4.999999999999991118 ) ) ;
#15581=CARTESIAN_POINT ( 'NONE',  ( -4.458734124999999437, -58.31249999863440081, 0.000000000000000000 ) ) ;
#15582=CARTESIAN_POINT ( 'NONE',  ( 4.458734124999999437, -156.7500000013656063, 1.846868145590737864 ) ) ;
#15583=CARTESIAN_POINT ( 'NONE',  ( 5.000000000000000000, -56.37499999726880162, -6.123233995736766282E-16 ) ) ;
#15586=CARTESIAN_POINT ( 'NONE',  ( -4.458734124999999437, -0.6458333319677399542, -2.574251347313719407 ) ) ;
#15587=ORIENTED_EDGE ( 'NONE', *, *, #32677, .F. ) ;
#15590=CARTESIAN_POINT ( 'NONE',  ( -4.458734125000001214, -155.8750000013655779, 1.846868145590734089 ) ) ;
#15592=CARTESIAN_POINT ( 'NONE',  ( 5.000000000000000000, 25.50000000000000000, -6.123233995736766282E-16 ) ) ;
#15594=CARTESIAN_POINT ( 'NONE',  ( 3.061616997868383141E-16, -160.8750000027311842, -5.000000000000000000 ) ) ;
#15595=CARTESIAN_POINT ( 'NONE',  ( -4.458734124999999437, -44.56249999863440081, 0.000000000000000000 ) ) ;
#15596=ORIENTED_EDGE ( 'NONE', *, *, #11849, .F. ) ;
#15598=CARTESIAN_POINT ( 'NONE',  ( -3.152548672688508926E-16, 28.43750000136559208, -5.148502694627439702 ) ) ;
#15600=LINE ( 'NONE', #35218, #62412 ) ;
#15610=CARTESIAN_POINT ( 'NONE',  ( -5.000000000000000000, 4.916666666666666075, -2.886751345948128211 ) ) ;
#15612=CARTESIAN_POINT ( 'NONE',  ( -4.458734124999999437, -88.64583333196773651, -2.574251347313719407 ) ) ;
#15615=( BOUNDED_CURVE ( )  B_SPLINE_CURVE ( 2, ( #37248, #12794, #7984, #35225, #50654, #11089, #16561, #1790, #11408 ),
 .UNSPECIFIED., .F., .F. ) 
 B_SPLINE_CURVE_WITH_KNOTS ( ( 3, 2, 2, 2, 3 ),
 ( 0.2562499999999999778, 0.2569444444444444198, 0.2583333333333333592, 0.2597222222222222432, 0.2604166666666666852 ),
 .UNSPECIFIED. ) 
 CURVE ( )  GEOMETRIC_REPRESENTATION_ITEM ( )  RATIONAL_B_SPLINE_CURVE ( ( 0.9330127018922194093, 0.9330127018922194093, 1.000000000000000000, 0.8660254037844387076, 1.000000000000000000, 0.8660254037844387076, 1.000000000000000000, 0.9330127018922194093, 0.9330127018922194093 ) ) 
 REPRESENTATION_ITEM ( '' )  );
#15616=ORIENTED_EDGE ( 'NONE', *, *, #20028, .T. ) ;
#15619=CARTESIAN_POINT ( 'NONE',  ( -3.535533905932737309, -160.7500000027312126, -3.535533905932738197 ) ) ;
#15622=CARTESIAN_POINT ( 'NONE',  ( -2.500000000000000444, 21.83333333333333215, -4.330127018922193649 ) ) ;
#15631=CARTESIAN_POINT ( 'NONE',  ( -4.458734124999999437, -18.39583333196774007, -2.574251347313719407 ) ) ;
#15632=CARTESIAN_POINT ( 'NONE',  ( -6.972266317189433020E-16, -80.12499999726881583, -5.000000000000000000 ) ) ;
#15633=CARTESIAN_POINT ( 'NONE',  ( -2.071067811865475061, -155.6875000000000284, -5.000000000000000888 ) ) ;
#15635=CARTESIAN_POINT ( 'NONE',  ( 4.458734124999999437, -157.4375000013655779, 0.000000000000000000 ) ) ;
#15636=VERTEX_POINT ( 'NONE', #55322 ) ;
#15637=CARTESIAN_POINT ( 'NONE',  ( -4.458734124999997661, -47.47916666530106511, 2.574251347313722516 ) ) ;
#15638=FACE_OUTER_BOUND ( 'NONE', #48883, .T. ) ;
#15640=CARTESIAN_POINT ( 'NONE',  ( -4.999999999999999112, 29.08333333333333215, 2.886751345948131764 ) ) ;
#15641=CARTESIAN_POINT ( 'NONE',  ( 2.229367062499998831, 4.354166668032260823, -3.861377020970580887 ) ) ;
#15645=CARTESIAN_POINT ( 'NONE',  ( -4.458734124999999437, 22.43750000136559564, 0.000000000000000000 ) ) ;
#15647=CARTESIAN_POINT ( 'NONE',  ( -5.000000000000000000, 6.125000002731185056, 0.000000000000000000 ) ) ;
#15651=CARTESIAN_POINT ( 'NONE',  ( -3.152548672688508926E-16, -36.56249999863441502, -5.148502694627439702 ) ) ;
#15652=CARTESIAN_POINT ( 'NONE',  ( -3.535250795749689387E-16, -40.12499999726880162, -5.773502691896257311 ) ) ;
#15653=EDGE_LOOP ( 'NONE', ( #608, #39296, #54029, #31022 ) ) ;
#15654=CARTESIAN_POINT ( 'NONE',  ( -2.229367062499996610, -12.14583333196774007, 3.861377020970582219 ) ) ;
#15655=EDGE_LOOP ( 'NONE', ( #44077, #34658, #57620, #14224 ) ) ;
#15656=CARTESIAN_POINT ( 'NONE',  ( 5.000000000000000000, -81.41666666666667140, -2.886751345948129988 ) ) ;
#15657=CYLINDRICAL_SURFACE ( 'NONE', #55619, 5.000000000000000000 ) ;
#15659=( BOUNDED_CURVE ( )  B_SPLINE_CURVE ( 2, ( #59845, #55338, #40209, #667, #11254, #15457, #25741, #55972, #50821 ),
 .UNSPECIFIED., .F., .F. ) 
 B_SPLINE_CURVE_WITH_KNOTS ( ( 3, 2, 2, 2, 3 ),
 ( 0.4645833333333333481, 0.4652777777777777901, 0.4666666666666666741, 0.4680555555555555580, 0.4687500000000000000 ),
 .UNSPECIFIED. ) 
 CURVE ( )  GEOMETRIC_REPRESENTATION_ITEM ( )  RATIONAL_B_SPLINE_CURVE ( ( 0.9330127018922194093, 0.9330127018922194093, 1.000000000000000000, 0.8660254037844387076, 1.000000000000000000, 0.8660254037844387076, 1.000000000000000000, 0.9330127018922194093, 0.9330127018922194093 ) ) 
 REPRESENTATION_ITEM ( '' )  );
#15660=CARTESIAN_POINT ( 'NONE',  ( -5.000000000000000000, -85.95833333060213022, -2.886751345948128211 ) ) ;
#15664=CARTESIAN_POINT ( 'NONE',  ( 2.229367062499998831, -24.89583333196773651, -3.861377020970580887 ) ) ;
#15666=VERTEX_POINT ( 'NONE', #59177 ) ;
#15668=CARTESIAN_POINT ( 'NONE',  ( -8.190561711645485556E-16, -162.9375000013655779, 4.458734124999999437 ) ) ;
#15670=CARTESIAN_POINT ( 'NONE',  ( 2.071067811865306751, -155.8125000000000284, -5.000000000000171418 ) ) ;
#15671=ORIENTED_EDGE ( 'NONE', *, *, #40871, .F. ) ;
#15673=CARTESIAN_POINT ( 'NONE',  ( 4.458734124999999437, -75.06249999863440792, -5.460374474430324690E-16 ) ) ;
#15676=CARTESIAN_POINT ( 'NONE',  ( 1.846868145590736310, -143.8750000013656063, 4.458734124999997661 ) ) ;
#15680=EDGE_CURVE ( 'NONE', #35595, #5760, #14839, .T. ) ;
#15683=CARTESIAN_POINT ( 'NONE',  ( -3.535533905932737309, -167.6250000000000284, -3.535533905932738197 ) ) ;
#15688=CARTESIAN_POINT ( 'NONE',  ( -4.458734124999999437, -76.64583333196775072, -2.574251347313719407 ) ) ;
#15689=CARTESIAN_POINT ( 'NONE',  ( -5.000000000000000888, -166.4375000000000853, 2.071067811865474617 ) ) ;
#15691=DIRECTION ( 'NONE',  ( -0.000000000000000000, 1.000000000000000000, -0.000000000000000000 ) ) ;
#15693=ORIENTED_EDGE ( 'NONE', *, *, #25113, .F. ) ;
#15694=CARTESIAN_POINT ( 'NONE',  ( 6.123233995736766282E-16, -170.0000000000000000, -5.000000000000000000 ) ) ;
#15695=CARTESIAN_POINT ( 'NONE',  ( 1.975475456537005874E-15, 12.24999999999999822, 5.000000000000000000 ) ) ;
#15701=CARTESIAN_POINT ( 'NONE',  ( 4.458734124999999437, 19.93750000136559208, -5.460374474430324690E-16 ) ) ;
#15709=CARTESIAN_POINT ( 'NONE',  ( 9.457646018065525792E-16, -87.06249999863440792, 5.148502694627439702 ) ) ;
#15710=CARTESIAN_POINT ( 'NONE',  ( 4.458734124999998549, -4.729166665301071326, -2.574251347313721627 ) ) ;
#15711=CARTESIAN_POINT ( 'NONE',  ( -4.458734124999999437, -27.64583333196774007, -2.574251347313719407 ) ) ;
#15715=CARTESIAN_POINT ( 'NONE',  ( -4.458734124999998549, 24.77083333469893134, 2.574251347313722516 ) ) ;
#15717=CARTESIAN_POINT ( 'NONE',  ( -2.071067811865391128, -145.8125000027312410, -5.000000000000086153 ) ) ;
#15718=CARTESIAN_POINT ( 'NONE',  ( 4.458734124999999437, -80.06249999863440792, -5.460374474430324690E-16 ) ) ;
#15721=CARTESIAN_POINT ( 'NONE',  ( -5.000000000000000000, 26.12500000273118417, 0.000000000000000000 ) ) ;
#15722=ORIENTED_EDGE ( 'NONE', *, *, #20853, .T. ) ;
#15724=DIRECTION ( 'NONE',  ( -0.000000000000000000, 1.000000000000000000, -0.000000000000000000 ) ) ;
#15725=LINE ( 'NONE', #26648, #58493 ) ;
#15726=CARTESIAN_POINT ( 'NONE',  ( 5.000000000000000888, -19.58333333333333215, 2.886751345948126879 ) ) ;
#15727=CARTESIAN_POINT ( 'NONE',  ( 4.458734124999999437, -19.81249999863440081, -5.460374474430324690E-16 ) ) ;
#15728=CARTESIAN_POINT ( 'NONE',  ( -4.458734124999999437, -83.39583333196773651, -2.574251347313719407 ) ) ;
#15729=CARTESIAN_POINT ( 'NONE',  ( 5.000000000000000000, -23.29166666393548368, -2.886751345948129988 ) ) ;
#15731=CARTESIAN_POINT ( 'NONE',  ( -4.458734124999998549, -52.22916666530106511, 2.574251347313722516 ) ) ;
#15733=CARTESIAN_POINT ( 'NONE',  ( 2.500000000000002220, -65.66666666666667140, 4.330127018922192761 ) ) ;
#15735=CARTESIAN_POINT ( 'NONE',  ( 2.229367062499998831, -2.895833331967738289, -3.861377020970580887 ) ) ;
#15736=VERTEX_POINT ( 'NONE', #54670 ) ;
#15738=CARTESIAN_POINT ( 'NONE',  ( -5.000000000000000000, -66.08333333333332860, -2.886751345948128211 ) ) ;
#15739=CARTESIAN_POINT ( 'NONE',  ( -8.190561711645485556E-16, -151.9375000013655779, 4.458734124999999437 ) ) ;
#15742=CARTESIAN_POINT ( 'NONE',  ( 2.071067811865476394, -157.1875000000000284, 5.000000000000000000 ) ) ;
#15743=CYLINDRICAL_SURFACE ( 'NONE', #29228, 5.000000000000000000 ) ;
#15745=CARTESIAN_POINT ( 'NONE',  ( 2.229367062499998831, -9.895833331967738289, -3.861377020970580887 ) ) ;
#15746=CARTESIAN_POINT ( 'NONE',  ( 2.229367062499998831, -44.89583333196774362, -3.861377020970580887 ) ) ;
#15747=( BOUNDED_CURVE ( )  B_SPLINE_CURVE ( 2, ( #12898, #56670, #60856, #61807, #27375, #21928, #12277, #31248, #17428 ),
 .UNSPECIFIED., .F., .F. ) 
 B_SPLINE_CURVE_WITH_KNOTS ( ( 3, 2, 2, 2, 3 ),
 ( 0.5916666666666671182, 0.5958333333333335480, 0.6000000000000000888, 0.6041666666666665186, 0.6083333333333329485 ),
 .UNSPECIFIED. ) 
 CURVE ( )  GEOMETRIC_REPRESENTATION_ITEM ( )  RATIONAL_B_SPLINE_CURVE ( ( 0.9999999999999918954, 0.9238795325112948431, 1.000000000000000000, 0.9238795325112867385, 1.000000000000000000, 0.9238795325112867385, 1.000000000000000000, 0.9238795325112928447, 0.9999999999999938938 ) ) 
 REPRESENTATION_ITEM ( '' )  );
#15749=CARTESIAN_POINT ( 'NONE',  ( -4.458734125000001214, -145.8750000013656063, 1.846868145590734089 ) ) ;
#15752=ORIENTED_EDGE ( 'NONE', *, *, #52232, .T. ) ;
#15754=CARTESIAN_POINT ( 'NONE',  ( -2.229367062500000163, 26.27083333469892779, -3.861377020970580443 ) ) ;
#15760=EDGE_CURVE ( 'NONE', #40578, #10208, #20586, .T. ) ;
#15764=CARTESIAN_POINT ( 'NONE',  ( 1.339745962155612702, 11.83034180399266688, -5.000000000000000000 ) ) ;
#15765=CARTESIAN_POINT ( 'NONE',  ( 2.229367062500001939, -9.979166665301068662, 3.861377020970579999 ) ) ;
#15767=CARTESIAN_POINT ( 'NONE',  ( 1.846868145590735200, -149.2500000013656063, -4.458734124999999437 ) ) ;
#15770=DIRECTION ( 'NONE',  ( -0.000000000000000000, 1.000000000000000000, -0.000000000000000000 ) ) ;
#15774=CARTESIAN_POINT ( 'NONE',  ( 2.499999999999998668, -88.20833333060214443, -4.330127018922193649 ) ) ;
#15777=CARTESIAN_POINT ( 'NONE',  ( 5.000000000000000888, -74.58333333333332860, 2.886751345948126879 ) ) ;
#15782=CARTESIAN_POINT ( 'NONE',  ( -4.458734124999999437, 13.60416666803226171, -2.574251347313719407 ) ) ;
#15785=CARTESIAN_POINT ( 'NONE',  ( -2.229367062500000163, -15.72916666530107399, -3.861377020970580443 ) ) ;
#15787=CARTESIAN_POINT ( 'NONE',  ( 3.152801135295366208, -162.5625000013656063, 3.152801135295367985 ) ) ;
#15788=CARTESIAN_POINT ( 'NONE',  ( -5.000000000000000000, -40.87499999726880162, 0.000000000000000000 ) ) ;
#15794=CARTESIAN_POINT ( 'NONE',  ( 0.000000000000000000, -170.0000000000000000, 5.000000000000000000 ) ) ;
#15796=CARTESIAN_POINT ( 'NONE',  ( 1.846868145590736310, -150.8750000013655779, 4.458734124999997661 ) ) ;
#15798=CARTESIAN_POINT ( 'NONE',  ( -4.999999999999998224, -57.79166666393548013, 2.886751345948131764 ) ) ;
#15804=CARTESIAN_POINT ( 'NONE',  ( 1.060575238724906964E-15, -0.7500000000000007772, 5.773502691896257311 ) ) ;
#15805=CARTESIAN_POINT ( 'NONE',  ( -3.152548672688508926E-16, -66.56249999863440792, -5.148502694627439702 ) ) ;
#15808=CARTESIAN_POINT ( 'NONE',  ( 5.000000000000000000, -5.291666663935480130, -2.886751345948129988 ) ) ;
#15809=CARTESIAN_POINT ( 'NONE',  ( 2.229367062500001939, -34.97916666530107221, 3.861377020970579999 ) ) ;
#15810=VERTEX_POINT ( 'NONE', #17024 ) ;
#15811=DIRECTION ( 'NONE',  ( 0.000000000000000000, 0.000000000000000000, 1.000000000000000000 ) ) ;
#15813=CARTESIAN_POINT ( 'NONE',  ( -4.458734124999999437, 14.35416666803226171, -2.574251347313719407 ) ) ;
#15814=ORIENTED_EDGE ( 'NONE', *, *, #1635, .T. ) ;
#15816=CARTESIAN_POINT ( 'NONE',  ( -5.000000000000000000, -49.00000000000000000, 0.000000000000000000 ) ) ;
#15818=CARTESIAN_POINT ( 'NONE',  ( 5.000000000000000888, -4.583333333333334814, 2.886751345948126879 ) ) ;
#15819=CARTESIAN_POINT ( 'NONE',  ( -2.229367062499996610, -74.14583333196773651, 3.861377020970582219 ) ) ;
#15820=( BOUNDED_CURVE ( )  B_SPLINE_CURVE ( 2, ( #13385, #42332, #57153, #13068, #4056, #39388, #34244, #8871, #28797 ),
 .UNSPECIFIED., .F., .F. ) 
 B_SPLINE_CURVE_WITH_KNOTS ( ( 3, 2, 2, 2, 3 ),
 ( 0.3062500000000000222, 0.3069444444444444642, 0.3083333333333333481, 0.3097222222222222321, 0.3104166666666666741 ),
 .UNSPECIFIED. ) 
 CURVE ( )  GEOMETRIC_REPRESENTATION_ITEM ( )  RATIONAL_B_SPLINE_CURVE ( ( 0.9330127018922194093, 0.9330127018922194093, 1.000000000000000000, 0.8660254037844387076, 1.000000000000000000, 0.8660254037844387076, 1.000000000000000000, 0.9330127018922194093, 0.9330127018922194093 ) ) 
 REPRESENTATION_ITEM ( '' )  );
#15821=CARTESIAN_POINT ( 'NONE',  ( -5.000000000000000888, -169.5625000000000284, -2.071067811865475949 ) ) ;
#15822=CARTESIAN_POINT ( 'NONE',  ( -2.229367062499996610, -80.14583333196773651, 3.861377020970582219 ) ) ;
#15824=CARTESIAN_POINT ( 'NONE',  ( -2.229367062499996610, -28.39583333196774007, 3.861377020970582219 ) ) ;
#15826=LINE ( 'NONE', #20006, #16626 ) ;
#15827=ORIENTED_EDGE ( 'NONE', *, *, #38463, .F. ) ;
#15834=CARTESIAN_POINT ( 'NONE',  ( 4.458734125000001214, -67.14583333196773651, 2.574251347313718519 ) ) ;
#15837=ADVANCED_FACE ( 'NONE', ( #46294 ), #51126, .T. ) ;
#15840=CARTESIAN_POINT ( 'NONE',  ( -4.458734124999998549, 9.770833334698927786, 2.574251347313722516 ) ) ;
#15843=CARTESIAN_POINT ( 'NONE',  ( -3.152801135295367985, -160.8125000013656063, 3.152801135295367096 ) ) ;
#15844=( BOUNDED_CURVE ( )  B_SPLINE_CURVE ( 2, ( #3741, #19136, #38753, #14318, #23362, #38443, #48101, #33940, #29097 ),
 .UNSPECIFIED., .F., .F. ) 
 B_SPLINE_CURVE_WITH_KNOTS ( ( 3, 2, 2, 2, 3 ),
 ( 0.5354166666666666519, 0.5361111111111110938, 0.5374999999999999778, 0.5388888888888888618, 0.5395833333333333037 ),
 .UNSPECIFIED. ) 
 CURVE ( )  GEOMETRIC_REPRESENTATION_ITEM ( )  RATIONAL_B_SPLINE_CURVE ( ( 0.9330127018922194093, 0.9330127018922194093, 1.000000000000000000, 0.8660254037844387076, 1.000000000000000000, 0.8660254037844387076, 1.000000000000000000, 0.9330127018922194093, 0.9330127018922194093 ) ) 
 REPRESENTATION_ITEM ( '' )  );
#15855=CARTESIAN_POINT ( 'NONE',  ( 2.229367062499998831, 27.35416666803225993, -3.861377020970580887 ) ) ;
#15856=EDGE_CURVE ( 'NONE', #52220, #14909, #39450, .T. ) ;
#15859=CARTESIAN_POINT ( 'NONE',  ( 9.457646018065525792E-16, 1.687500001365593194, 5.148502694627439702 ) ) ;
#15862=EDGE_CURVE ( 'NONE', #33371, #30129, #36639, .T. ) ;
#15863=CARTESIAN_POINT ( 'NONE',  ( 3.535533905932736864, -146.2500000027311842, 3.535533905932738641 ) ) ;
#15864=DIRECTION ( 'NONE',  ( 0.000000000000000000, 0.000000000000000000, 1.000000000000000000 ) ) ;
#15872=CARTESIAN_POINT ( 'NONE',  ( -3.152801135295367985, -163.0625000013656063, 3.152801135295367096 ) ) ;
#15873=DIRECTION ( 'NONE',  ( -0.000000000000000000, 1.000000000000000000, -0.000000000000000000 ) ) ;
#15876=CARTESIAN_POINT ( 'NONE',  ( -8.190561711645485556E-16, -141.6875000013656063, 4.458734124999999437 ) ) ;
#15878=CARTESIAN_POINT ( 'NONE',  ( -2.229367062499996610, 20.60416666803225993, 3.861377020970582219 ) ) ;
#15880=CARTESIAN_POINT ( 'NONE',  ( -2.229367062500000163, -59.72916666530106511, -3.861377020970580443 ) ) ;
#15883=CARTESIAN_POINT ( 'NONE',  ( 5.000000000000000888, 12.41666666666666607, 2.886751345948126879 ) ) ;
#15884=CARTESIAN_POINT ( 'NONE',  ( -4.458734124999999437, -51.39583333196773651, -2.574251347313719407 ) ) ;
#15885=CARTESIAN_POINT ( 'NONE',  ( 4.458734124999999437, -12.81249999863440259, -5.460374474430324690E-16 ) ) ;
#15887=DIRECTION ( 'NONE',  ( -0.000000000000000000, 1.000000000000000000, -0.000000000000000000 ) ) ;
#15888=CARTESIAN_POINT ( 'NONE',  ( -1.339745962155610925, 0.3303418039926660499, 5.000000000000000000 ) ) ;
#15889=DIRECTION ( 'NONE',  ( 0.000000000000000000, 0.000000000000000000, 1.000000000000000000 ) ) ;
#15890=CARTESIAN_POINT ( 'NONE',  ( -6.972266317189433020E-16, -66.12499999726881583, -5.000000000000000000 ) ) ;
#15893=CARTESIAN_POINT ( 'NONE',  ( -4.458734124999999437, -60.31249999863440081, 0.000000000000000000 ) ) ;
#15894=CARTESIAN_POINT ( 'NONE',  ( -3.152801135295367985, -153.0625000013656063, 3.152801135295367096 ) ) ;
#15895=CARTESIAN_POINT ( 'NONE',  ( 4.458734125000001214, -64.89583333196773651, 2.574251347313718519 ) ) ;
#15897=CARTESIAN_POINT ( 'NONE',  ( 2.499999999999998668, -53.20833333060213732, -4.330127018922193649 ) ) ;
#15900=CARTESIAN_POINT ( 'NONE',  ( -4.458734124999998549, -1.479166665301071770, 2.574251347313722516 ) ) ;
#15901=ORIENTED_EDGE ( 'NONE', *, *, #48802, .T. ) ;
#15902=CARTESIAN_POINT ( 'NONE',  ( 0.000000000000000000, -170.0000000000000000, 0.000000000000000000 ) ) ;
#15904=CARTESIAN_POINT ( 'NONE',  ( 3.152801135295367541, -157.3125000013656063, -3.152801135295367541 ) ) ;
#15908=CARTESIAN_POINT ( 'NONE',  ( 3.061616997868383141E-16, -152.7500000000000000, -5.000000000000000000 ) ) ;
#15909=CARTESIAN_POINT ( 'NONE',  ( -2.229367062499996610, -50.39583333196772941, 3.861377020970582219 ) ) ;
#15913=CARTESIAN_POINT ( 'NONE',  ( -2.229367062499996610, -90.39583333196773651, 3.861377020970582219 ) ) ;
#15920=( BOUNDED_CURVE ( )  B_SPLINE_CURVE ( 2, ( #18835, #4367, #40361, #1156, #34908, #20755, #30390, #15925, #5639 ),
 .UNSPECIFIED., .F., .F. ) 
 B_SPLINE_CURVE_WITH_KNOTS ( ( 3, 2, 2, 2, 3 ),
 ( 0.03958333333333333842, 0.04027777777777778040, 0.04166666666666666435, 0.04305555555555555525, 0.04375000000000000416 ),
 .UNSPECIFIED. ) 
 CURVE ( )  GEOMETRIC_REPRESENTATION_ITEM ( )  RATIONAL_B_SPLINE_CURVE ( ( 0.9330127018922192983, 0.9330127018922196314, 1.000000000000000000, 0.8660254037844387076, 1.000000000000000000, 0.8660254037844387076, 1.000000000000000000, 0.9330127018922189652, 0.9330127018922192983 ) ) 
 REPRESENTATION_ITEM ( '' )  );
#15921=CARTESIAN_POINT ( 'NONE',  ( -5.000000000000000000, 6.999999999999999112, 0.000000000000000000 ) ) ;
#15922=CARTESIAN_POINT ( 'NONE',  ( -1.339745962155564296, -27.20534180126147916, -5.000000000000028422 ) ) ;
#15925=CARTESIAN_POINT ( 'NONE',  ( -1.339745962155608039, 24.79465819873852439, -5.000000000000004441 ) ) ;
#15926=DIRECTION ( 'NONE',  ( 0.000000000000000000, 0.000000000000000000, 1.000000000000000000 ) ) ;
#15927=FACE_OUTER_BOUND ( 'NONE', #36222, .T. ) ;
#15928=DIRECTION ( 'NONE',  ( -0.000000000000000000, 1.000000000000000000, -0.000000000000000000 ) ) ;
#15931=CARTESIAN_POINT ( 'NONE',  ( 1.339745962155615144, -31.70534180126147916, 4.999999999999999112 ) ) ;
#15933=CARTESIAN_POINT ( 'NONE',  ( 3.061616997868383141E-16, -155.8750000027311842, -5.000000000000000000 ) ) ;
#15945=CARTESIAN_POINT ( 'NONE',  ( 2.229367062500001939, -19.97916666530107221, 3.861377020970579999 ) ) ;
#15947=CARTESIAN_POINT ( 'NONE',  ( -5.000000000000000000, -151.5000000000000284, -6.123233995736766282E-16 ) ) ;
#15949=CARTESIAN_POINT ( 'NONE',  ( 3.152801135295367541, -150.3125000013655779, -3.152801135295367541 ) ) ;
#15951=CARTESIAN_POINT ( 'NONE',  ( 9.457646018065525792E-16, -46.31249999863440792, 5.148502694627439702 ) ) ;
#15952=CARTESIAN_POINT ( 'NONE',  ( -9.184850993605147944E-16, -150.2500000000000284, 5.000000000000000000 ) ) ;
#15953=DIRECTION ( 'NONE',  ( -0.000000000000000000, 1.000000000000000000, -0.000000000000000000 ) ) ;
#15954=CARTESIAN_POINT ( 'NONE',  ( 4.458734124999999437, -89.81249999863440792, -5.460374474430324690E-16 ) ) ;
#15956=CARTESIAN_POINT ( 'NONE',  ( 4.458734124999998549, 4.270833334698926897, -2.574251347313721627 ) ) ;
#15957=CARTESIAN_POINT ( 'NONE',  ( -2.071067811865432873, -142.6875000000000284, -5.000000000000041744 ) ) ;
#15960=CARTESIAN_POINT ( 'NONE',  ( 9.457646018065525792E-16, 16.68750000136559564, 5.148502694627439702 ) ) ;
#15962=CARTESIAN_POINT ( 'NONE',  ( -2.500000000000000444, 10.95833333606451632, -4.330127018922193649 ) ) ;
#15963=ORIENTED_EDGE ( 'NONE', *, *, #46410, .F. ) ;
#15964=ORIENTED_EDGE ( 'NONE', *, *, #37421, .T. ) ;
#15966=CARTESIAN_POINT ( 'NONE',  ( -4.458734124999998549, -45.22916666530106511, 2.574251347313722516 ) ) ;
#15967=CARTESIAN_POINT ( 'NONE',  ( 1.060575238724906964E-15, -38.62499999726881583, 5.773502691896257311 ) ) ;
#15968=ORIENTED_EDGE ( 'NONE', *, *, #4349, .T. ) ;
#15969=CARTESIAN_POINT ( 'NONE',  ( -4.458734124999999437, -20.31249999863440081, 0.000000000000000000 ) ) ;
#15971=CARTESIAN_POINT ( 'NONE',  ( -5.000000000000000000, -83.08333333333332860, -2.886751345948128211 ) ) ;
#15972=CARTESIAN_POINT ( 'NONE',  ( -4.458734124999999437, -168.9375000013656063, -5.460374474430324690E-16 ) ) ;
#15973=CARTESIAN_POINT ( 'NONE',  ( 5.000000000000000000, -86.29166666393547303, -2.886751345948129988 ) ) ;
#15974=CARTESIAN_POINT ( 'NONE',  ( 1.339745962155565406, -20.58034179853029144, 5.000000000000028422 ) ) ;
#15975=EDGE_LOOP ( 'NONE', ( #22319, #15814, #18805, #19760 ) ) ;
#15977=CARTESIAN_POINT ( 'NONE',  ( -4.458734124999999437, -31.56249999863440436, 0.000000000000000000 ) ) ;
#15978=CARTESIAN_POINT ( 'NONE',  ( -1.339745962155610925, -49.79465819873851729, 5.000000000000000000 ) ) ;
#15980=AXIS2_PLACEMENT_3D ( 'NONE', #33798, #53106, #3910 ) ;
#15985=ORIENTED_EDGE ( 'NONE', *, *, #44872, .F. ) ;
#15988=CARTESIAN_POINT ( 'NONE',  ( -4.458734124999998549, -76.47916666530105090, 2.574251347313722516 ) ) ;
#15991=CARTESIAN_POINT ( 'NONE',  ( -3.152801135295367096, -141.3125000013655779, -3.152801135295367541 ) ) ;
#15993=CARTESIAN_POINT ( 'NONE',  ( 2.500000000000002220, -84.54166666393547303, 4.330127018922192761 ) ) ;
#15995=CARTESIAN_POINT ( 'NONE',  ( -2.229367062499996610, -43.14583333196773651, 3.861377020970582219 ) ) ;
#15999=CARTESIAN_POINT ( 'NONE',  ( 4.458734124999999437, -139.6875000013656063, 0.000000000000000000 ) ) ;
#16004=CARTESIAN_POINT ( 'NONE',  ( -3.152548672688508926E-16, -75.81249999863440792, -5.148502694627439702 ) ) ;
#16005=CARTESIAN_POINT ( 'NONE',  ( -5.000000000000000000, -166.5000000000000000, -6.123233995736766282E-16 ) ) ;
#16013=DIRECTION ( 'NONE',  ( 0.000000000000000000, 0.000000000000000000, 1.000000000000000000 ) ) ;
#16015=CARTESIAN_POINT ( 'NONE',  ( 2.229367062500001939, 19.77083333469892779, 3.861377020970579999 ) ) ;
#16022=CARTESIAN_POINT ( 'NONE',  ( 4.458734124999999437, -82.81249999863440792, -5.460374474430324690E-16 ) ) ;
#16023=CARTESIAN_POINT ( 'NONE',  ( -4.458734124999997661, -3.229166665301069550, 2.574251347313722516 ) ) ;
#16024=CARTESIAN_POINT ( 'NONE',  ( -1.339745962155610925, -30.79465819873851373, 5.000000000000000000 ) ) ;
#16025=VERTEX_POINT ( 'NONE', #52072 ) ;
#16026=CARTESIAN_POINT ( 'NONE',  ( -4.458734124999999437, -32.56249999863440792, 0.000000000000000000 ) ) ;
#16030=VECTOR ( 'NONE', #62769, 1000.000000000000000 ) ;
#16031=CARTESIAN_POINT ( 'NONE',  ( -3.152548672688508926E-16, 20.43750000136559208, -5.148502694627439702 ) ) ;
#16033=CARTESIAN_POINT ( 'NONE',  ( 9.457646018065525792E-16, -77.31249999863440792, 5.148502694627439702 ) ) ;
#16036=CARTESIAN_POINT ( 'NONE',  ( -2.499999999999996447, 25.29166666939785202, 4.330127018922195425 ) ) ;
#16038=CARTESIAN_POINT ( 'NONE',  ( 0.000000000000000000, -170.0000000000000000, 5.000000000000000000 ) ) ;
#16039=CARTESIAN_POINT ( 'NONE',  ( -9.184850993605147944E-16, -158.3750000027311842, 5.000000000000000000 ) ) ;
#16040=( BOUNDED_CURVE ( )  B_SPLINE_CURVE ( 2, ( #52867, #32296, #18133, #23286, #37139, #37446, #51616, #57077, #27161 ),
 .UNSPECIFIED., .F., .F. ) 
 B_SPLINE_CURVE_WITH_KNOTS ( ( 3, 2, 2, 2, 3 ),
 ( 0.9562500000000000444, 0.9569444444444444864, 0.9583333333333333703, 0.9597222222222222543, 0.9604166666666666963 ),
 .UNSPECIFIED. ) 
 CURVE ( )  GEOMETRIC_REPRESENTATION_ITEM ( )  RATIONAL_B_SPLINE_CURVE ( ( 0.9330127018922194093, 0.9330127018922194093, 1.000000000000000000, 0.8660254037844387076, 1.000000000000000000, 0.8660254037844387076, 1.000000000000000000, 0.9330127018922194093, 0.9330127018922194093 ) ) 
 REPRESENTATION_ITEM ( '' )  );
#16041=CARTESIAN_POINT ( 'NONE',  ( -2.500000000000000444, -22.16666666666666785, -4.330127018922193649 ) ) ;
#16042=CARTESIAN_POINT ( 'NONE',  ( 4.458734124999999437, -25.81249999863440792, -5.460374474430324690E-16 ) ) ;
#16043=EDGE_CURVE ( 'NONE', #22858, #13416, #52617, .T. ) ;
#16044=CARTESIAN_POINT ( 'NONE',  ( 9.457646018065525792E-16, -89.06249999863439371, 5.148502694627439702 ) ) ;
#16045=CARTESIAN_POINT ( 'NONE',  ( 1.060575238724906964E-15, -24.62499999726881228, 5.773502691896257311 ) ) ;
#16046=CARTESIAN_POINT ( 'NONE',  ( -4.458734124999999437, -53.31249999863439371, 0.000000000000000000 ) ) ;
#16047=VERTEX_POINT ( 'NONE', #22170 ) ;
#16048=LINE ( 'NONE', #46275, #29449 ) ;
#16049=CARTESIAN_POINT ( 'NONE',  ( 5.000000000000000000, -74.29166666393547303, -2.886751345948130876 ) ) ;
#16050=CARTESIAN_POINT ( 'NONE',  ( -2.229367062500000163, -2.729166665301069550, -3.861377020970580443 ) ) ;
#16051=VERTEX_POINT ( 'NONE', #17340 ) ;
#16053=CARTESIAN_POINT ( 'NONE',  ( 2.500000000000002220, -68.66666666666667140, 4.330127018922192761 ) ) ;
#16054=CARTESIAN_POINT ( 'NONE',  ( -4.458734125000001214, -151.1250000013655779, 1.846868145590734089 ) ) ;
#16057=CARTESIAN_POINT ( 'NONE',  ( -5.000000000000000888, -158.4375000000000568, 2.071067811865474617 ) ) ;
#16058=DIRECTION ( 'NONE',  ( -0.000000000000000000, 1.000000000000000000, -0.000000000000000000 ) ) ;
#16060=CARTESIAN_POINT ( 'NONE',  ( 4.458734125000001214, -11.14583333196774007, 2.574251347313718519 ) ) ;
#16061=CARTESIAN_POINT ( 'NONE',  ( -4.458734124999998549, -53.47916666530106511, 2.574251347313722516 ) ) ;
#16063=CARTESIAN_POINT ( 'NONE',  ( 1.339745962155615144, 10.29465819873852084, 4.999999999999999112 ) ) ;
#16064=CARTESIAN_POINT ( 'NONE',  ( 1.846868145590735200, -144.2500000013656063, -4.458734125000000326 ) ) ;
#16065=EDGE_CURVE ( 'NONE', #34014, #62883, #42089, .T. ) ;
#16068=ORIENTED_EDGE ( 'NONE', *, *, #52213, .T. ) ;
#16070=CARTESIAN_POINT ( 'NONE',  ( 2.229367062500001939, 27.77083333469892779, 3.861377020970579999 ) ) ;
#16074=ORIENTED_EDGE ( 'NONE', *, *, #33852, .T. ) ;
#16075=EDGE_CURVE ( 'NONE', #51351, #20487, #8013, .T. ) ;
#16081=CARTESIAN_POINT ( 'NONE',  ( -3.152548672688508926E-16, -7.562499998634404363, -5.148502694627439702 ) ) ;
#16083=CARTESIAN_POINT ( 'NONE',  ( -3.152801135295367096, -150.0625000013655779, -3.152801135295367541 ) ) ;
#16086=CARTESIAN_POINT ( 'NONE',  ( -9.184850993605147944E-16, -148.2500000000000284, 5.000000000000000000 ) ) ;
#16090=CARTESIAN_POINT ( 'NONE',  ( -1.339745962155613812, -6.205341801261478274, -5.000000000000000000 ) ) ;
#16092=EDGE_CURVE ( 'NONE', #328, #1738, #2117, .T. ) ;
#16096=CYLINDRICAL_SURFACE ( 'NONE', #31446, 5.000000000000000000 ) ;
#16098=CARTESIAN_POINT ( 'NONE',  ( -4.458734124999997661, 14.77083333469892779, 2.574251347313722516 ) ) ;
#16100=CARTESIAN_POINT ( 'NONE',  ( -4.458734124999999437, -16.64583333196773651, -2.574251347313719407 ) ) ;
#16102=CARTESIAN_POINT ( 'NONE',  ( -1.846868145590737420, -163.7500000013655779, 4.458734124999999437 ) ) ;
#16106=CARTESIAN_POINT ( 'NONE',  ( 2.500000000000002220, -38.66666666666667140, 4.330127018922192761 ) ) ;
#16109=CARTESIAN_POINT ( 'NONE',  ( -2.229367062499996610, -36.14583333196773651, 3.861377020970582219 ) ) ;
#16110=CARTESIAN_POINT ( 'NONE',  ( 5.000000000000000000, -51.37499999726881583, -6.123233995736766282E-16 ) ) ;
#16117=CARTESIAN_POINT ( 'NONE',  ( -3.535250795749689387E-16, -3.250000000000003109, -5.773502691896257311 ) ) ;
#16119=CARTESIAN_POINT ( 'NONE',  ( 2.229367062499998831, -70.64583333196773651, -3.861377020970580887 ) ) ;
#16120=AXIS2_PLACEMENT_3D ( 'NONE', #33944, #43583, #54194 ) ;
#16124=EDGE_CURVE ( 'NONE', #49284, #52288, #23124, .T. ) ;
#16125=CARTESIAN_POINT ( 'NONE',  ( -2.499999999999996447, -6.708333330602149758, 4.330127018922195425 ) ) ;
#16126=CARTESIAN_POINT ( 'NONE',  ( -4.458734124999998549, -38.22916666530107932, 2.574251347313722516 ) ) ;
#16130=CARTESIAN_POINT ( 'NONE',  ( 4.458734125000001214, 12.85416666803226171, 2.574251347313718519 ) ) ;
#16133=CARTESIAN_POINT ( 'NONE',  ( 2.499999999999998668, -48.33333333333332860, -4.330127018922193649 ) ) ;
#16135=CARTESIAN_POINT ( 'NONE',  ( -4.999999999999998224, 14.20833333606451987, 2.886751345948131764 ) ) ;
#16136=CARTESIAN_POINT ( 'NONE',  ( 4.458734124999999437, -73.81249999863440792, -5.460374474430324690E-16 ) ) ;
#16137=CARTESIAN_POINT ( 'NONE',  ( 4.458734124999999437, -139.6875000013656063, 0.000000000000000000 ) ) ;
#16138=CARTESIAN_POINT ( 'NONE',  ( -4.458734124999999437, -83.39583333196772230, -2.574251347313719407 ) ) ;
#16140=CARTESIAN_POINT ( 'NONE',  ( -2.229367062500000163, -37.72916666530107221, -3.861377020970580443 ) ) ;
#16142=ORIENTED_EDGE ( 'NONE', *, *, #41855, .F. ) ;
#16147=CARTESIAN_POINT ( 'NONE',  ( -5.000000000000000000, -75.87499999726880162, 0.000000000000000000 ) ) ;
#16148=CARTESIAN_POINT ( 'NONE',  ( 4.458734125000001214, -65.14583333196773651, 2.574251347313718519 ) ) ;
#16153=ORIENTED_EDGE ( 'NONE', *, *, #51519, .F. ) ;
#16155=CARTESIAN_POINT ( 'NONE',  ( 2.229367062500001939, 9.020833334698927786, 3.861377020970579999 ) ) ;
#16156=CARTESIAN_POINT ( 'NONE',  ( -6.972266317189433020E-16, -76.24999999999998579, -5.000000000000000000 ) ) ;
#16157=CARTESIAN_POINT ( 'NONE',  ( 3.152801135295367541, -159.3125000013656063, -3.152801135295367541 ) ) ;
#16163=VECTOR ( 'NONE', #41180, 1000.000000000000000 ) ;
#16165=DIRECTION ( 'NONE',  ( -0.000000000000000000, 1.000000000000000000, -0.000000000000000000 ) ) ;
#16167=VECTOR ( 'NONE', #5312, 1000.000000000000000 ) ;
#16169=CARTESIAN_POINT ( 'NONE',  ( 5.000000000000000000, 12.62500000273118417, -6.123233995736766282E-16 ) ) ;
#16172=CARTESIAN_POINT ( 'NONE',  ( 1.339745962155615144, -82.58034179853028434, 4.999999999999999112 ) ) ;
#16175=CARTESIAN_POINT ( 'NONE',  ( 2.229367062500001939, -0.2291666653010705768, 3.861377020970579999 ) ) ;
#16176=DIRECTION ( 'NONE',  ( -0.000000000000000000, 1.000000000000000000, -0.000000000000000000 ) ) ;
#16178=CARTESIAN_POINT ( 'NONE',  ( 5.000000000000000000, -144.1875000027312126, 2.071067811865478614 ) ) ;
#16183=DIRECTION ( 'NONE',  ( -0.000000000000000000, 1.000000000000000000, -0.000000000000000000 ) ) ;
#16184=CARTESIAN_POINT ( 'NONE',  ( 3.061616997868383141E-16, -140.8750000027312126, -5.000000000000000000 ) ) ;
#16186=CARTESIAN_POINT ( 'NONE',  ( 4.458734124999997661, -162.7500000013655779, 1.846868145590737864 ) ) ;
#16187=CARTESIAN_POINT ( 'NONE',  ( -5.000000000000000888, -159.5625000027312126, 2.071067811865474617 ) ) ;
#16189=CARTESIAN_POINT ( 'NONE',  ( -4.999999999999998224, -56.91666666666667140, 2.886751345948131764 ) ) ;
#16191=CARTESIAN_POINT ( 'NONE',  ( -2.229367062499996610, 24.60416666803225993, 3.861377020970582219 ) ) ;
#16192=ORIENTED_EDGE ( 'NONE', *, *, #38989, .F. ) ;
#16194=CARTESIAN_POINT ( 'NONE',  ( -1.339745962155613812, -3.080341798530293218, -5.000000000000000000 ) ) ;
#16195=CARTESIAN_POINT ( 'NONE',  ( 2.499999999999998668, 12.66666666666666607, -4.330127018922193649 ) ) ;
#16196=CARTESIAN_POINT ( 'NONE',  ( 4.458734124999998549, -48.72916666530106511, -2.574251347313721627 ) ) ;
#16197=CARTESIAN_POINT ( 'NONE',  ( 4.458734124999998549, -12.72916666530107044, -2.574251347313721627 ) ) ;
#16199=EDGE_CURVE ( 'NONE', #38064, #5879, #53546, .T. ) ;
#16200=EDGE_CURVE ( 'NONE', #9714, #62942, #25178, .T. ) ;
#16203=EDGE_CURVE ( 'NONE', #47984, #25841, #16550, .T. ) ;
#16204=CARTESIAN_POINT ( 'NONE',  ( 3.061616997868383141E-16, -153.7500000000000000, -5.000000000000000000 ) ) ;
#16205=CARTESIAN_POINT ( 'NONE',  ( -5.000000000000000000, -35.00000000000000000, 0.000000000000000000 ) ) ;
#16207=CARTESIAN_POINT ( 'NONE',  ( -5.000000000000000000, -59.00000000000000000, 0.000000000000000000 ) ) ;
#16209=EDGE_CURVE ( 'NONE', #20078, #50991, #49025, .T. ) ;
#16211=LINE ( 'NONE', #6885, #889 ) ;
#16212=CARTESIAN_POINT ( 'NONE',  ( 4.458734124999999437, -58.81249999863440081, -5.460374474430324690E-16 ) ) ;
#16213=CARTESIAN_POINT ( 'NONE',  ( -4.458734125000000326, -151.2500000013656063, -1.846868145590735644 ) ) ;
#16214=CARTESIAN_POINT ( 'NONE',  ( 4.458734125000001214, -67.89583333196773651, 2.574251347313718519 ) ) ;
#16215=VECTOR ( 'NONE', #12777, 1000.000000000000000 ) ;
#16216=EDGE_CURVE ( 'NONE', #46845, #47715, #60525, .T. ) ;
#16217=ADVANCED_FACE ( 'NONE', ( #10514 ), #252, .T. ) ;
#16218=CARTESIAN_POINT ( 'NONE',  ( 5.000000000000000000, -57.29166666393548013, -2.886751345948129988 ) ) ;
#16219=VERTEX_POINT ( 'NONE', #11157 ) ;
#16220=CARTESIAN_POINT ( 'NONE',  ( 2.500000000000002220, -26.66666666666666430, 4.330127018922192761 ) ) ;
#16221=ORIENTED_EDGE ( 'NONE', *, *, #13315, .F. ) ;
#16224=CARTESIAN_POINT ( 'NONE',  ( -1.846868145590734756, -153.1250000013656063, -4.458734125000000326 ) ) ;
#16225=EDGE_CURVE ( 'NONE', #2151, #51364, #44518, .T. ) ;
#16226=ORIENTED_EDGE ( 'NONE', *, *, #49152, .F. ) ;
#16227=( BOUNDED_CURVE ( )  B_SPLINE_CURVE ( 2, ( #45498, #25242, #179, #20097, #44857, #820, #20746, #39703, #20425 ),
 .UNSPECIFIED., .F., .F. ) 
 B_SPLINE_CURVE_WITH_KNOTS ( ( 3, 2, 2, 2, 3 ),
 ( 0.1416666666666667740, 0.1458333333333334814, 0.1500000000000001332, 0.1541666666666668406, 0.1583333333333334925 ),
 .UNSPECIFIED. ) 
 CURVE ( )  GEOMETRIC_REPRESENTATION_ITEM ( )  RATIONAL_B_SPLINE_CURVE ( ( 0.9999999999999980016, 0.9238795325112887369, 1.000000000000000000, 0.9238795325112867385, 1.000000000000000000, 0.9238795325112867385, 1.000000000000000000, 0.9238795325112837409, 1.000000000000003109 ) ) 
 REPRESENTATION_ITEM ( '' )  );
#16229=DIRECTION ( 'NONE',  ( -0.000000000000000000, 1.000000000000000000, -0.000000000000000000 ) ) ;
#16231=CARTESIAN_POINT ( 'NONE',  ( 5.000000000000000888, -80.45833333060213022, 2.886751345948126879 ) ) ;
#16232=CARTESIAN_POINT ( 'NONE',  ( -3.152548672688508926E-16, -48.81249999863440792, -5.148502694627439702 ) ) ;
#16235=EDGE_CURVE ( 'NONE', #34949, #18684, #53918, .T. ) ;
#16238=CARTESIAN_POINT ( 'NONE',  ( 9.457646018065525792E-16, 22.93750000136559919, 5.148502694627439702 ) ) ;
#16249=DIRECTION ( 'NONE',  ( -0.000000000000000000, 1.000000000000000000, -0.000000000000000000 ) ) ;
#16251=CARTESIAN_POINT ( 'NONE',  ( -6.972266317189433020E-16, -87.25000000000001421, -5.000000000000000000 ) ) ;
#16256=CARTESIAN_POINT ( 'NONE',  ( -3.535533905932737309, -143.7500000027311842, -3.535533905932738197 ) ) ;
#16258=CARTESIAN_POINT ( 'NONE',  ( 5.000000000000000888, -157.0625000027311842, -2.071067811865475505 ) ) ;
#16269=CARTESIAN_POINT ( 'NONE',  ( -2.229367062499996610, -18.14583333196773651, 3.861377020970582219 ) ) ;
#16271=CARTESIAN_POINT ( 'NONE',  ( 3.535533905932738197, -149.8750000000000000, -3.535533905932738197 ) ) ;
#16273=CARTESIAN_POINT ( 'NONE',  ( -1.846868145590734756, -153.1250000013656063, -4.458734125000000326 ) ) ;
#16274=VERTEX_POINT ( 'NONE', #50715 ) ;
#16275=CARTESIAN_POINT ( 'NONE',  ( 4.458734125000000326, -48.14583333196773651, 2.574251347313718519 ) ) ;
#16278=CARTESIAN_POINT ( 'NONE',  ( -4.999999999999999112, 27.08333333333333215, 2.886751345948131764 ) ) ;
#16279=CARTESIAN_POINT ( 'NONE',  ( 2.229367062499998831, 3.354166668032259935, -3.861377020970580887 ) ) ;
#16280=CARTESIAN_POINT ( 'NONE',  ( -1.339745962155613812, -74.08034179853029855, -5.000000000000000000 ) ) ;
#16281=CARTESIAN_POINT ( 'NONE',  ( -6.972266317189433020E-16, 13.74999999999999822, -5.000000000000000000 ) ) ;
#16282=CARTESIAN_POINT ( 'NONE',  ( -1.049326080737009628E-13, -17.75000000000000355, 5.000000000000000000 ) ) ;
#16283=CARTESIAN_POINT ( 'NONE',  ( -4.458734124999999437, 17.43750000136559208, 0.000000000000000000 ) ) ;
#16285=CARTESIAN_POINT ( 'NONE',  ( 2.499999999999998668, 7.791666669397852019, -4.330127018922193649 ) ) ;
#16290=CARTESIAN_POINT ( 'NONE',  ( -2.229367062499996610, -42.14583333196773651, 3.861377020970582219 ) ) ;
#16291=CARTESIAN_POINT ( 'NONE',  ( 4.458734125000000326, -162.6250000013655779, -1.846868145590734978 ) ) ;
#16292=CARTESIAN_POINT ( 'NONE',  ( -5.000000000000000000, -41.95833333060214443, -2.886751345948128211 ) ) ;
#16294=CARTESIAN_POINT ( 'NONE',  ( -2.229367062500000163, -15.47916666530107399, -3.861377020970580443 ) ) ;
#16296=CARTESIAN_POINT ( 'NONE',  ( 5.000000000000000000, -86.41666666666667140, -2.886751345948129988 ) ) ;
#16297=CARTESIAN_POINT ( 'NONE',  ( -4.458734124999999437, -167.9375000013655779, -5.460374474430324690E-16 ) ) ;
#16299=CARTESIAN_POINT ( 'NONE',  ( 2.499999999999998668, -88.20833333060214443, -4.330127018922193649 ) ) ;
#16303=CARTESIAN_POINT ( 'NONE',  ( 4.458734124999999437, -30.06249999863440436, -5.460374474430324690E-16 ) ) ;
#16306=( BOUNDED_CURVE ( )  B_SPLINE_CURVE ( 2, ( #45658, #46296, #26352, #41770, #1615, #26677, #21541, #45974, #41137 ),
 .UNSPECIFIED., .F., .F. ) 
 B_SPLINE_CURVE_WITH_KNOTS ( ( 3, 2, 2, 2, 3 ),
 ( 0.4750000000000004219, 0.4791666666666671293, 0.4833333333333337811, 0.4875000000000004330, 0.4916666666666670849 ),
 .UNSPECIFIED. ) 
 CURVE ( )  GEOMETRIC_REPRESENTATION_ITEM ( )  RATIONAL_B_SPLINE_CURVE ( ( 0.9999999999999918954, 0.9238795325112948431, 1.000000000000000000, 0.9238795325112867385, 1.000000000000000000, 0.9238795325112867385, 1.000000000000000000, 0.9238795325112786339, 1.000000000000008216 ) ) 
 REPRESENTATION_ITEM ( '' )  );
#16312=CARTESIAN_POINT ( 'NONE',  ( -5.000000000000000000, -26.08333333333332860, -2.886751345948128211 ) ) ;
#16314=CARTESIAN_POINT ( 'NONE',  ( 4.458734124999999437, -78.06249999863440792, -5.460374474430324690E-16 ) ) ;
#16317=CARTESIAN_POINT ( 'NONE',  ( 4.458734124999999437, -143.6250000013656347, -1.846868145590734978 ) ) ;
#16318=CARTESIAN_POINT ( 'NONE',  ( 1.975475456537005874E-15, 20.24999999999999289, 5.000000000000000000 ) ) ;
#16320=CARTESIAN_POINT ( 'NONE',  ( 4.458734124999999437, -43.81249999863440081, -5.460374474430324690E-16 ) ) ;
#16323=VECTOR ( 'NONE', #15873, 1000.000000000000000 ) ;
#16325=( BOUNDED_CURVE ( )  B_SPLINE_CURVE ( 2, ( #54376, #38928, #28959, #4523, #48582, #58562, #53728, #9659, #48897 ),
 .UNSPECIFIED., .F., .F. ) 
 B_SPLINE_CURVE_WITH_KNOTS ( ( 3, 2, 2, 2, 3 ),
 ( 0.5854166666666666963, 0.5861111111111111382, 0.5875000000000000222, 0.5888888888888889062, 0.5895833333333333481 ),
 .UNSPECIFIED. ) 
 CURVE ( )  GEOMETRIC_REPRESENTATION_ITEM ( )  RATIONAL_B_SPLINE_CURVE ( ( 0.9330127018922194093, 0.9330127018922194093, 1.000000000000000000, 0.8660254037844387076, 1.000000000000000000, 0.8660254037844387076, 1.000000000000000000, 0.9330127018922194093, 0.9330127018922194093 ) ) 
 REPRESENTATION_ITEM ( '' )  );
#16326=CARTESIAN_POINT ( 'NONE',  ( -2.071067811865446640, -167.3125000000000000, 5.000000000000031086 ) ) ;
#16330=CARTESIAN_POINT ( 'NONE',  ( -4.458734124999998549, -78.47916666530107932, 2.574251347313722516 ) ) ;
#16338=CARTESIAN_POINT ( 'NONE',  ( 5.000000000000000000, -169.1250000027312126, 0.000000000000000000 ) ) ;
#16340=CARTESIAN_POINT ( 'NONE',  ( 9.457646018065525792E-16, 18.68750000136559208, 5.148502694627439702 ) ) ;
#16341=CARTESIAN_POINT ( 'NONE',  ( 1.339745962155612702, -77.16965819600731891, -5.000000000000000000 ) ) ;
#16346=CARTESIAN_POINT ( 'NONE',  ( -6.972266317189433020E-16, -38.12499999726880873, -5.000000000000000000 ) ) ;
#16347=CARTESIAN_POINT ( 'NONE',  ( -2.229367062500000163, -87.47916666530107932, -3.861377020970580443 ) ) ;
#16348=CARTESIAN_POINT ( 'NONE',  ( -4.458734124999999437, -3.312499998634407916, 0.000000000000000000 ) ) ;
#16349=DIRECTION ( 'NONE',  ( -0.000000000000000000, 1.000000000000000000, -0.000000000000000000 ) ) ;
#16351=CARTESIAN_POINT ( 'NONE',  ( -3.152548672688508926E-16, -31.81249999863440436, -5.148502694627439702 ) ) ;
#16352=AXIS2_PLACEMENT_3D ( 'NONE', #40548, #11911, #36684 ) ;
#16356=VECTOR ( 'NONE', #7148, 1000.000000000000000 ) ;
#16357=CARTESIAN_POINT ( 'NONE',  ( -4.458734124999998549, 20.77083333469892779, 2.574251347313722516 ) ) ;
#16358=CARTESIAN_POINT ( 'NONE',  ( 0.000000000000000000, -170.0000000000000000, 5.000000000000000000 ) ) ;
#16359=CARTESIAN_POINT ( 'NONE',  ( -2.229367062499996610, -79.39583333196773651, 3.861377020970582219 ) ) ;
#16361=DIRECTION ( 'NONE',  ( 0.000000000000000000, 0.000000000000000000, 1.000000000000000000 ) ) ;
#16362=CARTESIAN_POINT ( 'NONE',  ( -2.500000000000000444, 24.95833333606451987, -4.330127018922193649 ) ) ;
#16363=ORIENTED_EDGE ( 'NONE', *, *, #56675, .F. ) ;
#16366=CARTESIAN_POINT ( 'NONE',  ( 1.975475456537005874E-15, -60.62499999726880162, 5.000000000000000000 ) ) ;
#16367=CARTESIAN_POINT ( 'NONE',  ( 5.000000000000000000, -22.50000000000000000, -6.123233995736766282E-16 ) ) ;
#16368=CARTESIAN_POINT ( 'NONE',  ( 2.229367062500001939, -27.97916666530107221, 3.861377020970579999 ) ) ;
#16370=CARTESIAN_POINT ( 'NONE',  ( -4.458734124999999437, -86.31249999863439371, 0.000000000000000000 ) ) ;
#16371=CARTESIAN_POINT ( 'NONE',  ( -5.000000000000000000, -20.95833333060214798, -2.886751345948128211 ) ) ;
#16372=CARTESIAN_POINT ( 'NONE',  ( -3.152548672688508926E-16, -56.56249999863439371, -5.148502694627439702 ) ) ;
#16373=ORIENTED_EDGE ( 'NONE', *, *, #33581, .T. ) ;
#16374=CARTESIAN_POINT ( 'NONE',  ( 5.000000000000000888, -49.58333333333332149, 2.886751345948126879 ) ) ;
#16376=CARTESIAN_POINT ( 'NONE',  ( -4.458734124999998549, -4.479166665301070438, 2.574251347313722516 ) ) ;
#16378=CARTESIAN_POINT ( 'NONE',  ( 2.500000000000002220, -70.66666666666667140, 4.330127018922192761 ) ) ;
#16379=CARTESIAN_POINT ( 'NONE',  ( 4.458734125000000326, -153.6250000013655779, -1.846868145590734978 ) ) ;
#16383=CARTESIAN_POINT ( 'NONE',  ( -3.535533905932738641, -157.3750000000000284, 3.535533905932737309 ) ) ;
#16384=CARTESIAN_POINT ( 'NONE',  ( -1.339745962155613812, -86.20534180126146850, -5.000000000000000000 ) ) ;
#16386=CARTESIAN_POINT ( 'NONE',  ( -2.229367062499996610, -17.39583333196773651, 3.861377020970582219 ) ) ;
#16387=CARTESIAN_POINT ( 'NONE',  ( 2.229367062499998831, -53.89583333196773651, -3.861377020970580887 ) ) ;
#16389=CARTESIAN_POINT ( 'NONE',  ( 3.152801135295366208, -145.5625000013655779, 3.152801135295367985 ) ) ;
#16392=VERTEX_POINT ( 'NONE', #7931 ) ;
#16394=CARTESIAN_POINT ( 'NONE',  ( 4.458734124999999437, 25.93750000136559564, -5.460374474430324690E-16 ) ) ;
#16396=CYLINDRICAL_SURFACE ( 'NONE', #63020, 5.000000000000000000 ) ;
#16397=AXIS2_PLACEMENT_3D ( 'NONE', #56987, #61077, #20560 ) ;
#16400=CARTESIAN_POINT ( 'NONE',  ( 3.061616997868383141E-16, -164.7500000000000000, -5.000000000000000000 ) ) ;
#16403=CARTESIAN_POINT ( 'NONE',  ( 4.458734124999999437, -8.812499998634406140, -5.460374474430324690E-16 ) ) ;
#16404=CARTESIAN_POINT ( 'NONE',  ( 5.000000000000000888, 6.541666669397851130, 2.886751345948126879 ) ) ;
#16405=CARTESIAN_POINT ( 'NONE',  ( 1.846868145590736310, -148.6250000013655779, 4.458734124999997661 ) ) ;
#16413=CARTESIAN_POINT ( 'NONE',  ( 5.000000000000000000, -85.29166666393547303, -2.886751345948130876 ) ) ;
#16414=CARTESIAN_POINT ( 'NONE',  ( 0.000000000000000000, -170.0000000000000000, 0.000000000000000000 ) ) ;
#16420=CARTESIAN_POINT ( 'NONE',  ( -6.972266317189433020E-16, 9.750000000000000000, -5.000000000000000000 ) ) ;
#16421=CARTESIAN_POINT ( 'NONE',  ( 4.458734124999998549, 14.27083333469892601, -2.574251347313721627 ) ) ;
#16423=CARTESIAN_POINT ( 'NONE',  ( -3.152548672688508926E-16, -16.81249999863440436, -5.148502694627439702 ) ) ;
#16425=CARTESIAN_POINT ( 'NONE',  ( -4.458734125000000326, -163.0000000013655779, -1.846868145590735644 ) ) ;
#16432=CARTESIAN_POINT ( 'NONE',  ( -2.229367062500000163, -37.47916666530107221, -3.861377020970580443 ) ) ;
#16440=CARTESIAN_POINT ( 'NONE',  ( -6.972266317189433020E-16, -9.124999997268814056, -5.000000000000000000 ) ) ;
#16441=CARTESIAN_POINT ( 'NONE',  ( -2.499999999999996447, -9.833333333333332149, 4.330127018922195425 ) ) ;
#16442=CARTESIAN_POINT ( 'NONE',  ( -3.152548672688508926E-16, -73.56249999863439371, -5.148502694627439702 ) ) ;
#16443=CARTESIAN_POINT ( 'NONE',  ( 1.975475456537005874E-15, -22.62499999726880873, 5.000000000000000000 ) ) ;
#16444=CARTESIAN_POINT ( 'NONE',  ( 2.500000000000002220, -7.541666663935481907, 4.330127018922192761 ) ) ;
#16445=VECTOR ( 'NONE', #43446, 1000.000000000000000 ) ;
#16446=CARTESIAN_POINT ( 'NONE',  ( -3.152548672688508926E-16, -37.56249999863440792, -5.148502694627439702 ) ) ;
#16447=ORIENTED_EDGE ( 'NONE', *, *, #1594, .F. ) ;
#16449=CARTESIAN_POINT ( 'NONE',  ( -2.229367062499996610, 10.60416666803225993, 3.861377020970582219 ) ) ;
#16452=CARTESIAN_POINT ( 'NONE',  ( -3.535250795749689387E-16, -57.25000000000000000, -5.773502691896257311 ) ) ;
#16454=CARTESIAN_POINT ( 'NONE',  ( 2.500000000000002220, -4.666666666666666075, 4.330127018922192761 ) ) ;
#16455=CARTESIAN_POINT ( 'NONE',  ( 2.229367062500001939, -77.97916666530106511, 3.861377020970579999 ) ) ;
#16456=CARTESIAN_POINT ( 'NONE',  ( 1.846868145590736310, -141.8750000013656063, 4.458734124999999437 ) ) ;
#16457=CARTESIAN_POINT ( 'NONE',  ( 2.229367062500001939, -86.97916666530107932, 3.861377020970579999 ) ) ;
#16459=CARTESIAN_POINT ( 'NONE',  ( -4.458734124999998549, -37.47916666530107221, 2.574251347313722516 ) ) ;
#16460=CARTESIAN_POINT ( 'NONE',  ( 1.255007937094098239E-14, 23.87500000273118417, -4.999999999999999112 ) ) ;
#16466=CARTESIAN_POINT ( 'NONE',  ( 6.123233995736766282E-16, -170.0000000000000000, -5.000000000000000000 ) ) ;
#16467=CARTESIAN_POINT ( 'NONE',  ( -3.152548672688508926E-16, -65.81249999863440792, -5.148502694627439702 ) ) ;
#16470=CARTESIAN_POINT ( 'NONE',  ( -5.000000000000000888, -156.5625000027311842, 2.071067811865474617 ) ) ;
#16474=CARTESIAN_POINT ( 'NONE',  ( 4.458734124999998549, 5.270833334698926897, -2.574251347313721627 ) ) ;
#16477=CARTESIAN_POINT ( 'NONE',  ( -8.190561711645485556E-16, -159.6875000013655779, 4.458734124999999437 ) ) ;
#16478=DIRECTION ( 'NONE',  ( -0.000000000000000000, 1.000000000000000000, -0.000000000000000000 ) ) ;
#16479=ORIENTED_EDGE ( 'NONE', *, *, #10548, .F. ) ;
#16485=CYLINDRICAL_SURFACE ( 'NONE', #19084, 5.000000000000000000 ) ;
#16487=CYLINDRICAL_SURFACE ( 'NONE', #55481, 5.000000000000000000 ) ;
#16490=CARTESIAN_POINT ( 'NONE',  ( 9.457646018065525792E-16, 25.93750000136559564, 5.148502694627439702 ) ) ;
#16493=CARTESIAN_POINT ( 'NONE',  ( -4.458734124999999437, 1.437500001365592972, 0.000000000000000000 ) ) ;
#16495=CARTESIAN_POINT ( 'NONE',  ( 2.071067811865475505, -145.9375000027312126, -5.000000000000000888 ) ) ;
#16496=CARTESIAN_POINT ( 'NONE',  ( 0.000000000000000000, -170.0000000000000000, 5.000000000000000000 ) ) ;
#16497=EDGE_CURVE ( 'NONE', #48477, #11293, #27630, .T. ) ;
#16501=( BOUNDED_CURVE ( )  B_SPLINE_CURVE ( 2, ( #54430, #17423, #31886, #30930, #46367, #56665, #2951, #35765, #16460 ),
 .UNSPECIFIED., .F., .F. ) 
 B_SPLINE_CURVE_WITH_KNOTS ( ( 3, 2, 2, 2, 3 ),
 ( 0.03958333333333333842, 0.04027777777777778040, 0.04166666666666666435, 0.04305555555555555525, 0.04375000000000000416 ),
 .UNSPECIFIED. ) 
 CURVE ( )  GEOMETRIC_REPRESENTATION_ITEM ( )  RATIONAL_B_SPLINE_CURVE ( ( 0.9330127018922192983, 0.9330127018922196314, 1.000000000000000000, 0.8660254037844387076, 1.000000000000000000, 0.8660254037844387076, 1.000000000000000000, 0.9330127018922189652, 0.9330127018922192983 ) ) 
 REPRESENTATION_ITEM ( '' )  );
#16502=CARTESIAN_POINT ( 'NONE',  ( 5.000000000000000000, -22.41666666666666785, -2.886751345948130876 ) ) ;
#16503=EDGE_CURVE ( 'NONE', #13218, #11760, #55642, .T. ) ;
#16505=CARTESIAN_POINT ( 'NONE',  ( 1.846868145590736310, -161.8750000013656063, 4.458734124999997661 ) ) ;
#16508=CARTESIAN_POINT ( 'NONE',  ( 4.458734124999999437, -139.5000000013655779, 1.846868145590737864 ) ) ;
#16509=ORIENTED_EDGE ( 'NONE', *, *, #36121, .T. ) ;
#16510=CARTESIAN_POINT ( 'NONE',  ( -3.152548672688508926E-16, 23.18750000136559208, -5.148502694627439702 ) ) ;
#16515=CARTESIAN_POINT ( 'NONE',  ( -2.499999999999996447, -2.708333330602146649, 4.330127018922195425 ) ) ;
#16516=CARTESIAN_POINT ( 'NONE',  ( 2.500000000000002220, 7.333333333333333925, 4.330127018922192761 ) ) ;
#16517=CARTESIAN_POINT ( 'NONE',  ( -4.458734124999997661, -57.22916666530107932, 2.574251347313722516 ) ) ;
#16518=CARTESIAN_POINT ( 'NONE',  ( 2.229367062499998831, -12.64583333196774007, -3.861377020970580887 ) ) ;
#16521=CARTESIAN_POINT ( 'NONE',  ( -5.000000000000000000, -63.87499999726880873, 0.000000000000000000 ) ) ;
#16522=CARTESIAN_POINT ( 'NONE',  ( -5.000000000000000000, -37.00000000000000711, 0.000000000000000000 ) ) ;
#16524=CARTESIAN_POINT ( 'NONE',  ( -5.000000000000000000, -34.08333333333332860, -2.886751345948128211 ) ) ;
#16528=CARTESIAN_POINT ( 'NONE',  ( -2.229367062500000163, -59.47916666530106511, -3.861377020970580443 ) ) ;
#16529=CARTESIAN_POINT ( 'NONE',  ( 3.152801135295366208, -151.8125000013655779, 3.152801135295367985 ) ) ;
#16530=AXIS2_PLACEMENT_3D ( 'NONE', #55758, #59959, #35822 ) ;
#16531=EDGE_CURVE ( 'NONE', #34465, #9066, #60146, .T. ) ;
#16532=CARTESIAN_POINT ( 'NONE',  ( 2.229367062500001939, -73.97916666530106511, 3.861377020970579999 ) ) ;
#16534=CARTESIAN_POINT ( 'NONE',  ( -2.229367062499996610, -21.39583333196774007, 3.861377020970582219 ) ) ;
#16535=CARTESIAN_POINT ( 'NONE',  ( 2.500000000000002220, -61.54166666393547303, 4.330127018922192761 ) ) ;
#16536=ORIENTED_EDGE ( 'NONE', *, *, #31543, .F. ) ;
#16541=CARTESIAN_POINT ( 'NONE',  ( 4.458734124999999437, -154.5000000013656347, 1.846868145590737864 ) ) ;
#16543=CARTESIAN_POINT ( 'NONE',  ( 1.339745962155615144, -54.70534180126148271, 4.999999999999999112 ) ) ;
#16546=CARTESIAN_POINT ( 'NONE',  ( 4.458734124999998549, -45.97916666530106511, -2.574251347313721627 ) ) ;
#16548=CARTESIAN_POINT ( 'NONE',  ( -2.071067811865562991, -145.3124999999999716, 4.999999999999913847 ) ) ;
#16550=( BOUNDED_CURVE ( )  B_SPLINE_CURVE ( 2, ( #15027, #569, #5703, #40737, #44609, #39776, #54909, #30779, #55235 ),
 .UNSPECIFIED., .F., .F. ) 
 B_SPLINE_CURVE_WITH_KNOTS ( ( 3, 2, 2, 2, 3 ),
 ( 0.4437499999999999778, 0.4444444444444444198, 0.4458333333333333592, 0.4472222222222222432, 0.4479166666666666852 ),
 .UNSPECIFIED. ) 
 CURVE ( )  GEOMETRIC_REPRESENTATION_ITEM ( )  RATIONAL_B_SPLINE_CURVE ( ( 0.9330127018922194093, 0.9330127018922194093, 1.000000000000000000, 0.8660254037844387076, 1.000000000000000000, 0.8660254037844387076, 1.000000000000000000, 0.9330127018922194093, 0.9330127018922194093 ) ) 
 REPRESENTATION_ITEM ( '' )  );
#16551=CARTESIAN_POINT ( 'NONE',  ( -2.229367062500000163, 23.52083333469892779, -3.861377020970580443 ) ) ;
#16553=CARTESIAN_POINT ( 'NONE',  ( 1.975475456537005874E-15, -13.62499999726881228, 5.000000000000000000 ) ) ;
#16555=ORIENTED_EDGE ( 'NONE', *, *, #36817, .T. ) ;
#16557=CARTESIAN_POINT ( 'NONE',  ( 1.339745962155615144, -28.58034179853029144, 4.999999999999999112 ) ) ;
#16561=CARTESIAN_POINT ( 'NONE',  ( -2.500000000000000444, -2.041666663935480575, -4.330127018922193649 ) ) ;
#16565=CARTESIAN_POINT ( 'NONE',  ( -1.339745962155613812, -20.08034179853029144, -5.000000000000000000 ) ) ;
#16566=EDGE_CURVE ( 'NONE', #42874, #44687, #46991, .T. ) ;
#16567=CARTESIAN_POINT ( 'NONE',  ( 1.975475456537005874E-15, 9.375000002731185944, 5.000000000000000000 ) ) ;
#16570=LINE ( 'NONE', #41954, #58707 ) ;
#16572=CARTESIAN_POINT ( 'NONE',  ( 3.061616997868383141E-16, -157.8750000027311842, -5.000000000000000000 ) ) ;
#16573=ORIENTED_EDGE ( 'NONE', *, *, #49454, .T. ) ;
#16575=AXIS2_PLACEMENT_3D ( 'NONE', #18345, #56014, #31558 ) ;
#16578=EDGE_CURVE ( 'NONE', #50806, #13144, #42325, .T. ) ;
#16582=EDGE_CURVE ( 'NONE', #1775, #6968, #23668, .T. ) ;
#16584=CARTESIAN_POINT ( 'NONE',  ( 9.457646018065525792E-16, -23.06249999863440792, 5.148502694627439702 ) ) ;
#16586=CARTESIAN_POINT ( 'NONE',  ( -3.535533905932738641, -151.3750000000000000, 3.535533905932737309 ) ) ;
#16588=CARTESIAN_POINT ( 'NONE',  ( -4.458734124999999437, -149.9375000013656063, -5.460374474430324690E-16 ) ) ;
#16590=CARTESIAN_POINT ( 'NONE',  ( -4.458734124999999437, -50.56249999863440792, 0.000000000000000000 ) ) ;
#16591=CARTESIAN_POINT ( 'NONE',  ( 6.972266317189433020E-16, 29.74999999999999645, -5.000000000000000000 ) ) ;
#16594=CARTESIAN_POINT ( 'NONE',  ( -5.000000000000000000, 28.91666666666666430, -2.886751345948128211 ) ) ;
#16596=CARTESIAN_POINT ( 'NONE',  ( -4.458734124999998549, 1.770833334698927786, 2.574251347313722516 ) ) ;
#16598=CARTESIAN_POINT ( 'NONE',  ( 5.000000000000000888, 13.41666666666666785, 2.886751345948126879 ) ) ;
#16599=CARTESIAN_POINT ( 'NONE',  ( 5.000000000000000000, -17.50000000000000000, -6.123233995736766282E-16 ) ) ;
#16600=CARTESIAN_POINT ( 'NONE',  ( 2.229367062499998831, 17.10416666803225993, -3.861377020970580887 ) ) ;
#16601=CARTESIAN_POINT ( 'NONE',  ( -5.000000000000000000, 3.125000002731185944, 0.000000000000000000 ) ) ;
#16602=ORIENTED_EDGE ( 'NONE', *, *, #2169, .F. ) ;
#16604=ORIENTED_EDGE ( 'NONE', *, *, #46256, .T. ) ;
#16605=( BOUNDED_CURVE ( )  B_SPLINE_CURVE ( 2, ( #21960, #51241, #7487, #6533, #60887, #21648, #27100, #30649, #50271 ),
 .UNSPECIFIED., .F., .F. ) 
 B_SPLINE_CURVE_WITH_KNOTS ( ( 3, 2, 2, 2, 3 ),
 ( 0.5187500000000000444, 0.5194444444444444864, 0.5208333333333333703, 0.5222222222222222543, 0.5229166666666666963 ),
 .UNSPECIFIED. ) 
 CURVE ( )  GEOMETRIC_REPRESENTATION_ITEM ( )  RATIONAL_B_SPLINE_CURVE ( ( 0.9330127018922194093, 0.9330127018922194093, 1.000000000000000000, 0.8660254037844387076, 1.000000000000000000, 0.8660254037844387076, 1.000000000000000000, 0.9330127018922194093, 0.9330127018922194093 ) ) 
 REPRESENTATION_ITEM ( '' )  );
#16606=CARTESIAN_POINT ( 'NONE',  ( -2.229367062499996610, -46.14583333196774362, 3.861377020970582219 ) ) ;
#16607=CARTESIAN_POINT ( 'NONE',  ( 4.458734124999999437, -164.6875000013655779, 0.000000000000000000 ) ) ;
#16608=CARTESIAN_POINT ( 'NONE',  ( 5.000000000000000000, -46.37499999726880873, -6.123233995736766282E-16 ) ) ;
#16609=ORIENTED_EDGE ( 'NONE', *, *, #24363, .F. ) ;
#16610=CARTESIAN_POINT ( 'NONE',  ( -3.152548672688508926E-16, -18.56249999863440792, -5.148502694627439702 ) ) ;
#16612=CARTESIAN_POINT ( 'NONE',  ( 1.060575238724906964E-15, -87.75000000000000000, 5.773502691896257311 ) ) ;
#16613=CARTESIAN_POINT ( 'NONE',  ( 1.846868145590735200, -164.2500000013656063, -4.458734125000000326 ) ) ;
#16617=CARTESIAN_POINT ( 'NONE',  ( 2.229367062500001939, -33.22916666530106511, 3.861377020970579999 ) ) ;
#16624=CARTESIAN_POINT ( 'NONE',  ( -3.535533905932738641, -161.3750000000000284, 3.535533905932737309 ) ) ;
#16626=VECTOR ( 'NONE', #10358, 1000.000000000000000 ) ;
#16627=CARTESIAN_POINT ( 'NONE',  ( 4.458734124999998549, -80.97916666530106511, -2.574251347313721627 ) ) ;
#16629=CARTESIAN_POINT ( 'NONE',  ( 2.500000000000002220, 22.33333333333333215, 4.330127018922192761 ) ) ;
#16630=CARTESIAN_POINT ( 'NONE',  ( 4.458734124999999437, -142.6875000013656063, 0.000000000000000000 ) ) ;
#16633=CARTESIAN_POINT ( 'NONE',  ( -4.458734124999997661, -46.22916666530106511, 2.574251347313722516 ) ) ;
#16636=FACE_OUTER_BOUND ( 'NONE', #55952, .T. ) ;
#16637=ADVANCED_FACE ( 'NONE', ( #29093 ), #43265, .T. ) ;
#16640=CARTESIAN_POINT ( 'NONE',  ( 2.499999999999998668, 16.79166666939785202, -4.330127018922193649 ) ) ;
#16642=CARTESIAN_POINT ( 'NONE',  ( -3.152548672688508926E-16, -80.81249999863440792, -5.148502694627439702 ) ) ;
#16643=CARTESIAN_POINT ( 'NONE',  ( 1.339745962155615144, -34.70534180126148271, 4.999999999999999112 ) ) ;
#16646=ORIENTED_EDGE ( 'NONE', *, *, #46409, .F. ) ;
#16648=CARTESIAN_POINT ( 'NONE',  ( -5.000000000000000000, -14.87499999726881228, 0.000000000000000000 ) ) ;
#16652=CARTESIAN_POINT ( 'NONE',  ( -2.229367062500000163, 11.27083333469892601, -3.861377020970580443 ) ) ;
#16653=CARTESIAN_POINT ( 'NONE',  ( -6.972266317189433020E-16, -39.25000000000000000, -5.000000000000000000 ) ) ;
#16658=CARTESIAN_POINT ( 'NONE',  ( 1.975475456537005874E-15, -38.62499999726880873, 5.000000000000000000 ) ) ;
#16659=CARTESIAN_POINT ( 'NONE',  ( 4.458734124999998549, -84.72916666530106511, -2.574251347313721627 ) ) ;
#16660=CARTESIAN_POINT ( 'NONE',  ( -2.229367062500000163, -2.479166665301069106, -3.861377020970580443 ) ) ;
#16665=CARTESIAN_POINT ( 'NONE',  ( 2.229367062499998831, -32.89583333196773651, -3.861377020970580887 ) ) ;
#16667=EDGE_CURVE ( 'NONE', #53830, #52296, #51506, .T. ) ;
#16670=CARTESIAN_POINT ( 'NONE',  ( -2.229367062499996610, 18.85416666803225993, 3.861377020970582219 ) ) ;
#16673=CARTESIAN_POINT ( 'NONE',  ( -5.000000000000000888, -145.5625000027311842, 2.071067811865474617 ) ) ;
#16674=CARTESIAN_POINT ( 'NONE',  ( -3.152548672688508926E-16, -78.81249999863442213, -5.148502694627439702 ) ) ;
#16677=CARTESIAN_POINT ( 'NONE',  ( -5.000000000000000000, 18.04166666939785557, -2.886751345948128211 ) ) ;
#16680=CARTESIAN_POINT ( 'NONE',  ( -5.000000000000000000, -168.6250000027312126, -6.123233995736766282E-16 ) ) ;
#16682=CARTESIAN_POINT ( 'NONE',  ( -2.500000000000000444, -23.16666666666666785, -4.330127018922193649 ) ) ;
#16683=CARTESIAN_POINT ( 'NONE',  ( 2.229367062499998831, -29.64583333196773296, -3.861377020970580887 ) ) ;
#16686=( BOUNDED_CURVE ( )  B_SPLINE_CURVE ( 2, ( #53312, #9246, #28860, #15343, #10828, #29799, #5375, #53937, #59734 ),
 .UNSPECIFIED., .F., .F. ) 
 B_SPLINE_CURVE_WITH_KNOTS ( ( 3, 2, 2, 2, 3 ),
 ( 0.5145833333333332815, 0.5152777777777777235, 0.5166666666666667185, 0.5180555555555556024, 0.5187500000000000444 ),
 .UNSPECIFIED. ) 
 CURVE ( )  GEOMETRIC_REPRESENTATION_ITEM ( )  RATIONAL_B_SPLINE_CURVE ( ( 0.9330127018922194093, 0.9330127018922194093, 1.000000000000000000, 0.8660254037844387076, 1.000000000000000000, 0.8660254037844387076, 1.000000000000000000, 0.9330127018922194093, 0.9330127018922194093 ) ) 
 REPRESENTATION_ITEM ( '' )  );
#16687=CARTESIAN_POINT ( 'NONE',  ( 1.060575238724906964E-15, -25.62499999726881583, 5.773502691896257311 ) ) ;
#16688=CARTESIAN_POINT ( 'NONE',  ( -4.458734124999999437, -57.31249999863440081, 0.000000000000000000 ) ) ;
#16689=VERTEX_POINT ( 'NONE', #63533 ) ;
#16690=DIRECTION ( 'NONE',  ( -0.000000000000000000, 1.000000000000000000, -0.000000000000000000 ) ) ;
#16691=CARTESIAN_POINT ( 'NONE',  ( 6.123233995736766282E-16, -170.0000000000000000, -5.000000000000000000 ) ) ;
#16692=CARTESIAN_POINT ( 'NONE',  ( 2.229367062500001939, -3.229166665301069550, 3.861377020970579999 ) ) ;
#16694=CARTESIAN_POINT ( 'NONE',  ( 2.499999999999998668, -72.33333333333332860, -4.330127018922193649 ) ) ;
#16698=CARTESIAN_POINT ( 'NONE',  ( 5.000000000000000000, -159.0625000000000284, 2.071067811865478614 ) ) ;
#16699=CARTESIAN_POINT ( 'NONE',  ( -5.000000000000000000, -72.87499999726880162, 0.000000000000000000 ) ) ;
#16700=CARTESIAN_POINT ( 'NONE',  ( 2.499999999999998668, -10.20833333060214621, -4.330127018922193649 ) ) ;
#16702=CARTESIAN_POINT ( 'NONE',  ( -3.152548672688508926E-16, -17.81249999863440792, -5.148502694627439702 ) ) ;
#16703=CARTESIAN_POINT ( 'NONE',  ( 4.458734124999999437, -53.06249999863440792, -5.460374474430324690E-16 ) ) ;
#16705=CARTESIAN_POINT ( 'NONE',  ( 5.000000000000000000, 10.49999999999999822, -6.123233995736766282E-16 ) ) ;
#16707=CARTESIAN_POINT ( 'NONE',  ( 3.152801135295366208, -142.5625000013655779, 3.152801135295367985 ) ) ;
#16709=CARTESIAN_POINT ( 'NONE',  ( 1.339745962155612702, -8.169658196007333117, -5.000000000000000000 ) ) ;
#16711=CARTESIAN_POINT ( 'NONE',  ( -4.458734124999999437, 24.43750000136559208, 0.000000000000000000 ) ) ;
#16715=EDGE_CURVE ( 'NONE', #54593, #2442, #34239, .T. ) ;
#16716=CARTESIAN_POINT ( 'NONE',  ( -8.190561711645485556E-16, -148.9375000013656063, 4.458734124999999437 ) ) ;
#16718=CARTESIAN_POINT ( 'NONE',  ( -4.458734124999998549, -65.47916666530107932, 2.574251347313722516 ) ) ;
#16720=CARTESIAN_POINT ( 'NONE',  ( -4.458734124999999437, -7.312499998634404363, 0.000000000000000000 ) ) ;
#16722=CARTESIAN_POINT ( 'NONE',  ( 3.152801135295367541, -146.3125000013655779, -3.152801135295367541 ) ) ;
#16724=ORIENTED_EDGE ( 'NONE', *, *, #51239, .T. ) ;
#16725=CARTESIAN_POINT ( 'NONE',  ( -2.500000000000000444, -63.04166666393547303, -4.330127018922193649 ) ) ;
#16735=CYLINDRICAL_SURFACE ( 'NONE', #24278, 5.000000000000000000 ) ;
#16736=CARTESIAN_POINT ( 'NONE',  ( 2.499999999999998668, -60.20833333060214443, -4.330127018922193649 ) ) ;
#16737=CARTESIAN_POINT ( 'NONE',  ( 2.229367062499998831, 14.35416666803226171, -3.861377020970580887 ) ) ;
#16739=CARTESIAN_POINT ( 'NONE',  ( 4.458734125000000326, -13.14583333196774184, 2.574251347313718519 ) ) ;
#16741=CARTESIAN_POINT ( 'NONE',  ( -1.846868145590734756, -165.1250000013656063, -4.458734125000000326 ) ) ;
#16746=CARTESIAN_POINT ( 'NONE',  ( 3.535533905932736864, -139.2500000027311842, 3.535533905932738641 ) ) ;
#16747=CARTESIAN_POINT ( 'NONE',  ( 4.458734125000000326, -35.89583333196773651, 2.574251347313718519 ) ) ;
#16748=CARTESIAN_POINT ( 'NONE',  ( 2.499999999999998668, -51.20833333060213732, -4.330127018922193649 ) ) ;
#16752=EDGE_LOOP ( 'NONE', ( #46278, #23428, #35696, #51316 ) ) ;
#16756=CARTESIAN_POINT ( 'NONE',  ( 5.000000000000000000, -89.37499999726880162, -6.123233995736766282E-16 ) ) ;
#16757=CARTESIAN_POINT ( 'NONE',  ( 5.000000000000000888, -9.583333333333333925, 2.886751345948126879 ) ) ;
#16758=CARTESIAN_POINT ( 'NONE',  ( 4.458734125000000326, -71.89583333196773651, 2.574251347313718519 ) ) ;
#16759=CARTESIAN_POINT ( 'NONE',  ( -6.972266317189433020E-16, -22.12499999726881228, -5.000000000000000000 ) ) ;
#16760=CARTESIAN_POINT ( 'NONE',  ( -2.500000000000000444, -10.04166666393547658, -4.330127018922193649 ) ) ;
#16761=CARTESIAN_POINT ( 'NONE',  ( 4.458734125000001214, -36.89583333196773651, 2.574251347313718519 ) ) ;
#16762=VERTEX_POINT ( 'NONE', #50567 ) ;
#16764=CARTESIAN_POINT ( 'NONE',  ( 4.458734124999998549, 12.02083333469892601, -2.574251347313721627 ) ) ;
#16767=CARTESIAN_POINT ( 'NONE',  ( 5.000000000000000000, -56.41666666666666430, -2.886751345948129988 ) ) ;
#16770=CARTESIAN_POINT ( 'NONE',  ( 4.458734124999998549, -73.72916666530106511, -2.574251347313721627 ) ) ;
#16771=CARTESIAN_POINT ( 'NONE',  ( -2.071067811865475061, -168.6875000000000568, -5.000000000000000888 ) ) ;
#16772=CARTESIAN_POINT ( 'NONE',  ( -2.229367062499996610, -88.14583333196773651, 3.861377020970582219 ) ) ;
#16775=CARTESIAN_POINT ( 'NONE',  ( 4.458734124999999437, -34.06249999863440792, -5.460374474430324690E-16 ) ) ;
#16780=ORIENTED_EDGE ( 'NONE', *, *, #59026, .T. ) ;
#16781=CARTESIAN_POINT ( 'NONE',  ( -5.000000000000000000, -3.958333330602147537, -2.886751345948128211 ) ) ;
#16782=( BOUNDED_CURVE ( )  B_SPLINE_CURVE ( 2, ( #42302, #52283, #47448, #56484, #3400, #23016, #32976, #37805, #27200 ),
 .UNSPECIFIED., .F., .F. ) 
 B_SPLINE_CURVE_WITH_KNOTS ( ( 3, 2, 2, 2, 3 ),
 ( 0.1750000000000001554, 0.1791666666666668351, 0.1833333333333334869, 0.1875000000000001665, 0.1916666666666668462 ),
 .UNSPECIFIED. ) 
 CURVE ( )  GEOMETRIC_REPRESENTATION_ITEM ( )  RATIONAL_B_SPLINE_CURVE ( ( 0.9999999999999970024, 0.9238795325112897361, 1.000000000000000000, 0.9238795325112867385, 1.000000000000000000, 0.9238795325112867385, 1.000000000000000000, 0.9238795325112837409, 1.000000000000003109 ) ) 
 REPRESENTATION_ITEM ( '' )  );
#16784=CARTESIAN_POINT ( 'NONE',  ( 4.458734124999998549, -61.97916666530106511, -2.574251347313721627 ) ) ;
#16786=ORIENTED_EDGE ( 'NONE', *, *, #25113, .T. ) ;
#16792=CARTESIAN_POINT ( 'NONE',  ( -4.458734124999999437, 7.687500001365594748, 0.000000000000000000 ) ) ;
#16793=CARTESIAN_POINT ( 'NONE',  ( -1.339745962155613812, -76.20534180126146850, -5.000000000000000000 ) ) ;
#16794=CARTESIAN_POINT ( 'NONE',  ( 3.152801135295366208, -157.5625000013656063, 3.152801135295367985 ) ) ;
#16795=DIRECTION ( 'NONE',  ( 0.000000000000000000, 0.000000000000000000, 1.000000000000000000 ) ) ;
#16800=CARTESIAN_POINT ( 'NONE',  ( 1.975475456537005874E-15, -71.62499999726878741, 5.000000000000000000 ) ) ;
#16805=CARTESIAN_POINT ( 'NONE',  ( 2.229367062499998831, 29.35416666803225993, -3.861377020970580887 ) ) ;
#16808=CARTESIAN_POINT ( 'NONE',  ( 2.229367062500001939, 0.7708333346989268975, 3.861377020970579999 ) ) ;
#16810=CARTESIAN_POINT ( 'NONE',  ( -2.071067811865478170, -145.4375000027312694, 5.000000000000000000 ) ) ;
#16815=VECTOR ( 'NONE', #41849, 1000.000000000000000 ) ;
#16817=CARTESIAN_POINT ( 'NONE',  ( 1.975475456537005874E-15, 18.24999999999999645, 5.000000000000000000 ) ) ;
#16819=CARTESIAN_POINT ( 'NONE',  ( -4.458734125000000326, -160.1250000013655779, 1.846868145590734089 ) ) ;
#16822=CARTESIAN_POINT ( 'NONE',  ( -4.458734124999999437, -140.9375000013656063, -5.460374474430324690E-16 ) ) ;
#16824=CARTESIAN_POINT ( 'NONE',  ( -4.458734124999998549, 21.52083333469893134, 2.574251347313722516 ) ) ;
#16830=CARTESIAN_POINT ( 'NONE',  ( -3.535250795749689387E-16, 10.74999999999999822, -5.773502691896257311 ) ) ;
#16831=CARTESIAN_POINT ( 'NONE',  ( 9.457646018065525792E-16, -55.06249999863440081, 5.148502694627439702 ) ) ;
#16832=CARTESIAN_POINT ( 'NONE',  ( 4.458734125000001214, -12.89583333196774184, 2.574251347313718519 ) ) ;
#16835=CARTESIAN_POINT ( 'NONE',  ( -2.499999999999996447, -63.70833333060215153, 4.330127018922195425 ) ) ;
#16838=CARTESIAN_POINT ( 'NONE',  ( -3.535250795749689387E-16, -38.24999999999999289, -5.773502691896257311 ) ) ;
#16839=CARTESIAN_POINT ( 'NONE',  ( -1.339745962155610925, 13.33034180399266688, 5.000000000000000000 ) ) ;
#16842=CARTESIAN_POINT ( 'NONE',  ( 4.458734124999999437, -61.81249999863440081, -5.460374474430324690E-16 ) ) ;
#16843=CARTESIAN_POINT ( 'NONE',  ( 3.152801135295367541, -153.5625000013656063, -3.152801135295367541 ) ) ;
#16844=CARTESIAN_POINT ( 'NONE',  ( 2.229367062499998831, -72.64583333196773651, -3.861377020970580887 ) ) ;
#16847=CARTESIAN_POINT ( 'NONE',  ( 9.457646018065525792E-16, -17.31249999863440436, 5.148502694627439702 ) ) ;
#16848=CARTESIAN_POINT ( 'NONE',  ( 1.060575238724906964E-15, -60.62499999726880873, 5.773502691896257311 ) ) ;
#16854=CARTESIAN_POINT ( 'NONE',  ( 3.152801135295366208, -150.5625000013655779, 3.152801135295367985 ) ) ;
#16855=EDGE_LOOP ( 'NONE', ( #63589, #21899, #55408, #54991 ) ) ;
#16859=CARTESIAN_POINT ( 'NONE',  ( -4.458734124999999437, -49.64583333196772941, -2.574251347313719407 ) ) ;
#16860=ORIENTED_EDGE ( 'NONE', *, *, #16715, .T. ) ;
#16861=AXIS2_PLACEMENT_3D ( 'NONE', #60793, #7713, #51142 ) ;
#16863=CARTESIAN_POINT ( 'NONE',  ( -2.499999999999996447, 17.29166666939785557, 4.330127018922195425 ) ) ;
#16867=CARTESIAN_POINT ( 'NONE',  ( -4.458734124999999437, 22.68750000136559564, 0.000000000000000000 ) ) ;
#16870=ORIENTED_EDGE ( 'NONE', *, *, #16578, .F. ) ;
#16872=CARTESIAN_POINT ( 'NONE',  ( 5.000000000000000888, -28.45833333060214443, 2.886751345948126879 ) ) ;
#16874=EDGE_CURVE ( 'NONE', #59810, #41033, #44533, .T. ) ;
#16875=( BOUNDED_CURVE ( )  B_SPLINE_CURVE ( 2, ( #55152, #40342, #6268, #60302, #59662, #16231, #26193, #35528, #49357 ),
 .UNSPECIFIED., .F., .F. ) 
 B_SPLINE_CURVE_WITH_KNOTS ( ( 3, 2, 2, 2, 3 ),
 ( 0.9104166666666666519, 0.9111111111111110938, 0.9124999999999999778, 0.9138888888888888618, 0.9145833333333333037 ),
 .UNSPECIFIED. ) 
 CURVE ( )  GEOMETRIC_REPRESENTATION_ITEM ( )  RATIONAL_B_SPLINE_CURVE ( ( 0.9330127018922194093, 0.9330127018922194093, 1.000000000000000000, 0.8660254037844387076, 1.000000000000000000, 0.8660254037844387076, 1.000000000000000000, 0.9330127018922194093, 0.9330127018922194093 ) ) 
 REPRESENTATION_ITEM ( '' )  );
#16881=LINE ( 'NONE', #22351, #8001 ) ;
#16882=CARTESIAN_POINT ( 'NONE',  ( 6.123233995736766282E-16, -170.0000000000000000, -5.000000000000000000 ) ) ;
#16885=CARTESIAN_POINT ( 'NONE',  ( 1.975475456537005874E-15, -4.624999997268815832, 5.000000000000000000 ) ) ;
#16887=CARTESIAN_POINT ( 'NONE',  ( -2.071067811865475061, -156.8125000027311842, -5.000000000000000888 ) ) ;
#16893=CARTESIAN_POINT ( 'NONE',  ( -5.000000000000000000, -148.5000000000000284, -6.123233995736766282E-16 ) ) ;
#16894=EDGE_CURVE ( 'NONE', #29389, #31402, #3039, .T. ) ;
#16897=CARTESIAN_POINT ( 'NONE',  ( -5.000000000000000000, -90.00000000000000000, 0.000000000000000000 ) ) ;
#16898=CARTESIAN_POINT ( 'NONE',  ( 4.458734124999999437, -22.81249999863440436, -5.460374474430324690E-16 ) ) ;
#16900=CARTESIAN_POINT ( 'NONE',  ( 5.000000000000000000, -152.0625000000000284, 2.071067811865478614 ) ) ;
#16902=CARTESIAN_POINT ( 'NONE',  ( 2.730187237215162345E-16, -151.1875000013656063, -4.458734124999999437 ) ) ;
#16903=ORIENTED_EDGE ( 'NONE', *, *, #7853, .F. ) ;
#16904=CARTESIAN_POINT ( 'NONE',  ( 4.458734125000000326, -52.14583333196773651, 2.574251347313718519 ) ) ;
#16906=CARTESIAN_POINT ( 'NONE',  ( 5.000000000000000888, 24.41666666666666785, 2.886751345948126879 ) ) ;
#16909=CARTESIAN_POINT ( 'NONE',  ( 2.229367062500001939, 5.020833334698926897, 3.861377020970579999 ) ) ;
#16910=FACE_OUTER_BOUND ( 'NONE', #44839, .T. ) ;
#16911=CARTESIAN_POINT ( 'NONE',  ( 1.339745962155612702, 13.70534180126148094, -5.000000000000000000 ) ) ;
#16912=LINE ( 'NONE', #42303, #38597 ) ;
#16913=CARTESIAN_POINT ( 'NONE',  ( 4.458734124999999437, 16.93750000136559564, -5.460374474430324690E-16 ) ) ;
#16914=CARTESIAN_POINT ( 'NONE',  ( 5.000000000000000000, 5.708333336064518981, -2.886751345948129988 ) ) ;
#16916=CARTESIAN_POINT ( 'NONE',  ( 5.000000000000000000, 26.58333333333333215, -2.886751345948130876 ) ) ;
#16919=CARTESIAN_POINT ( 'NONE',  ( -4.458734124999999437, -41.31249999863440081, 0.000000000000000000 ) ) ;
#16920=CARTESIAN_POINT ( 'NONE',  ( -1.846868145590737420, -165.0000000013655779, 4.458734124999999437 ) ) ;
#16921=EDGE_CURVE ( 'NONE', #56964, #33079, #7919, .T. ) ;
#16922=EDGE_CURVE ( 'NONE', #51005, #44335, #58054, .T. ) ;
#16923=CARTESIAN_POINT ( 'NONE',  ( 5.000000000000000000, -43.37499999726880873, -6.123233995736766282E-16 ) ) ;
#16924=EDGE_CURVE ( 'NONE', #11571, #41628, #42488, .T. ) ;
#16925=ORIENTED_EDGE ( 'NONE', *, *, #13075, .T. ) ;
#16926=CARTESIAN_POINT ( 'NONE',  ( 4.458734124999999437, -18.81249999863440792, -5.460374474430324690E-16 ) ) ;
#16927=ORIENTED_EDGE ( 'NONE', *, *, #7588, .F. ) ;
#16928=( BOUNDED_CURVE ( )  B_SPLINE_CURVE ( 2, ( #33152, #52766, #19603, #57292, #8394, #47615, #38897, #27995, #3568 ),
 .UNSPECIFIED., .F., .F. ) 
 B_SPLINE_CURVE_WITH_KNOTS ( ( 3, 2, 2, 2, 3 ),
 ( 0.3687500000000000222, 0.3694444444444444642, 0.3708333333333333481, 0.3722222222222222321, 0.3729166666666666741 ),
 .UNSPECIFIED. ) 
 CURVE ( )  GEOMETRIC_REPRESENTATION_ITEM ( )  RATIONAL_B_SPLINE_CURVE ( ( 0.9330127018922194093, 0.9330127018922194093, 1.000000000000000000, 0.8660254037844387076, 1.000000000000000000, 0.8660254037844387076, 1.000000000000000000, 0.9330127018922194093, 0.9330127018922194093 ) ) 
 REPRESENTATION_ITEM ( '' )  );
#16929=CARTESIAN_POINT ( 'NONE',  ( 1.060575238724906964E-15, -89.74999999999998579, 5.773502691896257311 ) ) ;
#16930=CARTESIAN_POINT ( 'NONE',  ( 4.458734124999999437, -166.5000000013655779, 1.846868145590737864 ) ) ;
#16932=CARTESIAN_POINT ( 'NONE',  ( -5.000000000000000000, -18.99999999999999645, 0.000000000000000000 ) ) ;
#16935=CARTESIAN_POINT ( 'NONE',  ( 4.458734124999998549, -33.97916666530107221, -2.574251347313721627 ) ) ;
#16937=EDGE_CURVE ( 'NONE', #41952, #33720, #33820, .T. ) ;
#16938=EDGE_LOOP ( 'NONE', ( #45880, #35452, #23660, #9410 ) ) ;
#16940=EDGE_CURVE ( 'NONE', #35906, #35595, #12281, .T. ) ;
#16943=ORIENTED_EDGE ( 'NONE', *, *, #41756, .T. ) ;
#16946=CARTESIAN_POINT ( 'NONE',  ( 9.457646018065525792E-16, -80.31249999863440792, 5.148502694627439702 ) ) ;
#16949=CARTESIAN_POINT ( 'NONE',  ( 2.730187237215162345E-16, -141.4375000013656063, -4.458734124999999437 ) ) ;
#16950=CARTESIAN_POINT ( 'NONE',  ( -5.000000000000000000, 6.125000002731185056, 0.000000000000000000 ) ) ;
#16952=CARTESIAN_POINT ( 'NONE',  ( -2.229367062500000163, -43.47916666530106511, -3.861377020970580443 ) ) ;
#16956=CARTESIAN_POINT ( 'NONE',  ( -5.000000000000000000, 3.916666666666665630, -2.886751345948128211 ) ) ;
#16960=CARTESIAN_POINT ( 'NONE',  ( -2.499999999999996447, -45.70833333060214443, 4.330127018922195425 ) ) ;
#16962=CARTESIAN_POINT ( 'NONE',  ( 4.458734125000001214, -78.14583333196775072, 2.574251347313718519 ) ) ;
#16970=CARTESIAN_POINT ( 'NONE',  ( -1.339745962155613812, -5.205341801261476498, -5.000000000000000000 ) ) ;
#16972=CARTESIAN_POINT ( 'NONE',  ( -2.229367062499996610, 11.60416666803225993, 3.861377020970582219 ) ) ;
#16973=CARTESIAN_POINT ( 'NONE',  ( -2.499999999999996447, -29.83333333333332860, 4.330127018922195425 ) ) ;
#16979=CARTESIAN_POINT ( 'NONE',  ( -3.152548672688508926E-16, -83.56249999863440792, -5.148502694627439702 ) ) ;
#16980=CARTESIAN_POINT ( 'NONE',  ( 4.458734125000000326, -6.895833331967734736, 2.574251347313718519 ) ) ;
#16982=CARTESIAN_POINT ( 'NONE',  ( 2.229367062500001939, -38.22916666530107221, 3.861377020970579999 ) ) ;
#16987=CARTESIAN_POINT ( 'NONE',  ( -4.458734124999999437, -150.2500000013656347, -1.846868145590735644 ) ) ;
#16988=CARTESIAN_POINT ( 'NONE',  ( -4.458734124999999437, 18.68750000136559564, 0.000000000000000000 ) ) ;
#16990=CARTESIAN_POINT ( 'NONE',  ( 5.000000000000000000, -66.50000000000000000, -6.123233995736766282E-16 ) ) ;
#16991=CARTESIAN_POINT ( 'NONE',  ( 9.457646018065525792E-16, -82.31249999863440792, 5.148502694627439702 ) ) ;
#16994=CARTESIAN_POINT ( 'NONE',  ( 2.500000000000002220, 17.45833333606451987, 4.330127018922192761 ) ) ;
#16998=CARTESIAN_POINT ( 'NONE',  ( 5.000000000000000888, -0.5833333333333350357, 2.886751345948126879 ) ) ;
#16999=CARTESIAN_POINT ( 'NONE',  ( 5.000000000000000888, -24.58333333333333215, 2.886751345948126879 ) ) ;
#17000=CARTESIAN_POINT ( 'NONE',  ( -4.458734124999998549, -29.22916666530107221, 2.574251347313722516 ) ) ;
#17001=CARTESIAN_POINT ( 'NONE',  ( 4.458734125000000326, -89.89583333196773651, 2.574251347313718519 ) ) ;
#17002=ADVANCED_FACE ( 'NONE', ( #46690 ), #8411, .T. ) ;
#17003=CARTESIAN_POINT ( 'NONE',  ( -4.999999999999999112, -27.79166666393547658, 2.886751345948131764 ) ) ;
#17004=CARTESIAN_POINT ( 'NONE',  ( -4.458734124999999437, -53.39583333196773651, -2.574251347313719407 ) ) ;
#17007=CARTESIAN_POINT ( 'NONE',  ( 4.458734125000001214, -3.145833331967738733, 2.574251347313718519 ) ) ;
#17009=CARTESIAN_POINT ( 'NONE',  ( 2.500000000000002220, -72.66666666666667140, 4.330127018922192761 ) ) ;
#17014=CARTESIAN_POINT ( 'NONE',  ( -3.535250795749689387E-16, -70.12499999726880162, -5.773502691896257311 ) ) ;
#17015=CARTESIAN_POINT ( 'NONE',  ( -2.499999999999996447, -85.83333333333332860, 4.330127018922195425 ) ) ;
#17018=CARTESIAN_POINT ( 'NONE',  ( 9.457646018065525792E-16, -16.31249999863440436, 5.148502694627439702 ) ) ;
#17019=CARTESIAN_POINT ( 'NONE',  ( 9.457646018065525792E-16, -52.31249999863440792, 5.148502694627439702 ) ) ;
#17021=( LENGTH_UNIT ( ) NAMED_UNIT ( * ) SI_UNIT ( .MILLI., .METRE. ) );
#17022=CARTESIAN_POINT ( 'NONE',  ( -4.458734125000001214, -140.8750000013656063, 1.846868145590734089 ) ) ;
#17024=CARTESIAN_POINT ( 'NONE',  ( -6.972266317189433020E-16, -1.250000000000000000, -5.000000000000000000 ) ) ;
#17026=ADVANCED_FACE ( 'NONE', ( #22579 ), #37357, .T. ) ;
#17029=EDGE_CURVE ( 'NONE', #46822, #12246, #15725, .T. ) ;
#17032=ADVANCED_FACE ( 'NONE', ( #30508 ), #7038, .T. ) ;
#17033=CARTESIAN_POINT ( 'NONE',  ( -3.152801135295367096, -148.3125000013655779, -3.152801135295367541 ) ) ;
#17037=CARTESIAN_POINT ( 'NONE',  ( -2.229367062499996610, -63.39583333196774362, 3.861377020970582219 ) ) ;
#17038=CARTESIAN_POINT ( 'NONE',  ( -2.071067811865308972, -154.4375000027312126, 5.000000000000169642 ) ) ;
#17040=CARTESIAN_POINT ( 'NONE',  ( 1.846868145590736310, -143.6250000013655779, 4.458734124999997661 ) ) ;
#17042=ORIENTED_EDGE ( 'NONE', *, *, #3241, .T. ) ;
#17044=DIRECTION ( 'NONE',  ( 0.000000000000000000, 0.000000000000000000, 1.000000000000000000 ) ) ;
#17047=CARTESIAN_POINT ( 'NONE',  ( 1.975475456537005874E-15, -5.750000000000000000, 5.000000000000000000 ) ) ;
#17049=VECTOR ( 'NONE', #49929, 1000.000000000000000 ) ;
#17054=CARTESIAN_POINT ( 'NONE',  ( 5.000000000000000888, -56.45833333060214443, 2.886751345948126879 ) ) ;
#17055=CARTESIAN_POINT ( 'NONE',  ( 4.458734125000000326, 5.104166668032261711, 2.574251347313718519 ) ) ;
#17057=CARTESIAN_POINT ( 'NONE',  ( 4.458734124999998549, -18.97916666530106511, -2.574251347313721627 ) ) ;
#17059=CARTESIAN_POINT ( 'NONE',  ( 4.458734125000000326, -160.3750000013656063, -1.846868145590734978 ) ) ;
#17065=CARTESIAN_POINT ( 'NONE',  ( 4.458734124999998549, -34.72916666530107221, -2.574251347313721627 ) ) ;
#17066=FACE_OUTER_BOUND ( 'NONE', #52238, .T. ) ;
#17067=CARTESIAN_POINT ( 'NONE',  ( -4.458734124999999437, -60.56249999863440081, 0.000000000000000000 ) ) ;
#17069=CARTESIAN_POINT ( 'NONE',  ( -4.999999999999998224, -40.91666666666667140, 2.886751345948131764 ) ) ;
#17071=VERTEX_POINT ( 'NONE', #16366 ) ;
#17075=CARTESIAN_POINT ( 'NONE',  ( -3.535250795749689387E-16, -5.249999999999997335, -5.773502691896257311 ) ) ;
#17076=CARTESIAN_POINT ( 'NONE',  ( -3.152548672688508926E-16, -69.56249999863439371, -5.148502694627439702 ) ) ;
#17079=CARTESIAN_POINT ( 'NONE',  ( -3.535250795749689387E-16, -11.12499999726881761, -5.773502691896257311 ) ) ;
#17080=CARTESIAN_POINT ( 'NONE',  ( 4.458734125000001214, -39.89583333196772941, 2.574251347313718519 ) ) ;
#17081=VERTEX_POINT ( 'NONE', #959 ) ;
#17082=FACE_OUTER_BOUND ( 'NONE', #60665, .T. ) ;
#17083=CARTESIAN_POINT ( 'NONE',  ( 2.229367062499998831, 13.10416666803226171, -3.861377020970580887 ) ) ;
#17084=ORIENTED_EDGE ( 'NONE', *, *, #60657, .F. ) ;
#17085=CARTESIAN_POINT ( 'NONE',  ( 5.000000000000000000, -81.50000000000000000, -6.123233995736766282E-16 ) ) ;
#17086=CARTESIAN_POINT ( 'NONE',  ( 2.499999999999998668, -56.33333333333333570, -4.330127018922193649 ) ) ;
#17087=CARTESIAN_POINT ( 'NONE',  ( -4.458734124999999437, -160.1875000013655779, -5.460374474430324690E-16 ) ) ;
#17090=CARTESIAN_POINT ( 'NONE',  ( -2.229367062500000163, -79.47916666530106511, -3.861377020970580443 ) ) ;
#17091=CARTESIAN_POINT ( 'NONE',  ( 1.846868145590735200, -140.5000000013656347, -4.458734125000000326 ) ) ;
#17092=CARTESIAN_POINT ( 'NONE',  ( 2.229367062499998831, -86.64583333196773651, -3.861377020970580887 ) ) ;
#17094=CARTESIAN_POINT ( 'NONE',  ( -4.458734124999999437, -2.645833331967737845, -2.574251347313719407 ) ) ;
#17095=CARTESIAN_POINT ( 'NONE',  ( -4.458734124999998549, -34.47916666530107221, 2.574251347313722516 ) ) ;
#17096=CARTESIAN_POINT ( 'NONE',  ( -6.972266317189433020E-16, -16.12499999726881228, -5.000000000000000000 ) ) ;
#17100=FACE_OUTER_BOUND ( 'NONE', #9333, .T. ) ;
#17101=DIRECTION ( 'NONE',  ( -0.000000000000000000, 1.000000000000000000, -0.000000000000000000 ) ) ;
#17102=CARTESIAN_POINT ( 'NONE',  ( -4.458734124999999437, -68.64583333196773651, -2.574251347313719407 ) ) ;
#17104=ORIENTED_EDGE ( 'NONE', *, *, #3872, .T. ) ;
#17105=CARTESIAN_POINT ( 'NONE',  ( -6.972266317189433020E-16, -5.249999999999998224, -5.000000000000000000 ) ) ;
#17106=CARTESIAN_POINT ( 'NONE',  ( -5.000000000000000888, -146.5625000027311842, 2.071067811865474617 ) ) ;
#17108=DIRECTION ( 'NONE',  ( -0.000000000000000000, 1.000000000000000000, -0.000000000000000000 ) ) ;
#17109=CARTESIAN_POINT ( 'NONE',  ( 4.458734124999998549, 7.270833334698928674, -2.574251347313721627 ) ) ;
#17110=DIRECTION ( 'NONE',  ( -0.000000000000000000, 1.000000000000000000, -0.000000000000000000 ) ) ;
#17111=CARTESIAN_POINT ( 'NONE',  ( 1.846868145590736310, -155.6250000013655779, 4.458734124999997661 ) ) ;
#17113=VERTEX_POINT ( 'NONE', #10893 ) ;
#17117=LINE ( 'NONE', #61830, #58078 ) ;
#17119=LINE ( 'NONE', #51229, #36805 ) ;
#17121=CARTESIAN_POINT ( 'NONE',  ( 1.975475456537005874E-15, -10.75000000000000000, 5.000000000000000000 ) ) ;
#17122=CARTESIAN_POINT ( 'NONE',  ( 5.000000000000000888, -82.45833333060214443, 2.886751345948126879 ) ) ;
#17125=CARTESIAN_POINT ( 'NONE',  ( 9.457646018065525792E-16, -5.312499998634401699, 5.148502694627439702 ) ) ;
#17127=AXIS2_PLACEMENT_3D ( 'NONE', #34367, #44016, #9925 ) ;
#17130=CARTESIAN_POINT ( 'NONE',  ( -3.535533905932738641, -142.5000000027311842, 3.535533905932737309 ) ) ;
#17140=CARTESIAN_POINT ( 'NONE',  ( -4.458734124999999437, -163.1875000013655779, -5.460374474430324690E-16 ) ) ;
#17142=CARTESIAN_POINT ( 'NONE',  ( -5.000000000000000000, -56.99999999999999289, 0.000000000000000000 ) ) ;
#17144=CARTESIAN_POINT ( 'NONE',  ( 4.458734125000001214, 15.85416666803226171, 2.574251347313718519 ) ) ;
#17149=CARTESIAN_POINT ( 'NONE',  ( 5.000000000000000000, -16.50000000000000000, -6.123233995736766282E-16 ) ) ;
#17150=CARTESIAN_POINT ( 'NONE',  ( -2.499999999999996447, 6.166666666666667851, 4.330127018922195425 ) ) ;
#17151=CARTESIAN_POINT ( 'NONE',  ( -4.458734124999999437, -54.39583333196773651, -2.574251347313719407 ) ) ;
#17152=CARTESIAN_POINT ( 'NONE',  ( 2.499999999999998668, -6.333333333333336590, -4.330127018922193649 ) ) ;
#17154=CARTESIAN_POINT ( 'NONE',  ( 0.000000000000000000, -170.0000000000000000, 5.000000000000000000 ) ) ;
#17155=CARTESIAN_POINT ( 'NONE',  ( -5.000000000000000000, -64.00000000000000000, 0.000000000000000000 ) ) ;
#17156=DIRECTION ( 'NONE',  ( -0.000000000000000000, 1.000000000000000000, -0.000000000000000000 ) ) ;
#17157=CARTESIAN_POINT ( 'NONE',  ( -2.500000000000000444, -39.16666666666667140, -4.330127018922193649 ) ) ;
#17161=CARTESIAN_POINT ( 'NONE',  ( -3.152548672688508926E-16, -63.56249999863440792, -5.148502694627439702 ) ) ;
#17162=CARTESIAN_POINT ( 'NONE',  ( -4.458734124999999437, -150.1875000013656063, -5.460374474430324690E-16 ) ) ;
#17163=CARTESIAN_POINT ( 'NONE',  ( 9.457646018065525792E-16, -72.06249999863439371, 5.148502694627439702 ) ) ;
#17165=CARTESIAN_POINT ( 'NONE',  ( -4.458734124999999437, -19.56249999863440081, 0.000000000000000000 ) ) ;
#17166=CARTESIAN_POINT ( 'NONE',  ( 5.000000000000000000, -60.29166666393546592, -2.886751345948129988 ) ) ;
#17167=EDGE_LOOP ( 'NONE', ( #31869, #26738, #49910, #16373 ) ) ;
#17168=CARTESIAN_POINT ( 'NONE',  ( -5.000000000000000000, -49.08333333333332860, -2.886751345948128211 ) ) ;
#17171=DIRECTION ( 'NONE',  ( 0.000000000000000000, 0.000000000000000000, 1.000000000000000000 ) ) ;
#17172=CARTESIAN_POINT ( 'NONE',  ( 4.458734124999999437, -153.5000000013656063, 1.846868145590737864 ) ) ;
#17174=AXIS2_PLACEMENT_3D ( 'NONE', #6853, #2352, #15864 ) ;
#17176=CARTESIAN_POINT ( 'NONE',  ( 4.729367062499999719, -169.2812500020484094, 0.000000000000000000 ) ) ;
#17177=CARTESIAN_POINT ( 'NONE',  ( -5.000000000000000000, -74.87499999726880162, 0.000000000000000000 ) ) ;
#17178=CARTESIAN_POINT ( 'NONE',  ( -4.458734124999999437, -50.64583333196773651, -2.574251347313719407 ) ) ;
#17180=CARTESIAN_POINT ( 'NONE',  ( 1.339745962155615144, 10.41965820146970501, 4.999999999999999112 ) ) ;
#17183=CARTESIAN_POINT ( 'NONE',  ( -4.458734124999998549, 21.77083333469892779, 2.574251347313722516 ) ) ;
#17186=CARTESIAN_POINT ( 'NONE',  ( 3.535533905932738197, -164.8750000000000284, -3.535533905932738197 ) ) ;
#17195=CARTESIAN_POINT ( 'NONE',  ( 2.071067811865561215, -161.1874999999999716, 4.999999999999913847 ) ) ;
#17196=CARTESIAN_POINT ( 'NONE',  ( -5.000000000000000000, 18.91666666666666430, -2.886751345948128211 ) ) ;
#17200=LINE ( 'NONE', #50988, #5177 ) ;
#17202=CARTESIAN_POINT ( 'NONE',  ( -5.000000000000000888, -158.6875000027312126, -2.071067811865475949 ) ) ;
#17209=CARTESIAN_POINT ( 'NONE',  ( -5.000000000000000000, -146.5000000000000284, -6.123233995736766282E-16 ) ) ;
#17213=CARTESIAN_POINT ( 'NONE',  ( 4.458734124999999437, -24.81249999863440436, -5.460374474430324690E-16 ) ) ;
#17214=CARTESIAN_POINT ( 'NONE',  ( 1.975475456537005874E-15, 14.25000000000000000, 5.000000000000000000 ) ) ;
#17215=CARTESIAN_POINT ( 'NONE',  ( 5.000000000000000000, -153.0000000000000284, 0.000000000000000000 ) ) ;
#17217=CARTESIAN_POINT ( 'NONE',  ( 4.458734125000000326, -152.3750000013655779, -1.846868145590734978 ) ) ;
#17218=ORIENTED_EDGE ( 'NONE', *, *, #16075, .T. ) ;
#17220=CARTESIAN_POINT ( 'NONE',  ( 4.458734124999998549, -52.97916666530107932, -2.574251347313721627 ) ) ;
#17223=CARTESIAN_POINT ( 'NONE',  ( -5.000000000000000000, 22.91666666666666430, -2.886751345948128211 ) ) ;
#17224=VECTOR ( 'NONE', #37862, 1000.000000000000000 ) ;
#17226=CARTESIAN_POINT ( 'NONE',  ( 9.457646018065525792E-16, -1.062499998634405696, 5.148502694627439702 ) ) ;
#17229=EDGE_CURVE ( 'NONE', #62891, #19199, #36283, .T. ) ;
#17230=CARTESIAN_POINT ( 'NONE',  ( 3.061616997868383141E-16, -140.7500000000000000, -5.000000000000000000 ) ) ;
#17232=CARTESIAN_POINT ( 'NONE',  ( -2.229367062499996610, 15.60416666803225993, 3.861377020970582219 ) ) ;
#17233=CARTESIAN_POINT ( 'NONE',  ( -5.000000000000000000, 5.041666669397853795, -2.886751345948128211 ) ) ;
#17238=CARTESIAN_POINT ( 'NONE',  ( 3.535533905932736864, -168.2500000027312126, 3.535533905932738641 ) ) ;
#17239=CARTESIAN_POINT ( 'NONE',  ( 4.458734124999999437, -44.81249999863440081, -5.460374474430324690E-16 ) ) ;
#17240=CARTESIAN_POINT ( 'NONE',  ( 1.846868145590735200, -163.5000000013655779, -4.458734125000000326 ) ) ;
#17241=CARTESIAN_POINT ( 'NONE',  ( 5.000000000000000000, -44.37499999726880873, -6.123233995736766282E-16 ) ) ;
#17243=CARTESIAN_POINT ( 'NONE',  ( 4.458734125000001214, -19.89583333196773651, 2.574251347313718519 ) ) ;
#17245=CARTESIAN_POINT ( 'NONE',  ( 2.499999999999998668, -88.33333333333332860, -4.330127018922193649 ) ) ;
#17246=CARTESIAN_POINT ( 'NONE',  ( -1.846868145590737420, -163.7500000013655779, 4.458734124999999437 ) ) ;
#17248=VERTEX_POINT ( 'NONE', #36613 ) ;
#17250=CARTESIAN_POINT ( 'NONE',  ( 4.458734124999999437, -34.06249999863440792, -5.460374474430324690E-16 ) ) ;
#17251=CARTESIAN_POINT ( 'NONE',  ( -5.000000000000000888, -147.6875000027312126, -2.071067811865475949 ) ) ;
#17258=DIRECTION ( 'NONE',  ( -0.000000000000000000, 1.000000000000000000, -0.000000000000000000 ) ) ;
#17260=CARTESIAN_POINT ( 'NONE',  ( 2.229367062499998831, -80.89583333196773651, -3.861377020970580887 ) ) ;
#17262=CARTESIAN_POINT ( 'NONE',  ( 5.000000000000000888, -142.9375000000000284, -2.071067811865475505 ) ) ;
#17263=CARTESIAN_POINT ( 'NONE',  ( 5.000000000000000000, 24.50000000000000000, -6.123233995736766282E-16 ) ) ;
#17265=CARTESIAN_POINT ( 'NONE',  ( 4.458734124999998549, -47.72916666530106511, -2.574251347313721627 ) ) ;
#17266=CARTESIAN_POINT ( 'NONE',  ( -2.499999999999996447, 21.16666666666666785, 4.330127018922195425 ) ) ;
#17267=VECTOR ( 'NONE', #29786, 1000.000000000000000 ) ;
#17269=CARTESIAN_POINT ( 'NONE',  ( 2.499999999999998668, -3.333333333333333925, -4.330127018922193649 ) ) ;
#17272=CARTESIAN_POINT ( 'NONE',  ( 5.000000000000000000, 16.70833333606451987, -2.886751345948130876 ) ) ;
#17273=DIRECTION ( 'NONE',  ( -0.000000000000000000, 1.000000000000000000, -0.000000000000000000 ) ) ;
#17274=CARTESIAN_POINT ( 'NONE',  ( -3.152548672688508926E-16, -79.81249999863440792, -5.148502694627439702 ) ) ;
#17275=CARTESIAN_POINT ( 'NONE',  ( 0.000000000000000000, -170.0000000000000000, 0.000000000000000000 ) ) ;
#17278=ORIENTED_EDGE ( 'NONE', *, *, #60157, .F. ) ;
#17279=CARTESIAN_POINT ( 'NONE',  ( -1.339745962155613812, -15.08034179853029322, -5.000000000000000000 ) ) ;
#17281=CARTESIAN_POINT ( 'NONE',  ( 2.071067811865476394, -168.3125000027312410, 5.000000000000000000 ) ) ;
#17283=EDGE_CURVE ( 'NONE', #12901, #16392, #55925, .T. ) ;
#17284=CARTESIAN_POINT ( 'NONE',  ( -4.458734124999999437, 12.35416666803226171, -2.574251347313719407 ) ) ;
#17292=CARTESIAN_POINT ( 'NONE',  ( 4.458734124999999437, -8.812499998634406140, -5.460374474430324690E-16 ) ) ;
#17293=VERTEX_POINT ( 'NONE', #46268 ) ;
#17294=CARTESIAN_POINT ( 'NONE',  ( -4.458734124999999437, -35.56249999863440792, 0.000000000000000000 ) ) ;
#17299=CARTESIAN_POINT ( 'NONE',  ( -1.846868145590734756, -150.3750000013655779, -4.458734124999999437 ) ) ;
#17300=CARTESIAN_POINT ( 'NONE',  ( -2.229367062499996610, 21.85416666803226349, 3.861377020970582219 ) ) ;
#17302=EDGE_CURVE ( 'NONE', #34331, #60539, #9583, .T. ) ;
#17303=CARTESIAN_POINT ( 'NONE',  ( -1.339745962155564296, -26.08034179853029499, -5.000000000000028422 ) ) ;
#17304=CARTESIAN_POINT ( 'NONE',  ( -2.229367062500000163, -82.72916666530106511, -3.861377020970580443 ) ) ;
#17307=LINE ( 'NONE', #7032, #60397 ) ;
#17308=CARTESIAN_POINT ( 'NONE',  ( 1.060575238724906964E-15, 21.37500000273118417, 5.773502691896257311 ) ) ;
#17310=CARTESIAN_POINT ( 'NONE',  ( 1.339745962155612702, -35.29465819873851729, -5.000000000000000000 ) ) ;
#17312=( BOUNDED_CURVE ( )  B_SPLINE_CURVE ( 2, ( #23335, #26896, #2770, #18502, #13358, #22710, #17867, #47453, #22069 ),
 .UNSPECIFIED., .F., .F. ) 
 B_SPLINE_CURVE_WITH_KNOTS ( ( 3, 2, 2, 2, 3 ),
 ( 0.4395833333333333259, 0.4402777777777777679, 0.4416666666666666519, 0.4430555555555555358, 0.4437499999999999778 ),
 .UNSPECIFIED. ) 
 CURVE ( )  GEOMETRIC_REPRESENTATION_ITEM ( )  RATIONAL_B_SPLINE_CURVE ( ( 0.9330127018922194093, 0.9330127018922194093, 1.000000000000000000, 0.8660254037844387076, 1.000000000000000000, 0.8660254037844387076, 1.000000000000000000, 0.9330127018922194093, 0.9330127018922194093 ) ) 
 REPRESENTATION_ITEM ( '' )  );
#17313=VECTOR ( 'NONE', #34475, 1000.000000000000000 ) ;
#17316=CARTESIAN_POINT ( 'NONE',  ( 2.499999999999998668, -24.33333333333333215, -4.330127018922193649 ) ) ;
#17317=CARTESIAN_POINT ( 'NONE',  ( 9.457646018065525792E-16, -30.06249999863440081, 5.148502694627439702 ) ) ;
#17319=CARTESIAN_POINT ( 'NONE',  ( 4.458734124999999437, -86.81249999863439371, -5.460374474430324690E-16 ) ) ;
#17320=CARTESIAN_POINT ( 'NONE',  ( 5.000000000000000888, -31.45833333060214798, 2.886751345948126879 ) ) ;
#17321=CARTESIAN_POINT ( 'NONE',  ( -2.229367062500000163, -56.47916666530107221, -3.861377020970580443 ) ) ;
#17322=VERTEX_POINT ( 'NONE', #11213 ) ;
#17323=CARTESIAN_POINT ( 'NONE',  ( -6.972266317189433020E-16, -62.12499999726880162, -5.000000000000000000 ) ) ;
#17324=CARTESIAN_POINT ( 'NONE',  ( -2.229367062499996610, -6.395833331967741842, 3.861377020970582219 ) ) ;
#17326=CARTESIAN_POINT ( 'NONE',  ( 5.000000000000000000, -70.41666666666667140, -2.886751345948129988 ) ) ;
#17329=CARTESIAN_POINT ( 'NONE',  ( -2.500000000000000444, -79.04166666393547303, -4.330127018922193649 ) ) ;
#17330=CARTESIAN_POINT ( 'NONE',  ( -1.339745962155610925, -53.66965819600733312, 5.000000000000000000 ) ) ;
#17331=ORIENTED_EDGE ( 'NONE', *, *, #31543, .T. ) ;
#17334=CARTESIAN_POINT ( 'NONE',  ( 4.458734124999998549, -18.97916666530107221, -2.574251347313721627 ) ) ;
#17335=CARTESIAN_POINT ( 'NONE',  ( -2.229367062499996610, -56.39583333196773651, 3.861377020970582219 ) ) ;
#17337=( NAMED_UNIT ( * ) PLANE_ANGLE_UNIT ( ) SI_UNIT ( $, .RADIAN. ) );
#17338=CARTESIAN_POINT ( 'NONE',  ( 2.730187237215162345E-16, -142.1875000013656063, -4.458734124999999437 ) ) ;
#17340=CARTESIAN_POINT ( 'NONE',  ( 1.975475456537005874E-15, -60.75000000000000000, 5.000000000000000000 ) ) ;
#17341=( BOUNDED_CURVE ( )  B_SPLINE_CURVE ( 2, ( #33903, #58984, #53214, #34210, #8837, #48381, #53526, #43233, #44497 ),
 .UNSPECIFIED., .F., .F. ) 
 B_SPLINE_CURVE_WITH_KNOTS ( ( 3, 2, 2, 2, 3 ),
 ( 0.2416666666666668628, 0.2458333333333335147, 0.2500000000000002220, 0.2541666666666668739, 0.2583333333333335813 ),
 .UNSPECIFIED. ) 
 CURVE ( )  GEOMETRIC_REPRESENTATION_ITEM ( )  RATIONAL_B_SPLINE_CURVE ( ( 0.9999999999999964473, 0.9238795325112902912, 1.000000000000000000, 0.9238795325112867385, 1.000000000000000000, 0.9238795325112867385, 1.000000000000000000, 0.9238795325112826307, 1.000000000000003997 ) ) 
 REPRESENTATION_ITEM ( '' )  );
#17342=ORIENTED_EDGE ( 'NONE', *, *, #51926, .T. ) ;
#17345=FACE_OUTER_BOUND ( 'NONE', #19545, .T. ) ;
#17348=CARTESIAN_POINT ( 'NONE',  ( 4.458734124999999437, -148.7500000013656063, 1.846868145590737864 ) ) ;
#17352=CARTESIAN_POINT ( 'NONE',  ( -3.152548672688508926E-16, -62.81249999863440792, -5.148502694627439702 ) ) ;
#17353=CARTESIAN_POINT ( 'NONE',  ( -2.500000000000000444, -84.04166666393547303, -4.330127018922193649 ) ) ;
#17354=CARTESIAN_POINT ( 'NONE',  ( 1.339745962155612702, 6.830341803992665994, -5.000000000000000000 ) ) ;
#17355=CARTESIAN_POINT ( 'NONE',  ( 1.846868145590735200, -143.2500000013655779, -4.458734124999999437 ) ) ;
#17356=VECTOR ( 'NONE', #51646, 1000.000000000000000 ) ;
#17359=ORIENTED_EDGE ( 'NONE', *, *, #49692, .F. ) ;
#17364=CYLINDRICAL_SURFACE ( 'NONE', #47972, 5.000000000000000000 ) ;
#17366=CARTESIAN_POINT ( 'NONE',  ( 4.458734125000000326, 28.85416666803226704, 2.574251347313718519 ) ) ;
#17367=CARTESIAN_POINT ( 'NONE',  ( 1.339745962155615144, -76.58034179853029855, 4.999999999999999112 ) ) ;
#17370=EDGE_CURVE ( 'NONE', #7918, #47469, #47745, .T. ) ;
#17374=CARTESIAN_POINT ( 'NONE',  ( 1.975475456537005874E-15, -24.74999999999999645, 5.000000000000000000 ) ) ;
#17375=DIRECTION ( 'NONE',  ( -0.000000000000000000, 1.000000000000000000, -0.000000000000000000 ) ) ;
#17376=EDGE_CURVE ( 'NONE', #58377, #30399, #29676, .T. ) ;
#17377=CARTESIAN_POINT ( 'NONE',  ( 4.458734124999999437, 6.187500001365593860, -5.460374474430324690E-16 ) ) ;
#17379=VECTOR ( 'NONE', #57638, 1000.000000000000000 ) ;
#17380=CARTESIAN_POINT ( 'NONE',  ( 4.458734124999999437, -18.06249999863440792, -5.460374474430324690E-16 ) ) ;
#17383=CARTESIAN_POINT ( 'NONE',  ( -1.846868145590734756, -159.1250000013656063, -4.458734125000000326 ) ) ;
#17384=DIRECTION ( 'NONE',  ( -0.000000000000000000, 1.000000000000000000, -0.000000000000000000 ) ) ;
#17388=EDGE_CURVE ( 'NONE', #29321, #53941, #40775, .T. ) ;
#17389=CARTESIAN_POINT ( 'NONE',  ( 1.975475456537005874E-15, -35.75000000000000711, 5.000000000000000000 ) ) ;
#17390=CARTESIAN_POINT ( 'NONE',  ( 2.229367062499998831, -40.64583333196773651, -3.861377020970580887 ) ) ;
#17392=CARTESIAN_POINT ( 'NONE',  ( 2.500000000000002220, -60.66666666666665719, 4.330127018922192761 ) ) ;
#17393=CARTESIAN_POINT ( 'NONE',  ( -2.229367062500000163, -68.72916666530107932, -3.861377020970580443 ) ) ;
#17398=CARTESIAN_POINT ( 'NONE',  ( -2.499999999999996447, -84.83333333333332860, 4.330127018922195425 ) ) ;
#17399=CARTESIAN_POINT ( 'NONE',  ( 3.061616997868383141E-16, -143.8750000027312126, -5.000000000000000000 ) ) ;
#17401=CARTESIAN_POINT ( 'NONE',  ( 2.500000000000002220, -6.666666666666667851, 4.330127018922192761 ) ) ;
#17403=CARTESIAN_POINT ( 'NONE',  ( 9.457646018065525792E-16, -70.06249999863439371, 5.148502694627439702 ) ) ;
#17405=CARTESIAN_POINT ( 'NONE',  ( 1.060575238724906964E-15, -12.62499999726881050, 5.773502691896257311 ) ) ;
#17406=CARTESIAN_POINT ( 'NONE',  ( -2.229367062500000163, -41.47916666530107932, -3.861377020970580443 ) ) ;
#17407=ORIENTED_EDGE ( 'NONE', *, *, #19682, .T. ) ;
#17408=DIRECTION ( 'NONE',  ( -0.000000000000000000, 1.000000000000000000, -0.000000000000000000 ) ) ;
#17409=CARTESIAN_POINT ( 'NONE',  ( -4.458734124999998549, 5.520833334698927786, 2.574251347313722516 ) ) ;
#17411=CARTESIAN_POINT ( 'NONE',  ( -5.000000000000000888, -151.4375000000000000, 2.071067811865474617 ) ) ;
#17412=CARTESIAN_POINT ( 'NONE',  ( 5.000000000000000888, -57.58333333333334281, 2.886751345948126879 ) ) ;
#17413=CARTESIAN_POINT ( 'NONE',  ( -4.458734124999999437, -162.1875000013655779, -5.460374474430324690E-16 ) ) ;
#17415=CARTESIAN_POINT ( 'NONE',  ( 2.071067811865392461, -145.1875000000000568, 5.000000000000084377 ) ) ;
#17416=CARTESIAN_POINT ( 'NONE',  ( -3.152548672688508926E-16, -79.56249999863440792, -5.148502694627439702 ) ) ;
#17417=CARTESIAN_POINT ( 'NONE',  ( 3.535533905932736864, -167.1250000000000284, 3.535533905932738641 ) ) ;
#17418=CARTESIAN_POINT ( 'NONE',  ( -4.458734124999998549, -89.22916666530106511, 2.574251347313722516 ) ) ;
#17421=CARTESIAN_POINT ( 'NONE',  ( 4.458734124999999437, -0.06249999863440491854, -5.460374474430324690E-16 ) ) ;
#17422=CARTESIAN_POINT ( 'NONE',  ( 2.229367062500001939, -36.22916666530107221, 3.861377020970579999 ) ) ;
#17423=CARTESIAN_POINT ( 'NONE',  ( -1.339745962155617365, 24.33034180399266688, 4.999999999999998224 ) ) ;
#17425=CARTESIAN_POINT ( 'NONE',  ( -2.500000000000000444, 15.95833333606451809, -4.330127018922193649 ) ) ;
#17428=CARTESIAN_POINT ( 'NONE',  ( 3.061616997868383141E-16, -151.7500000000000284, -5.000000000000000000 ) ) ;
#17429=CARTESIAN_POINT ( 'NONE',  ( 2.229367062499998831, -67.89583333196773651, -3.861377020970580887 ) ) ;
#17432=CARTESIAN_POINT ( 'NONE',  ( 3.061616997868383141E-16, -163.7500000000000000, -5.000000000000000000 ) ) ;
#17433=DIRECTION ( 'NONE',  ( -0.000000000000000000, 1.000000000000000000, -0.000000000000000000 ) ) ;
#17436=CARTESIAN_POINT ( 'NONE',  ( 4.458734124999999437, 4.187500001365595637, -5.460374474430324690E-16 ) ) ;
#17438=CARTESIAN_POINT ( 'NONE',  ( -4.458734125000000326, -158.8750000013655779, 1.846868145590734089 ) ) ;
#17449=DIRECTION ( 'NONE',  ( -0.000000000000000000, 1.000000000000000000, -0.000000000000000000 ) ) ;
#17452=CARTESIAN_POINT ( 'NONE',  ( -4.458734124999999437, 21.60416666803226349, -2.574251347313719407 ) ) ;
#17454=CARTESIAN_POINT ( 'NONE',  ( -4.458734124999999437, -2.562499998634407028, 0.000000000000000000 ) ) ;
#17457=CARTESIAN_POINT ( 'NONE',  ( -5.000000000000000888, -141.6875000027312126, -2.071067811865475949 ) ) ;
#17458=CARTESIAN_POINT ( 'NONE',  ( -1.339745962155613812, -52.20534180126148271, -5.000000000000000000 ) ) ;
#17463=CARTESIAN_POINT ( 'NONE',  ( 4.458734124999999437, -139.5625000013656063, 0.000000000000000000 ) ) ;
#17467=CARTESIAN_POINT ( 'NONE',  ( 4.458734124999999437, -159.6250000013655779, -1.846868145590734978 ) ) ;
#17471=CARTESIAN_POINT ( 'NONE',  ( -4.458734124999999437, 15.35416666803225993, -2.574251347313719407 ) ) ;
#17472=ORIENTED_EDGE ( 'NONE', *, *, #4642, .F. ) ;
#17477=CARTESIAN_POINT ( 'NONE',  ( -4.999999999999999112, 6.083333333333333037, 2.886751345948131764 ) ) ;
#17478=CARTESIAN_POINT ( 'NONE',  ( -4.458734124999999437, -54.31249999863440081, 0.000000000000000000 ) ) ;
#17485=CYLINDRICAL_SURFACE ( 'NONE', #4266, 5.000000000000000000 ) ;
#17486=CARTESIAN_POINT ( 'NONE',  ( 2.499999999999998668, -37.33333333333332860, -4.330127018922193649 ) ) ;
#17487=DIRECTION ( 'NONE',  ( -0.000000000000000000, 1.000000000000000000, -0.000000000000000000 ) ) ;
#17488=CARTESIAN_POINT ( 'NONE',  ( -5.000000000000000000, -48.00000000000000000, 0.000000000000000000 ) ) ;
#17491=CARTESIAN_POINT ( 'NONE',  ( -4.458734124999998549, -65.22916666530106511, 2.574251347313722516 ) ) ;
#17492=CARTESIAN_POINT ( 'NONE',  ( -8.190561711645485556E-16, -149.9375000013656063, 4.458734124999999437 ) ) ;
#17493=CARTESIAN_POINT ( 'NONE',  ( 2.229367062499998831, -71.64583333196773651, -3.861377020970580887 ) ) ;
#17495=CARTESIAN_POINT ( 'NONE',  ( -4.458734124999999437, -17.56249999863440792, 0.000000000000000000 ) ) ;
#17496=CARTESIAN_POINT ( 'NONE',  ( 5.000000000000000000, -61.37499999726880873, -6.123233995736766282E-16 ) ) ;
#17501=CARTESIAN_POINT ( 'NONE',  ( 1.339745962155612702, -21.16965819600733312, -5.000000000000000000 ) ) ;
#17503=CARTESIAN_POINT ( 'NONE',  ( -3.152801135295367096, -152.0625000013655779, -3.152801135295367541 ) ) ;
#17508=CARTESIAN_POINT ( 'NONE',  ( -6.972266317189433020E-16, -56.12499999726880162, -5.000000000000000000 ) ) ;
#17509=CARTESIAN_POINT ( 'NONE',  ( 9.457646018065525792E-16, -53.31249999863441502, 5.148502694627439702 ) ) ;
#17513=CARTESIAN_POINT ( 'NONE',  ( -4.458734124999999437, 23.60416666803225993, -2.574251347313719407 ) ) ;
#17516=CARTESIAN_POINT ( 'NONE',  ( 1.846868145590736310, -167.6250000013656347, 4.458734124999997661 ) ) ;
#17531=ORIENTED_EDGE ( 'NONE', *, *, #15862, .F. ) ;
#17534=CARTESIAN_POINT ( 'NONE',  ( -5.000000000000000888, -153.5625000027312126, 2.071067811865474617 ) ) ;
#17540=CARTESIAN_POINT ( 'NONE',  ( 3.061616997868383141E-16, -145.7500000000000284, -5.000000000000000000 ) ) ;
#17543=CARTESIAN_POINT ( 'NONE',  ( -9.184850993605147944E-16, -141.3750000027312126, 5.000000000000000000 ) ) ;
#17544=CARTESIAN_POINT ( 'NONE',  ( -4.458734124999999437, -26.31249999863440792, 0.000000000000000000 ) ) ;
#17546=CARTESIAN_POINT ( 'NONE',  ( 5.000000000000000888, 18.54166666939785202, 2.886751345948126879 ) ) ;
#17548=CARTESIAN_POINT ( 'NONE',  ( -4.458734124999999437, -147.9375000013656063, -5.460374474430324690E-16 ) ) ;
#17549=ORIENTED_EDGE ( 'NONE', *, *, #53458, .T. ) ;
#17551=CARTESIAN_POINT ( 'NONE',  ( -2.229367062499996610, -50.39583333196772941, 3.861377020970582219 ) ) ;
#17552=( BOUNDED_CURVE ( )  B_SPLINE_CURVE ( 2, ( #30701, #25558, #31658, #11711, #50326, #60944, #5949, #17180, #45175 ),
 .UNSPECIFIED., .F., .F. ) 
 B_SPLINE_CURVE_WITH_KNOTS ( ( 3, 2, 2, 2, 3 ),
 ( 0.1520833333333333481, 0.1527777777777777901, 0.1541666666666666741, 0.1555555555555555580, 0.1562500000000000000 ),
 .UNSPECIFIED. ) 
 CURVE ( )  GEOMETRIC_REPRESENTATION_ITEM ( )  RATIONAL_B_SPLINE_CURVE ( ( 0.9330127018922194093, 0.9330127018922207416, 1.000000000000000000, 0.8660254037844387076, 1.000000000000000000, 0.8660254037844387076, 1.000000000000000000, 0.9330127018922194093, 0.9330127018922194093 ) ) 
 REPRESENTATION_ITEM ( '' )  );
#17553=DIRECTION ( 'NONE',  ( -0.000000000000000000, 1.000000000000000000, -0.000000000000000000 ) ) ;
#17555=CARTESIAN_POINT ( 'NONE',  ( 5.000000000000000000, 26.58333333333333570, -2.886751345948129988 ) ) ;
#17556=DIRECTION ( 'NONE',  ( 0.000000000000000000, 0.000000000000000000, 1.000000000000000000 ) ) ;
#17557=CARTESIAN_POINT ( 'NONE',  ( 4.458734124999998549, -0.7291666653010709931, -2.574251347313721627 ) ) ;
#17558=CARTESIAN_POINT ( 'NONE',  ( -2.500000000000000444, -11.16666666666666430, -4.330127018922193649 ) ) ;
#17561=CARTESIAN_POINT ( 'NONE',  ( -3.152548672688508926E-16, 11.18750000136559564, -5.148502694627439702 ) ) ;
#17562=ORIENTED_EDGE ( 'NONE', *, *, #5516, .T. ) ;
#17566=CARTESIAN_POINT ( 'NONE',  ( 4.458734124999999437, -50.81249999863440792, -5.460374474430324690E-16 ) ) ;
#17567=CARTESIAN_POINT ( 'NONE',  ( -4.458734124999999437, -163.1875000013655779, -5.460374474430324690E-16 ) ) ;
#17568=CARTESIAN_POINT ( 'NONE',  ( 5.000000000000000888, -43.45833333060214443, 2.886751345948126879 ) ) ;
#17570=CARTESIAN_POINT ( 'NONE',  ( -4.458734124999999437, -25.39583333196773651, -2.574251347313719407 ) ) ;
#17571=ORIENTED_EDGE ( 'NONE', *, *, #6431, .F. ) ;
#17573=CARTESIAN_POINT ( 'NONE',  ( -1.846868145590737420, -164.7500000013656063, 4.458734124999999437 ) ) ;
#17574=CARTESIAN_POINT ( 'NONE',  ( 5.000000000000000000, -39.29166666393548724, -2.886751345948130876 ) ) ;
#17576=EDGE_CURVE ( 'NONE', #41033, #21097, #42842, .T. ) ;
#17577=CARTESIAN_POINT ( 'NONE',  ( -4.458734124999999437, -38.64583333196772941, -2.574251347313719407 ) ) ;
#17578=CARTESIAN_POINT ( 'NONE',  ( -2.500000000000000444, 19.95833333606451987, -4.330127018922193649 ) ) ;
#17579=ORIENTED_EDGE ( 'NONE', *, *, #11849, .T. ) ;
#17583=CARTESIAN_POINT ( 'NONE',  ( 1.339745962155612702, 24.83034180399266333, -5.000000000000000000 ) ) ;
#17584=ORIENTED_EDGE ( 'NONE', *, *, #40951, .T. ) ;
#17587=CARTESIAN_POINT ( 'NONE',  ( 4.458734125000001214, -79.14583333196772230, 2.574251347313718519 ) ) ;
#17593=CARTESIAN_POINT ( 'NONE',  ( -2.500000000000000444, -72.04166666393548724, -4.330127018922193649 ) ) ;
#17597=CARTESIAN_POINT ( 'NONE',  ( -5.000000000000000000, 4.000000000000000000, 0.000000000000000000 ) ) ;
#17601=CYLINDRICAL_SURFACE ( 'NONE', #36758, 5.000000000000000000 ) ;
#17602=CARTESIAN_POINT ( 'NONE',  ( 9.457646018065525792E-16, -78.31249999863442213, 5.148502694627439702 ) ) ;
#17608=CARTESIAN_POINT ( 'NONE',  ( -5.000000000000000888, -164.6875000027311842, -2.071067811865475949 ) ) ;
#17610=CARTESIAN_POINT ( 'NONE',  ( 4.458734124999998549, 13.02083333469892779, -2.574251347313721627 ) ) ;
#17616=CARTESIAN_POINT ( 'NONE',  ( 3.061616997868383141E-16, -168.7500000000000000, -5.000000000000000000 ) ) ;
#17617=CARTESIAN_POINT ( 'NONE',  ( 0.000000000000000000, -170.0000000000000000, 0.000000000000000000 ) ) ;
#17618=CARTESIAN_POINT ( 'NONE',  ( -4.458734124999999437, -7.395833331967734736, -2.574251347313719407 ) ) ;
#17619=CARTESIAN_POINT ( 'NONE',  ( -6.972266317189433020E-16, -29.25000000000000000, -5.000000000000000000 ) ) ;
#17621=CARTESIAN_POINT ( 'NONE',  ( 2.229367062499998831, -35.89583333196773651, -3.861377020970580887 ) ) ;
#17626=CARTESIAN_POINT ( 'NONE',  ( 4.458734124999997661, -150.7500000013656347, 1.846868145590737864 ) ) ;
#17627=CARTESIAN_POINT ( 'NONE',  ( -2.229367062500000163, 15.52083333469892779, -3.861377020970580443 ) ) ;
#17629=CARTESIAN_POINT ( 'NONE',  ( 2.229367062499998831, -85.89583333196773651, -3.861377020970580887 ) ) ;
#17632=CARTESIAN_POINT ( 'NONE',  ( 2.500000000000002220, 19.45833333606451632, 4.330127018922192761 ) ) ;
#17634=CARTESIAN_POINT ( 'NONE',  ( -6.972266317189433020E-16, -66.12499999726881583, -5.000000000000000000 ) ) ;
#17636=CARTESIAN_POINT ( 'NONE',  ( 5.000000000000000888, -27.58333333333333215, 2.886751345948126879 ) ) ;
#17637=CARTESIAN_POINT ( 'NONE',  ( 2.229367062500001939, -31.97916666530106866, 3.861377020970579999 ) ) ;
#17640=CARTESIAN_POINT ( 'NONE',  ( 2.500000000000002220, -26.54166666393547658, 4.330127018922192761 ) ) ;
#17641=CARTESIAN_POINT ( 'NONE',  ( -2.229367062499996610, -59.14583333196773651, 3.861377020970582219 ) ) ;
#17644=CARTESIAN_POINT ( 'NONE',  ( 4.458734124999998549, -10.97916666530107044, -2.574251347313721627 ) ) ;
#17646=CARTESIAN_POINT ( 'NONE',  ( -5.000000000000000000, -71.00000000000000000, 0.000000000000000000 ) ) ;
#17650=CARTESIAN_POINT ( 'NONE',  ( 5.000000000000000888, -77.45833333060213022, 2.886751345948126879 ) ) ;
#17651=CARTESIAN_POINT ( 'NONE',  ( -6.972266317189433020E-16, -13.25000000000000000, -5.000000000000000000 ) ) ;
#17654=EDGE_CURVE ( 'NONE', #62091, #21757, #24566, .T. ) ;
#17655=CARTESIAN_POINT ( 'NONE',  ( -4.458734124999999437, -17.64583333196773651, -2.574251347313719407 ) ) ;
#17656=CARTESIAN_POINT ( 'NONE',  ( 2.229367062500001939, -55.22916666530107221, 3.861377020970579999 ) ) ;
#17657=CARTESIAN_POINT ( 'NONE',  ( -5.000000000000000000, -24.08333333333333215, -2.886751345948128211 ) ) ;
#17658=CARTESIAN_POINT ( 'NONE',  ( -4.458734125000000326, -142.0000000013655495, -1.846868145590735644 ) ) ;
#17660=CARTESIAN_POINT ( 'NONE',  ( 0.000000000000000000, -170.0000000000000000, 0.000000000000000000 ) ) ;
#17661=ORIENTED_EDGE ( 'NONE', *, *, #3313, .F. ) ;
#17665=DIRECTION ( 'NONE',  ( 0.000000000000000000, 0.000000000000000000, 1.000000000000000000 ) ) ;
#17668=CARTESIAN_POINT ( 'NONE',  ( 1.846868145590736310, -146.8750000013656063, 4.458734124999999437 ) ) ;
#17670=ADVANCED_FACE ( 'NONE', ( #23935 ), #9756, .T. ) ;
#17671=CARTESIAN_POINT ( 'NONE',  ( -6.972266317189433020E-16, 1.875000002731185722, -5.000000000000000000 ) ) ;
#17673=CARTESIAN_POINT ( 'NONE',  ( 4.458734125000001214, -64.14583333196773651, 2.574251347313718519 ) ) ;
#17674=CARTESIAN_POINT ( 'NONE',  ( -5.000000000000000888, -154.5625000027311842, 2.071067811865474617 ) ) ;
#17675=CARTESIAN_POINT ( 'NONE',  ( -8.190561711645485556E-16, -146.6875000013656063, 4.458734124999999437 ) ) ;
#17677=ORIENTED_EDGE ( 'NONE', *, *, #31726, .T. ) ;
#17682=CARTESIAN_POINT ( 'NONE',  ( 1.339745962155615144, -36.70534180126148271, 4.999999999999999112 ) ) ;
#17684=CARTESIAN_POINT ( 'NONE',  ( 4.458734124999998549, 27.02083333469892068, -2.574251347313721627 ) ) ;
#17685=CARTESIAN_POINT ( 'NONE',  ( 2.500000000000002220, -76.54166666393547303, 4.330127018922192761 ) ) ;
#17688=FACE_OUTER_BOUND ( 'NONE', #4824, .T. ) ;
#17690=CARTESIAN_POINT ( 'NONE',  ( -4.458734124999997661, 5.770833334698928674, 2.574251347313722516 ) ) ;
#17692=CARTESIAN_POINT ( 'NONE',  ( 4.458734124999999437, -20.06249999863440081, -5.460374474430324690E-16 ) ) ;
#17693=( BOUNDED_CURVE ( )  B_SPLINE_CURVE ( 2, ( #30577, #9681, #5189, #1343, #25438, #24486, #45058, #58892, #34126 ),
 .UNSPECIFIED., .F., .F. ) 
 B_SPLINE_CURVE_WITH_KNOTS ( ( 3, 2, 2, 2, 3 ),
 ( 0.8270833333333332815, 0.8277777777777777235, 0.8291666666666667185, 0.8305555555555556024, 0.8312500000000000444 ),
 .UNSPECIFIED. ) 
 CURVE ( )  GEOMETRIC_REPRESENTATION_ITEM ( )  RATIONAL_B_SPLINE_CURVE ( ( 0.9330127018922194093, 0.9330127018922194093, 1.000000000000000000, 0.8660254037844387076, 1.000000000000000000, 0.8660254037844387076, 1.000000000000000000, 0.9330127018922194093, 0.9330127018922194093 ) ) 
 REPRESENTATION_ITEM ( '' )  );
#17695=CARTESIAN_POINT ( 'NONE',  ( -1.846868145590734756, -158.1250000013656063, -4.458734125000000326 ) ) ;
#17696=CARTESIAN_POINT ( 'NONE',  ( -1.339745962155613368, 28.91965820146970501, -5.000000000000000000 ) ) ;
#17699=CARTESIAN_POINT ( 'NONE',  ( -4.458734124999999437, -39.39583333196773651, -2.574251347313719407 ) ) ;
#17702=CARTESIAN_POINT ( 'NONE',  ( -2.229367062499996610, -69.39583333196773651, 3.861377020970582219 ) ) ;
#17704=CARTESIAN_POINT ( 'NONE',  ( 2.499999999999998668, -57.20833333060214443, -4.330127018922193649 ) ) ;
#17706=ORIENTED_EDGE ( 'NONE', *, *, #46410, .T. ) ;
#17709=CARTESIAN_POINT ( 'NONE',  ( 5.000000000000000000, -5.416666666666666963, -2.886751345948129988 ) ) ;
#17710=CARTESIAN_POINT ( 'NONE',  ( -4.458734124999999437, -75.39583333196773651, -2.574251347313719407 ) ) ;
#17712=CARTESIAN_POINT ( 'NONE',  ( -5.000000000000000000, -14.87499999726881228, 0.000000000000000000 ) ) ;
#17713=CARTESIAN_POINT ( 'NONE',  ( 9.457646018065525792E-16, -42.06249999863440081, 5.148502694627439702 ) ) ;
#17714=ORIENTED_EDGE ( 'NONE', *, *, #15336, .T. ) ;
#17716=CARTESIAN_POINT ( 'NONE',  ( 2.229367062500001939, 4.770833334698926897, 3.861377020970579999 ) ) ;
#17718=CARTESIAN_POINT ( 'NONE',  ( -6.972266317189433020E-16, -81.12499999726881583, -5.000000000000000000 ) ) ;
#17719=CARTESIAN_POINT ( 'NONE',  ( -3.535250795749689387E-16, -58.24999999999999289, -5.773502691896257311 ) ) ;
#17720=CARTESIAN_POINT ( 'NONE',  ( 3.152801135295366208, -158.8125000013656063, 3.152801135295367985 ) ) ;
#17722=CARTESIAN_POINT ( 'NONE',  ( 4.458734124999998549, -79.72916666530107932, -2.574251347313721627 ) ) ;
#17723=CARTESIAN_POINT ( 'NONE',  ( 2.071067811865475505, -166.8125000000000000, -5.000000000000000888 ) ) ;
#17724=CARTESIAN_POINT ( 'NONE',  ( 4.458734125000001214, -89.89583333196775072, 2.574251347313718519 ) ) ;
#17726=CARTESIAN_POINT ( 'NONE',  ( 4.458734125000001214, -2.145833331967737845, 2.574251347313718519 ) ) ;
#17727=CARTESIAN_POINT ( 'NONE',  ( -2.229367062500000163, -39.72916666530107221, -3.861377020970580443 ) ) ;
#17728=ADVANCED_FACE ( 'NONE', ( #43848 ), #49324, .T. ) ;
#17729=ADVANCED_FACE ( 'NONE', ( #48996 ), #9139, .T. ) ;
#17731=CARTESIAN_POINT ( 'NONE',  ( 3.061616997868383141E-16, -154.7500000000000000, -5.000000000000000000 ) ) ;
#17732=ORIENTED_EDGE ( 'NONE', *, *, #45025, .F. ) ;
#17735=CARTESIAN_POINT ( 'NONE',  ( 2.229367062500001939, -68.22916666530106511, 3.861377020970579999 ) ) ;
#17738=ORIENTED_EDGE ( 'NONE', *, *, #33852, .F. ) ;
#17739=EDGE_CURVE ( 'NONE', #51645, #22889, #14466, .T. ) ;
#17741=CARTESIAN_POINT ( 'NONE',  ( 3.061616997868383141E-16, -146.8750000027312126, -5.000000000000000000 ) ) ;
#17745=CARTESIAN_POINT ( 'NONE',  ( 4.458734125000001214, 2.104166668032262599, 2.574251347313718519 ) ) ;
#17746=CARTESIAN_POINT ( 'NONE',  ( -5.000000000000000000, -43.08333333333333570, -2.886751345948128211 ) ) ;
#17747=CARTESIAN_POINT ( 'NONE',  ( 4.458734124999999437, -156.3750000013655779, -1.846868145590734978 ) ) ;
#17749=ORIENTED_EDGE ( 'NONE', *, *, #58946, .T. ) ;
#17753=CYLINDRICAL_SURFACE ( 'NONE', #15980, 5.000000000000000000 ) ;
#17754=CARTESIAN_POINT ( 'NONE',  ( 1.339745962155615144, -23.58034179853029144, 4.999999999999999112 ) ) ;
#17757=DIRECTION ( 'NONE',  ( 0.000000000000000000, 0.000000000000000000, 1.000000000000000000 ) ) ;
#17759=CARTESIAN_POINT ( 'NONE',  ( -3.152548672688508926E-16, 25.43750000136559208, -5.148502694627439702 ) ) ;
#17761=CARTESIAN_POINT ( 'NONE',  ( 4.458734125000000326, -4.145833331967739177, 2.574251347313718519 ) ) ;
#17764=CARTESIAN_POINT ( 'NONE',  ( 5.000000000000000000, -140.1250000027312126, 0.000000000000000000 ) ) ;
#17771=CARTESIAN_POINT ( 'NONE',  ( -3.152801135295367096, -157.3125000013656063, -3.152801135295367541 ) ) ;
#17774=ORIENTED_EDGE ( 'NONE', *, *, #5933, .F. ) ;
#17775=CARTESIAN_POINT ( 'NONE',  ( 4.458734124999999437, 18.93750000136559564, -5.460374474430324690E-16 ) ) ;
#17781=CARTESIAN_POINT ( 'NONE',  ( -5.000000000000000000, 10.91666666666666607, -2.886751345948128211 ) ) ;
#17782=CARTESIAN_POINT ( 'NONE',  ( -2.229367062499996610, -54.14583333196773651, 3.861377020970582219 ) ) ;
#17783=CARTESIAN_POINT ( 'NONE',  ( 1.975475456537005874E-15, -7.750000000000000000, 5.000000000000000000 ) ) ;
#17786=CARTESIAN_POINT ( 'NONE',  ( 2.500000000000002220, 7.458333336064517205, 4.330127018922192761 ) ) ;
#17788=CARTESIAN_POINT ( 'NONE',  ( -4.999999999999999112, -41.91666666666667140, 2.886751345948131764 ) ) ;
#17789=LINE ( 'NONE', #26495, #11980 ) ;
#17793=CARTESIAN_POINT ( 'NONE',  ( -4.458734124999999437, -65.31249999863440792, 0.000000000000000000 ) ) ;
#17794=CARTESIAN_POINT ( 'NONE',  ( -3.152801135295367096, -148.3125000013655779, -3.152801135295367541 ) ) ;
#17795=CARTESIAN_POINT ( 'NONE',  ( 4.458734125000001214, -71.89583333196773651, 2.574251347313718519 ) ) ;
#17797=CARTESIAN_POINT ( 'NONE',  ( 2.229367062500001939, -23.22916666530107221, 3.861377020970579999 ) ) ;
#17798=CARTESIAN_POINT ( 'NONE',  ( -4.999999999999999112, -59.79166666393547303, 2.886751345948131764 ) ) ;
#17809=CARTESIAN_POINT ( 'NONE',  ( 4.458734124999999437, -55.06249999863440081, -5.460374474430324690E-16 ) ) ;
#17810=ORIENTED_EDGE ( 'NONE', *, *, #57781, .F. ) ;
#17811=( BOUNDED_CURVE ( )  B_SPLINE_CURVE ( 2, ( #50500, #30220, #41463, #2568, #7396, #17674, #61114, #17038, #46622 ),
 .UNSPECIFIED., .F., .F. ) 
 B_SPLINE_CURVE_WITH_KNOTS ( ( 3, 2, 2, 2, 3 ),
 ( 0.4750000000000004219, 0.4791666666666671293, 0.4833333333333337811, 0.4875000000000004330, 0.4916666666666670849 ),
 .UNSPECIFIED. ) 
 CURVE ( )  GEOMETRIC_REPRESENTATION_ITEM ( )  RATIONAL_B_SPLINE_CURVE ( ( 0.9999999999999918954, 0.9238795325112948431, 1.000000000000000000, 0.9238795325112867385, 1.000000000000000000, 0.9238795325112867385, 1.000000000000000000, 0.9238795325112786339, 1.000000000000008216 ) ) 
 REPRESENTATION_ITEM ( '' )  );
#17815=CARTESIAN_POINT ( 'NONE',  ( 4.458734125000001214, 20.10416666803225993, 2.574251347313718519 ) ) ;
#17819=ORIENTED_EDGE ( 'NONE', *, *, #21284, .T. ) ;
#17822=CARTESIAN_POINT ( 'NONE',  ( 6.123233995736766282E-16, -170.0000000000000000, -5.000000000000000000 ) ) ;
#17824=EDGE_CURVE ( 'NONE', #37366, #11915, #47362, .T. ) ;
#17825=CARTESIAN_POINT ( 'NONE',  ( 1.339745962155615144, -69.58034179853028434, 4.999999999999999112 ) ) ;
#17828=CARTESIAN_POINT ( 'NONE',  ( -6.972266317189433020E-16, 4.749999999999999112, -5.000000000000000000 ) ) ;
#17830=CARTESIAN_POINT ( 'NONE',  ( -6.972266317189433020E-16, -76.24999999999998579, -5.000000000000000000 ) ) ;
#17835=CARTESIAN_POINT ( 'NONE',  ( -2.500000000000000444, -5.041666663935480130, -4.330127018922193649 ) ) ;
#17837=CARTESIAN_POINT ( 'NONE',  ( 3.061616997868383141E-16, -152.8750000027311842, -5.000000000000000000 ) ) ;
#17838=VERTEX_POINT ( 'NONE', #35814 ) ;
#17843=CARTESIAN_POINT ( 'NONE',  ( 3.061616997868383141E-16, -146.7500000000000284, -5.000000000000000000 ) ) ;
#17846=CARTESIAN_POINT ( 'NONE',  ( -4.458734124999999437, -169.2500000013655779, -1.846868145590735644 ) ) ;
#17847=CARTESIAN_POINT ( 'NONE',  ( -4.458734124999999437, -26.39583333196774007, -2.574251347313719407 ) ) ;
#17851=CARTESIAN_POINT ( 'NONE',  ( 4.458734124999999437, -149.4375000013656063, 0.000000000000000000 ) ) ;
#17852=ORIENTED_EDGE ( 'NONE', *, *, #18155, .T. ) ;
#17854=CARTESIAN_POINT ( 'NONE',  ( -3.152548672688508926E-16, -49.81249999863440081, -5.148502694627439702 ) ) ;
#17856=CARTESIAN_POINT ( 'NONE',  ( 6.123233995736766282E-16, -170.0000000000000000, -5.000000000000000000 ) ) ;
#17857=CARTESIAN_POINT ( 'NONE',  ( -4.999999999999999112, 24.08333333333333215, 2.886751345948131764 ) ) ;
#17859=CARTESIAN_POINT ( 'NONE',  ( 4.458734124999999437, -0.8124999986344055847, -5.460374474430324690E-16 ) ) ;
#17860=CARTESIAN_POINT ( 'NONE',  ( 2.500000000000002220, 19.33333333333333570, 4.330127018922192761 ) ) ;
#17862=CARTESIAN_POINT ( 'NONE',  ( -1.339745962155613812, -74.20534180126145429, -5.000000000000000000 ) ) ;
#17863=CARTESIAN_POINT ( 'NONE',  ( 2.229367062499998831, 9.104166668032261711, -3.861377020970580887 ) ) ;
#17866=ORIENTED_EDGE ( 'NONE', *, *, #23328, .T. ) ;
#17867=CARTESIAN_POINT ( 'NONE',  ( -2.500000000000000444, -24.04166666393548368, -4.330127018922193649 ) ) ;
#17868=CARTESIAN_POINT ( 'NONE',  ( -4.458734124999999437, -49.31249999863440792, 0.000000000000000000 ) ) ;
#17869=CARTESIAN_POINT ( 'NONE',  ( 1.846868145590736310, -159.8750000013655779, 4.458734124999999437 ) ) ;
#17872=CARTESIAN_POINT ( 'NONE',  ( 1.060575238724906964E-15, -44.62499999726881583, 5.773502691896257311 ) ) ;
#17873=ORIENTED_EDGE ( 'NONE', *, *, #60583, .T. ) ;
#17874=CARTESIAN_POINT ( 'NONE',  ( 4.458734125000001214, -25.89583333196774007, 2.574251347313718519 ) ) ;
#17877=CARTESIAN_POINT ( 'NONE',  ( -1.846868145590734756, -165.1250000013656063, -4.458734125000000326 ) ) ;
#17878=( BOUNDED_CURVE ( )  B_SPLINE_CURVE ( 2, ( #16346, #41406, #12464, #35968, #41718, #12776, #26951, #61685, #16658 ),
 .UNSPECIFIED., .F., .F. ) 
 B_SPLINE_CURVE_WITH_KNOTS ( ( 3, 2, 2, 2, 3 ),
 ( 0.5604166666666666741, 0.5611111111111111160, 0.5625000000000000000, 0.5638888888888888840, 0.5645833333333333259 ),
 .UNSPECIFIED. ) 
 CURVE ( )  GEOMETRIC_REPRESENTATION_ITEM ( )  RATIONAL_B_SPLINE_CURVE ( ( 0.9330127018922194093, 0.9330127018922194093, 1.000000000000000000, 0.8660254037844387076, 1.000000000000000000, 0.8660254037844387076, 1.000000000000000000, 0.9330127018922194093, 0.9330127018922194093 ) ) 
 REPRESENTATION_ITEM ( '' )  );
#17879=CARTESIAN_POINT ( 'NONE',  ( 2.499999999999998668, -39.20833333060214443, -4.330127018922193649 ) ) ;
#17881=CARTESIAN_POINT ( 'NONE',  ( 9.457646018065525792E-16, -39.31249999863439371, 5.148502694627439702 ) ) ;
#17887=VERTEX_POINT ( 'NONE', #52741 ) ;
#17890=CARTESIAN_POINT ( 'NONE',  ( 4.458734125000001214, -87.14583333196772230, 2.574251347313718519 ) ) ;
#17892=CARTESIAN_POINT ( 'NONE',  ( 5.000000000000000000, -143.0625000000000000, 2.071067811865478614 ) ) ;
#17893=DIRECTION ( 'NONE',  ( 0.000000000000000000, 0.000000000000000000, 1.000000000000000000 ) ) ;
#17897=LINE ( 'NONE', #22104, #48417 ) ;
#17902=CARTESIAN_POINT ( 'NONE',  ( -4.458734124999999437, -86.56249999863439371, 0.000000000000000000 ) ) ;
#17906=ORIENTED_EDGE ( 'NONE', *, *, #29564, .F. ) ;
#17909=CARTESIAN_POINT ( 'NONE',  ( 5.000000000000000000, -167.1250000027312126, 0.000000000000000000 ) ) ;
#17911=CARTESIAN_POINT ( 'NONE',  ( -3.152548672688508926E-16, 11.18750000136559386, -5.148502694627439702 ) ) ;
#17912=CARTESIAN_POINT ( 'NONE',  ( -1.339745962155610925, -15.79465819873852261, 5.000000000000000000 ) ) ;
#17920=CARTESIAN_POINT ( 'NONE',  ( -3.152548672688508926E-16, -9.562499998634409692, -5.148502694627439702 ) ) ;
#17922=CARTESIAN_POINT ( 'NONE',  ( 4.458734125000000326, -33.14583333196774362, 2.574251347313718519 ) ) ;
#17927=CARTESIAN_POINT ( 'NONE',  ( -2.229367062500000163, 13.52083333469892779, -3.861377020970580443 ) ) ;
#17928=CARTESIAN_POINT ( 'NONE',  ( 5.000000000000000000, -55.41666666666667140, -2.886751345948130876 ) ) ;
#17929=CARTESIAN_POINT ( 'NONE',  ( 2.229367062500001939, -82.22916666530106511, 3.861377020970579999 ) ) ;
#17932=CARTESIAN_POINT ( 'NONE',  ( 5.000000000000000000, 19.62500000273118772, -6.123233995736766282E-16 ) ) ;
#17934=CARTESIAN_POINT ( 'NONE',  ( 3.535533905932738197, -147.0000000027311842, -3.535533905932738197 ) ) ;
#17937=CARTESIAN_POINT ( 'NONE',  ( 5.000000000000000000, -28.41666666666666430, -2.886751345948129988 ) ) ;
#17938=CARTESIAN_POINT ( 'NONE',  ( -2.229367062500000163, -33.47916666530107221, -3.861377020970580443 ) ) ;
#17939=CARTESIAN_POINT ( 'NONE',  ( 1.975475456537005874E-15, -1.749999999999999334, 5.000000000000000000 ) ) ;
#17940=CARTESIAN_POINT ( 'NONE',  ( -2.500000000000000444, -29.04166666393548013, -4.330127018922193649 ) ) ;
#17941=CARTESIAN_POINT ( 'NONE',  ( -4.458734124999998549, -58.22916666530105800, 2.574251347313722516 ) ) ;
#17942=ORIENTED_EDGE ( 'NONE', *, *, #36617, .F. ) ;
#17944=CARTESIAN_POINT ( 'NONE',  ( -4.458734124999999437, -10.64583333196773829, -2.574251347313719407 ) ) ;
#17945=ORIENTED_EDGE ( 'NONE', *, *, #58229, .F. ) ;
#17946=CARTESIAN_POINT ( 'NONE',  ( 1.060575238724906964E-15, -74.75000000000000000, 5.773502691896257311 ) ) ;
#17950=CARTESIAN_POINT ( 'NONE',  ( -3.535250795749689387E-16, -77.12499999726880162, -5.773502691896257311 ) ) ;
#17951=CARTESIAN_POINT ( 'NONE',  ( -9.184850993605147944E-16, -145.3750000027312126, 5.000000000000000000 ) ) ;
#17952=ORIENTED_EDGE ( 'NONE', *, *, #62555, .F. ) ;
#17954=CARTESIAN_POINT ( 'NONE',  ( -4.458734124999999437, -20.64583333196774007, -2.574251347313719407 ) ) ;
#17955=CARTESIAN_POINT ( 'NONE',  ( -3.152548672688508926E-16, -55.81249999863440081, -5.148502694627439702 ) ) ;
#17956=ORIENTED_EDGE ( 'NONE', *, *, #25193, .T. ) ;
#17957=AXIS2_PLACEMENT_3D ( 'NONE', #13757, #8003, #33379 ) ;
#17958=CARTESIAN_POINT ( 'NONE',  ( 4.458734124999999437, -142.4375000013656063, 0.000000000000000000 ) ) ;
#17960=CARTESIAN_POINT ( 'NONE',  ( -9.184850993605147944E-16, -148.3750000027312126, 5.000000000000000000 ) ) ;
#17961=EDGE_LOOP ( 'NONE', ( #20617, #34728, #5998, #54733 ) ) ;
#17966=CARTESIAN_POINT ( 'NONE',  ( -4.458734124999999437, -149.1875000013656063, -5.460374474430324690E-16 ) ) ;
#17970=CARTESIAN_POINT ( 'NONE',  ( 4.458734124999998549, -63.97916666530107221, -2.574251347313721627 ) ) ;
#17973=CARTESIAN_POINT ( 'NONE',  ( -4.458734124999999437, -142.0000000013655495, -1.846868145590735644 ) ) ;
#17980=DIRECTION ( 'NONE',  ( 0.000000000000000000, 0.000000000000000000, 1.000000000000000000 ) ) ;
#17983=CARTESIAN_POINT ( 'NONE',  ( 5.000000000000000888, -76.45833333060215864, 2.886751345948126879 ) ) ;
#17989=CARTESIAN_POINT ( 'NONE',  ( -3.152548672688508926E-16, 9.437500001365593860, -5.148502694627439702 ) ) ;
#17991=CARTESIAN_POINT ( 'NONE',  ( 4.458734124999999437, -19.06249999863440792, -5.460374474430324690E-16 ) ) ;
#17993=CARTESIAN_POINT ( 'NONE',  ( 1.846868145590736310, -159.6250000013656063, 4.458734124999999437 ) ) ;
#17997=ADVANCED_FACE ( 'NONE', ( #18002 ), #48532, .T. ) ;
#17999=( BOUNDED_CURVE ( )  B_SPLINE_CURVE ( 2, ( #59997, #14635, #34249, #54527, #15921, #45504, #25571, #40032, #19465 ),
 .UNSPECIFIED., .F., .F. ) 
 B_SPLINE_CURVE_WITH_KNOTS ( ( 3, 2, 2, 2, 3 ),
 ( 0.1895833333333333259, 0.1902777777777777679, 0.1916666666666666796, 0.1930555555555555636, 0.1937500000000000056 ),
 .UNSPECIFIED. ) 
 CURVE ( )  GEOMETRIC_REPRESENTATION_ITEM ( )  RATIONAL_B_SPLINE_CURVE ( ( 0.9330127018922194093, 0.9330127018922194093, 1.000000000000000000, 0.8660254037844387076, 1.000000000000000000, 0.8660254037844387076, 1.000000000000000000, 0.9330127018922194093, 0.9330127018922194093 ) ) 
 REPRESENTATION_ITEM ( '' )  );
#18001=CARTESIAN_POINT ( 'NONE',  ( -3.152548672688508926E-16, -42.56249999863439371, -5.148502694627439702 ) ) ;
#18002=FACE_OUTER_BOUND ( 'NONE', #25798, .T. ) ;
#18004=CARTESIAN_POINT ( 'NONE',  ( -4.458734124999999437, -66.64583333196773651, -2.574251347313719407 ) ) ;
#18006=CARTESIAN_POINT ( 'NONE',  ( 5.000000000000000000, -57.37499999726880162, -6.123233995736766282E-16 ) ) ;
#18007=CARTESIAN_POINT ( 'NONE',  ( 1.975475456537005874E-15, -89.74999999999998579, 5.000000000000000000 ) ) ;
#18008=ORIENTED_EDGE ( 'NONE', *, *, #59061, .F. ) ;
#18011=CARTESIAN_POINT ( 'NONE',  ( -4.999999999999999112, -11.91666666666666607, 2.886751345948131764 ) ) ;
#18012=CARTESIAN_POINT ( 'NONE',  ( 2.229367062499998831, -15.64583333196773651, -3.861377020970580887 ) ) ;
#18013=CARTESIAN_POINT ( 'NONE',  ( -4.458734124999999437, -79.39583333196773651, -2.574251347313719407 ) ) ;
#18014=CARTESIAN_POINT ( 'NONE',  ( 1.339745962155612702, -59.16965819600732601, -5.000000000000000000 ) ) ;
#18015=EDGE_CURVE ( 'NONE', #55065, #54054, #5461, .T. ) ;
#18016=CARTESIAN_POINT ( 'NONE',  ( 5.000000000000000888, -13.45833333060214976, 2.886751345948126879 ) ) ;
#18017=CARTESIAN_POINT ( 'NONE',  ( -2.229367062500000163, -45.47916666530106511, -3.861377020970580443 ) ) ;
#18018=ORIENTED_EDGE ( 'NONE', *, *, #1126, .T. ) ;
#18019=CARTESIAN_POINT ( 'NONE',  ( 1.339745962155615144, -41.70534180126147561, 4.999999999999999112 ) ) ;
#18020=EDGE_CURVE ( 'NONE', #19960, #49819, #23152, .T. ) ;
#18021=CARTESIAN_POINT ( 'NONE',  ( 4.458734124999998549, 8.020833334698926009, -2.574251347313721627 ) ) ;
#18022=VERTEX_POINT ( 'NONE', #53676 ) ;
#18024=CARTESIAN_POINT ( 'NONE',  ( 1.060575238724906964E-15, -61.75000000000000000, 5.773502691896257311 ) ) ;
#18025=CARTESIAN_POINT ( 'NONE',  ( -4.458734125000000326, -162.2500000013656347, -1.846868145590735644 ) ) ;
#18028=CARTESIAN_POINT ( 'NONE',  ( 2.229367062499998831, -82.64583333196773651, -3.861377020970580887 ) ) ;
#18029=CARTESIAN_POINT ( 'NONE',  ( 3.535533905932736864, -168.1250000000000284, 3.535533905932738641 ) ) ;
#18032=CARTESIAN_POINT ( 'NONE',  ( -4.458734124999998549, -4.479166665301070438, 2.574251347313722516 ) ) ;
#18034=CARTESIAN_POINT ( 'NONE',  ( 9.457646018065525792E-16, -42.31249999863440081, 5.148502694627439702 ) ) ;
#18035=CARTESIAN_POINT ( 'NONE',  ( 5.000000000000000000, -151.1875000027312410, 2.071067811865478614 ) ) ;
#18037=CYLINDRICAL_SURFACE ( 'NONE', #12219, 5.000000000000000000 ) ;
#18038=ORIENTED_EDGE ( 'NONE', *, *, #9096, .F. ) ;
#18039=CARTESIAN_POINT ( 'NONE',  ( 1.975475456537005874E-15, -47.74999999999999289, 5.000000000000000000 ) ) ;
#18040=CARTESIAN_POINT ( 'NONE',  ( -2.229367062499996610, -68.39583333196773651, 3.861377020970582219 ) ) ;
#18041=CARTESIAN_POINT ( 'NONE',  ( 4.458734124999999437, -145.6875000013656063, 0.000000000000000000 ) ) ;
#18042=ORIENTED_EDGE ( 'NONE', *, *, #44884, .F. ) ;
#18043=CARTESIAN_POINT ( 'NONE',  ( -5.147856630858197489E-14, 3.375000002731183280, 5.000000000000000000 ) ) ;
#18047=CARTESIAN_POINT ( 'NONE',  ( -4.999999999999998224, 3.083333333333333925, 2.886751345948131764 ) ) ;
#18048=CARTESIAN_POINT ( 'NONE',  ( 4.458734125000001214, 4.104166668032260823, 2.574251347313718519 ) ) ;
#18049=CARTESIAN_POINT ( 'NONE',  ( -1.339745962155613812, -80.20534180126148271, -5.000000000000000000 ) ) ;
#18050=CARTESIAN_POINT ( 'NONE',  ( -4.458734124999999437, -158.9375000013655779, -5.460374474430324690E-16 ) ) ;
#18053=EDGE_LOOP ( 'NONE', ( #53778, #46189, #6504, #59767 ) ) ;
#18058=LINE ( 'NONE', #47026, #10834 ) ;
#18059=CARTESIAN_POINT ( 'NONE',  ( -9.184850993605147944E-16, -166.3750000027312126, 5.000000000000000000 ) ) ;
#18065=CARTESIAN_POINT ( 'NONE',  ( 9.457646018065525792E-16, 21.93750000136559208, 5.148502694627439702 ) ) ;
#18067=CARTESIAN_POINT ( 'NONE',  ( 4.458734125000000326, -6.145833331967740953, 2.574251347313718519 ) ) ;
#18070=CARTESIAN_POINT ( 'NONE',  ( 2.071067811865475505, -139.9375000027311842, -5.000000000000000888 ) ) ;
#18071=DIRECTION ( 'NONE',  ( -0.000000000000000000, 1.000000000000000000, -0.000000000000000000 ) ) ;
#18072=AXIS2_PLACEMENT_3D ( 'NONE', #37069, #50901, #6843 ) ;
#18077=CARTESIAN_POINT ( 'NONE',  ( -1.339745962155613812, -87.20534180126148271, -5.000000000000000000 ) ) ;
#18081=CARTESIAN_POINT ( 'NONE',  ( -4.458734124999999437, -156.2500000013656063, -1.846868145590735644 ) ) ;
#18084=EDGE_LOOP ( 'NONE', ( #47365, #28050, #24174, #19116 ) ) ;
#18085=CARTESIAN_POINT ( 'NONE',  ( -4.458734124999999437, 17.43750000136559208, 0.000000000000000000 ) ) ;
#18090=CARTESIAN_POINT ( 'NONE',  ( 5.000000000000000888, -16.58333333333333215, 2.886751345948126879 ) ) ;
#18091=CARTESIAN_POINT ( 'NONE',  ( -5.000000000000000000, 4.916666666666666075, -2.886751345948128211 ) ) ;
#18093=CARTESIAN_POINT ( 'NONE',  ( 9.457646018065525792E-16, -61.06249999863440081, 5.148502694627439702 ) ) ;
#18096=CARTESIAN_POINT ( 'NONE',  ( -4.458734124999999437, -31.31249999863440436, 0.000000000000000000 ) ) ;
#18098=DIRECTION ( 'NONE',  ( -0.000000000000000000, 1.000000000000000000, -0.000000000000000000 ) ) ;
#18101=CARTESIAN_POINT ( 'NONE',  ( 2.499999999999998668, -39.33333333333332860, -4.330127018922193649 ) ) ;
#18102=CARTESIAN_POINT ( 'NONE',  ( 1.339745962155612702, -70.16965819600731891, -5.000000000000000000 ) ) ;
#18106=CARTESIAN_POINT ( 'NONE',  ( -2.229367062500000163, -65.47916666530106511, -3.861377020970580443 ) ) ;
#18108=CARTESIAN_POINT ( 'NONE',  ( 1.846868145590736310, -148.8750000013655495, 4.458734124999999437 ) ) ;
#18109=CARTESIAN_POINT ( 'NONE',  ( 2.229367062499998831, -77.64583333196773651, -3.861377020970580887 ) ) ;
#18111=CARTESIAN_POINT ( 'NONE',  ( 4.458734125000001214, -26.14583333196774007, 2.574251347313718519 ) ) ;
#18112=CARTESIAN_POINT ( 'NONE',  ( 2.499999999999998668, -68.20833333060214443, -4.330127018922193649 ) ) ;
#18113=ORIENTED_EDGE ( 'NONE', *, *, #2512, .F. ) ;
#18114=CARTESIAN_POINT ( 'NONE',  ( -2.499999999999996447, -21.83333333333332860, 4.330127018922195425 ) ) ;
#18115=ORIENTED_EDGE ( 'NONE', *, *, #42137, .F. ) ;
#18121=CARTESIAN_POINT ( 'NONE',  ( -5.000000000000000000, -74.95833333060214443, -2.886751345948128211 ) ) ;
#18122=CARTESIAN_POINT ( 'NONE',  ( 4.458734125000001214, -52.14583333196772941, 2.574251347313718519 ) ) ;
#18126=CARTESIAN_POINT ( 'NONE',  ( 9.457646018065525792E-16, 15.93750000136559564, 5.148502694627439702 ) ) ;
#18129=CARTESIAN_POINT ( 'NONE',  ( 4.458734124999999437, -169.3750000013656347, -1.846868145590734978 ) ) ;
#18133=CARTESIAN_POINT ( 'NONE',  ( -2.499999999999996447, -85.70833333060214443, 4.330127018922195425 ) ) ;
#18136=CARTESIAN_POINT ( 'NONE',  ( 0.000000000000000000, -170.0000000000000000, 5.000000000000000000 ) ) ;
#18139=CARTESIAN_POINT ( 'NONE',  ( 5.000000000000000000, 4.500000000000000888, -6.123233995736766282E-16 ) ) ;
#18148=CARTESIAN_POINT ( 'NONE',  ( 3.061616997868383141E-16, -154.8750000027311842, -5.000000000000000000 ) ) ;
#18154=CARTESIAN_POINT ( 'NONE',  ( -3.535533905932737309, -146.6250000000000000, -3.535533905932738197 ) ) ;
#18155=EDGE_CURVE ( 'NONE', #24664, #51343, #14115, .T. ) ;
#18159=CARTESIAN_POINT ( 'NONE',  ( -4.458734125000000326, -168.1250000013656063, 1.846868145590734089 ) ) ;
#18160=CARTESIAN_POINT ( 'NONE',  ( -4.458734124999999437, -30.31249999863440436, 0.000000000000000000 ) ) ;
#18163=CARTESIAN_POINT ( 'NONE',  ( 2.499999999999998668, 18.79166666939785202, -4.330127018922193649 ) ) ;
#18165=CARTESIAN_POINT ( 'NONE',  ( 4.458734124999999437, -148.5000000013656347, 1.846868145590737864 ) ) ;
#18166=ORIENTED_EDGE ( 'NONE', *, *, #57567, .F. ) ;
#18168=CARTESIAN_POINT ( 'NONE',  ( -4.458734124999997661, -56.47916666530107221, 2.574251347313722516 ) ) ;
#18171=CARTESIAN_POINT ( 'NONE',  ( 5.000000000000000000, 26.50000000000000000, -6.123233995736766282E-16 ) ) ;
#18173=EDGE_CURVE ( 'NONE', #52605, #60408, #48842, .T. ) ;
#18174=CARTESIAN_POINT ( 'NONE',  ( -6.972266317189433020E-16, -44.25000000000000000, -5.000000000000000000 ) ) ;
#18175=CARTESIAN_POINT ( 'NONE',  ( -2.229367062500000163, 0.5208333346989266754, -3.861377020970580443 ) ) ;
#18177=CARTESIAN_POINT ( 'NONE',  ( 4.458734124999999437, 7.937500001365595637, -5.460374474430324690E-16 ) ) ;
#18180=CARTESIAN_POINT ( 'NONE',  ( 5.000000000000000888, 26.41666666666666430, 2.886751345948126879 ) ) ;
#18181=VERTEX_POINT ( 'NONE', #40470 ) ;
#18183=CARTESIAN_POINT ( 'NONE',  ( 1.339745962155613146, 27.41965820146970145, 5.000000000000000888 ) ) ;
#18184=CARTESIAN_POINT ( 'NONE',  ( 4.458734124999999437, -46.81249999863440792, -5.460374474430324690E-16 ) ) ;
#18186=CARTESIAN_POINT ( 'NONE',  ( 1.846868145590736310, -161.8750000013656063, 4.458734124999999437 ) ) ;
#18191=CARTESIAN_POINT ( 'NONE',  ( 1.060575238724906964E-15, -50.62499999726881583, 5.773502691896257311 ) ) ;
#18193=CARTESIAN_POINT ( 'NONE',  ( -3.152548672688508926E-16, -24.56249999863440792, -5.148502694627439702 ) ) ;
#18194=EDGE_LOOP ( 'NONE', ( #37258, #30608, #10923, #23192 ) ) ;
#18196=CARTESIAN_POINT ( 'NONE',  ( 3.061616997868383141E-16, -142.8750000027312126, -5.000000000000000000 ) ) ;
#18197=CARTESIAN_POINT ( 'NONE',  ( 3.152801135295366208, -160.5625000013656063, 3.152801135295367985 ) ) ;
#18200=CARTESIAN_POINT ( 'NONE',  ( -4.458734124999998549, -40.47916666530107221, 2.574251347313722516 ) ) ;
#18204=CARTESIAN_POINT ( 'NONE',  ( 2.500000000000002220, -59.66666666666665719, 4.330127018922192761 ) ) ;
#18205=ORIENTED_EDGE ( 'NONE', *, *, #31092, .T. ) ;
#18208=CARTESIAN_POINT ( 'NONE',  ( -4.458734124999999437, -83.64583333196773651, -2.574251347313719407 ) ) ;
#18210=CARTESIAN_POINT ( 'NONE',  ( -1.339745962155613812, 24.91965820146970501, -5.000000000000000000 ) ) ;
#18212=CARTESIAN_POINT ( 'NONE',  ( -5.000000000000000000, -44.87499999726880873, 0.000000000000000000 ) ) ;
#18214=CARTESIAN_POINT ( 'NONE',  ( 5.000000000000000000, -37.41666666666666430, -2.886751345948130876 ) ) ;
#18216=DIRECTION ( 'NONE',  ( -0.000000000000000000, 1.000000000000000000, -0.000000000000000000 ) ) ;
#18219=DIRECTION ( 'NONE',  ( -0.000000000000000000, 1.000000000000000000, -0.000000000000000000 ) ) ;
#18221=CARTESIAN_POINT ( 'NONE',  ( 4.458734125000001214, -84.14583333196772230, 2.574251347313718519 ) ) ;
#18225=CARTESIAN_POINT ( 'NONE',  ( -6.972266317189433020E-16, 17.87500000273118417, -5.000000000000000000 ) ) ;
#18227=CARTESIAN_POINT ( 'NONE',  ( 5.000000000000000000, -164.1250000027311842, 0.000000000000000000 ) ) ;
#18230=CARTESIAN_POINT ( 'NONE',  ( -6.972266317189433020E-16, -16.25000000000000000, -5.000000000000000000 ) ) ;
#18237=CARTESIAN_POINT ( 'NONE',  ( -6.972266317189433020E-16, -86.12499999726880162, -5.000000000000000000 ) ) ;
#18238=CARTESIAN_POINT ( 'NONE',  ( 1.975475456537005874E-15, 17.25000000000000000, 5.000000000000000000 ) ) ;
#18239=CARTESIAN_POINT ( 'NONE',  ( 9.457646018065525792E-16, -11.06249999863440969, 5.148502694627439702 ) ) ;
#18241=ORIENTED_EDGE ( 'NONE', *, *, #18020, .T. ) ;
#18242=CARTESIAN_POINT ( 'NONE',  ( -3.152548672688508926E-16, -40.81249999863440081, -5.148502694627439702 ) ) ;
#18245=CARTESIAN_POINT ( 'NONE',  ( 6.123233995736766282E-16, -170.0000000000000000, -5.000000000000000000 ) ) ;
#18248=CARTESIAN_POINT ( 'NONE',  ( 4.458734124999999437, 17.18750000136559564, -5.460374474430324690E-16 ) ) ;
#18249=CARTESIAN_POINT ( 'NONE',  ( 0.000000000000000000, -170.0000000000000000, 0.000000000000000000 ) ) ;
#18250=CARTESIAN_POINT ( 'NONE',  ( 5.000000000000000000, -55.49999999999999289, -6.123233995736766282E-16 ) ) ;
#18251=CARTESIAN_POINT ( 'NONE',  ( 2.229367062499998831, -84.89583333196773651, -3.861377020970580887 ) ) ;
#18253=CARTESIAN_POINT ( 'NONE',  ( 2.499999999999998668, 15.79166666939785202, -4.330127018922193649 ) ) ;
#18255=CARTESIAN_POINT ( 'NONE',  ( 2.499999999999998668, -35.33333333333332860, -4.330127018922193649 ) ) ;
#18257=CARTESIAN_POINT ( 'NONE',  ( 5.000000000000000888, -52.58333333333332860, 2.886751345948126879 ) ) ;
#18258=CARTESIAN_POINT ( 'NONE',  ( 5.000000000000000000, -27.49999999999999645, -6.123233995736766282E-16 ) ) ;
#18259=CARTESIAN_POINT ( 'NONE',  ( 4.458734124999998549, -32.72916666530107221, -2.574251347313721627 ) ) ;
#18262=CARTESIAN_POINT ( 'NONE',  ( 2.499999999999998668, -28.20833333060214798, -4.330127018922193649 ) ) ;
#18263=CARTESIAN_POINT ( 'NONE',  ( 2.229367062500001939, -59.97916666530106511, 3.861377020970579999 ) ) ;
#18266=CARTESIAN_POINT ( 'NONE',  ( 2.229367062500001939, -8.229166665301073991, 3.861377020970579999 ) ) ;
#18268=CARTESIAN_POINT ( 'NONE',  ( 2.500000000000002220, -75.66666666666665719, 4.330127018922192761 ) ) ;
#18271=VECTOR ( 'NONE', #20688, 1000.000000000000000 ) ;
#18272=CARTESIAN_POINT ( 'NONE',  ( 5.000000000000000888, -78.45833333060214443, 2.886751345948126879 ) ) ;
#18276=AXIS2_PLACEMENT_3D ( 'NONE', #48288, #23549, #13256 ) ;
#18277=CARTESIAN_POINT ( 'NONE',  ( 4.458734124999999437, -23.06249999863440436, -5.460374474430324690E-16 ) ) ;
#18278=CARTESIAN_POINT ( 'NONE',  ( -3.152548672688508926E-16, -54.81249999863440081, -5.148502694627439702 ) ) ;
#18281=CARTESIAN_POINT ( 'NONE',  ( -4.458734125000001214, -169.1250000013656347, 1.846868145590734089 ) ) ;
#18292=CARTESIAN_POINT ( 'NONE',  ( -1.846868145590734756, -143.3750000013656063, -4.458734125000000326 ) ) ;
#18294=CARTESIAN_POINT ( 'NONE',  ( 0.000000000000000000, -170.0000000000000000, 0.000000000000000000 ) ) ;
#18296=CARTESIAN_POINT ( 'NONE',  ( -2.229367062499996610, -69.39583333196773651, 3.861377020970582219 ) ) ;
#18297=CARTESIAN_POINT ( 'NONE',  ( 1.975475456537005874E-15, -43.75000000000000000, 5.000000000000000000 ) ) ;
#18298=CARTESIAN_POINT ( 'NONE',  ( -4.999999999999998224, -42.79166666393548013, 2.886751345948131764 ) ) ;
#18299=CARTESIAN_POINT ( 'NONE',  ( 4.458734124999999437, -141.3750000013656063, -1.846868145590734978 ) ) ;
#18307=CARTESIAN_POINT ( 'NONE',  ( 9.457646018065525792E-16, 24.68750000136559208, 5.148502694627439702 ) ) ;
#18313=CARTESIAN_POINT ( 'NONE',  ( 0.000000000000000000, -170.0000000000000000, 0.000000000000000000 ) ) ;
#18314=CARTESIAN_POINT ( 'NONE',  ( -3.152548672688508926E-16, 6.437500001365592972, -5.148502694627439702 ) ) ;
#18316=CARTESIAN_POINT ( 'NONE',  ( -4.458734124999999437, -20.56249999863440081, 0.000000000000000000 ) ) ;
#18318=CARTESIAN_POINT ( 'NONE',  ( -8.190561711645485556E-16, -160.6875000013655779, 4.458734124999999437 ) ) ;
#18319=CARTESIAN_POINT ( 'NONE',  ( 5.000000000000000000, 23.58333333333333215, -2.886751345948130876 ) ) ;
#18322=AXIS2_PLACEMENT_3D ( 'NONE', #49079, #19814, #48455 ) ;
#18323=DIRECTION ( 'NONE',  ( -0.000000000000000000, 1.000000000000000000, -0.000000000000000000 ) ) ;
#18324=CARTESIAN_POINT ( 'NONE',  ( 4.458734124999998549, -42.72916666530107932, -2.574251347313721627 ) ) ;
#18327=CARTESIAN_POINT ( 'NONE',  ( -4.458734124999999437, -68.56249999863439371, 0.000000000000000000 ) ) ;
#18330=CARTESIAN_POINT ( 'NONE',  ( 2.500000000000002220, -89.66666666666665719, 4.330127018922192761 ) ) ;
#18333=CARTESIAN_POINT ( 'NONE',  ( 5.000000000000000888, 2.541666669397851130, 2.886751345948126879 ) ) ;
#18334=CARTESIAN_POINT ( 'NONE',  ( -2.499999999999996447, -13.83333333333333570, 4.330127018922195425 ) ) ;
#18335=CARTESIAN_POINT ( 'NONE',  ( 4.458734124999998549, -18.72916666530106866, -2.574251347313721627 ) ) ;
#18336=CARTESIAN_POINT ( 'NONE',  ( 2.229367062500001939, -77.97916666530106511, 3.861377020970579999 ) ) ;
#18339=CARTESIAN_POINT ( 'NONE',  ( 5.000000000000000888, -10.45833333060214621, 2.886751345948126879 ) ) ;
#18340=CARTESIAN_POINT ( 'NONE',  ( 2.229367062499998831, -45.64583333196774362, -3.861377020970580887 ) ) ;
#18342=CARTESIAN_POINT ( 'NONE',  ( 3.535533905932738197, -143.8750000000000000, -3.535533905932738197 ) ) ;
#18343=CARTESIAN_POINT ( 'NONE',  ( -2.229367062500000163, 7.270833334698929562, -3.861377020970580443 ) ) ;
#18345=CARTESIAN_POINT ( 'NONE',  ( 0.000000000000000000, -170.0000000000000000, 0.000000000000000000 ) ) ;
#18346=CARTESIAN_POINT ( 'NONE',  ( 2.500000000000002220, -60.66666666666665719, 4.330127018922192761 ) ) ;
#18347=CARTESIAN_POINT ( 'NONE',  ( 1.846868145590736310, -156.8750000013655779, 4.458734124999999437 ) ) ;
#18349=CARTESIAN_POINT ( 'NONE',  ( -1.339745962155610925, -55.79465819873851729, 5.000000000000000000 ) ) ;
#18350=CARTESIAN_POINT ( 'NONE',  ( 3.535533905932738197, -167.8750000000000284, -3.535533905932738197 ) ) ;
#18351=LINE ( 'NONE', #37975, #31313 ) ;
#18353=CARTESIAN_POINT ( 'NONE',  ( 4.458734124999998549, -5.979166665301073103, -2.574251347313721627 ) ) ;
#18354=CARTESIAN_POINT ( 'NONE',  ( 4.458734124999998549, -42.97916666530107221, -2.574251347313721627 ) ) ;
#18357=CARTESIAN_POINT ( 'NONE',  ( 5.000000000000000000, 8.500000000000000000, -6.123233995736766282E-16 ) ) ;
#18360=AXIS2_PLACEMENT_3D ( 'NONE', #49266, #24821, #33528 ) ;
#18361=CARTESIAN_POINT ( 'NONE',  ( -2.498395430326213474E-14, 21.37500000273118062, 5.000000000000000000 ) ) ;
#18362=CARTESIAN_POINT ( 'NONE',  ( -2.229367062500000163, -69.72916666530107932, -3.861377020970580443 ) ) ;
#18363=EDGE_CURVE ( 'NONE', #26556, #41789, #20690, .T. ) ;
#18365=CARTESIAN_POINT ( 'NONE',  ( 3.152801135295367541, -147.5625000013655779, -3.152801135295367541 ) ) ;
#18367=( BOUNDED_CURVE ( )  B_SPLINE_CURVE ( 2, ( #11389, #31009, #35526, #26838, #60938, #40981, #60623, #16543, #36166 ),
 .UNSPECIFIED., .F., .F. ) 
 B_SPLINE_CURVE_WITH_KNOTS ( ( 3, 2, 2, 2, 3 ),
 ( 0.7020833333333332815, 0.7027777777777777235, 0.7041666666666667185, 0.7055555555555556024, 0.7062500000000000444 ),
 .UNSPECIFIED. ) 
 CURVE ( )  GEOMETRIC_REPRESENTATION_ITEM ( )  RATIONAL_B_SPLINE_CURVE ( ( 0.9330127018922194093, 0.9330127018922194093, 1.000000000000000000, 0.8660254037844387076, 1.000000000000000000, 0.8660254037844387076, 1.000000000000000000, 0.9330127018922194093, 0.9330127018922194093 ) ) 
 REPRESENTATION_ITEM ( '' )  );
#18370=CARTESIAN_POINT ( 'NONE',  ( 1.975475456537005874E-15, -79.62499999726881583, 5.000000000000000000 ) ) ;
#18371=CARTESIAN_POINT ( 'NONE',  ( -2.229367062500000163, 0.5208333346989266754, -3.861377020970580443 ) ) ;
#18373=CARTESIAN_POINT ( 'NONE',  ( -4.458734124999999437, -152.0000000013656063, -1.846868145590735644 ) ) ;
#18375=ORIENTED_EDGE ( 'NONE', *, *, #12995, .T. ) ;
#18378=CARTESIAN_POINT ( 'NONE',  ( 5.000000000000000888, -63.58333333333332860, 2.886751345948126879 ) ) ;
#18381=AXIS2_PLACEMENT_3D ( 'NONE', #1811, #59700, #34591 ) ;
#18383=( BOUNDED_CURVE ( )  B_SPLINE_CURVE ( 2, ( #39329, #50268, #25503, #34842, #29349, #30001, #58962, #11024, #761 ),
 .UNSPECIFIED., .F., .F. ) 
 B_SPLINE_CURVE_WITH_KNOTS ( ( 3, 2, 2, 2, 3 ),
 ( 0.7583333333333330817, 0.7624999999999997335, 0.7666666666666664964, 0.7708333333333331483, 0.7749999999999998002 ),
 .UNSPECIFIED. ) 
 CURVE ( )  GEOMETRIC_REPRESENTATION_ITEM ( )  RATIONAL_B_SPLINE_CURVE ( ( 1.000000000000003997, 0.9238795325112826307, 1.000000000000000000, 0.9238795325112867385, 1.000000000000000000, 0.9238795325112867385, 1.000000000000000000, 0.9238795325112908463, 0.9999999999999958922 ) ) 
 REPRESENTATION_ITEM ( '' )  );
#18384=CARTESIAN_POINT ( 'NONE',  ( 5.000000000000000000, -87.41666666666667140, -2.886751345948130876 ) ) ;
#18389=CARTESIAN_POINT ( 'NONE',  ( 2.229367062499998831, 23.35416666803225993, -3.861377020970580887 ) ) ;
#18391=CARTESIAN_POINT ( 'NONE',  ( -4.458734124999997661, -4.479166665301070438, 2.574251347313722516 ) ) ;
#18392=CARTESIAN_POINT ( 'NONE',  ( -5.000000000000000000, -33.95833333060213732, -2.886751345948128211 ) ) ;
#18394=CARTESIAN_POINT ( 'NONE',  ( -5.000000000000000000, -141.6250000027312126, -6.123233995736766282E-16 ) ) ;
#18395=CARTESIAN_POINT ( 'NONE',  ( -1.339745962155660663, -20.66965819600733667, 4.999999999999972466 ) ) ;
#18402=CARTESIAN_POINT ( 'NONE',  ( 1.846868145590735200, -156.5000000013656347, -4.458734124999999437 ) ) ;
#18404=CYLINDRICAL_SURFACE ( 'NONE', #8949, 5.000000000000000000 ) ;
#18405=ORIENTED_EDGE ( 'NONE', *, *, #55792, .T. ) ;
#18406=CARTESIAN_POINT ( 'NONE',  ( -2.229367062499996610, 16.60416666803225638, 3.861377020970582219 ) ) ;
#18412=CARTESIAN_POINT ( 'NONE',  ( -2.500000000000000444, -88.04166666393548724, -4.330127018922193649 ) ) ;
#18413=CARTESIAN_POINT ( 'NONE',  ( 2.500000000000002220, 5.333333333333332149, 4.330127018922192761 ) ) ;
#18414=CARTESIAN_POINT ( 'NONE',  ( -4.458734124999999437, -59.31249999863440081, 0.000000000000000000 ) ) ;
#18415=CARTESIAN_POINT ( 'NONE',  ( -4.999999999999999112, 4.208333336064518093, 2.886751345948131764 ) ) ;
#18416=CARTESIAN_POINT ( 'NONE',  ( -4.458734124999999437, -26.39583333196773651, -2.574251347313719407 ) ) ;
#18419=CARTESIAN_POINT ( 'NONE',  ( -2.071067811865308972, -151.4375000027312126, 5.000000000000169642 ) ) ;
#18420=CARTESIAN_POINT ( 'NONE',  ( 5.000000000000000888, -44.58333333333333570, 2.886751345948126879 ) ) ;
#18424=CARTESIAN_POINT ( 'NONE',  ( -4.458734124999999437, -65.39583333196773651, -2.574251347313719407 ) ) ;
#18425=CARTESIAN_POINT ( 'NONE',  ( 1.846868145590735200, -146.5000000013656347, -4.458734125000000326 ) ) ;
#18426=CARTESIAN_POINT ( 'NONE',  ( -2.229367062499996610, -78.14583333196773651, 3.861377020970582219 ) ) ;
#18429=CARTESIAN_POINT ( 'NONE',  ( -4.458734124999999437, -22.64583333196773296, -2.574251347313719407 ) ) ;
#18430=CARTESIAN_POINT ( 'NONE',  ( 5.000000000000000000, -64.37499999726881583, -6.123233995736766282E-16 ) ) ;
#18432=CARTESIAN_POINT ( 'NONE',  ( -2.071067811865686448, -152.8125000027312126, -4.999999999999789502 ) ) ;
#18433=ORIENTED_EDGE ( 'NONE', *, *, #36761, .F. ) ;
#18435=CARTESIAN_POINT ( 'NONE',  ( 3.061616997868383141E-16, -148.8750000027312126, -5.000000000000000000 ) ) ;
#18437=ORIENTED_EDGE ( 'NONE', *, *, #48806, .F. ) ;
#18438=( BOUNDED_CURVE ( )  B_SPLINE_CURVE ( 2, ( #43827, #38383, #4597, #48348, #8803, #34180, #58324, #23607, #15205 ),
 .UNSPECIFIED., .F., .F. ) 
 B_SPLINE_CURVE_WITH_KNOTS ( ( 3, 2, 2, 2, 3 ),
 ( 0.2083333333333335091, 0.2125000000000001610, 0.2166666666666668406, 0.2208333333333335202, 0.2250000000000001998 ),
 .UNSPECIFIED. ) 
 CURVE ( )  GEOMETRIC_REPRESENTATION_ITEM ( )  RATIONAL_B_SPLINE_CURVE ( ( 0.9999999999999970024, 0.9238795325112897361, 1.000000000000000000, 0.9238795325112867385, 1.000000000000000000, 0.9238795325112867385, 1.000000000000000000, 0.9238795325112831858, 1.000000000000003553 ) ) 
 REPRESENTATION_ITEM ( '' )  );
#18439=CARTESIAN_POINT ( 'NONE',  ( -5.000000000000000000, -3.000000000000002665, 0.000000000000000000 ) ) ;
#18440=CARTESIAN_POINT ( 'NONE',  ( -4.458734124999999437, -54.64583333196774362, -2.574251347313719407 ) ) ;
#18444=LINE ( 'NONE', #48025, #55293 ) ;
#18446=CARTESIAN_POINT ( 'NONE',  ( -2.229367062499996610, 18.85416666803225993, 3.861377020970582219 ) ) ;
#18449=CARTESIAN_POINT ( 'NONE',  ( 3.152801135295366208, -165.5625000013656063, 3.152801135295367985 ) ) ;
#18453=EDGE_CURVE ( 'NONE', #25022, #13616, #18611, .T. ) ;
#18454=CARTESIAN_POINT ( 'NONE',  ( 1.975475456537005874E-15, -39.75000000000000000, 5.000000000000000000 ) ) ;
#18457=FACE_OUTER_BOUND ( 'NONE', #35853, .T. ) ;
#18460=EDGE_CURVE ( 'NONE', #29728, #13416, #56871, .T. ) ;
#18464=CARTESIAN_POINT ( 'NONE',  ( -9.184850993605147944E-16, -156.2500000000000000, 5.000000000000000000 ) ) ;
#18465=CARTESIAN_POINT ( 'NONE',  ( -5.000000000000000888, -159.5625000000000853, -2.071067811865475949 ) ) ;
#18467=( BOUNDED_CURVE ( )  B_SPLINE_CURVE ( 2, ( #47062, #32899, #21986, #52524, #51575, #41579, #28066, #7513, #8148 ),
 .UNSPECIFIED., .F., .F. ) 
 B_SPLINE_CURVE_WITH_KNOTS ( ( 3, 2, 2, 2, 3 ),
 ( 0.5562500000000000222, 0.5569444444444444642, 0.5583333333333333481, 0.5597222222222222321, 0.5604166666666666741 ),
 .UNSPECIFIED. ) 
 CURVE ( )  GEOMETRIC_REPRESENTATION_ITEM ( )  RATIONAL_B_SPLINE_CURVE ( ( 0.9330127018922194093, 0.9330127018922194093, 1.000000000000000000, 0.8660254037844387076, 1.000000000000000000, 0.8660254037844387076, 1.000000000000000000, 0.9330127018922194093, 0.9330127018922194093 ) ) 
 REPRESENTATION_ITEM ( '' )  );
#18469=DIRECTION ( 'NONE',  ( -0.000000000000000000, 1.000000000000000000, -0.000000000000000000 ) ) ;
#18471=CARTESIAN_POINT ( 'NONE',  ( 5.000000000000000888, -152.0625000027311842, -2.071067811865475505 ) ) ;
#18477=CARTESIAN_POINT ( 'NONE',  ( -2.071067811865478170, -143.3125000000000000, 5.000000000000000000 ) ) ;
#18481=CARTESIAN_POINT ( 'NONE',  ( -4.458734124999997661, -29.22916666530107221, 2.574251347313722516 ) ) ;
#18485=CARTESIAN_POINT ( 'NONE',  ( 1.846868145590735200, -146.2500000013656063, -4.458734125000000326 ) ) ;
#18486=ORIENTED_EDGE ( 'NONE', *, *, #62834, .T. ) ;
#18488=CARTESIAN_POINT ( 'NONE',  ( 4.458734124999999437, -59.06249999863440081, -5.460374474430324690E-16 ) ) ;
#18490=( BOUNDED_CURVE ( )  B_SPLINE_CURVE ( 2, ( #18454, #3046, #33247, #43200, #22664, #61903, #8491, #8181, #37759 ),
 .UNSPECIFIED., .F., .F. ) 
 B_SPLINE_CURVE_WITH_KNOTS ( ( 3, 2, 2, 2, 3 ),
 ( 0.5812500000000000444, 0.5819444444444444864, 0.5833333333333333703, 0.5847222222222222543, 0.5854166666666666963 ),
 .UNSPECIFIED. ) 
 CURVE ( )  GEOMETRIC_REPRESENTATION_ITEM ( )  RATIONAL_B_SPLINE_CURVE ( ( 0.9330127018922194093, 0.9330127018922194093, 1.000000000000000000, 0.8660254037844387076, 1.000000000000000000, 0.8660254037844387076, 1.000000000000000000, 0.9330127018922194093, 0.9330127018922194093 ) ) 
 REPRESENTATION_ITEM ( '' )  );
#18492=CARTESIAN_POINT ( 'NONE',  ( -5.000000000000000000, 20.91666666666666785, -2.886751345948128211 ) ) ;
#18493=EDGE_CURVE ( 'NONE', #42348, #61074, #42462, .T. ) ;
#18495=CARTESIAN_POINT ( 'NONE',  ( 2.229367062500001939, 0.02083333469892964529, 3.861377020970579999 ) ) ;
#18497=DIRECTION ( 'NONE',  ( -0.000000000000000000, 1.000000000000000000, -0.000000000000000000 ) ) ;
#18498=CARTESIAN_POINT ( 'NONE',  ( -4.458734124999999437, 8.354166668032261711, -2.574251347313719407 ) ) ;
#18499=EDGE_CURVE ( 'NONE', #27206, #11807, #7665, .T. ) ;
#18500=DIRECTION ( 'NONE',  ( 0.000000000000000000, 0.000000000000000000, 1.000000000000000000 ) ) ;
#18502=CARTESIAN_POINT ( 'NONE',  ( -4.999999999999998224, -23.79166666393548368, 2.886751345948131764 ) ) ;
#18503=CARTESIAN_POINT ( 'NONE',  ( -4.458734124999998549, -51.22916666530107221, 2.574251347313722516 ) ) ;
#18504=CARTESIAN_POINT ( 'NONE',  ( 2.730187237215162345E-16, -158.4375000013655779, -4.458734124999999437 ) ) ;
#18506=CARTESIAN_POINT ( 'NONE',  ( -2.500000000000000444, -50.04166666393547303, -4.330127018922193649 ) ) ;
#18507=ORIENTED_EDGE ( 'NONE', *, *, #56408, .F. ) ;
#18508=CARTESIAN_POINT ( 'NONE',  ( 9.457646018065525792E-16, -21.06249999863440436, 5.148502694627439702 ) ) ;
#18509=ORIENTED_EDGE ( 'NONE', *, *, #20789, .T. ) ;
#18510=CARTESIAN_POINT ( 'NONE',  ( 0.000000000000000000, -170.0000000000000000, 5.000000000000000000 ) ) ;
#18511=CARTESIAN_POINT ( 'NONE',  ( -1.846868145590737420, -160.7500000013655779, 4.458734124999999437 ) ) ;
#18512=ORIENTED_EDGE ( 'NONE', *, *, #50779, .T. ) ;
#18515=CARTESIAN_POINT ( 'NONE',  ( -4.458734124999999437, -36.56249999863440792, 0.000000000000000000 ) ) ;
#18516=VERTEX_POINT ( 'NONE', #36929 ) ;
#18525=CARTESIAN_POINT ( 'NONE',  ( -4.458734124999998549, -86.47916666530107932, 2.574251347313722516 ) ) ;
#18528=CARTESIAN_POINT ( 'NONE',  ( -4.458734124999999437, -140.1875000013656063, -5.460374474430324690E-16 ) ) ;
#18529=CARTESIAN_POINT ( 'NONE',  ( 5.000000000000000000, -145.1875000027312410, 2.071067811865478614 ) ) ;
#18531=CARTESIAN_POINT ( 'NONE',  ( -2.500000000000000444, -85.04166666393547303, -4.330127018922193649 ) ) ;
#18535=DIRECTION ( 'NONE',  ( -0.000000000000000000, 1.000000000000000000, -0.000000000000000000 ) ) ;
#18538=FACE_OUTER_BOUND ( 'NONE', #60438, .T. ) ;
#18541=CARTESIAN_POINT ( 'NONE',  ( 4.458734125000001214, -86.14583333196775072, 2.574251347313718519 ) ) ;
#18547=CARTESIAN_POINT ( 'NONE',  ( -9.184850993605147944E-16, -166.3750000027312126, 5.000000000000000000 ) ) ;
#18556=DIRECTION ( 'NONE',  ( -0.000000000000000000, 1.000000000000000000, -0.000000000000000000 ) ) ;
#18557=CARTESIAN_POINT ( 'NONE',  ( -4.458734124999997661, -16.22916666530107577, 2.574251347313722516 ) ) ;
#18558=CARTESIAN_POINT ( 'NONE',  ( -6.972266317189433020E-16, 18.87500000273118772, -5.000000000000000000 ) ) ;
#18559=ORIENTED_EDGE ( 'NONE', *, *, #1280, .T. ) ;
#18560=CARTESIAN_POINT ( 'NONE',  ( 9.457646018065525792E-16, -42.31249999863440081, 5.148502694627439702 ) ) ;
#18561=CARTESIAN_POINT ( 'NONE',  ( -6.972266317189433020E-16, -83.12499999726878741, -5.000000000000000000 ) ) ;
#18562=CARTESIAN_POINT ( 'NONE',  ( 5.000000000000000000, 0.7083333360645185373, -2.886751345948130876 ) ) ;
#18563=CARTESIAN_POINT ( 'NONE',  ( -1.339745962155613812, 26.91965820146970501, -5.000000000000000000 ) ) ;
#18567=CARTESIAN_POINT ( 'NONE',  ( -4.458734124999998549, 16.77083333469892779, 2.574251347313722516 ) ) ;
#18570=CARTESIAN_POINT ( 'NONE',  ( 9.457646018065525792E-16, -89.31249999863440792, 5.148502694627439702 ) ) ;
#18572=CARTESIAN_POINT ( 'NONE',  ( -2.499999999999996447, 11.29166666939785202, 4.330127018922195425 ) ) ;
#18573=ORIENTED_EDGE ( 'NONE', *, *, #30109, .T. ) ;
#18574=CARTESIAN_POINT ( 'NONE',  ( 1.975475456537005874E-15, -79.74999999999998579, 5.000000000000000000 ) ) ;
#18576=CARTESIAN_POINT ( 'NONE',  ( -9.184850993605147944E-16, -159.3750000027311842, 5.000000000000000000 ) ) ;
#18577=CARTESIAN_POINT ( 'NONE',  ( 5.000000000000000000, -26.41666666666666430, -2.886751345948129988 ) ) ;
#18578=CARTESIAN_POINT ( 'NONE',  ( 2.229367062499998831, -34.64583333196772941, -3.861377020970580887 ) ) ;
#18579=CARTESIAN_POINT ( 'NONE',  ( -5.000000000000000000, -31.87499999726880873, 0.000000000000000000 ) ) ;
#18580=CARTESIAN_POINT ( 'NONE',  ( 2.229367062499998831, -62.64583333196774362, -3.861377020970580887 ) ) ;
#18583=CARTESIAN_POINT ( 'NONE',  ( -3.152548672688508926E-16, -7.812499998634405252, -5.148502694627439702 ) ) ;
#18584=ORIENTED_EDGE ( 'NONE', *, *, #4027, .F. ) ;
#18585=CARTESIAN_POINT ( 'NONE',  ( 5.000000000000000000, -74.50000000000000000, -6.123233995736766282E-16 ) ) ;
#18586=CARTESIAN_POINT ( 'NONE',  ( 5.000000000000000000, 28.62500000273118417, -6.123233995736766282E-16 ) ) ;
#18588=CARTESIAN_POINT ( 'NONE',  ( 2.499999999999998668, -81.20833333060213022, -4.330127018922193649 ) ) ;
#18593=CARTESIAN_POINT ( 'NONE',  ( -4.458734124999999437, -20.56249999863440081, 0.000000000000000000 ) ) ;
#18594=CARTESIAN_POINT ( 'NONE',  ( 9.457646018065525792E-16, -57.31249999863440081, 5.148502694627439702 ) ) ;
#18595=EDGE_LOOP ( 'NONE', ( #23586, #50215, #30090, #21841 ) ) ;
#18598=CARTESIAN_POINT ( 'NONE',  ( -1.846868145590734756, -166.3750000013655779, -4.458734125000000326 ) ) ;
#18600=CARTESIAN_POINT ( 'NONE',  ( 1.339745962155615144, -50.58034179853029144, 4.999999999999999112 ) ) ;
#18601=VERTEX_POINT ( 'NONE', #13424 ) ;
#18607=CARTESIAN_POINT ( 'NONE',  ( 1.846868145590735200, -143.5000000013656063, -4.458734125000000326 ) ) ;
#18611=( BOUNDED_CURVE ( )  B_SPLINE_CURVE ( 2, ( #1578, #26316, #46898, #2217, #40785, #51091, #42055, #60432, #12158 ),
 .UNSPECIFIED., .F., .F. ) 
 B_SPLINE_CURVE_WITH_KNOTS ( ( 3, 2, 2, 2, 3 ),
 ( 0.6937499999999999778, 0.6944444444444444198, 0.6958333333333333037, 0.6972222222222221877, 0.6979166666666666297 ),
 .UNSPECIFIED. ) 
 CURVE ( )  GEOMETRIC_REPRESENTATION_ITEM ( )  RATIONAL_B_SPLINE_CURVE ( ( 0.9330127018922194093, 0.9330127018922194093, 1.000000000000000000, 0.8660254037844387076, 1.000000000000000000, 0.8660254037844387076, 1.000000000000000000, 0.9330127018922194093, 0.9330127018922194093 ) ) 
 REPRESENTATION_ITEM ( '' )  );
#18612=CARTESIAN_POINT ( 'NONE',  ( 4.458734125000001214, -71.14583333196773651, 2.574251347313718519 ) ) ;
#18616=CARTESIAN_POINT ( 'NONE',  ( 2.499999999999998668, -68.33333333333332860, -4.330127018922193649 ) ) ;
#18618=ORIENTED_EDGE ( 'NONE', *, *, #18015, .F. ) ;
#18619=CARTESIAN_POINT ( 'NONE',  ( -6.972266317189433020E-16, -71.12499999726878741, -5.000000000000000000 ) ) ;
#18620=EDGE_CURVE ( 'NONE', #43870, #18978, #38335, .T. ) ;
#18626=CARTESIAN_POINT ( 'NONE',  ( 4.458734124999999437, 24.93750000136559208, -5.460374474430324690E-16 ) ) ;
#18629=EDGE_CURVE ( 'NONE', #29232, #3859, #32728, .T. ) ;
#18633=CARTESIAN_POINT ( 'NONE',  ( 2.500000000000002220, -60.54166666393547303, 4.330127018922192761 ) ) ;
#18634=CARTESIAN_POINT ( 'NONE',  ( -2.229367062500000163, -0.4791666653010707710, -3.861377020970580443 ) ) ;
#18635=CARTESIAN_POINT ( 'NONE',  ( 4.458734125000000326, -25.14583333196774007, 2.574251347313718519 ) ) ;
#18636=CARTESIAN_POINT ( 'NONE',  ( 3.152801135295367541, -154.3125000013656063, -3.152801135295367541 ) ) ;
#18642=CARTESIAN_POINT ( 'NONE',  ( 4.458734124999998549, -69.97916666530107932, -2.574251347313721627 ) ) ;
#18644=FACE_OUTER_BOUND ( 'NONE', #34297, .T. ) ;
#18645=CARTESIAN_POINT ( 'NONE',  ( -2.499999999999996447, 27.29166666939785202, 4.330127018922195425 ) ) ;
#18647=AXIS2_PLACEMENT_3D ( 'NONE', #12738, #51983, #7925 ) ;
#18649=CARTESIAN_POINT ( 'NONE',  ( 5.000000000000000888, -10.58333333333333393, 2.886751345948126879 ) ) ;
#18650=CARTESIAN_POINT ( 'NONE',  ( 2.229367062500001939, -16.97916666530106866, 3.861377020970579999 ) ) ;
#18651=CARTESIAN_POINT ( 'NONE',  ( 4.458734124999999437, -76.81249999863440792, -5.460374474430324690E-16 ) ) ;
#18652=CARTESIAN_POINT ( 'NONE',  ( 1.339745962155615144, -59.58034179853028434, 4.999999999999999112 ) ) ;
#18653=CARTESIAN_POINT ( 'NONE',  ( 5.000000000000000888, -17.45833333060214443, 2.886751345948126879 ) ) ;
#18654=CARTESIAN_POINT ( 'NONE',  ( -4.458734124999999437, -46.39583333196774362, -2.574251347313719407 ) ) ;
#18655=ORIENTED_EDGE ( 'NONE', *, *, #54347, .F. ) ;
#18656=CARTESIAN_POINT ( 'NONE',  ( 5.000000000000000000, -15.37499999726881228, -6.123233995736766282E-16 ) ) ;
#18657=CARTESIAN_POINT ( 'NONE',  ( 2.229367062500001939, 6.770833334698928674, 3.861377020970579999 ) ) ;
#18658=ORIENTED_EDGE ( 'NONE', *, *, #51133, .T. ) ;
#18660=CARTESIAN_POINT ( 'NONE',  ( 2.500000000000002220, -61.66666666666666430, 4.330127018922192761 ) ) ;
#18661=CARTESIAN_POINT ( 'NONE',  ( 2.730187237215162345E-16, -155.4375000013655779, -4.458734124999999437 ) ) ;
#18663=( BOUNDED_CURVE ( )  B_SPLINE_CURVE ( 2, ( #61592, #17195, #37145, #32621, #52247, #12375, #27790, #7556, #46471 ),
 .UNSPECIFIED., .F., .F. ) 
 B_SPLINE_CURVE_WITH_KNOTS ( ( 3, 2, 2, 2, 3 ),
 ( 0.2916666666666669072, 0.2958333333333335591, 0.3000000000000002665, 0.3041666666666669183, 0.3083333333333336257 ),
 .UNSPECIFIED. ) 
 CURVE ( )  GEOMETRIC_REPRESENTATION_ITEM ( )  RATIONAL_B_SPLINE_CURVE ( ( 0.9999999999999958922, 0.9238795325112908463, 1.000000000000000000, 0.9238795325112867385, 1.000000000000000000, 0.9238795325112867385, 1.000000000000000000, 0.9238795325112816315, 1.000000000000005107 ) ) 
 REPRESENTATION_ITEM ( '' )  );
#18664=CARTESIAN_POINT ( 'NONE',  ( 5.000000000000000888, -165.9375000000000000, -2.071067811865475505 ) ) ;
#18665=CARTESIAN_POINT ( 'NONE',  ( 2.500000000000002220, -11.66666666666666607, 4.330127018922192761 ) ) ;
#18667=CARTESIAN_POINT ( 'NONE',  ( -4.458734124999998549, -6.479166665301073103, 2.574251347313722516 ) ) ;
#18668=CARTESIAN_POINT ( 'NONE',  ( -4.458734124999998549, -40.47916666530107221, 2.574251347313722516 ) ) ;
#18670=CARTESIAN_POINT ( 'NONE',  ( -3.152801135295367985, -149.8125000013655779, 3.152801135295367096 ) ) ;
#18675=CARTESIAN_POINT ( 'NONE',  ( 4.458734125000001214, -74.14583333196773651, 2.574251347313718519 ) ) ;
#18680=CARTESIAN_POINT ( 'NONE',  ( -2.229367062499996610, 1.854166668032262377, 3.861377020970582219 ) ) ;
#18681=CARTESIAN_POINT ( 'NONE',  ( -1.339745962155610925, -42.79465819873851729, 5.000000000000000000 ) ) ;
#18682=CARTESIAN_POINT ( 'NONE',  ( 3.152801135295367541, -151.3125000013655779, -3.152801135295367541 ) ) ;
#18684=VERTEX_POINT ( 'NONE', #23719 ) ;
#18686=CARTESIAN_POINT ( 'NONE',  ( -1.339745962155613812, -47.20534180126147561, -5.000000000000000000 ) ) ;
#18690=CARTESIAN_POINT ( 'NONE',  ( 2.499999999999998668, -23.20833333060214443, -4.330127018922193649 ) ) ;
#18693=CARTESIAN_POINT ( 'NONE',  ( -6.972266317189433020E-16, -64.12499999726880162, -5.000000000000000000 ) ) ;
#18696=CARTESIAN_POINT ( 'NONE',  ( 4.458734125000000326, 24.10416666803225993, 2.574251347313718519 ) ) ;
#18698=CARTESIAN_POINT ( 'NONE',  ( 4.458734125000000326, -11.14583333196773829, 2.574251347313718519 ) ) ;
#18701=CARTESIAN_POINT ( 'NONE',  ( 1.846868145590735200, -168.2500000013656063, -4.458734125000000326 ) ) ;
#18709=CARTESIAN_POINT ( 'NONE',  ( -4.458734124999999437, -158.1875000013655779, -5.460374474430324690E-16 ) ) ;
#18719=CARTESIAN_POINT ( 'NONE',  ( -5.000000000000000000, 3.916666666666665630, -2.886751345948128211 ) ) ;
#18720=ADVANCED_FACE ( 'NONE', ( #33050 ), #3468, .T. ) ;
#18721=CARTESIAN_POINT ( 'NONE',  ( 2.229367062500001939, -60.97916666530106511, 3.861377020970579999 ) ) ;
#18723=CARTESIAN_POINT ( 'NONE',  ( 5.000000000000000000, 1.625000002731184834, -6.123233995736766282E-16 ) ) ;
#18724=CARTESIAN_POINT ( 'NONE',  ( 4.458734124999998549, -29.72916666530107221, -2.574251347313721627 ) ) ;
#18725=CARTESIAN_POINT ( 'NONE',  ( -2.499999999999996447, -41.83333333333333570, 4.330127018922195425 ) ) ;
#18727=CARTESIAN_POINT ( 'NONE',  ( -4.999999999999999112, -42.91666666666665719, 2.886751345948131764 ) ) ;
#18728=CARTESIAN_POINT ( 'NONE',  ( -6.972266317189433020E-16, -19.12499999726880873, -5.000000000000000000 ) ) ;
#18731=CARTESIAN_POINT ( 'NONE',  ( -3.152548672688508926E-16, -70.56249999863439371, -5.148502694627439702 ) ) ;
#18732=CARTESIAN_POINT ( 'NONE',  ( 3.152801135295366208, -149.8125000013655779, 3.152801135295367985 ) ) ;
#18733=CARTESIAN_POINT ( 'NONE',  ( 4.458734124999998549, -77.72916666530106511, -2.574251347313721627 ) ) ;
#18736=CARTESIAN_POINT ( 'NONE',  ( 4.458734125000001214, -23.14583333196773651, 2.574251347313718519 ) ) ;
#18737=CARTESIAN_POINT ( 'NONE',  ( 2.500000000000002220, -66.54166666393547303, 4.330127018922192761 ) ) ;
#18739=CARTESIAN_POINT ( 'NONE',  ( -1.339745962155610925, -21.79465819873851729, 5.000000000000000000 ) ) ;
#18740=VERTEX_POINT ( 'NONE', #19181 ) ;
#18742=CARTESIAN_POINT ( 'NONE',  ( 1.975475456537005874E-15, 8.375000002731187720, 5.000000000000000000 ) ) ;
#18744=FACE_OUTER_BOUND ( 'NONE', #40475, .T. ) ;
#18745=CARTESIAN_POINT ( 'NONE',  ( -4.458734124999998549, -55.47916666530107221, 2.574251347313722516 ) ) ;
#18747=VERTEX_POINT ( 'NONE', #38794 ) ;
#18748=( BOUNDED_CURVE ( )  B_SPLINE_CURVE ( 2, ( #20834, #7632, #61345, #27547, #17597, #16956, #56199, #22425, #12756 ),
 .UNSPECIFIED., .F., .F. ) 
 B_SPLINE_CURVE_WITH_KNOTS ( ( 3, 2, 2, 2, 3 ),
 ( 0.2145833333333333481, 0.2152777777777777901, 0.2166666666666666741, 0.2180555555555555580, 0.2187500000000000000 ),
 .UNSPECIFIED. ) 
 CURVE ( )  GEOMETRIC_REPRESENTATION_ITEM ( )  RATIONAL_B_SPLINE_CURVE ( ( 0.9330127018922194093, 0.9330127018922207416, 1.000000000000000000, 0.8660254037844387076, 1.000000000000000000, 0.8660254037844387076, 1.000000000000000000, 0.9330127018922194093, 0.9330127018922194093 ) ) 
 REPRESENTATION_ITEM ( '' )  );
#18750=CARTESIAN_POINT ( 'NONE',  ( -2.229367062500000163, 19.52083333469893134, -3.861377020970580443 ) ) ;
#18753=CARTESIAN_POINT ( 'NONE',  ( 3.152801135295367541, -164.3125000013656063, -3.152801135295367541 ) ) ;
#18754=VERTEX_POINT ( 'NONE', #52663 ) ;
#18758=CARTESIAN_POINT ( 'NONE',  ( 1.975475456537005874E-15, -40.62499999726879452, 5.000000000000000000 ) ) ;
#18769=CARTESIAN_POINT ( 'NONE',  ( -5.000000000000000000, -154.6250000027311842, -6.123233995736766282E-16 ) ) ;
#18775=CARTESIAN_POINT ( 'NONE',  ( -5.000000000000000888, -144.4375000000000284, 2.071067811865474617 ) ) ;
#18777=CARTESIAN_POINT ( 'NONE',  ( 3.152801135295367541, -169.5625000013656063, -3.152801135295367541 ) ) ;
#18778=CARTESIAN_POINT ( 'NONE',  ( 4.458734124999999437, -29.81249999863440436, -5.460374474430324690E-16 ) ) ;
#18782=CARTESIAN_POINT ( 'NONE',  ( -3.152801135295367985, -146.8125000013655779, 3.152801135295367096 ) ) ;
#18783=ORIENTED_EDGE ( 'NONE', *, *, #449, .T. ) ;
#18784=CARTESIAN_POINT ( 'NONE',  ( -4.458734124999999437, -57.56249999863440081, 0.000000000000000000 ) ) ;
#18787=CARTESIAN_POINT ( 'NONE',  ( -5.000000000000000000, 16.91666666666666430, -2.886751345948128211 ) ) ;
#18789=CARTESIAN_POINT ( 'NONE',  ( -6.972266317189433020E-16, -84.12499999726880162, -5.000000000000000000 ) ) ;
#18790=CARTESIAN_POINT ( 'NONE',  ( -2.229367062499996610, -6.145833331967740953, 3.861377020970582219 ) ) ;
#18792=FACE_OUTER_BOUND ( 'NONE', #49989, .T. ) ;
#18793=CARTESIAN_POINT ( 'NONE',  ( -4.458734124999998549, 12.52083333469892779, 2.574251347313722516 ) ) ;
#18795=ORIENTED_EDGE ( 'NONE', *, *, #28315, .F. ) ;
#18798=CARTESIAN_POINT ( 'NONE',  ( 2.229367062500001939, -46.97916666530106511, 3.861377020970579999 ) ) ;
#18799=CARTESIAN_POINT ( 'NONE',  ( -8.190561711645485556E-16, -160.9375000013655779, 4.458734124999999437 ) ) ;
#18801=CARTESIAN_POINT ( 'NONE',  ( 5.000000000000000000, -49.37499999726880873, -6.123233995736766282E-16 ) ) ;
#18803=CARTESIAN_POINT ( 'NONE',  ( 4.458734124999998549, -23.72916666530107221, -2.574251347313721627 ) ) ;
#18805=ORIENTED_EDGE ( 'NONE', *, *, #13105, .T. ) ;
#18807=CARTESIAN_POINT ( 'NONE',  ( 5.000000000000000000, -170.0000000000000000, 0.000000000000000000 ) ) ;
#18808=CARTESIAN_POINT ( 'NONE',  ( -1.846868145590734756, -159.1250000013656063, -4.458734125000000326 ) ) ;
#18812=CARTESIAN_POINT ( 'NONE',  ( -2.500000000000000444, -59.04166666393546592, -4.330127018922193649 ) ) ;
#18813=CARTESIAN_POINT ( 'NONE',  ( 2.229367062500001939, -37.22916666530107221, 3.861377020970579999 ) ) ;
#18814=ORIENTED_EDGE ( 'NONE', *, *, #45086, .T. ) ;
#18820=ORIENTED_EDGE ( 'NONE', *, *, #7570, .T. ) ;
#18822=CARTESIAN_POINT ( 'NONE',  ( -2.229367062499996610, -87.39583333196773651, 3.861377020970582219 ) ) ;
#18835=CARTESIAN_POINT ( 'NONE',  ( -1.127183054612291972E-14, 25.24999999999999645, 4.999999999999999112 ) ) ;
#18837=CARTESIAN_POINT ( 'NONE',  ( -2.229367062500000163, -83.72916666530106511, -3.861377020970580443 ) ) ;
#18841=CARTESIAN_POINT ( 'NONE',  ( 3.061616997868383141E-16, -163.8750000027311842, -5.000000000000000000 ) ) ;
#18843=CARTESIAN_POINT ( 'NONE',  ( -2.071067811865475061, -163.8125000027311842, -5.000000000000000888 ) ) ;
#18853=CARTESIAN_POINT ( 'NONE',  ( 5.000000000000000000, 3.583333333333333925, -2.886751345948130876 ) ) ;
#18854=CARTESIAN_POINT ( 'NONE',  ( -3.152548672688508926E-16, -13.56249999863440259, -5.148502694627439702 ) ) ;
#18855=DIRECTION ( 'NONE',  ( 0.000000000000000000, 0.000000000000000000, 1.000000000000000000 ) ) ;
#18857=CARTESIAN_POINT ( 'NONE',  ( -4.458734124999999437, -42.64583333196773651, -2.574251347313719407 ) ) ;
#18858=CARTESIAN_POINT ( 'NONE',  ( 0.000000000000000000, -170.0000000000000000, 5.000000000000000000 ) ) ;
#18863=EDGE_CURVE ( 'NONE', #30019, #51834, #44914, .T. ) ;
#18865=CARTESIAN_POINT ( 'NONE',  ( -2.229367062499996610, 14.85416666803226171, 3.861377020970582219 ) ) ;
#18867=EDGE_CURVE ( 'NONE', #61933, #5022, #1189, .T. ) ;
#18868=CARTESIAN_POINT ( 'NONE',  ( 0.000000000000000000, -170.0000000000000000, 5.000000000000000000 ) ) ;
#18870=CARTESIAN_POINT ( 'NONE',  ( -4.458734124999999437, -86.64583333196773651, -2.574251347313719407 ) ) ;
#18872=CARTESIAN_POINT ( 'NONE',  ( 2.499999999999998668, 13.79166666939785202, -4.330127018922193649 ) ) ;
#18873=VERTEX_POINT ( 'NONE', #20148 ) ;
#18876=ORIENTED_EDGE ( 'NONE', *, *, #54347, .T. ) ;
#18877=CARTESIAN_POINT ( 'NONE',  ( 5.000000000000000000, -167.0000000000000000, 0.000000000000000000 ) ) ;
#18879=CARTESIAN_POINT ( 'NONE',  ( -2.500000000000000444, -31.16666666666666785, -4.330127018922193649 ) ) ;
#18880=CARTESIAN_POINT ( 'NONE',  ( 2.229367062499998831, -33.64583333196772941, -3.861377020970580887 ) ) ;
#18882=CARTESIAN_POINT ( 'NONE',  ( -5.000000000000000000, -35.87499999726881583, 0.000000000000000000 ) ) ;
#18883=CARTESIAN_POINT ( 'NONE',  ( -2.229367062499996610, -58.14583333196773651, 3.861377020970582219 ) ) ;
#18884=ORIENTED_EDGE ( 'NONE', *, *, #16667, .T. ) ;
#18887=CARTESIAN_POINT ( 'NONE',  ( -4.458734124999999437, -14.64583333196773474, -2.574251347313719407 ) ) ;
#18888=VERTEX_POINT ( 'NONE', #5031 ) ;
#18889=CARTESIAN_POINT ( 'NONE',  ( -5.000000000000000000, -79.08333333333331439, -2.886751345948128211 ) ) ;
#18892=CARTESIAN_POINT ( 'NONE',  ( 2.500000000000002220, -83.54166666393547303, 4.330127018922192761 ) ) ;
#18893=CARTESIAN_POINT ( 'NONE',  ( 5.000000000000000888, -13.58333333333333570, 2.886751345948126879 ) ) ;
#18896=CARTESIAN_POINT ( 'NONE',  ( -2.229367062499996610, -23.39583333196773651, 3.861377020970582219 ) ) ;
#18897=CARTESIAN_POINT ( 'NONE',  ( -4.458734124999999437, -60.56249999863440081, 0.000000000000000000 ) ) ;
#18900=CARTESIAN_POINT ( 'NONE',  ( -1.846868145590737420, -165.0000000013655779, 4.458734124999999437 ) ) ;
#18902=CARTESIAN_POINT ( 'NONE',  ( -2.500000000000000444, 17.83333333333333215, -4.330127018922193649 ) ) ;
#18911=CARTESIAN_POINT ( 'NONE',  ( 4.458734125000000326, -142.6250000013655779, -1.846868145590734978 ) ) ;
#18913=DIRECTION ( 'NONE',  ( -0.000000000000000000, 1.000000000000000000, -0.000000000000000000 ) ) ;
#18915=CARTESIAN_POINT ( 'NONE',  ( -4.458734124999999437, -67.64583333196773651, -2.574251347313719407 ) ) ;
#18918=CARTESIAN_POINT ( 'NONE',  ( 4.458734124999997661, -141.5000000013655779, 1.846868145590737864 ) ) ;
#18920=ORIENTED_EDGE ( 'NONE', *, *, #54966, .F. ) ;
#18921=CARTESIAN_POINT ( 'NONE',  ( 3.061616997868383141E-16, -159.7500000000000000, -5.000000000000000000 ) ) ;
#18926=CARTESIAN_POINT ( 'NONE',  ( -3.152548672688508926E-16, 25.18750000136558853, -5.148502694627439702 ) ) ;
#18927=( BOUNDED_CURVE ( )  B_SPLINE_CURVE ( 2, ( #63457, #48331, #29324, #9407, #18439, #4906, #9719, #19376, #53786 ),
 .UNSPECIFIED., .F., .F. ) 
 B_SPLINE_CURVE_WITH_KNOTS ( ( 3, 2, 2, 2, 3 ),
 ( 0.2729166666666666963, 0.2736111111111111382, 0.2750000000000000222, 0.2763888888888889062, 0.2770833333333333481 ),
 .UNSPECIFIED. ) 
 CURVE ( )  GEOMETRIC_REPRESENTATION_ITEM ( )  RATIONAL_B_SPLINE_CURVE ( ( 0.9330127018922194093, 0.9330127018922220739, 1.000000000000000000, 0.8660254037844387076, 1.000000000000000000, 0.8660254037844387076, 1.000000000000000000, 0.9330127018922194093, 0.9330127018922194093 ) ) 
 REPRESENTATION_ITEM ( '' )  );
#18932=CARTESIAN_POINT ( 'NONE',  ( 5.000000000000000000, -80.50000000000000000, -6.123233995736766282E-16 ) ) ;
#18933=CARTESIAN_POINT ( 'NONE',  ( 4.458734125000000326, 1.104166668032261711, 2.574251347313718519 ) ) ;
#18934=CARTESIAN_POINT ( 'NONE',  ( 4.458734124999998549, -26.97916666530107221, -2.574251347313721627 ) ) ;
#18935=CARTESIAN_POINT ( 'NONE',  ( 1.846868145590736310, -156.6250000013655779, 4.458734124999999437 ) ) ;
#18942=CARTESIAN_POINT ( 'NONE',  ( 2.229367062500001939, -73.22916666530107932, 3.861377020970579999 ) ) ;
#18944=FACE_OUTER_BOUND ( 'NONE', #39615, .T. ) ;
#18946=DIRECTION ( 'NONE',  ( -0.000000000000000000, 1.000000000000000000, -0.000000000000000000 ) ) ;
#18949=CARTESIAN_POINT ( 'NONE',  ( -3.535250795749689387E-16, -14.25000000000000178, -5.773502691896257311 ) ) ;
#18950=CARTESIAN_POINT ( 'NONE',  ( -4.458734124999999437, -19.31249999863440081, 0.000000000000000000 ) ) ;
#18952=CARTESIAN_POINT ( 'NONE',  ( 4.458734124999998549, -75.72916666530106511, -2.574251347313721627 ) ) ;
#18953=EDGE_CURVE ( 'NONE', #11945, #10944, #22763, .T. ) ;
#18954=CARTESIAN_POINT ( 'NONE',  ( 2.730187237215162345E-16, -169.4375000013656063, -4.458734124999999437 ) ) ;
#18955=CARTESIAN_POINT ( 'NONE',  ( 5.000000000000000000, -19.29166666393548013, -2.886751345948129988 ) ) ;
#18956=CARTESIAN_POINT ( 'NONE',  ( -4.458734124999998549, -43.22916666530105800, 2.574251347313722516 ) ) ;
#18957=ORIENTED_EDGE ( 'NONE', *, *, #10548, .T. ) ;
#18959=CARTESIAN_POINT ( 'NONE',  ( 2.229367062500001939, 2.770833334698928674, 3.861377020970579999 ) ) ;
#18962=CARTESIAN_POINT ( 'NONE',  ( -5.000000000000000000, -62.00000000000000000, 0.000000000000000000 ) ) ;
#18964=CARTESIAN_POINT ( 'NONE',  ( -4.458734125000001214, -155.1250000013655779, 1.846868145590734089 ) ) ;
#18966=CARTESIAN_POINT ( 'NONE',  ( -4.999999999999998224, -55.91666666666667140, 2.886751345948131764 ) ) ;
#18967=CARTESIAN_POINT ( 'NONE',  ( 3.535533905932738197, -163.8750000000000284, -3.535533905932738197 ) ) ;
#18970=CARTESIAN_POINT ( 'NONE',  ( 4.458734125000001214, -6.145833331967741842, 2.574251347313718519 ) ) ;
#18971=CARTESIAN_POINT ( 'NONE',  ( -2.229367062500000163, -38.72916666530107221, -3.861377020970580443 ) ) ;
#18972=EDGE_CURVE ( 'NONE', #38824, #28871, #35903, .T. ) ;
#18973=CARTESIAN_POINT ( 'NONE',  ( 3.061616997868383141E-16, -151.8750000027311842, -5.000000000000000000 ) ) ;
#18974=CARTESIAN_POINT ( 'NONE',  ( 2.730187237215162345E-16, -149.1875000013656063, -4.458734124999999437 ) ) ;
#18977=( BOUNDED_CURVE ( )  B_SPLINE_CURVE ( 2, ( #39300, #63454, #19372, #45093, #50236, #21614, #25470, #20664, #35768 ),
 .UNSPECIFIED., .F., .F. ) 
 B_SPLINE_CURVE_WITH_KNOTS ( ( 3, 2, 2, 2, 3 ),
 ( 0.05625000000000000139, 0.05694444444444444337, 0.05833333333333333426, 0.05972222222222222515, 0.06041666666666666713 ),
 .UNSPECIFIED. ) 
 CURVE ( )  GEOMETRIC_REPRESENTATION_ITEM ( )  RATIONAL_B_SPLINE_CURVE ( ( 0.9330127018922192983, 0.9330127018922196314, 1.000000000000000000, 0.8660254037844387076, 1.000000000000000000, 0.8660254037844387076, 1.000000000000000000, 0.9330127018922194093, 0.9330127018922194093 ) ) 
 REPRESENTATION_ITEM ( '' )  );
#18978=VERTEX_POINT ( 'NONE', #60675 ) ;
#18979=CARTESIAN_POINT ( 'NONE',  ( 3.061616997868383141E-16, -154.8750000027311842, -5.000000000000000000 ) ) ;
#18982=CARTESIAN_POINT ( 'NONE',  ( -1.339745962155613812, -12.08034179853029322, -5.000000000000000000 ) ) ;
#18983=CARTESIAN_POINT ( 'NONE',  ( 2.229367062500001939, -74.22916666530106511, 3.861377020970579999 ) ) ;
#18984=ORIENTED_EDGE ( 'NONE', *, *, #30109, .F. ) ;
#18987=CARTESIAN_POINT ( 'NONE',  ( -2.229367062500000163, -0.4791666653010707710, -3.861377020970580443 ) ) ;
#18989=CARTESIAN_POINT ( 'NONE',  ( 3.152801135295366208, -154.5625000013656063, 3.152801135295367985 ) ) ;
#18991=ORIENTED_EDGE ( 'NONE', *, *, #16582, .F. ) ;
#18998=VECTOR ( 'NONE', #43958, 1000.000000000000000 ) ;
#19003=CARTESIAN_POINT ( 'NONE',  ( 1.339745962155615144, -44.70534180126146850, 4.999999999999999112 ) ) ;
#19006=CARTESIAN_POINT ( 'NONE',  ( -4.458734124999999437, 18.68750000136559564, 0.000000000000000000 ) ) ;
#19008=CARTESIAN_POINT ( 'NONE',  ( 4.458734125000000326, -9.145833331967736513, 2.574251347313718519 ) ) ;
#19011=CARTESIAN_POINT ( 'NONE',  ( -4.458734125000001214, -166.8750000013655779, 1.846868145590734089 ) ) ;
#19012=CARTESIAN_POINT ( 'NONE',  ( -6.972266317189433020E-16, -9.250000000000000000, -5.000000000000000000 ) ) ;
#19019=CARTESIAN_POINT ( 'NONE',  ( 2.730187237215162345E-16, -155.4375000013655779, -4.458734124999999437 ) ) ;
#19022=CARTESIAN_POINT ( 'NONE',  ( 5.000000000000000000, -163.0000000000000000, 0.000000000000000000 ) ) ;
#19023=ORIENTED_EDGE ( 'NONE', *, *, #58229, .T. ) ;
#19027=( BOUNDED_CURVE ( )  B_SPLINE_CURVE ( 2, ( #29221, #52747, #48847, #63347, #14750, #53364, #13815, #33434, #24415 ),
 .UNSPECIFIED., .F., .F. ) 
 B_SPLINE_CURVE_WITH_KNOTS ( ( 3, 2, 2, 2, 3 ),
 ( 0.4250000000000003220, 0.4291666666666669738, 0.4333333333333336812, 0.4375000000000003886, 0.4416666666666670404 ),
 .UNSPECIFIED. ) 
 CURVE ( )  GEOMETRIC_REPRESENTATION_ITEM ( )  RATIONAL_B_SPLINE_CURVE ( ( 0.9999999999999938938, 0.9238795325112928447, 1.000000000000000000, 0.9238795325112867385, 1.000000000000000000, 0.9238795325112867385, 1.000000000000000000, 0.9238795325112796331, 1.000000000000007105 ) ) 
 REPRESENTATION_ITEM ( '' )  );
#19028=CARTESIAN_POINT ( 'NONE',  ( -2.499999999999996447, -87.70833333060214443, 4.330127018922195425 ) ) ;
#19029=CARTESIAN_POINT ( 'NONE',  ( 5.000000000000000888, 0.4166666666666659080, 2.886751345948126879 ) ) ;
#19030=CARTESIAN_POINT ( 'NONE',  ( -4.458734124999997661, -59.22916666530106511, 2.574251347313722516 ) ) ;
#19032=CARTESIAN_POINT ( 'NONE',  ( -2.499999999999996447, -4.708333330602147981, 4.330127018922195425 ) ) ;
#19033=CARTESIAN_POINT ( 'NONE',  ( 4.458734124999998549, -27.72916666530107221, -2.574251347313721627 ) ) ;
#19034=CARTESIAN_POINT ( 'NONE',  ( -6.972266317189433020E-16, -42.24999999999998579, -5.000000000000000000 ) ) ;
#19037=CARTESIAN_POINT ( 'NONE',  ( -2.500000000000000444, -43.16666666666665719, -4.330127018922193649 ) ) ;
#19040=CARTESIAN_POINT ( 'NONE',  ( 5.000000000000000000, -4.291666663935479242, -2.886751345948130876 ) ) ;
#19041=CARTESIAN_POINT ( 'NONE',  ( 4.458734124999999437, -67.81249999863440792, -5.460374474430324690E-16 ) ) ;
#19042=CARTESIAN_POINT ( 'NONE',  ( -8.190561711645485556E-16, -143.9375000013656063, 4.458734124999999437 ) ) ;
#19043=CARTESIAN_POINT ( 'NONE',  ( -3.152548672688508926E-16, -78.56249999863440792, -5.148502694627439702 ) ) ;
#19046=CARTESIAN_POINT ( 'NONE',  ( -4.458734124999998549, -23.47916666530107577, 2.574251347313722516 ) ) ;
#19047=CARTESIAN_POINT ( 'NONE',  ( 5.000000000000000000, -66.37499999726881583, -6.123233995736766282E-16 ) ) ;
#19048=EDGE_CURVE ( 'NONE', #59664, #58377, #31372, .T. ) ;
#19051=ORIENTED_EDGE ( 'NONE', *, *, #12950, .F. ) ;
#19053=CARTESIAN_POINT ( 'NONE',  ( 5.000000000000000000, -166.0625000000000000, 2.071067811865478614 ) ) ;
#19055=CARTESIAN_POINT ( 'NONE',  ( -2.229367062499996610, -58.39583333196773651, 3.861377020970582219 ) ) ;
#19057=ORIENTED_EDGE ( 'NONE', *, *, #12302, .T. ) ;
#19058=CYLINDRICAL_SURFACE ( 'NONE', #12166, 5.000000000000000000 ) ;
#19059=CARTESIAN_POINT ( 'NONE',  ( -3.152548672688508926E-16, 14.43750000136559386, -5.148502694627439702 ) ) ;
#19062=CARTESIAN_POINT ( 'NONE',  ( 2.730187237215162345E-16, -163.1875000013655779, -4.458734124999999437 ) ) ;
#19065=CARTESIAN_POINT ( 'NONE',  ( -5.000000000000000000, -51.95833333060214443, -2.886751345948128211 ) ) ;
#19067=CARTESIAN_POINT ( 'NONE',  ( 1.339745962155615144, -19.58034179853029499, 4.999999999999999112 ) ) ;
#19077=CARTESIAN_POINT ( 'NONE',  ( -4.458734124999999437, 6.354166668032259047, -2.574251347313719407 ) ) ;
#19080=CARTESIAN_POINT ( 'NONE',  ( -5.000000000000000000, -147.6250000027312126, -6.123233995736766282E-16 ) ) ;
#19084=AXIS2_PLACEMENT_3D ( 'NONE', #54770, #30634, #25170 ) ;
#19086=CARTESIAN_POINT ( 'NONE',  ( 5.000000000000000000, -145.0000000000000284, 0.000000000000000000 ) ) ;
#19089=CARTESIAN_POINT ( 'NONE',  ( -4.458734124999999437, -28.39583333196773651, -2.574251347313719407 ) ) ;
#19091=DIRECTION ( 'NONE',  ( 0.000000000000000000, 0.000000000000000000, 1.000000000000000000 ) ) ;
#19093=CARTESIAN_POINT ( 'NONE',  ( 1.846868145590736310, -143.6250000013655779, 4.458734124999999437 ) ) ;
#19095=CARTESIAN_POINT ( 'NONE',  ( -4.458734124999998549, 26.52083333469892779, 2.574251347313722516 ) ) ;
#19097=CARTESIAN_POINT ( 'NONE',  ( -4.458734124999999437, -56.64583333196773651, -2.574251347313719407 ) ) ;
#19099=LINE ( 'NONE', #48687, #50415 ) ;
#19100=CARTESIAN_POINT ( 'NONE',  ( 5.000000000000000000, 18.50000000000000000, -6.123233995736766282E-16 ) ) ;
#19103=CARTESIAN_POINT ( 'NONE',  ( -4.458734124999999437, -4.395833331967740065, -2.574251347313719407 ) ) ;
#19104=LINE ( 'NONE', #14597, #58536 ) ;
#19110=CARTESIAN_POINT ( 'NONE',  ( 4.458734124999998549, -54.72916666530107932, -2.574251347313721627 ) ) ;
#19111=CARTESIAN_POINT ( 'NONE',  ( 3.152801135295366208, -161.8125000013656063, 3.152801135295367985 ) ) ;
#19113=CARTESIAN_POINT ( 'NONE',  ( 5.000000000000000888, -49.45833333060213732, 2.886751345948126879 ) ) ;
#19115=CARTESIAN_POINT ( 'NONE',  ( 2.229367062500001939, 4.770833334698926897, 3.861377020970579999 ) ) ;
#19116=ORIENTED_EDGE ( 'NONE', *, *, #1270, .F. ) ;
#19119=CARTESIAN_POINT ( 'NONE',  ( 4.458734124999999437, -160.4375000013655779, 0.000000000000000000 ) ) ;
#19121=UNCERTAINTY_MEASURE_WITH_UNIT (LENGTH_MEASURE( 1.000000000000000082E-05 ), #4901, 'distance_accuracy_value', 'NONE');
#19123=FACE_OUTER_BOUND ( 'NONE', #58926, .T. ) ;
#19126=CARTESIAN_POINT ( 'NONE',  ( -2.229367062500000163, -41.72916666530107932, -3.861377020970580443 ) ) ;
#19128=ORIENTED_EDGE ( 'NONE', *, *, #38843, .T. ) ;
#19132=CARTESIAN_POINT ( 'NONE',  ( 2.499999999999998668, -24.20833333060214443, -4.330127018922193649 ) ) ;
#19134=CARTESIAN_POINT ( 'NONE',  ( 2.229367062500001939, -84.22916666530107932, 3.861377020970579999 ) ) ;
#19136=CARTESIAN_POINT ( 'NONE',  ( 1.339745962155612702, -35.16965819600734022, -5.000000000000000000 ) ) ;
#19138=CARTESIAN_POINT ( 'NONE',  ( 5.000000000000000000, -52.29166666393547303, -2.886751345948130876 ) ) ;
#19140=CARTESIAN_POINT ( 'NONE',  ( -1.339745962155610925, 10.33034180399266333, 5.000000000000000000 ) ) ;
#19142=ADVANCED_FACE ( 'NONE', ( #16910 ), #41344, .F. ) ;
#19146=CARTESIAN_POINT ( 'NONE',  ( -1.049326080737009628E-13, -17.75000000000000355, 5.000000000000000000 ) ) ;
#19148=CARTESIAN_POINT ( 'NONE',  ( -4.458734124999999437, -85.64583333196773651, -2.574251347313719407 ) ) ;
#19152=CARTESIAN_POINT ( 'NONE',  ( -1.339745962155610925, 18.33034180399266333, 5.000000000000000000 ) ) ;
#19154=CARTESIAN_POINT ( 'NONE',  ( -3.535533905932738641, -162.5000000027312126, 3.535533905932737309 ) ) ;
#19159=EDGE_CURVE ( 'NONE', #47541, #39239, #31377, .T. ) ;
#19163=EDGE_CURVE ( 'NONE', #62831, #49893, #37967, .T. ) ;
#19165=DIRECTION ( 'NONE',  ( -0.000000000000000000, 1.000000000000000000, -0.000000000000000000 ) ) ;
#19166=CARTESIAN_POINT ( 'NONE',  ( -4.458734124999997661, -13.22916666530107399, 2.574251347313722516 ) ) ;
#19168=CARTESIAN_POINT ( 'NONE',  ( -2.071067811865475061, -153.6875000000000000, -5.000000000000000888 ) ) ;
#19170=CARTESIAN_POINT ( 'NONE',  ( 2.229367062500001939, -41.22916666530107932, 3.861377020970579999 ) ) ;
#19172=VECTOR ( 'NONE', #17258, 1000.000000000000000 ) ;
#19173=CARTESIAN_POINT ( 'NONE',  ( 1.339745962155615144, -83.58034179853031276, 4.999999999999999112 ) ) ;
#19178=VECTOR ( 'NONE', #14602, 1000.000000000000000 ) ;
#19180=CARTESIAN_POINT ( 'NONE',  ( 4.458734124999998549, 11.27083333469892779, -2.574251347313721627 ) ) ;
#19181=CARTESIAN_POINT ( 'NONE',  ( -9.184850993605147944E-16, -167.2500000000000000, 5.000000000000000000 ) ) ;
#19183=CARTESIAN_POINT ( 'NONE',  ( 4.458734124999998549, -87.97916666530107932, -2.574251347313721627 ) ) ;
#19185=CARTESIAN_POINT ( 'NONE',  ( -5.000000000000000000, 16.12500000273118417, 0.000000000000000000 ) ) ;
#19186=ORIENTED_EDGE ( 'NONE', *, *, #16566, .F. ) ;
#19189=CARTESIAN_POINT ( 'NONE',  ( 2.626220312808019583E-14, 15.74999999999999645, -5.000000000000000000 ) ) ;
#19191=CARTESIAN_POINT ( 'NONE',  ( -5.000000000000000000, -37.00000000000000711, 0.000000000000000000 ) ) ;
#19192=CARTESIAN_POINT ( 'NONE',  ( -2.229367062500000163, -36.47916666530107221, -3.861377020970580443 ) ) ;
#19193=CARTESIAN_POINT ( 'NONE',  ( -3.535250795749689387E-16, -36.12499999726880873, -5.773502691896257311 ) ) ;
#19194=CARTESIAN_POINT ( 'NONE',  ( -4.458734124999999437, -66.39583333196773651, -2.574251347313719407 ) ) ;
#19197=CARTESIAN_POINT ( 'NONE',  ( -4.458734124999999437, -14.39583333196773474, -2.574251347313719407 ) ) ;
#19198=CARTESIAN_POINT ( 'NONE',  ( 4.458734124999999437, -15.06249999863440436, -5.460374474430324690E-16 ) ) ;
#19199=VERTEX_POINT ( 'NONE', #41983 ) ;
#19200=CARTESIAN_POINT ( 'NONE',  ( 2.499999999999998668, -76.33333333333334281, -4.330127018922193649 ) ) ;
#19203=CARTESIAN_POINT ( 'NONE',  ( -4.999999999999999112, -79.79166666393545881, 2.886751345948131764 ) ) ;
#19204=DIRECTION ( 'NONE',  ( -0.000000000000000000, 1.000000000000000000, -0.000000000000000000 ) ) ;
#19207=CARTESIAN_POINT ( 'NONE',  ( 2.229367062500001939, -24.22916666530107577, 3.861377020970579999 ) ) ;
#19208=ORIENTED_EDGE ( 'NONE', *, *, #57738, .F. ) ;
#19210=CARTESIAN_POINT ( 'NONE',  ( -4.458734125000000326, -166.2500000013656347, -1.846868145590735644 ) ) ;
#19212=CARTESIAN_POINT ( 'NONE',  ( -3.535533905932738641, -167.5000000027312126, 3.535533905932737309 ) ) ;
#19217=VECTOR ( 'NONE', #23281, 1000.000000000000000 ) ;
#19219=CARTESIAN_POINT ( 'NONE',  ( -9.184850993605147944E-16, -146.3750000027312126, 5.000000000000000000 ) ) ;
#19221=AXIS2_PLACEMENT_3D ( 'NONE', #43152, #8447, #51874 ) ;
#19223=VECTOR ( 'NONE', #14725, 1000.000000000000000 ) ;
#19226=CARTESIAN_POINT ( 'NONE',  ( -1.846868145590734756, -144.3750000013656063, -4.458734125000000326 ) ) ;
#19230=CARTESIAN_POINT ( 'NONE',  ( -4.458734124999999437, -69.64583333196773651, -2.574251347313719407 ) ) ;
#19232=CARTESIAN_POINT ( 'NONE',  ( -2.500000000000000444, -1.041666663935479686, -4.330127018922193649 ) ) ;
#19233=CARTESIAN_POINT ( 'NONE',  ( -4.458734125000000326, -139.8750000013656063, 1.846868145590734089 ) ) ;
#19236=CARTESIAN_POINT ( 'NONE',  ( 1.975475456537005874E-15, -59.74999999999999289, 5.000000000000000000 ) ) ;
#19239=EDGE_CURVE ( 'NONE', #22662, #8603, #43605, .T. ) ;
#19242=CARTESIAN_POINT ( 'NONE',  ( 2.229367062499998831, 22.10416666803225993, -3.861377020970580887 ) ) ;
#19247=EDGE_CURVE ( 'NONE', #27844, #49754, #25594, .T. ) ;
#19249=CARTESIAN_POINT ( 'NONE',  ( 5.000000000000000888, -60.45833333060213732, 2.886751345948126879 ) ) ;
#19250=CARTESIAN_POINT ( 'NONE',  ( 9.457646018065525792E-16, 0.9375000013655959696, 5.148502694627439702 ) ) ;
#19252=CARTESIAN_POINT ( 'NONE',  ( -4.458734124999999437, -25.56249999863440792, 0.000000000000000000 ) ) ;
#19255=CARTESIAN_POINT ( 'NONE',  ( 2.229367062500001939, 26.02083333469892779, 3.861377020970579999 ) ) ;
#19256=DIRECTION ( 'NONE',  ( -0.000000000000000000, 1.000000000000000000, -0.000000000000000000 ) ) ;
#19258=CARTESIAN_POINT ( 'NONE',  ( -3.152548672688508926E-16, -73.81249999863440792, -5.148502694627439702 ) ) ;
#19260=CARTESIAN_POINT ( 'NONE',  ( -1.339745962155610925, -65.66965819600733312, 5.000000000000000000 ) ) ;
#19261=CARTESIAN_POINT ( 'NONE',  ( -1.339745962155610925, -10.66965819600733312, 5.000000000000000000 ) ) ;
#19263=CARTESIAN_POINT ( 'NONE',  ( -2.071067811865520358, -140.3125000000000284, 4.999999999999957367 ) ) ;
#19264=LINE ( 'NONE', #1587, #11378 ) ;
#19265=CARTESIAN_POINT ( 'NONE',  ( -5.000000000000000000, -12.08333333333333393, -2.886751345948128211 ) ) ;
#19266=CARTESIAN_POINT ( 'NONE',  ( 9.457646018065525792E-16, -15.06249999863440259, 5.148502694627439702 ) ) ;
#19267=EDGE_CURVE ( 'NONE', #16051, #17071, #57432, .T. ) ;
#19268=VECTOR ( 'NONE', #61212, 1000.000000000000000 ) ;
#19269=CARTESIAN_POINT ( 'NONE',  ( -3.152548672688508926E-16, -81.56249999863440792, -5.148502694627439702 ) ) ;
#19270=CARTESIAN_POINT ( 'NONE',  ( -4.458734124999999437, -167.1875000013655779, -5.460374474430324690E-16 ) ) ;
#19271=CARTESIAN_POINT ( 'NONE',  ( -2.500000000000000444, -17.04166666393548368, -4.330127018922193649 ) ) ;
#19272=CARTESIAN_POINT ( 'NONE',  ( 2.229367062499998831, -50.64583333196772941, -3.861377020970580887 ) ) ;
#19276=CARTESIAN_POINT ( 'NONE',  ( -4.458734124999999437, 3.437500001365594748, 0.000000000000000000 ) ) ;
#19279=CARTESIAN_POINT ( 'NONE',  ( 5.000000000000000888, -62.58333333333333570, 2.886751345948126879 ) ) ;
#19280=CARTESIAN_POINT ( 'NONE',  ( -3.152801135295367096, -154.3125000013656063, -3.152801135295367541 ) ) ;
#19283=CARTESIAN_POINT ( 'NONE',  ( -6.972266317189433020E-16, -56.25000000000000000, -5.000000000000000000 ) ) ;
#19284=CARTESIAN_POINT ( 'NONE',  ( -5.000000000000000888, -161.4375000000000000, 2.071067811865474617 ) ) ;
#19285=DIRECTION ( 'NONE',  ( -0.000000000000000000, 1.000000000000000000, -0.000000000000000000 ) ) ;
#19287=CARTESIAN_POINT ( 'NONE',  ( -4.458734124999999437, -6.645833331967741842, -2.574251347313719407 ) ) ;
#19288=CARTESIAN_POINT ( 'NONE',  ( 9.457646018065525792E-16, -46.31249999863440792, 5.148502694627439702 ) ) ;
#19289=CARTESIAN_POINT ( 'NONE',  ( 3.061616997868383141E-16, -150.8750000027312126, -5.000000000000000000 ) ) ;
#19290=CARTESIAN_POINT ( 'NONE',  ( 1.846868145590736310, -149.6250000013655779, 4.458734124999999437 ) ) ;
#19294=CARTESIAN_POINT ( 'NONE',  ( -1.339745962155636017, 3.330341803992664218, 4.999999999999985789 ) ) ;
#19295=CARTESIAN_POINT ( 'NONE',  ( 2.229367062499998831, 29.10416666803225993, -3.861377020970580887 ) ) ;
#19299=( BOUNDED_CURVE ( )  B_SPLINE_CURVE ( 2, ( #4387, #52963, #209, #58423, #33660, #23708, #28516, #59054, #43305 ),
 .UNSPECIFIED., .F., .F. ) 
 B_SPLINE_CURVE_WITH_KNOTS ( ( 3, 2, 2, 2, 3 ),
 ( 0.8437500000000000000, 0.8444444444444444420, 0.8458333333333333259, 0.8472222222222222099, 0.8479166666666666519 ),
 .UNSPECIFIED. ) 
 CURVE ( )  GEOMETRIC_REPRESENTATION_ITEM ( )  RATIONAL_B_SPLINE_CURVE ( ( 0.9330127018922194093, 0.9330127018922194093, 1.000000000000000000, 0.8660254037844387076, 1.000000000000000000, 0.8660254037844387076, 1.000000000000000000, 0.9330127018922194093, 0.9330127018922194093 ) ) 
 REPRESENTATION_ITEM ( '' )  );
#19300=EDGE_CURVE ( 'NONE', #15327, #38362, #4190, .T. ) ;
#19301=EDGE_CURVE ( 'NONE', #5022, #29389, #8802, .T. ) ;
#19302=DIRECTION ( 'NONE',  ( 0.000000000000000000, 0.000000000000000000, 1.000000000000000000 ) ) ;
#19304=EDGE_CURVE ( 'NONE', #32533, #47984, #63362, .T. ) ;
#19306=CARTESIAN_POINT ( 'NONE',  ( 4.458734124999999437, -0.8124999986344055847, -5.460374474430324690E-16 ) ) ;
#19308=CARTESIAN_POINT ( 'NONE',  ( -4.458734124999999437, -154.9375000013655779, -5.460374474430324690E-16 ) ) ;
#19310=VERTEX_POINT ( 'NONE', #44824 ) ;
#19312=CARTESIAN_POINT ( 'NONE',  ( -3.535533905932737309, -148.6250000000000000, -3.535533905932738197 ) ) ;
#19316=ADVANCED_FACE ( 'NONE', ( #14288 ), #4957, .T. ) ;
#19318=CARTESIAN_POINT ( 'NONE',  ( 5.000000000000000000, -64.29166666393547303, -2.886751345948130876 ) ) ;
#19321=EDGE_CURVE ( 'NONE', #1448, #33786, #19104, .T. ) ;
#19322=ORIENTED_EDGE ( 'NONE', *, *, #25943, .T. ) ;
#19323=CARTESIAN_POINT ( 'NONE',  ( -4.458734124999997661, 18.77083333469892779, 2.574251347313722516 ) ) ;
#19326=CARTESIAN_POINT ( 'NONE',  ( -4.458734124999999437, -6.645833331967741842, -2.574251347313719407 ) ) ;
#19329=CARTESIAN_POINT ( 'NONE',  ( 2.071067811865476394, -139.3125000027312126, 5.000000000000000000 ) ) ;
#19331=EDGE_CURVE ( 'NONE', #871, #51921, #12823, .T. ) ;
#19334=VECTOR ( 'NONE', #40293, 1000.000000000000000 ) ;
#19336=FACE_OUTER_BOUND ( 'NONE', #19452, .T. ) ;
#19338=CARTESIAN_POINT ( 'NONE',  ( 3.152801135295366208, -152.8125000013656063, 3.152801135295367985 ) ) ;
#19341=CARTESIAN_POINT ( 'NONE',  ( 2.071067811865550556, -163.1875000000000000, 4.999999999999925393 ) ) ;
#19346=CARTESIAN_POINT ( 'NONE',  ( 2.500000000000002220, 0.3333333333333348136, 4.330127018922192761 ) ) ;
#19347=CARTESIAN_POINT ( 'NONE',  ( -4.458734124999997661, -60.22916666530105800, 2.574251347313722516 ) ) ;
#19349=CARTESIAN_POINT ( 'NONE',  ( -2.500000000000000444, -3.041666663935477910, -4.330127018922193649 ) ) ;
#19350=CARTESIAN_POINT ( 'NONE',  ( -3.152548672688508926E-16, -35.56249999863440792, -5.148502694627439702 ) ) ;
#19351=ORIENTED_EDGE ( 'NONE', *, *, #34157, .T. ) ;
#19352=CARTESIAN_POINT ( 'NONE',  ( 1.975475456537005874E-15, 17.37500000273118417, 5.000000000000000000 ) ) ;
#19353=CARTESIAN_POINT ( 'NONE',  ( 1.975475456537005874E-15, -78.62499999726881583, 5.000000000000000000 ) ) ;
#19356=CARTESIAN_POINT ( 'NONE',  ( 2.500000000000002220, -43.66666666666665719, 4.330127018922192761 ) ) ;
#19358=( BOUNDED_CURVE ( )  B_SPLINE_CURVE ( 2, ( #55031, #45697, #46013, #31530, #57504, #47512, #1976, #21577, #8593 ),
 .UNSPECIFIED., .F., .F. ) 
 B_SPLINE_CURVE_WITH_KNOTS ( ( 3, 2, 2, 2, 3 ),
 ( 0.4812500000000000111, 0.4819444444444444531, 0.4833333333333333370, 0.4847222222222222210, 0.4854166666666666630 ),
 .UNSPECIFIED. ) 
 CURVE ( )  GEOMETRIC_REPRESENTATION_ITEM ( )  RATIONAL_B_SPLINE_CURVE ( ( 0.9330127018922194093, 0.9330127018922194093, 1.000000000000000000, 0.8660254037844387076, 1.000000000000000000, 0.8660254037844387076, 1.000000000000000000, 0.9330127018922194093, 0.9330127018922194093 ) ) 
 REPRESENTATION_ITEM ( '' )  );
#19361=CARTESIAN_POINT ( 'NONE',  ( 2.229367062499998831, -72.64583333196773651, -3.861377020970580887 ) ) ;
#19362=CARTESIAN_POINT ( 'NONE',  ( -3.152801135295367985, -144.0625000013655779, 3.152801135295367096 ) ) ;
#19363=CARTESIAN_POINT ( 'NONE',  ( -4.458734124999998549, -79.22916666530107932, 2.574251347313722516 ) ) ;
#19366=CARTESIAN_POINT ( 'NONE',  ( -4.458734124999998549, -32.47916666530107221, 2.574251347313722516 ) ) ;
#19367=CARTESIAN_POINT ( 'NONE',  ( -5.000000000000000000, -67.95833333060214443, -2.886751345948128211 ) ) ;
#19368=ORIENTED_EDGE ( 'NONE', *, *, #27165, .F. ) ;
#19370=EDGE_LOOP ( 'NONE', ( #43248, #59510, #14687, #19051 ) ) ;
#19372=CARTESIAN_POINT ( 'NONE',  ( -2.499999999999996447, 22.29166666939785202, 4.330127018922195425 ) ) ;
#19374=EDGE_LOOP ( 'NONE', ( #22006, #38675, #19529, #12195 ) ) ;
#19375=CARTESIAN_POINT ( 'NONE',  ( -4.764381983412779477E-15, 27.25000000000000000, 5.000000000000000000 ) ) ;
#19376=CARTESIAN_POINT ( 'NONE',  ( -1.339745962155613812, -3.205341801261480938, -5.000000000000000000 ) ) ;
#19377=CARTESIAN_POINT ( 'NONE',  ( 2.229367062499998831, -60.89583333196774362, -3.861377020970580887 ) ) ;
#19381=CARTESIAN_POINT ( 'NONE',  ( -3.535533905932738641, -146.3750000000000000, 3.535533905932737309 ) ) ;
#19383=CARTESIAN_POINT ( 'NONE',  ( -3.152548672688508926E-16, 15.43750000136559564, -5.148502694627439702 ) ) ;
#19386=CARTESIAN_POINT ( 'NONE',  ( -4.458734124999999437, -166.9375000013655779, -5.460374474430324690E-16 ) ) ;
#19389=CARTESIAN_POINT ( 'NONE',  ( -9.184850993605147944E-16, -153.2500000000000000, 5.000000000000000000 ) ) ;
#19391=CARTESIAN_POINT ( 'NONE',  ( 2.500000000000002220, -40.54166666393548013, 4.330127018922192761 ) ) ;
#19401=CARTESIAN_POINT ( 'NONE',  ( 2.229367062499998831, 5.104166668032261711, -3.861377020970580887 ) ) ;
#19403=( BOUNDED_CURVE ( )  B_SPLINE_CURVE ( 2, ( #20293, #49, #15475, #59540, #34766, #14816, #29609, #49239, #39894 ),
 .UNSPECIFIED., .F., .F. ) 
 B_SPLINE_CURVE_WITH_KNOTS ( ( 3, 2, 2, 2, 3 ),
 ( 0.7687500000000000444, 0.7694444444444444864, 0.7708333333333333703, 0.7722222222222222543, 0.7729166666666666963 ),
 .UNSPECIFIED. ) 
 CURVE ( )  GEOMETRIC_REPRESENTATION_ITEM ( )  RATIONAL_B_SPLINE_CURVE ( ( 0.9330127018922194093, 0.9330127018922194093, 1.000000000000000000, 0.8660254037844387076, 1.000000000000000000, 0.8660254037844387076, 1.000000000000000000, 0.9330127018922194093, 0.9330127018922194093 ) ) 
 REPRESENTATION_ITEM ( '' )  );
#19407=CARTESIAN_POINT ( 'NONE',  ( -5.000000000000000888, -148.6875000027311842, -2.071067811865475949 ) ) ;
#19409=VECTOR ( 'NONE', #63217, 1000.000000000000000 ) ;
#19413=CARTESIAN_POINT ( 'NONE',  ( 5.000000000000000888, -143.9375000000000000, -2.071067811865475505 ) ) ;
#19414=EDGE_CURVE ( 'NONE', #46250, #34014, #14867, .T. ) ;
#19416=CARTESIAN_POINT ( 'NONE',  ( 4.458734124999999437, -167.6250000013656347, -1.846868145590734978 ) ) ;
#19417=CARTESIAN_POINT ( 'NONE',  ( -2.229367062500000163, -31.47916666530107577, -3.861377020970580443 ) ) ;
#19418=CARTESIAN_POINT ( 'NONE',  ( 0.000000000000000000, -170.0000000000000000, 0.000000000000000000 ) ) ;
#19421=CARTESIAN_POINT ( 'NONE',  ( 3.152801135295366208, -143.5625000013655779, 3.152801135295367985 ) ) ;
#19423=CARTESIAN_POINT ( 'NONE',  ( 4.458734125000001214, 25.85416666803225638, 2.574251347313718519 ) ) ;
#19425=CARTESIAN_POINT ( 'NONE',  ( -2.229367062499996610, -54.39583333196773651, 3.861377020970582219 ) ) ;
#19428=CARTESIAN_POINT ( 'NONE',  ( -3.535250795749689387E-16, 18.75000000000000000, -5.773502691896257311 ) ) ;
#19430=CARTESIAN_POINT ( 'NONE',  ( 4.458734125000001214, -6.895833331967734736, 2.574251347313718519 ) ) ;
#19431=CARTESIAN_POINT ( 'NONE',  ( -6.972266317189433020E-16, -23.24999999999999645, -5.000000000000000000 ) ) ;
#19433=DIRECTION ( 'NONE',  ( -0.000000000000000000, 1.000000000000000000, -0.000000000000000000 ) ) ;
#19437=LINE ( 'NONE', #44191, #3959 ) ;
#19438=CARTESIAN_POINT ( 'NONE',  ( -4.458734124999999437, -54.31249999863440081, 0.000000000000000000 ) ) ;
#19439=CARTESIAN_POINT ( 'NONE',  ( 2.730187237215162345E-16, -154.4375000013655779, -4.458734124999999437 ) ) ;
#19440=CARTESIAN_POINT ( 'NONE',  ( 5.000000000000000888, -51.45833333060214443, 2.886751345948126879 ) ) ;
#19441=ORIENTED_EDGE ( 'NONE', *, *, #30734, .F. ) ;
#19442=CARTESIAN_POINT ( 'NONE',  ( -4.458734124999999437, 7.354166668032259935, -2.574251347313719407 ) ) ;
#19446=CARTESIAN_POINT ( 'NONE',  ( 1.846868145590735200, -157.2500000013656063, -4.458734125000000326 ) ) ;
#19449=CYLINDRICAL_SURFACE ( 'NONE', #31256, 5.000000000000000000 ) ;
#19451=CARTESIAN_POINT ( 'NONE',  ( -2.229367062500000163, -42.72916666530107932, -3.861377020970580443 ) ) ;
#19452=EDGE_LOOP ( 'NONE', ( #15596, #45547, #9686, #21300 ) ) ;
#19453=ADVANCED_FACE ( 'NONE', ( #2065 ), #21031, .T. ) ;
#19458=CARTESIAN_POINT ( 'NONE',  ( 9.457646018065525792E-16, 28.93750000136559564, 5.148502694627439702 ) ) ;
#19461=CARTESIAN_POINT ( 'NONE',  ( -6.972266317189433020E-16, -36.25000000000000000, -5.000000000000000000 ) ) ;
#19465=CARTESIAN_POINT ( 'NONE',  ( -6.972266317189433020E-16, 6.750000000000000000, -5.000000000000000000 ) ) ;
#19473=ORIENTED_EDGE ( 'NONE', *, *, #5906, .T. ) ;
#19474=CARTESIAN_POINT ( 'NONE',  ( 1.975475456537005874E-15, -16.62499999726881583, 5.000000000000000000 ) ) ;
#19476=CARTESIAN_POINT ( 'NONE',  ( 5.000000000000000000, -160.1875000027311842, 2.071067811865478614 ) ) ;
#19479=CARTESIAN_POINT ( 'NONE',  ( 2.500000000000002220, -49.54166666393547303, 4.330127018922192761 ) ) ;
#19489=CARTESIAN_POINT ( 'NONE',  ( 2.229367062500001939, -15.97916666530107399, 3.861377020970579999 ) ) ;
#19490=CARTESIAN_POINT ( 'NONE',  ( 5.000000000000000000, -156.0625000000000284, 2.071067811865478614 ) ) ;
#19492=ORIENTED_EDGE ( 'NONE', *, *, #12505, .F. ) ;
#19493=CARTESIAN_POINT ( 'NONE',  ( 4.458734125000000326, -41.14583333196773651, 2.574251347313718519 ) ) ;
#19499=VECTOR ( 'NONE', #45467, 1000.000000000000000 ) ;
#19500=CARTESIAN_POINT ( 'NONE',  ( 2.229367062499998831, 8.354166668032261711, -3.861377020970580887 ) ) ;
#19501=( BOUNDED_CURVE ( )  B_SPLINE_CURVE ( 2, ( #38281, #54011, #43717, #38577, #28618, #53066, #44351, #47917, #29237 ),
 .UNSPECIFIED., .F., .F. ) 
 B_SPLINE_CURVE_WITH_KNOTS ( ( 3, 2, 2, 2, 3 ),
 ( 0.9645833333333333481, 0.9652777777777777901, 0.9666666666666666741, 0.9680555555555555580, 0.9687500000000000000 ),
 .UNSPECIFIED. ) 
 CURVE ( )  GEOMETRIC_REPRESENTATION_ITEM ( )  RATIONAL_B_SPLINE_CURVE ( ( 0.9330127018922194093, 0.9330127018922194093, 1.000000000000000000, 0.8660254037844387076, 1.000000000000000000, 0.8660254037844387076, 1.000000000000000000, 0.9330127018922194093, 0.9330127018922194093 ) ) 
 REPRESENTATION_ITEM ( '' )  );
#19502=DIRECTION ( 'NONE',  ( -0.000000000000000000, 1.000000000000000000, -0.000000000000000000 ) ) ;
#19504=CARTESIAN_POINT ( 'NONE',  ( -4.458734124999997661, -89.47916666530105090, 2.574251347313722516 ) ) ;
#19505=CARTESIAN_POINT ( 'NONE',  ( 4.458734125000001214, 21.85416666803225993, 2.574251347313718519 ) ) ;
#19507=CARTESIAN_POINT ( 'NONE',  ( 5.000000000000000000, 11.62500000273118594, -6.123233995736766282E-16 ) ) ;
#19508=ORIENTED_EDGE ( 'NONE', *, *, #42212, .T. ) ;
#19509=DIRECTION ( 'NONE',  ( 0.000000000000000000, 0.000000000000000000, 1.000000000000000000 ) ) ;
#19511=CARTESIAN_POINT ( 'NONE',  ( -5.000000000000000000, -34.00000000000000000, 0.000000000000000000 ) ) ;
#19512=CARTESIAN_POINT ( 'NONE',  ( -4.458734124999999437, -37.31249999863440792, 0.000000000000000000 ) ) ;
#19513=EDGE_CURVE ( 'NONE', #45731, #13785, #28034, .T. ) ;
#19514=CARTESIAN_POINT ( 'NONE',  ( -2.499999999999996447, -33.70833333060213732, 4.330127018922195425 ) ) ;
#19515=CARTESIAN_POINT ( 'NONE',  ( 4.458734124999999437, -67.81249999863440792, -5.460374474430324690E-16 ) ) ;
#19516=VERTEX_POINT ( 'NONE', #2374 ) ;
#19518=CARTESIAN_POINT ( 'NONE',  ( 4.458734124999998549, -10.72916666530106866, -2.574251347313721627 ) ) ;
#19519=CARTESIAN_POINT ( 'NONE',  ( 4.458734124999998549, -14.97916666530107221, -2.574251347313721627 ) ) ;
#19520=ORIENTED_EDGE ( 'NONE', *, *, #15680, .F. ) ;
#19521=CARTESIAN_POINT ( 'NONE',  ( 5.000000000000000888, -81.58333333333332860, 2.886751345948126879 ) ) ;
#19524=CARTESIAN_POINT ( 'NONE',  ( 5.000000000000000888, -81.45833333060213022, 2.886751345948126879 ) ) ;
#19526=ORIENTED_EDGE ( 'NONE', *, *, #27490, .F. ) ;
#19528=CARTESIAN_POINT ( 'NONE',  ( 2.229367062499998831, -28.89583333196774007, -3.861377020970580887 ) ) ;
#19529=ORIENTED_EDGE ( 'NONE', *, *, #24137, .T. ) ;
#19531=CARTESIAN_POINT ( 'NONE',  ( 4.458734124999999437, -166.6875000013655779, 0.000000000000000000 ) ) ;
#19536=AXIS2_PLACEMENT_3D ( 'NONE', #3520, #41791, #27322 ) ;
#19539=CARTESIAN_POINT ( 'NONE',  ( 4.458734124999997661, -145.7500000013656063, 1.846868145590737864 ) ) ;
#19540=CARTESIAN_POINT ( 'NONE',  ( -2.500000000000000444, 22.83333333333333215, -4.330127018922193649 ) ) ;
#19541=AXIS2_PLACEMENT_3D ( 'NONE', #31928, #12935, #51245 ) ;
#19545=EDGE_LOOP ( 'NONE', ( #55115, #3209, #13159, #19861, #21837, #28676 ) ) ;
#19546=CARTESIAN_POINT ( 'NONE',  ( -1.846868145590737420, -144.0000000013655779, 4.458734124999999437 ) ) ;
#19550=CARTESIAN_POINT ( 'NONE',  ( -3.152548672688508926E-16, -69.81249999863439371, -5.148502694627439702 ) ) ;
#19552=DIRECTION ( 'NONE',  ( -0.000000000000000000, 1.000000000000000000, -0.000000000000000000 ) ) ;
#19555=( BOUNDED_CURVE ( )  B_SPLINE_CURVE ( 2, ( #16420, #36038, #49231, #5173, #50185, #25751, #59533, #24790, #54704 ),
 .UNSPECIFIED., .F., .F. ) 
 B_SPLINE_CURVE_WITH_KNOTS ( ( 3, 2, 2, 2, 3 ),
 ( 0.1687500000000000111, 0.1694444444444444531, 0.1708333333333333370, 0.1722222222222222210, 0.1729166666666666630 ),
 .UNSPECIFIED. ) 
 CURVE ( )  GEOMETRIC_REPRESENTATION_ITEM ( )  RATIONAL_B_SPLINE_CURVE ( ( 0.9330127018922194093, 0.9330127018922194093, 1.000000000000000000, 0.8660254037844387076, 1.000000000000000000, 0.8660254037844387076, 1.000000000000000000, 0.9330127018922194093, 0.9330127018922194093 ) ) 
 REPRESENTATION_ITEM ( '' )  );
#19558=CARTESIAN_POINT ( 'NONE',  ( 0.000000000000000000, -170.0000000000000000, 0.000000000000000000 ) ) ;
#19563=CARTESIAN_POINT ( 'NONE',  ( -4.458734124999997661, 23.52083333469892779, 2.574251347313722516 ) ) ;
#19564=CARTESIAN_POINT ( 'NONE',  ( 6.042630808230842148E-15, 26.75000000000000000, -4.999999999999999112 ) ) ;
#19569=CARTESIAN_POINT ( 'NONE',  ( 5.000000000000000888, -43.45833333060214443, 2.886751345948126879 ) ) ;
#19570=CARTESIAN_POINT ( 'NONE',  ( 4.458734124999998549, 1.270833334698927342, -2.574251347313721627 ) ) ;
#19572=CARTESIAN_POINT ( 'NONE',  ( 2.229367062500001939, -23.22916666530107221, 3.861377020970579999 ) ) ;
#19575=CARTESIAN_POINT ( 'NONE',  ( -2.229367062499996610, 25.85416666803225993, 3.861377020970582219 ) ) ;
#19578=CARTESIAN_POINT ( 'NONE',  ( -4.458734124999997661, -73.47916666530106511, 2.574251347313722516 ) ) ;
#19581=FACE_OUTER_BOUND ( 'NONE', #21774, .T. ) ;
#19583=CARTESIAN_POINT ( 'NONE',  ( -2.071067811865432873, -140.6875000000000284, -5.000000000000041744 ) ) ;
#19586=CARTESIAN_POINT ( 'NONE',  ( -5.000000000000000000, -20.08333333333333215, -2.886751345948128211 ) ) ;
#19587=CARTESIAN_POINT ( 'NONE',  ( 9.457646018065525792E-16, -24.06249999863440436, 5.148502694627439702 ) ) ;
#19588=VECTOR ( 'NONE', #30340, 1000.000000000000000 ) ;
#19590=CARTESIAN_POINT ( 'NONE',  ( 4.458734124999999437, -83.81249999863439371, -5.460374474430324690E-16 ) ) ;
#19591=CARTESIAN_POINT ( 'NONE',  ( -4.458734125000000326, -169.2500000013655779, -1.846868145590735644 ) ) ;
#19592=CARTESIAN_POINT ( 'NONE',  ( 5.000000000000000000, -18.29166666393548013, -2.886751345948129988 ) ) ;
#19593=CARTESIAN_POINT ( 'NONE',  ( 4.458734125000001214, -49.89583333196772941, 2.574251347313718519 ) ) ;
#19597=CARTESIAN_POINT ( 'NONE',  ( -4.458734124999998549, 2.520833334698928674, 2.574251347313722516 ) ) ;
#19598=ORIENTED_EDGE ( 'NONE', *, *, #16874, .F. ) ;
#19600=CARTESIAN_POINT ( 'NONE',  ( -2.499999999999996447, -68.83333333333332860, 4.330127018922195425 ) ) ;
#19601=CARTESIAN_POINT ( 'NONE',  ( 3.152801135295366208, -154.8125000013656063, 3.152801135295367985 ) ) ;
#19603=CARTESIAN_POINT ( 'NONE',  ( 2.499999999999998668, -14.33333333333333037, -4.330127018922193649 ) ) ;
#19604=CARTESIAN_POINT ( 'NONE',  ( -9.184850993605147944E-16, -164.2500000000000000, 5.000000000000000000 ) ) ;
#19605=CARTESIAN_POINT ( 'NONE',  ( -4.999999999999998224, 11.08333333333333393, 2.886751345948131764 ) ) ;
#19607=CARTESIAN_POINT ( 'NONE',  ( -2.229367062500000163, -10.72916666530106866, -3.861377020970580443 ) ) ;
#19608=CARTESIAN_POINT ( 'NONE',  ( -3.152548672688508926E-16, -47.81249999863440792, -5.148502694627439702 ) ) ;
#19609=CARTESIAN_POINT ( 'NONE',  ( -5.000000000000000000, -7.958333330602144429, -2.886751345948128211 ) ) ;
#19610=CARTESIAN_POINT ( 'NONE',  ( -4.458734125000001214, -146.8750000013656063, 1.846868145590734089 ) ) ;
#19614=ORIENTED_EDGE ( 'NONE', *, *, #33496, .F. ) ;
#19619=EDGE_LOOP ( 'NONE', ( #57068, #41829, #42609, #42185 ) ) ;
#19624=CARTESIAN_POINT ( 'NONE',  ( -2.500000000000000444, -51.16666666666666430, -4.330127018922193649 ) ) ;
#19625=CARTESIAN_POINT ( 'NONE',  ( 2.229367062500001939, -1.979166665301068662, 3.861377020970579999 ) ) ;
#19626=FACE_OUTER_BOUND ( 'NONE', #15975, .T. ) ;
#19627=CARTESIAN_POINT ( 'NONE',  ( -3.152801135295367985, -151.8125000013655779, 3.152801135295367096 ) ) ;
#19634=CARTESIAN_POINT ( 'NONE',  ( 5.000000000000000000, 29.58333333333332860, -2.886751345948130876 ) ) ;
#19636=EDGE_CURVE ( 'NONE', #38838, #13440, #35506, .T. ) ;
#19641=EDGE_LOOP ( 'NONE', ( #20274, #60937, #30621, #10673 ) ) ;
#19642=CARTESIAN_POINT ( 'NONE',  ( -2.229367062499996610, 17.85416666803225993, 3.861377020970582219 ) ) ;
#19644=CARTESIAN_POINT ( 'NONE',  ( -2.229367062500000163, -9.729166665301068662, -3.861377020970580443 ) ) ;
#19647=CARTESIAN_POINT ( 'NONE',  ( 2.730187237215162345E-16, -169.1875000013656063, -4.458734124999999437 ) ) ;
#19654=CARTESIAN_POINT ( 'NONE',  ( 1.846868145590736310, -151.8750000013655779, 4.458734124999997661 ) ) ;
#19662=CARTESIAN_POINT ( 'NONE',  ( -2.500000000000000444, -3.166666666666664742, -4.330127018922193649 ) ) ;
#19664=CARTESIAN_POINT ( 'NONE',  ( 4.458734124999999437, -66.81249999863440792, -5.460374474430324690E-16 ) ) ;
#19665=CARTESIAN_POINT ( 'NONE',  ( -4.999999999999998224, 20.08333333333333925, 2.886751345948131764 ) ) ;
#19666=EDGE_CURVE ( 'NONE', #16025, #34977, #32164, .T. ) ;
#19668=CARTESIAN_POINT ( 'NONE',  ( -2.499999999999996447, -0.7083333306021483144, 4.330127018922195425 ) ) ;
#19669=CARTESIAN_POINT ( 'NONE',  ( 4.458734124999999437, -34.81249999863440792, -5.460374474430324690E-16 ) ) ;
#19671=CARTESIAN_POINT ( 'NONE',  ( 1.339745962155612702, 17.83034180399266688, -5.000000000000000000 ) ) ;
#19673=FACE_OUTER_BOUND ( 'NONE', #52638, .T. ) ;
#19674=CARTESIAN_POINT ( 'NONE',  ( 5.000000000000000000, -43.41666666666666430, -2.886751345948129988 ) ) ;
#19675=FACE_OUTER_BOUND ( 'NONE', #51505, .T. ) ;
#19677=CARTESIAN_POINT ( 'NONE',  ( 5.000000000000000000, -64.41666666666665719, -2.886751345948130876 ) ) ;
#19678=CARTESIAN_POINT ( 'NONE',  ( 4.458734124999998549, -71.72916666530107932, -2.574251347313721627 ) ) ;
#19679=CARTESIAN_POINT ( 'NONE',  ( 1.846868145590735200, -144.5000000013656063, -4.458734125000000326 ) ) ;
#19680=CARTESIAN_POINT ( 'NONE',  ( -4.458734124999998549, -80.22916666530106511, 2.574251347313722516 ) ) ;
#19682=EDGE_CURVE ( 'NONE', #15117, #12901, #31943, .T. ) ;
#19683=CARTESIAN_POINT ( 'NONE',  ( 4.458734125000001214, -30.14583333196773296, 2.574251347313718519 ) ) ;
#19685=CARTESIAN_POINT ( 'NONE',  ( -2.500000000000000444, -72.04166666393548724, -4.330127018922193649 ) ) ;
#19688=ADVANCED_FACE ( 'NONE', ( #62497 ), #42222, .T. ) ;
#19689=ORIENTED_EDGE ( 'NONE', *, *, #21290, .T. ) ;
#19693=ORIENTED_EDGE ( 'NONE', *, *, #11189, .F. ) ;
#19696=CARTESIAN_POINT ( 'NONE',  ( -2.229367062500000163, -58.72916666530106511, -3.861377020970580443 ) ) ;
#19701=CARTESIAN_POINT ( 'NONE',  ( -2.229367062500000163, 12.52083333469892601, -3.861377020970580443 ) ) ;
#19704=CARTESIAN_POINT ( 'NONE',  ( 2.730187237215162345E-16, -165.1875000013655779, -4.458734124999999437 ) ) ;
#19705=VERTEX_POINT ( 'NONE', #28063 ) ;
#19707=CARTESIAN_POINT ( 'NONE',  ( 1.339745962155612702, -39.29465819873851729, -5.000000000000000000 ) ) ;
#19710=CARTESIAN_POINT ( 'NONE',  ( 5.000000000000000888, -19.45833333060214798, 2.886751345948126879 ) ) ;
#19715=CARTESIAN_POINT ( 'NONE',  ( -6.972266317189433020E-16, 4.749999999999999112, -5.000000000000000000 ) ) ;
#19719=CARTESIAN_POINT ( 'NONE',  ( 2.229367062499998831, 7.104166668032259935, -3.861377020970580887 ) ) ;
#19722=CARTESIAN_POINT ( 'NONE',  ( 3.535533905932738197, -150.0000000027312126, -3.535533905932738197 ) ) ;
#19723=CARTESIAN_POINT ( 'NONE',  ( 1.975475456537005874E-15, -14.62499999726881228, 5.000000000000000000 ) ) ;
#19727=CARTESIAN_POINT ( 'NONE',  ( -5.000000000000000888, -144.5625000000000000, -2.071067811865475949 ) ) ;
#19729=CARTESIAN_POINT ( 'NONE',  ( -1.846868145590734756, -165.3750000013656347, -4.458734124999999437 ) ) ;
#19730=CARTESIAN_POINT ( 'NONE',  ( -4.458734124999997661, -36.22916666530106511, 2.574251347313722516 ) ) ;
#19732=CARTESIAN_POINT ( 'NONE',  ( 0.000000000000000000, -170.0000000000000000, 0.000000000000000000 ) ) ;
#19734=CARTESIAN_POINT ( 'NONE',  ( -1.846868145590737420, -142.7500000013656063, 4.458734124999999437 ) ) ;
#19735=EDGE_LOOP ( 'NONE', ( #33645, #3689, #2137, #40723 ) ) ;
#19736=CARTESIAN_POINT ( 'NONE',  ( -2.229367062499996610, 28.60416666803226349, 3.861377020970582219 ) ) ;
#19738=CARTESIAN_POINT ( 'NONE',  ( 4.458734124999998549, -60.97916666530106511, -2.574251347313721627 ) ) ;
#19742=CARTESIAN_POINT ( 'NONE',  ( -2.500000000000000444, 16.83333333333333215, -4.330127018922193649 ) ) ;
#19743=CARTESIAN_POINT ( 'NONE',  ( 2.229367062500001939, -52.97916666530107221, 3.861377020970579999 ) ) ;
#19744=CARTESIAN_POINT ( 'NONE',  ( 2.229367062499998831, -6.645833331967741842, -3.861377020970580887 ) ) ;
#19747=CARTESIAN_POINT ( 'NONE',  ( 6.123233995736766282E-16, -170.0000000000000000, -5.000000000000000000 ) ) ;
#19749=CARTESIAN_POINT ( 'NONE',  ( 1.975475456537005874E-15, -53.62499999726880162, 5.000000000000000000 ) ) ;
#19753=CARTESIAN_POINT ( 'NONE',  ( -3.152548672688508926E-16, -52.56249999863440792, -5.148502694627439702 ) ) ;
#19754=CARTESIAN_POINT ( 'NONE',  ( 3.152801135295367541, -156.5625000013656063, -3.152801135295367541 ) ) ;
#19755=EDGE_CURVE ( 'NONE', #1513, #26750, #30469, .T. ) ;
#19756=CARTESIAN_POINT ( 'NONE',  ( -3.535250795749689387E-16, -53.12499999726881583, -5.773502691896257311 ) ) ;
#19757=ORIENTED_EDGE ( 'NONE', *, *, #1109, .F. ) ;
#19758=CARTESIAN_POINT ( 'NONE',  ( 2.499999999999998668, -26.33333333333333215, -4.330127018922193649 ) ) ;
#19759=CARTESIAN_POINT ( 'NONE',  ( -2.229367062499996610, 5.604166668032261711, 3.861377020970582219 ) ) ;
#19760=ORIENTED_EDGE ( 'NONE', *, *, #54778, .F. ) ;
#19761=CARTESIAN_POINT ( 'NONE',  ( -6.972266317189433020E-16, -7.124999997268814056, -5.000000000000000000 ) ) ;
#19762=CARTESIAN_POINT ( 'NONE',  ( 0.000000000000000000, -170.0000000000000000, 0.000000000000000000 ) ) ;
#19763=CARTESIAN_POINT ( 'NONE',  ( 4.458734125000000326, -155.3750000013656347, -1.846868145590734978 ) ) ;
#19766=ADVANCED_FACE ( 'NONE', ( #13272 ), #32896, .T. ) ;
#19769=FACE_OUTER_BOUND ( 'NONE', #13062, .T. ) ;
#19770=CARTESIAN_POINT ( 'NONE',  ( -4.458734124999999437, -45.64583333196774362, -2.574251347313719407 ) ) ;
#19771=ORIENTED_EDGE ( 'NONE', *, *, #51233, .F. ) ;
#19772=ADVANCED_FACE ( 'NONE', ( #49573 ), #29948, .T. ) ;
#19777=CARTESIAN_POINT ( 'NONE',  ( -4.458734124999999437, 29.60416666803225993, -2.574251347313719407 ) ) ;
#19779=DIRECTION ( 'NONE',  ( -0.000000000000000000, 1.000000000000000000, -0.000000000000000000 ) ) ;
#19781=( BOUNDED_CURVE ( )  B_SPLINE_CURVE ( 2, ( #30033, #59312, #5927, #6560, #16207, #10421, #59645, #55456, #30995 ),
 .UNSPECIFIED., .F., .F. ) 
 B_SPLINE_CURVE_WITH_KNOTS ( ( 3, 2, 2, 2, 3 ),
 ( 0.7395833333333333703, 0.7402777777777778123, 0.7416666666666666963, 0.7430555555555555802, 0.7437500000000000222 ),
 .UNSPECIFIED. ) 
 CURVE ( )  GEOMETRIC_REPRESENTATION_ITEM ( )  RATIONAL_B_SPLINE_CURVE ( ( 0.9330127018922194093, 0.9330127018922194093, 1.000000000000000000, 0.8660254037844387076, 1.000000000000000000, 0.8660254037844387076, 1.000000000000000000, 0.9330127018922194093, 0.9330127018922194093 ) ) 
 REPRESENTATION_ITEM ( '' )  );
#19785=DIRECTION ( 'NONE',  ( -0.000000000000000000, 1.000000000000000000, -0.000000000000000000 ) ) ;
#19789=DIRECTION ( 'NONE',  ( 0.000000000000000000, 0.000000000000000000, 1.000000000000000000 ) ) ;
#19795=CARTESIAN_POINT ( 'NONE',  ( 3.535533905932736864, -161.2500000027312126, 3.535533905932738641 ) ) ;
#19797=CARTESIAN_POINT ( 'NONE',  ( 1.339745962155615144, -49.58034179853029144, 4.999999999999999112 ) ) ;
#19805=CARTESIAN_POINT ( 'NONE',  ( 2.499999999999998668, -48.20833333060215153, -4.330127018922193649 ) ) ;
#19806=CARTESIAN_POINT ( 'NONE',  ( -2.229367062500000163, -16.47916666530107577, -3.861377020970580443 ) ) ;
#19807=DIRECTION ( 'NONE',  ( 0.000000000000000000, 0.000000000000000000, 1.000000000000000000 ) ) ;
#19808=CARTESIAN_POINT ( 'NONE',  ( 2.071067811865476394, -153.1875000000000284, 5.000000000000000000 ) ) ;
#19811=CARTESIAN_POINT ( 'NONE',  ( -2.229367062500000163, -47.72916666530106511, -3.861377020970580443 ) ) ;
#19812=CARTESIAN_POINT ( 'NONE',  ( 0.000000000000000000, -170.0000000000000000, 5.000000000000000000 ) ) ;
#19814=DIRECTION ( 'NONE',  ( -0.000000000000000000, 1.000000000000000000, -0.000000000000000000 ) ) ;
#19817=CARTESIAN_POINT ( 'NONE',  ( 4.458734125000001214, 11.10416666803225993, 2.574251347313718519 ) ) ;
#19819=CARTESIAN_POINT ( 'NONE',  ( 5.000000000000000000, -37.37499999726881583, -6.123233995736766282E-16 ) ) ;
#19821=CARTESIAN_POINT ( 'NONE',  ( -3.152548672688508926E-16, 22.18750000136559564, -5.148502694627439702 ) ) ;
#19823=CARTESIAN_POINT ( 'NONE',  ( -3.535250795749689387E-16, 7.875000002731186832, -5.773502691896257311 ) ) ;
#19828=CARTESIAN_POINT ( 'NONE',  ( -5.000000000000000000, -32.00000000000000000, 0.000000000000000000 ) ) ;
#19829=CARTESIAN_POINT ( 'NONE',  ( 9.457646018065525792E-16, -40.06249999863439371, 5.148502694627439702 ) ) ;
#19830=CARTESIAN_POINT ( 'NONE',  ( 5.000000000000000000, -33.29166666393547303, -2.886751345948129988 ) ) ;
#19831=CARTESIAN_POINT ( 'NONE',  ( -4.458734124999999437, -64.39583333196772230, -2.574251347313719407 ) ) ;
#19834=CARTESIAN_POINT ( 'NONE',  ( -4.458734124999998549, -15.22916666530107754, 2.574251347313722516 ) ) ;
#19835=CARTESIAN_POINT ( 'NONE',  ( -4.458734124999998549, -14.47916666530107221, 2.574251347313722516 ) ) ;
#19836=ORIENTED_EDGE ( 'NONE', *, *, #24849, .F. ) ;
#19837=CARTESIAN_POINT ( 'NONE',  ( -4.999999999999999112, -79.91666666666667140, 2.886751345948131764 ) ) ;
#19838=CARTESIAN_POINT ( 'NONE',  ( -4.458734125000001214, -166.8750000013655779, 1.846868145590734089 ) ) ;
#19840=CARTESIAN_POINT ( 'NONE',  ( -4.999999999999999112, -81.79166666393547303, 2.886751345948131764 ) ) ;
#19841=DIRECTION ( 'NONE',  ( 0.000000000000000000, 0.000000000000000000, 1.000000000000000000 ) ) ;
#19844=CARTESIAN_POINT ( 'NONE',  ( -3.152548672688508926E-16, -29.81249999863440436, -5.148502694627439702 ) ) ;
#19848=CARTESIAN_POINT ( 'NONE',  ( 3.152801135295367541, -167.5625000013656063, -3.152801135295367541 ) ) ;
#19850=CARTESIAN_POINT ( 'NONE',  ( -9.184850993605147944E-16, -148.2500000000000284, 5.000000000000000000 ) ) ;
#19851=ORIENTED_EDGE ( 'NONE', *, *, #5250, .T. ) ;
#19855=CARTESIAN_POINT ( 'NONE',  ( 2.730187237215162345E-16, -144.4375000013656063, -4.458734124999999437 ) ) ;
#19856=LINE ( 'NONE', #54274, #32195 ) ;
#19861=ORIENTED_EDGE ( 'NONE', *, *, #48785, .F. ) ;
#19862=CARTESIAN_POINT ( 'NONE',  ( 1.846868145590736310, -140.8750000013656063, 4.458734124999999437 ) ) ;
#19865=CYLINDRICAL_SURFACE ( 'NONE', #37564, 5.000000000000000000 ) ;
#19867=CARTESIAN_POINT ( 'NONE',  ( 9.457646018065525792E-16, -75.31249999863440792, 5.148502694627439702 ) ) ;
#19869=CARTESIAN_POINT ( 'NONE',  ( -2.499999999999996447, -69.83333333333332860, 4.330127018922195425 ) ) ;
#19872=VERTEX_POINT ( 'NONE', #48304 ) ;
#19879=CARTESIAN_POINT ( 'NONE',  ( 4.458734125000000326, 19.85416666803226349, 2.574251347313718519 ) ) ;
#19880=CARTESIAN_POINT ( 'NONE',  ( 2.499999999999998668, -18.33333333333333215, -4.330127018922193649 ) ) ;
#19881=CIRCLE ( 'NONE', #26049, 5.000000000000000000 ) ;
#19886=DIRECTION ( 'NONE',  ( -0.000000000000000000, 1.000000000000000000, -0.000000000000000000 ) ) ;
#19887=CARTESIAN_POINT ( 'NONE',  ( 2.229367062500001939, 0.02083333469892964529, 3.861377020970579999 ) ) ;
#19888=CARTESIAN_POINT ( 'NONE',  ( 2.229367062500001939, -26.22916666530106866, 3.861377020970579999 ) ) ;
#19891=CARTESIAN_POINT ( 'NONE',  ( 4.458734124999998549, 25.27083333469892779, -2.574251347313721627 ) ) ;
#19894=CARTESIAN_POINT ( 'NONE',  ( -4.458734124999999437, -74.64583333196773651, -2.574251347313719407 ) ) ;
#19897=CARTESIAN_POINT ( 'NONE',  ( 5.000000000000000000, 27.70833333606451987, -2.886751345948129988 ) ) ;
#19900=CARTESIAN_POINT ( 'NONE',  ( -5.000000000000000000, -56.95833333060214443, -2.886751345948128211 ) ) ;
#19901=CARTESIAN_POINT ( 'NONE',  ( -5.000000000000000000, -17.08333333333333215, -2.886751345948128211 ) ) ;
#19902=CARTESIAN_POINT ( 'NONE',  ( 4.458734124999999437, -23.81249999863440436, -5.460374474430324690E-16 ) ) ;
#19903=CARTESIAN_POINT ( 'NONE',  ( -2.229367062499996610, -81.14583333196773651, 3.861377020970582219 ) ) ;
#19904=CARTESIAN_POINT ( 'NONE',  ( -1.846868145590734756, -166.3750000013655779, -4.458734125000000326 ) ) ;
#19905=CARTESIAN_POINT ( 'NONE',  ( 2.499999999999998668, -20.20833333060214798, -4.330127018922193649 ) ) ;
#19906=CARTESIAN_POINT ( 'NONE',  ( 4.458734125000001214, -48.89583333196772941, 2.574251347313718519 ) ) ;
#19907=ORIENTED_EDGE ( 'NONE', *, *, #55157, .T. ) ;
#19909=CARTESIAN_POINT ( 'NONE',  ( 0.000000000000000000, -170.0000000000000000, 5.000000000000000000 ) ) ;
#19910=CARTESIAN_POINT ( 'NONE',  ( 4.458734125000001214, 0.8541666680322613781, 2.574251347313718519 ) ) ;
#19913=CARTESIAN_POINT ( 'NONE',  ( 1.060575238724906964E-15, -65.75000000000000000, 5.773502691896257311 ) ) ;
#19914=CARTESIAN_POINT ( 'NONE',  ( 1.846868145590735200, -151.5000000013655779, -4.458734125000000326 ) ) ;
#19917=CARTESIAN_POINT ( 'NONE',  ( -3.535533905932737309, -163.6250000000000284, -3.535533905932738197 ) ) ;
#19918=CARTESIAN_POINT ( 'NONE',  ( 0.000000000000000000, -170.0000000000000000, 0.000000000000000000 ) ) ;
#19920=CARTESIAN_POINT ( 'NONE',  ( -4.458734124999999437, -11.56249999863440792, 0.000000000000000000 ) ) ;
#19921=CARTESIAN_POINT ( 'NONE',  ( -2.229367062499996610, -46.39583333196774362, 3.861377020970582219 ) ) ;
#19924=CARTESIAN_POINT ( 'NONE',  ( 3.152801135295367541, -149.3125000013655779, -3.152801135295367541 ) ) ;
#19929=CARTESIAN_POINT ( 'NONE',  ( 0.000000000000000000, -170.0000000000000000, 0.000000000000000000 ) ) ;
#19932=( BOUNDED_CURVE ( )  B_SPLINE_CURVE ( 2, ( #2798, #62605, #36886, #42648, #38148, #51685, #33314, #62289, #22417 ),
 .UNSPECIFIED., .F., .F. ) 
 B_SPLINE_CURVE_WITH_KNOTS ( ( 3, 2, 2, 2, 3 ),
 ( 0.3270833333333333370, 0.3277777777777777790, 0.3291666666666666630, 0.3305555555555555469, 0.3312499999999999889 ),
 .UNSPECIFIED. ) 
 CURVE ( )  GEOMETRIC_REPRESENTATION_ITEM ( )  RATIONAL_B_SPLINE_CURVE ( ( 0.9330127018922194093, 0.9330127018922194093, 1.000000000000000000, 0.8660254037844387076, 1.000000000000000000, 0.8660254037844387076, 1.000000000000000000, 0.9330127018922194093, 0.9330127018922194093 ) ) 
 REPRESENTATION_ITEM ( '' )  );
#19938=CARTESIAN_POINT ( 'NONE',  ( -2.499999999999996447, 9.166666666666666075, 4.330127018922195425 ) ) ;
#19939=CARTESIAN_POINT ( 'NONE',  ( -2.229367062500000163, -1.479166665301071770, -3.861377020970580443 ) ) ;
#19941=CARTESIAN_POINT ( 'NONE',  ( 3.152801135295366208, -150.5625000013655779, 3.152801135295367985 ) ) ;
#19950=CARTESIAN_POINT ( 'NONE',  ( -1.339745962155612480, 27.91965820146970856, -5.000000000000000888 ) ) ;
#19954=FACE_OUTER_BOUND ( 'NONE', #23284, .T. ) ;
#19957=CARTESIAN_POINT ( 'NONE',  ( 0.000000000000000000, -170.0000000000000000, 0.000000000000000000 ) ) ;
#19958=CARTESIAN_POINT ( 'NONE',  ( -4.458734124999999437, 17.60416666803225993, -2.574251347313719407 ) ) ;
#19960=VERTEX_POINT ( 'NONE', #67 ) ;
#19961=CARTESIAN_POINT ( 'NONE',  ( 4.458734124999998549, -9.979166665301068662, -2.574251347313721627 ) ) ;
#19965=CARTESIAN_POINT ( 'NONE',  ( -9.184850993605147944E-16, -139.3750000027312126, 5.000000000000000000 ) ) ;
#19970=VECTOR ( 'NONE', #54008, 1000.000000000000000 ) ;
#19973=CARTESIAN_POINT ( 'NONE',  ( 5.000000000000000000, -142.1250000027312126, 0.000000000000000000 ) ) ;
#19976=CARTESIAN_POINT ( 'NONE',  ( 3.152801135295367541, -153.5625000013656063, -3.152801135295367541 ) ) ;
#19979=ORIENTED_EDGE ( 'NONE', *, *, #39441, .F. ) ;
#19983=CARTESIAN_POINT ( 'NONE',  ( -2.499999999999996447, -2.833333333333333481, 4.330127018922195425 ) ) ;
#19985=CARTESIAN_POINT ( 'NONE',  ( -2.229367062499996610, -68.14583333196773651, 3.861377020970582219 ) ) ;
#19986=CARTESIAN_POINT ( 'NONE',  ( -1.339745962155610925, -30.66965819600732956, 5.000000000000000000 ) ) ;
#19987=CARTESIAN_POINT ( 'NONE',  ( 5.000000000000000000, -1.374999997268814500, -6.123233995736766282E-16 ) ) ;
#19988=CARTESIAN_POINT ( 'NONE',  ( 2.229367062500001939, -32.97916666530106511, 3.861377020970579999 ) ) ;
#19990=CARTESIAN_POINT ( 'NONE',  ( -6.972266317189433020E-16, 17.87500000273118417, -5.000000000000000000 ) ) ;
#19993=CARTESIAN_POINT ( 'NONE',  ( 1.339745962155615144, 5.294658198738519950, 4.999999999999999112 ) ) ;
#19994=CARTESIAN_POINT ( 'NONE',  ( -3.535250795749689387E-16, -50.25000000000000711, -5.773502691896257311 ) ) ;
#19995=CARTESIAN_POINT ( 'NONE',  ( 1.339745962155612702, -17.16965819600733312, -5.000000000000000000 ) ) ;
#19997=CARTESIAN_POINT ( 'NONE',  ( -2.500000000000000444, -4.166666666666666075, -4.330127018922193649 ) ) ;
#19998=CARTESIAN_POINT ( 'NONE',  ( 4.458734124999999437, -72.81249999863439371, -5.460374474430324690E-16 ) ) ;
#19999=CARTESIAN_POINT ( 'NONE',  ( -4.458734125000001214, -143.1250000013656063, 1.846868145590734089 ) ) ;
#20000=CARTESIAN_POINT ( 'NONE',  ( 2.229367062499998831, -83.64583333196773651, -3.861377020970580887 ) ) ;
#20002=CARTESIAN_POINT ( 'NONE',  ( -2.229367062500000163, -31.72916666530107577, -3.861377020970580443 ) ) ;
#20003=CARTESIAN_POINT ( 'NONE',  ( -5.000000000000000000, -71.87499999726880162, 0.000000000000000000 ) ) ;
#20006=CARTESIAN_POINT ( 'NONE',  ( 0.000000000000000000, -170.0000000000000000, 5.000000000000000000 ) ) ;
#20007=ORIENTED_EDGE ( 'NONE', *, *, #22457, .T. ) ;
#20009=CARTESIAN_POINT ( 'NONE',  ( 1.339745962155613146, 28.29465819873852084, 5.000000000000000888 ) ) ;
#20012=CARTESIAN_POINT ( 'NONE',  ( -2.500000000000000444, -39.16666666666667140, -4.330127018922193649 ) ) ;
#20014=CARTESIAN_POINT ( 'NONE',  ( 4.458734124999999437, -58.06249999863440081, -5.460374474430324690E-16 ) ) ;
#20016=EDGE_LOOP ( 'NONE', ( #7290, #28433, #6643, #46526 ) ) ;
#20018=CARTESIAN_POINT ( 'NONE',  ( -5.000000000000000888, -146.4375000000000000, 2.071067811865474617 ) ) ;
#20019=CARTESIAN_POINT ( 'NONE',  ( -6.972266317189433020E-16, -2.124999997268814056, -5.000000000000000000 ) ) ;
#20020=CARTESIAN_POINT ( 'NONE',  ( -2.229367062499996610, 12.85416666803226171, 3.861377020970582219 ) ) ;
#20022=CARTESIAN_POINT ( 'NONE',  ( -6.972266317189433020E-16, -24.24999999999999645, -5.000000000000000000 ) ) ;
#20023=CARTESIAN_POINT ( 'NONE',  ( -8.190561711645485556E-16, -161.6875000013655779, 4.458734124999999437 ) ) ;
#20026=CARTESIAN_POINT ( 'NONE',  ( 5.000000000000000000, -39.41666666666667851, -2.886751345948130876 ) ) ;
#20028=EDGE_CURVE ( 'NONE', #48755, #30395, #10371, .T. ) ;
#20030=CARTESIAN_POINT ( 'NONE',  ( 1.339745962155615144, -40.58034179853029144, 4.999999999999999112 ) ) ;
#20034=CARTESIAN_POINT ( 'NONE',  ( -6.972266317189433020E-16, 12.87500000273118417, -5.000000000000000000 ) ) ;
#20035=CARTESIAN_POINT ( 'NONE',  ( 2.500000000000002220, -78.54166666393547303, 4.330127018922192761 ) ) ;
#20040=CARTESIAN_POINT ( 'NONE',  ( -2.229367062500000163, 5.270833334698927786, -3.861377020970580443 ) ) ;
#20041=CARTESIAN_POINT ( 'NONE',  ( -5.000000000000000000, -9.958333330602144429, -2.886751345948128211 ) ) ;
#20043=CARTESIAN_POINT ( 'NONE',  ( 3.535533905932736864, -151.2500000027312126, 3.535533905932738641 ) ) ;
#20047=( BOUNDED_CURVE ( )  B_SPLINE_CURVE ( 2, ( #62463, #24784, #671, #29270, #48900, #4844, #58247, #29917, #9349 ),
 .UNSPECIFIED., .F., .F. ) 
 B_SPLINE_CURVE_WITH_KNOTS ( ( 3, 2, 2, 2, 3 ),
 ( 0.1687500000000000111, 0.1694444444444444531, 0.1708333333333333370, 0.1722222222222222210, 0.1729166666666666630 ),
 .UNSPECIFIED. ) 
 CURVE ( )  GEOMETRIC_REPRESENTATION_ITEM ( )  RATIONAL_B_SPLINE_CURVE ( ( 0.9330127018922194093, 0.9330127018922194093, 1.000000000000000000, 0.8660254037844387076, 1.000000000000000000, 0.8660254037844387076, 1.000000000000000000, 0.9330127018922194093, 0.9330127018922194093 ) ) 
 REPRESENTATION_ITEM ( '' )  );
#20049=FACE_OUTER_BOUND ( 'NONE', #48229, .T. ) ;
#20051=EDGE_CURVE ( 'NONE', #7918, #62831, #5872, .T. ) ;
#20053=CARTESIAN_POINT ( 'NONE',  ( -4.458734124999999437, -166.1875000013655779, -5.460374474430324690E-16 ) ) ;
#20057=CARTESIAN_POINT ( 'NONE',  ( 3.152801135295367541, -145.3125000013655779, -3.152801135295367541 ) ) ;
#20059=CARTESIAN_POINT ( 'NONE',  ( -2.499999999999996447, -90.70833333060214443, 4.330127018922195425 ) ) ;
#20061=CARTESIAN_POINT ( 'NONE',  ( 4.458734124999999437, -61.06249999863440081, -5.460374474430324690E-16 ) ) ;
#20063=CARTESIAN_POINT ( 'NONE',  ( -2.499999999999996447, 15.16666666666666607, 4.330127018922195425 ) ) ;
#20064=CARTESIAN_POINT ( 'NONE',  ( -2.229367062499996610, -50.14583333196772941, 3.861377020970582219 ) ) ;
#20065=VECTOR ( 'NONE', #45338, 1000.000000000000000 ) ;
#20066=CARTESIAN_POINT ( 'NONE',  ( -4.458734124999999437, -4.312499998634401699, 0.000000000000000000 ) ) ;
#20068=CARTESIAN_POINT ( 'NONE',  ( -1.339745962155613812, -23.20534180126147916, -5.000000000000000000 ) ) ;
#20069=CARTESIAN_POINT ( 'NONE',  ( 3.061616997868383141E-16, -164.8750000027311842, -5.000000000000000000 ) ) ;
#20070=FACE_OUTER_BOUND ( 'NONE', #12780, .T. ) ;
#20073=CARTESIAN_POINT ( 'NONE',  ( -5.000000000000000000, -31.87499999726880873, 0.000000000000000000 ) ) ;
#20074=CARTESIAN_POINT ( 'NONE',  ( 4.458734124999998549, -52.72916666530107221, -2.574251347313721627 ) ) ;
#20075=CARTESIAN_POINT ( 'NONE',  ( 4.458734125000000326, -156.6250000013655779, -1.846868145590734978 ) ) ;
#20076=EDGE_CURVE ( 'NONE', #25951, #34696, #39278, .T. ) ;
#20077=CARTESIAN_POINT ( 'NONE',  ( -5.000000000000000000, -57.87499999726880873, 0.000000000000000000 ) ) ;
#20078=VERTEX_POINT ( 'NONE', #49261 ) ;
#20079=CARTESIAN_POINT ( 'NONE',  ( 5.000000000000000888, -26.58333333333333215, 2.886751345948126879 ) ) ;
#20080=CARTESIAN_POINT ( 'NONE',  ( 4.458734125000001214, 5.854166668032262599, 2.574251347313718519 ) ) ;
#20081=VERTEX_POINT ( 'NONE', #24817 ) ;
#20084=CARTESIAN_POINT ( 'NONE',  ( -4.458734125000000326, -156.0000000013656063, -1.846868145590735644 ) ) ;
#20086=CARTESIAN_POINT ( 'NONE',  ( 1.339745962155615144, -87.58034179853028434, 4.999999999999999112 ) ) ;
#20089=CARTESIAN_POINT ( 'NONE',  ( 4.458734124999998549, -42.97916666530107221, -2.574251347313721627 ) ) ;
#20090=ORIENTED_EDGE ( 'NONE', *, *, #56503, .F. ) ;
#20091=CARTESIAN_POINT ( 'NONE',  ( 5.000000000000000888, -143.0625000027312126, -2.071067811865475505 ) ) ;
#20093=CARTESIAN_POINT ( 'NONE',  ( 2.499999999999998668, 3.791666669397852019, -4.330127018922193649 ) ) ;
#20094=ORIENTED_EDGE ( 'NONE', *, *, #19636, .T. ) ;
#20095=CARTESIAN_POINT ( 'NONE',  ( -3.152548672688508926E-16, -89.81249999863439371, -5.148502694627439702 ) ) ;
#20097=CARTESIAN_POINT ( 'NONE',  ( -5.000000000000000888, -165.5625000000000568, -2.071067811865475949 ) ) ;
#20099=CARTESIAN_POINT ( 'NONE',  ( -2.500000000000000444, 23.83333333333333215, -4.330127018922193649 ) ) ;
#20106=EDGE_CURVE ( 'NONE', #27694, #30611, #54833, .T. ) ;
#20109=CARTESIAN_POINT ( 'NONE',  ( -1.339745962155613812, 4.794658198738519950, -5.000000000000000000 ) ) ;
#20111=CARTESIAN_POINT ( 'NONE',  ( 4.458734124999998549, -89.97916666530105090, -2.574251347313721627 ) ) ;
#20112=ADVANCED_FACE ( 'NONE', ( #11920 ), #30590, .T. ) ;
#20113=CARTESIAN_POINT ( 'NONE',  ( 1.975475456537005874E-15, 11.37500000273118239, 5.000000000000000000 ) ) ;
#20115=( BOUNDED_CURVE ( )  B_SPLINE_CURVE ( 2, ( #22978, #38079, #8184, #2728, #37448, #22347, #51618, #17825, #23290 ),
 .UNSPECIFIED., .F., .F. ) 
 B_SPLINE_CURVE_WITH_KNOTS ( ( 3, 2, 2, 2, 3 ),
 ( 0.8187499999999999778, 0.8194444444444444198, 0.8208333333333333037, 0.8222222222222221877, 0.8229166666666666297 ),
 .UNSPECIFIED. ) 
 CURVE ( )  GEOMETRIC_REPRESENTATION_ITEM ( )  RATIONAL_B_SPLINE_CURVE ( ( 0.9330127018922194093, 0.9330127018922194093, 1.000000000000000000, 0.8660254037844387076, 1.000000000000000000, 0.8660254037844387076, 1.000000000000000000, 0.9330127018922194093, 0.9330127018922194093 ) ) 
 REPRESENTATION_ITEM ( '' )  );
#20116=ADVANCED_FACE ( 'NONE', ( #41188 ), #36376, .T. ) ;
#20117=ORIENTED_EDGE ( 'NONE', *, *, #13898, .T. ) ;
#20118=CARTESIAN_POINT ( 'NONE',  ( 5.000000000000000000, -31.41666666666667140, -2.886751345948130876 ) ) ;
#20120=CARTESIAN_POINT ( 'NONE',  ( -5.000000000000000888, -162.6875000027311557, -2.071067811865475949 ) ) ;
#20124=EDGE_CURVE ( 'NONE', #48949, #14934, #51905, .T. ) ;
#20132=CARTESIAN_POINT ( 'NONE',  ( -5.000000000000000888, -141.6875000027311842, -2.071067811865475949 ) ) ;
#20133=CARTESIAN_POINT ( 'NONE',  ( 4.458734125000000326, -18.89583333196774362, 2.574251347313718519 ) ) ;
#20134=CARTESIAN_POINT ( 'NONE',  ( -5.000000000000000888, -154.4375000000000284, 2.071067811865474617 ) ) ;
#20137=CARTESIAN_POINT ( 'NONE',  ( -8.190561711645485556E-16, -157.6875000013655779, 4.458734124999999437 ) ) ;
#20139=CARTESIAN_POINT ( 'NONE',  ( 4.458734125000000326, -44.14583333196774362, 2.574251347313718519 ) ) ;
#20142=CARTESIAN_POINT ( 'NONE',  ( -4.999999999999998224, -11.91666666666666607, 2.886751345948131764 ) ) ;
#20143=EDGE_CURVE ( 'NONE', #5292, #7216, #21268, .T. ) ;
#20144=CARTESIAN_POINT ( 'NONE',  ( 2.500000000000002220, 27.33333333333333215, 4.330127018922192761 ) ) ;
#20147=CARTESIAN_POINT ( 'NONE',  ( 4.458734125000001214, 9.104166668032261711, 2.574251347313718519 ) ) ;
#20148=CARTESIAN_POINT ( 'NONE',  ( 1.975475456537005874E-15, -81.74999999999998579, 5.000000000000000000 ) ) ;
#20150=CARTESIAN_POINT ( 'NONE',  ( -3.152548672688508926E-16, 23.18750000136559208, -5.148502694627439702 ) ) ;
#20152=CARTESIAN_POINT ( 'NONE',  ( 5.000000000000000000, 6.625000002731185944, -6.123233995736766282E-16 ) ) ;
#20154=CARTESIAN_POINT ( 'NONE',  ( 0.000000000000000000, -170.0000000000000000, 5.000000000000000000 ) ) ;
#20157=CARTESIAN_POINT ( 'NONE',  ( 9.457646018065525792E-16, -36.06249999863441502, 5.148502694627439702 ) ) ;
#20159=CARTESIAN_POINT ( 'NONE',  ( -2.499999999999996447, -40.70833333060214443, 4.330127018922195425 ) ) ;
#20162=CARTESIAN_POINT ( 'NONE',  ( 9.457646018065525792E-16, -12.06249999863440081, 5.148502694627439702 ) ) ;
#20163=CARTESIAN_POINT ( 'NONE',  ( -4.458734124999999437, -13.56249999863440259, 0.000000000000000000 ) ) ;
#20164=ORIENTED_EDGE ( 'NONE', *, *, #1565, .T. ) ;
#20165=CARTESIAN_POINT ( 'NONE',  ( -2.500000000000000444, -80.16666666666665719, -4.330127018922193649 ) ) ;
#20167=( BOUNDED_CURVE ( )  B_SPLINE_CURVE ( 2, ( #50586, #20691, #11969, #11020, #40296, #17122, #12301, #16172, #35797 ),
 .UNSPECIFIED., .F., .F. ) 
 B_SPLINE_CURVE_WITH_KNOTS ( ( 3, 2, 2, 2, 3 ),
 ( 0.9270833333333333703, 0.9277777777777778123, 0.9291666666666666963, 0.9305555555555555802, 0.9312500000000000222 ),
 .UNSPECIFIED. ) 
 CURVE ( )  GEOMETRIC_REPRESENTATION_ITEM ( )  RATIONAL_B_SPLINE_CURVE ( ( 0.9330127018922194093, 0.9330127018922194093, 1.000000000000000000, 0.8660254037844387076, 1.000000000000000000, 0.8660254037844387076, 1.000000000000000000, 0.9330127018922194093, 0.9330127018922194093 ) ) 
 REPRESENTATION_ITEM ( '' )  );
#20168=CARTESIAN_POINT ( 'NONE',  ( -4.999999999999999112, -87.79166666393550145, 2.886751345948131764 ) ) ;
#20172=CARTESIAN_POINT ( 'NONE',  ( 4.458734124999999437, -29.06249999863440436, -5.460374474430324690E-16 ) ) ;
#20174=VERTEX_POINT ( 'NONE', #60516 ) ;
#20176=CARTESIAN_POINT ( 'NONE',  ( -4.458734125000000326, -163.2500000013655495, -1.846868145590735644 ) ) ;
#20181=CARTESIAN_POINT ( 'NONE',  ( 4.458734124999998549, -75.97916666530106511, -2.574251347313721627 ) ) ;
#20184=CARTESIAN_POINT ( 'NONE',  ( -1.846868145590737420, -148.0000000013656063, 4.458734124999997661 ) ) ;
#20190=CARTESIAN_POINT ( 'NONE',  ( -4.458734124999999437, -142.1875000013656063, -5.460374474430324690E-16 ) ) ;
#20194=CARTESIAN_POINT ( 'NONE',  ( -2.229367062499996610, -74.39583333196773651, 3.861377020970582219 ) ) ;
#20196=FACE_OUTER_BOUND ( 'NONE', #29147, .T. ) ;
#20207=CARTESIAN_POINT ( 'NONE',  ( -3.152548672688508926E-16, 18.18750000136559564, -5.148502694627439702 ) ) ;
#20208=CARTESIAN_POINT ( 'NONE',  ( 1.975475456537005874E-15, -77.62499999726881583, 5.000000000000000000 ) ) ;
#20211=VECTOR ( 'NONE', #4463, 1000.000000000000000 ) ;
#20215=LINE ( 'NONE', #10873, #37701 ) ;
#20216=CARTESIAN_POINT ( 'NONE',  ( -4.458734124999999437, -2.312499998634407028, 0.000000000000000000 ) ) ;
#20218=CARTESIAN_POINT ( 'NONE',  ( -2.229367062500000163, -29.72916666530107221, -3.861377020970580443 ) ) ;
#20222=CARTESIAN_POINT ( 'NONE',  ( 4.458734124999999437, 24.18750000136559564, -5.460374474430324690E-16 ) ) ;
#20226=CARTESIAN_POINT ( 'NONE',  ( 4.458734125000000326, -76.14583333196773651, 2.574251347313718519 ) ) ;
#20229=CARTESIAN_POINT ( 'NONE',  ( 5.000000000000000888, 25.54166666939784847, 2.886751345948126879 ) ) ;
#20230=EDGE_LOOP ( 'NONE', ( #20587, #54388, #41048, #2548 ) ) ;
#20232=DIRECTION ( 'NONE',  ( -0.000000000000000000, 1.000000000000000000, -0.000000000000000000 ) ) ;
#20233=CARTESIAN_POINT ( 'NONE',  ( 1.060575238724906964E-15, -15.75000000000000178, 5.773502691896257311 ) ) ;
#20234=CARTESIAN_POINT ( 'NONE',  ( -2.229367062500000163, -21.47916666530107221, -3.861377020970580443 ) ) ;
#20235=CARTESIAN_POINT ( 'NONE',  ( -4.458734124999997661, -83.22916666530106511, 2.574251347313722516 ) ) ;
#20236=CARTESIAN_POINT ( 'NONE',  ( 5.000000000000000888, -23.45833333060214443, 2.886751345948126879 ) ) ;
#20237=CARTESIAN_POINT ( 'NONE',  ( 4.458734124999998549, -51.72916666530107221, -2.574251347313721627 ) ) ;
#20240=CARTESIAN_POINT ( 'NONE',  ( 5.000000000000000888, -74.45833333060214443, 2.886751345948126879 ) ) ;
#20241=CARTESIAN_POINT ( 'NONE',  ( -4.458734124999998549, 3.520833334698929118, 2.574251347313722516 ) ) ;
#20244=CARTESIAN_POINT ( 'NONE',  ( -4.999999999999999112, -68.91666666666667140, 2.886751345948131764 ) ) ;
#20245=CARTESIAN_POINT ( 'NONE',  ( 1.846868145590736310, -151.8750000013655779, 4.458734124999999437 ) ) ;
#20248=CARTESIAN_POINT ( 'NONE',  ( 2.071067811865476394, -162.1875000000000000, 5.000000000000000000 ) ) ;
#20251=AXIS2_PLACEMENT_3D ( 'NONE', #22118, #11505, #16013 ) ;
#20252=CARTESIAN_POINT ( 'NONE',  ( -3.152548672688508926E-16, -10.81249999863440792, -5.148502694627439702 ) ) ;
#20253=VECTOR ( 'NONE', #4222, 1000.000000000000000 ) ;
#20254=CARTESIAN_POINT ( 'NONE',  ( 4.458734124999998549, -46.97916666530106511, -2.574251347313721627 ) ) ;
#20255=( BOUNDED_CURVE ( )  B_SPLINE_CURVE ( 2, ( #20428, #4665, #48414, #58393, #5314, #43891, #33942, #24610, #63540 ),
 .UNSPECIFIED., .F., .F. ) 
 B_SPLINE_CURVE_WITH_KNOTS ( ( 3, 2, 2, 2, 3 ),
 ( 0.02500000000000002220, 0.02916666666666669488, 0.03333333333333336757, 0.03750000000000003331, 0.04166666666666670599 ),
 .UNSPECIFIED. ) 
 CURVE ( )  GEOMETRIC_REPRESENTATION_ITEM ( )  RATIONAL_B_SPLINE_CURVE ( ( 0.9999999999999996669, 0.9238795325112870716, 1.000000000000000000, 0.9238795325112867385, 1.000000000000000000, 0.9238795325112867385, 1.000000000000000000, 0.9238795325112859613, 1.000000000000000666 ) ) 
 REPRESENTATION_ITEM ( '' )  );
#20257=CARTESIAN_POINT ( 'NONE',  ( 2.730187237215162345E-16, -145.1875000013656063, -4.458734124999999437 ) ) ;
#20262=CARTESIAN_POINT ( 'NONE',  ( -4.458734124999999437, 28.43750000136559208, 0.000000000000000000 ) ) ;
#20264=CARTESIAN_POINT ( 'NONE',  ( -2.498395430326213474E-14, 21.24999999999999289, 5.000000000000000000 ) ) ;
#20265=ORIENTED_EDGE ( 'NONE', *, *, #1264, .T. ) ;
#20269=CARTESIAN_POINT ( 'NONE',  ( -6.972266317189433020E-16, 8.750000000000000000, -5.000000000000000000 ) ) ;
#20270=CARTESIAN_POINT ( 'NONE',  ( -4.458734124999999437, -5.312499998634402587, 0.000000000000000000 ) ) ;
#20271=DIRECTION ( 'NONE',  ( 0.000000000000000000, 0.000000000000000000, 1.000000000000000000 ) ) ;
#20272=CARTESIAN_POINT ( 'NONE',  ( -1.846868145590737420, -149.7500000013656063, 4.458734124999997661 ) ) ;
#20274=ORIENTED_EDGE ( 'NONE', *, *, #24500, .F. ) ;
#20280=CARTESIAN_POINT ( 'NONE',  ( -1.339745962155610925, -12.79465819873851906, 5.000000000000000000 ) ) ;
#20287=CARTESIAN_POINT ( 'NONE',  ( 4.458734124999998549, 15.27083333469893134, -2.574251347313721627 ) ) ;
#20290=CARTESIAN_POINT ( 'NONE',  ( -4.458734124999997661, -15.47916666530107399, 2.574251347313722516 ) ) ;
#20292=CARTESIAN_POINT ( 'NONE',  ( 2.730187237215162345E-16, -165.1875000013655779, -4.458734124999999437 ) ) ;
#20293=CARTESIAN_POINT ( 'NONE',  ( -6.972266317189433020E-16, -63.12499999726880162, -5.000000000000000000 ) ) ;
#20298=VECTOR ( 'NONE', #9701, 1000.000000000000000 ) ;
#20302=CARTESIAN_POINT ( 'NONE',  ( -1.846868145590737420, -153.0000000013656063, 4.458734124999997661 ) ) ;
#20311=CARTESIAN_POINT ( 'NONE',  ( 5.000000000000000000, -4.499999999999997335, -6.123233995736766282E-16 ) ) ;
#20312=CARTESIAN_POINT ( 'NONE',  ( -4.458734124999997661, -66.22916666530106511, 2.574251347313722516 ) ) ;
#20313=CARTESIAN_POINT ( 'NONE',  ( 5.000000000000000888, -4.458333330602148870, 2.886751345948126879 ) ) ;
#20314=CARTESIAN_POINT ( 'NONE',  ( -4.458734124999999437, -35.31249999863440792, 0.000000000000000000 ) ) ;
#20315=EDGE_LOOP ( 'NONE', ( #14335, #21271, #26880, #31552 ) ) ;
#20318=ORIENTED_EDGE ( 'NONE', *, *, #36967, .F. ) ;
#20320=CARTESIAN_POINT ( 'NONE',  ( -4.999999999999999112, -49.91666666666666430, 2.886751345948131764 ) ) ;
#20323=CARTESIAN_POINT ( 'NONE',  ( 1.339745962155612702, -32.16965819600733312, -5.000000000000000000 ) ) ;
#20324=CARTESIAN_POINT ( 'NONE',  ( 9.457646018065525792E-16, -74.06249999863440792, 5.148502694627439702 ) ) ;
#20325=CARTESIAN_POINT ( 'NONE',  ( -4.458734124999999437, -142.1875000013656063, -5.460374474430324690E-16 ) ) ;
#20326=CARTESIAN_POINT ( 'NONE',  ( -4.458734124999999437, -83.31249999863439371, 0.000000000000000000 ) ) ;
#20329=CARTESIAN_POINT ( 'NONE',  ( 2.229367062499998831, -30.89583333196773651, -3.861377020970580887 ) ) ;
#20330=CARTESIAN_POINT ( 'NONE',  ( -3.535250795749689387E-16, -73.12499999726881583, -5.773502691896257311 ) ) ;
#20333=ORIENTED_EDGE ( 'NONE', *, *, #11412, .T. ) ;
#20341=CARTESIAN_POINT ( 'NONE',  ( 4.458734125000001214, -57.14583333196773651, 2.574251347313718519 ) ) ;
#20344=CARTESIAN_POINT ( 'NONE',  ( 2.071067811865517694, -141.8125000000000000, -4.999999999999958256 ) ) ;
#20346=CARTESIAN_POINT ( 'NONE',  ( 4.458734124999999437, 13.18750000136559208, -5.460374474430324690E-16 ) ) ;
#20348=CARTESIAN_POINT ( 'NONE',  ( -6.972266317189433020E-16, -27.12499999726881228, -5.000000000000000000 ) ) ;
#20349=CARTESIAN_POINT ( 'NONE',  ( -4.458734124999999437, -162.9375000013655779, -5.460374474430324690E-16 ) ) ;
#20351=DIRECTION ( 'NONE',  ( -0.000000000000000000, 1.000000000000000000, -0.000000000000000000 ) ) ;
#20354=CARTESIAN_POINT ( 'NONE',  ( 0.000000000000000000, -170.0000000000000000, 5.000000000000000000 ) ) ;
#20356=CARTESIAN_POINT ( 'NONE',  ( 1.975475456537005874E-15, -71.75000000000000000, 5.000000000000000000 ) ) ;
#20357=VECTOR ( 'NONE', #61806, 1000.000000000000000 ) ;
#20368=CARTESIAN_POINT ( 'NONE',  ( 4.458734124999999437, 8.937500001365592084, -5.460374474430324690E-16 ) ) ;
#20369=CARTESIAN_POINT ( 'NONE',  ( -1.339745962155610925, -9.669658196007334894, 5.000000000000000000 ) ) ;
#20371=CARTESIAN_POINT ( 'NONE',  ( -9.184850993605147944E-16, -144.3750000027312126, 5.000000000000000000 ) ) ;
#20372=CYLINDRICAL_SURFACE ( 'NONE', #46933, 5.000000000000000000 ) ;
#20376=CARTESIAN_POINT ( 'NONE',  ( 5.000000000000000888, -140.9375000000000284, -2.071067811865475505 ) ) ;
#20379=CARTESIAN_POINT ( 'NONE',  ( 4.458734124999997661, -164.7500000013655779, 1.846868145590737864 ) ) ;
#20380=CARTESIAN_POINT ( 'NONE',  ( 0.000000000000000000, -170.0000000000000000, 5.000000000000000000 ) ) ;
#20383=CARTESIAN_POINT ( 'NONE',  ( 1.846868145590735200, -142.2500000013656063, -4.458734125000000326 ) ) ;
#20384=EDGE_LOOP ( 'NONE', ( #26426, #29537, #45460, #7751 ) ) ;
#20385=CARTESIAN_POINT ( 'NONE',  ( 2.229367062500001939, 26.77083333469892423, 3.861377020970579999 ) ) ;
#20387=CARTESIAN_POINT ( 'NONE',  ( -4.458734124999999437, -64.64583333196773651, -2.574251347313719407 ) ) ;
#20390=CARTESIAN_POINT ( 'NONE',  ( -3.535250795749689387E-16, 15.75000000000000178, -5.773502691896257311 ) ) ;
#20392=CARTESIAN_POINT ( 'NONE',  ( 4.458734124999999437, -48.81249999863440792, -5.460374474430324690E-16 ) ) ;
#20393=CARTESIAN_POINT ( 'NONE',  ( -2.229367062499996610, -11.14583333196773829, 3.861377020970582219 ) ) ;
#20395=CARTESIAN_POINT ( 'NONE',  ( -5.000000000000000000, 13.91666666666666785, -2.886751345948128211 ) ) ;
#20397=FACE_OUTER_BOUND ( 'NONE', #19619, .T. ) ;
#20398=CARTESIAN_POINT ( 'NONE',  ( -2.499999999999996447, -9.833333333333332149, 4.330127018922195425 ) ) ;
#20401=CARTESIAN_POINT ( 'NONE',  ( -5.000000000000000888, -140.6875000027311842, -2.071067811865475949 ) ) ;
#20402=CARTESIAN_POINT ( 'NONE',  ( 2.229367062499998831, -52.64583333196773651, -3.861377020970580887 ) ) ;
#20403=CARTESIAN_POINT ( 'NONE',  ( -4.458734124999999437, -156.1875000013655779, -5.460374474430324690E-16 ) ) ;
#20405=CARTESIAN_POINT ( 'NONE',  ( 5.000000000000000888, -53.45833333060213732, 2.886751345948126879 ) ) ;
#20408=CARTESIAN_POINT ( 'NONE',  ( -3.152548672688508926E-16, 2.187500001365593416, -5.148502694627439702 ) ) ;
#20410=CARTESIAN_POINT ( 'NONE',  ( -5.000000000000000888, -157.6875000027312126, -2.071067811865475949 ) ) ;
#20411=DIRECTION ( 'NONE',  ( 0.000000000000000000, 0.000000000000000000, 1.000000000000000000 ) ) ;
#20412=CARTESIAN_POINT ( 'NONE',  ( -3.152801135295367985, -154.8125000013656063, 3.152801135295367096 ) ) ;
#20415=CARTESIAN_POINT ( 'NONE',  ( 2.500000000000002220, -83.66666666666667140, 4.330127018922192761 ) ) ;
#20418=CARTESIAN_POINT ( 'NONE',  ( 4.458734124999999437, -44.06249999863440081, -5.460374474430324690E-16 ) ) ;
#20423=CARTESIAN_POINT ( 'NONE',  ( 9.457646018065525792E-16, -90.31249999863439371, 5.148502694627439702 ) ) ;
#20425=CARTESIAN_POINT ( 'NONE',  ( -9.184850993605147944E-16, -165.2500000000000000, 5.000000000000000000 ) ) ;
#20428=CARTESIAN_POINT ( 'NONE',  ( -9.184850993605147944E-16, -169.2500000000000000, 5.000000000000000000 ) ) ;
#20430=CARTESIAN_POINT ( 'NONE',  ( -5.000000000000000000, -61.95833333060213732, -2.886751345948128211 ) ) ;
#20433=( BOUNDED_CURVE ( )  B_SPLINE_CURVE ( 2, ( #36664, #41472, #51151, #51780, #42112, #51467, #26699, #17366, #56291, #31506, #32790, #7723, #52420, #7085, #46633, #27327, #8352, #2579, #41796, #47270, #2904, #61123, #22518, #56928, #61757, #27951, #12849, #60802, #3525, #17684, #46316, #2274, #32466, #37299, #37609, #47574, #22836, #36345, #8037, #55976, #57250, #21877, #13166, #23135, #11888, #38249, #24393, #39175, #33414, #13489, #38857, #18926, #63019, #29203, #18626, #34349, #62386, #18307, #38540, #62701, #14417, #28895, #57870, #9595, #43373, #63322, #4455, #14731, #43996, #23772, #63643, #19563, #8654, #28581, #34040, #53978, #33106, #58494, #42742, #28267, #48828, #4155, #37932, #58171, #57564, #52720, #58800, #13791, #19242, #47881, #3840, #29516, #14101, #4767, #53031, #8970, #43063, #9906, #49148, #33727, #53345, #53661, #9280, #48202, #23459, #48516, #5094, #24084, #43679, #30157, #20850, #55268, #11507, #29841, #15701, #19879, #16015, #25674, #44639, #5411, #15063, #6062, #15383, #54296, #25347, #598, #59129, #60415, #931, #16340, #34677, #35007, #44968, #35962, #59452, #20207, #11186, #54622, #10866, #10546, #39810, #49786, #55587, #40453, #24712, #31123, #50106, #10236, #49473, #60093, #45283, #6380, #50745, #50439, #44317, #5732, #281, #1249, #25028, #20536, #40133, #39493, #59775, #35320, #54940, #30482, #35641, #30809, #25986, #45602, #1560, #21162, #40769, #7960, #7646, #56217, #61992, #47193, #41400, #55900, #22440, #21486, #57173, #7334, #37226, #61051, #21805, #7012, #42353, #32392, #31759, #26945, #41712, #27250, #61361, #31431, #6690, #17610, #46877, #41084, #37532, #2820, #56852, #13089, #11812, #17284, #1881, #61677, #42036, #26620, #51069, #60730, #46561, #51706, #16972, #36277, #2502, #46239, #16652, #17911, #22120, #12769, #27560, #12458, #36907, #45919, #36583, #56538, #32069, #52017, #2201, #3136, #22755, #12137, #32710, #26295, #51392, #59613, #14887, #43522, #63166, #59283, #47495, #58334, #9743, #44475, #20368, #48982, #4931, #24550, #14260, #58648, #34494, #8272, #48665, #9432, #4606, #125, #33882, #29680, #44154, #53502, #34840, #49632, #43835, #23920, #49310, #29348, #19719, #39644, #29042, #44796, #27876, #3448, #39328, #24229, #24874, #19077, #58961, #434, #38697, #10067, #54129, #25182, #54464, #34190, #10390, #30000, #63481, #39019, #20040, #760, #19401, #5252, #52338, #14568, #5568, #15214, #53813, #39967, #15545, #11023, #55737, #45121, #49940, #21956, #35800, #2038, #25827, #50266, #35481, #7172, #60883, #60256, #55423, #6529, #36114, #26143, #59937, #35165, #46080, #21643, #55097, #40612, #31273, #41236, #41552, #40299, #45762, #30319, #26463, #11653, #30644, #15859, #25502, #11341, #16493, #45442, #1086, #30964, #6214, #1716, #50907, #11972, #16808, #36428, #40925, #50589, #10712, #1405, #21324, #60568, #56056, #21007, #6849, #31602, #16175, #46399, #51236, #54781, #61203, #26781, #2348, #5895, #20694, #12305, #22276, #37378, #8433, #47965, #12926, #32548, #52174, #41877, #22601, #62149, #36751, #12614, #37076, #32227, #27722, #52804, #61524, #28037, #17454, #62471, #13571, #7801, #51547, #13247, #57011, #8118, #3608, #56698, #8741, #56381, #31920, #47349, #51858, #52499, #7483, #27403, #47655, #17761, #37689, #42511, #28348, #18391, #61841, #38010, #57643, #46712, #2984, #23216, #3920, #27096, #32870, #17125, #2657, #42826, #33189, #47034, #42198, #57331, #3298, #23539, #22919, #18067, #43138, #29605, #5178, #57952, #4233, #19326, #54055, #29927, #58576, #14495, #34117, #23848, #4535, #53738, #9359, #14182, #9671, #44400, #29279, #34763, #43451, #9992, #63096, #359, #59212, #53426, #33498, #58881, #38940, #48909, #49235, #38621, #54389, #4854, #28971, #19008, #48594, #33809, #24474, #58258, #24795, #63408, #19644, #44081, #10315, #19961, #43763, #39572, #15141, #28661, #24160, #34426, #49552, #45, #39255, #14812, #5494, #48277, #25108, #18698, #62778, #13873, #38323, #53115, #9051, #1646, #54708, #59537, #31520, #45369, #11587, #35401, #59860, #31206, #15471, #35088, #20619, #60814, #21245, #35723, #40225, #30241, #20932, #16739, #50836, #45048, #50189, #40852, #6776, #51163, #49864, #55353, #39891, #6141, #50522, #7096, #10628, #25756, #26387, #36356, #5812, #46004, #44718, #1335, #11267, #60495, #21570, #1969, #41167, #6462, #40537, #20290, #10945, #55986, #15785, #30892, #30564, #36042, #55023, #11900, #681, #60178, #26071, #25429, #1015, #16100, #45689, #16423, #55672, #57258, #33115, #32153, #56936, #2912, #62395, #36674, #37000, #46967, #37941, #61450, #22207, #13175, #17380, #12857, #12540, #46643, #26710, #56304, #47278, #7415, #62077, #51789, #27025, #17057, #17991, #3227, #8360, #57573, #52428, #46325, #7731, #2284, #22845, #2588, #41806, #42123, #17692, #56626, #27336, #61765, #27961, #37307, #18316, #22527, #8046, #47584, #12232, #21887, #32476, #52732, #41483, #13499, #52105, #27651, #42435, #37617, #32799, #3535, #23144, #42752, #61134, #31846, #51478, #28277, #23468, #43071, #63653, #62709, #15072, #44006, #4777, #38550, #24404, #34048, #19572, #9288, #58503, #28589, #14426, #39184, #57878, #33735, #47891, #58182, #290, #49159, #43382, #13803, #58810, #63334, #34357, #5104, #14741, #9915, #4164, #53671, #53987, #18635, #38257, #48210, #24722, #48837, #19252, #33423, #8664, #29524, #29212, #53041, #39502, #44326, #19888, #59138, #14110, #34685, #3847, #63027, #8979, #23780, #38866, #18934, #53353, #28905, #48525, #4466, #24093, #43688, #9604, #15711, #54949, #25685, #55279, #45294, #15393, #54305, #1572, #11198, #25036, #21497, #30821, #50452, #1893, #45616, #49795, #49483, #21172, #6392, #10555, #35017, #44648, #30494, #35653, #44978, #20218, #10878, #30166, #609, #26308, #50116, #45930, #39819, #943, #6072, #41095, #5740, #40780, #25359, #40465, #40143, #20546, #10247, #59460, #25997, #54631, #60426, #35329, #59787, #35973, #16351, #55600, #5421, #1259, #20862, #11518, #60105, #29850, #31133, #16026, #50757, #6702, #60742, #16665, #51402, #51717, #17922, #7658, #8283, #41412, #47204, #36594, #37544, #32720, #26955, #7023, #55911, #23073, #2514, #27263, #46888, #2832, #22450, #22130, #56230, #46573, #7344, #42047, #12151, #3148, #36919, #56863, #61690, #27887, #57183, #17294, #32403, #41723, #52030, #17621, #22768, #56549, #37237, #31770, #12781, #42364, #21815, #61373, #11823, #62003, #36288, #12469, #31441, #7972, #32080, #27571, #13103, #51085, #52348, #47509, #3459, #42677, #61063, #62317, #26631, #46251, #2212, #16982, #13417, #4390, #44249, #37867, #5023, #48136, #53280, #9215, #57499, #33039, #58104, #38182, #53595, #52655, #28829, #9527, #8590, #28200, #47815, #29133, #3772, #24642, #48756, #14353, #4087, #33975, #43612, #4698, #23396, #24320, #18242, #42996, #43927, #63574, #19493, #19170, #23711, #9832, #58736, #52965, #62639, #39108, #48451, #14662, #34282, #53906, #29443, #13726, #18560, #49075, #57804, #43307, #18857, #24009, #38787, #63254, #33350, #8902, #28518, #58426, #62943, #38477, #14033, #33662, #11438, #55197, #59378, #21098, #11117, #1182, #20139, #44570, #54226, #40062, #45217, #54555, #29769, #860, #39738, #34595, #35894, #59705, #55526, #10164, #10478, #20463, #31056, #34934, #50040, #54873, #45534, #528, #10804, #60028, #30091, #50679, #15951, #213, #6621, #25603, #49403, #5347, #35573, #20782, #1495, #26234, #5666, #40387, #49721, #15312, #15637, #40702, #35253, #19811, #24965, #30744, #25279, #60347, #16275, #44901, #30416, #50365, #5999, #6312, #25916, #39420, #59059, #14986, #12072, #46177, #36520, #60983, #32013, #2138, #12712, #46496, #2755, #7581, #17854, #47130, #26882, #27501, #3078, #11747, #31697, #17551, #37476, #16590, #21741, #51647, #56794, #31365, #7270, #1816, #2444, #60667, #21420, #42294, #41337, #22375, #55832, #36210, #32645, #22053, #32328, #56150, #16904, #51331, #51006, #6946, #41646, #61935, #41975, #36847, #61298, #26557, #17220, #57111, #51958, #56477, #12399, #61617, #7896, #52276, #27193, #46809, #41023, #37171, #22696, #8213, #13028, #45854, #33901, #19425, #32967, #58354, #34208, #33279, #58035, #23941, #4625, #53524, #29061, #33592, #48063, #3393, #57734, #13965, #9452, #28132, #38411, #43542, #62569, #39038, #63186, #27816, #53833, #53211, #18168, #37795, #19097, #48379, #48685, #58665, #24250, #47441, #52899, #23010, #23637, #52590, #38715, #18784, #43854, #63500, #14282, #14588, #23321, #9145, #42611, #62249, #57425, #3706, #13346, #4321, #28754, #42922, #8522, #4015, #47750, #18488, #38111, #13660, #8835, #28448, #43231, #62873, #30667, #15880, #15234, #15565, #36685, #4949, #34862, #35500, #1426, #14910, #40319, #17067, #44177, #45461, #49650, #21025, #19738, #20061, #30022, #40632, #44495, #5273, #59957, #457, #59632, #59302, #29699, #9762, #39352, #30338, #54149, #45141, #35185, #144, #58982, #1105, #49964, #55118, #61145, #11043, #29369, #54483, #49002, #5917, #10088, #24894, #25204, #780, #39665, #10410, #44818, #50287, #34518, #25523, #5587, #54803, #6234, #49330, #24572, #10731, #20387, #39987, #20714, #25844, #27660, #47288, #3238, #22854, #22538, #56637, #46975, #7740, #42445, #27973, #12242, #7426, #27035, #47594, #46652, #62717, #3546, #52438, #42134, #8372, #18004, #23154, #56946, #62087, #12551, #37627, #42763, #41814, #57584, #57268, #61775, #47899, #33127, #27344, #61461, #3855, #31855, #51488, #32485, #32163, #62405, #2597, #13186, #18327, #22217, #17393, #37008, #37951, #13511, #37316, #52744, #8673, #51798, #17702, #28287, #23476, #2923, #43079, #56319, #12867, #18642, #52114, #8058, #32809, #24100, #29856, #15078, #9295, #58817, #48217, #53050, #25044, #38875, #5110, #28911, #53361, #38560, #10255, #297, #63344, #58509, #9611, #39192, #29218, #63034, #38264, #49170, #14747, #58189, #43696, #34364, #24729, #44655, #43389, #48844, #33431, #29533, #53994, #14118, #18942, #28599, #14433, #19578, #48534, #44331, #616, #19258, #4785, #34056, #49489, #4172, #4473, #53678, #5427, #24412, #33744, #19894, #44013, #63661, #9921, #39509, #57886, #23787, #59146, #34691, #54316, #13812, #8987, #10563, #55609, #40787, #1900, #31452, #45937, #20226, #25691, #39826, #60434, #20552, #35337, #35662, #11207, #30502, #54956, #55287, #21507, #30830, #55918, #16033, #1580, #41104, #5748, #15402, #6399, #46260, #59469, #7030, #50124, #50459, #26007, #45625, #11832, #25366, #31141, #40153, #60749, #16674, #10886, #35027, #54639, #26641, #6081, #21180, #16359, #35980, #11525, #45301, #59797, #1268, #20870, #50767, #15718, #6710, #40472, #26318, #36295, #51093, #30173, #49803, #44986, #952, #60112, #37553, #57510, #36607, #62011, #2219, #31779, #32730, #13113, #3470, #3158, #51727, #13426, #42686, #36931, #51410, #17929, #16991, #52666, #2841, #52357, #56557, #17304, #2524, #37878, #27898, #27274, #22461, #37246, #22777, #56873, #26963, #21822, #8295, #42372, #56239, #33052, #57193, #47519, #8600, #7353, #12791, #61070, #23083, #62330, #22139, #46582, #12160, #18251, #28210, #41734, #41421, #42058, #61384, #12478, #32091, #61700, #7667, #46900, #7982, #17629, #32412, #52043, #27580, #47215, #29456, #48146, #58434, #43936, #18870, #59070, #63583, #47824, #54235, #9539, #38191, #57816, #53915, #43005, #52974, #4399, #39117, #14995, #43623, #63265, #19183, #8915, #53289, #29143, #3783, #43317, #4098, #62952, #23721, #222, #24335, #38796, #28528, #23406, #58744, #4710, #18570, #34608, #19504, #14672, #10176, #34293, #38487, #5033, #9841, #9225, #53605, #62651, #13738, #14362, #33359, #58114 ),
 .UNSPECIFIED., .F., .F. ) 
 B_SPLINE_CURVE_WITH_KNOTS ( ( 3, 2, 2, 2, 2, 2, 2, 2, 2, 2, 2, 2, 2, 2, 2, 2, 2, 2, 2, 2, 2, 2, 2, 2, 2, 2, 2, 2, 2, 2, 2, 2, 2, 2, 2, 2, 2, 2, 2, 2, 2, 2, 2, 2, 2, 2, 2, 2, 2, 2, 2, 2, 2, 2, 2, 2, 2, 2, 2, 2, 2, 2, 2, 2, 2, 2, 2, 2, 2, 2, 2, 2, 2, 2, 2, 2, 2, 2, 2, 2, 2, 2, 2, 2, 2, 2, 2, 2, 2, 2, 2, 2, 2, 2, 2, 2, 2, 2, 2, 2, 2, 2, 2, 2, 2, 2, 2, 2, 2, 2, 2, 2, 2, 2, 2, 2, 2, 2, 2, 2, 2, 2, 2, 2, 2, 2, 2, 2, 2, 2, 2, 2, 2, 2, 2, 2, 2, 2, 2, 2, 2, 2, 2, 2, 2, 2, 2, 2, 2, 2, 2, 2, 2, 2, 2, 2, 2, 2, 2, 2, 2, 2, 2, 2, 2, 2, 2, 2, 2, 2, 2, 2, 2, 2, 2, 2, 2, 2, 2, 2, 2, 2, 2, 2, 2, 2, 2, 2, 2, 2, 2, 2, 2, 2, 2, 2, 2, 2, 2, 2, 2, 2, 2, 2, 2, 2, 2, 2, 2, 2, 2, 2, 2, 2, 2, 2, 2, 2, 2, 2, 2, 2, 2, 2, 2, 2, 2, 2, 2, 2, 2, 2, 2, 2, 2, 2, 2, 2, 2, 2, 2, 2, 2, 2, 2, 2, 2, 2, 2, 2, 2, 2, 2, 2, 2, 2, 2, 2, 2, 2, 2, 2, 2, 2, 2, 2, 2, 2, 2, 2, 2, 2, 2, 2, 2, 2, 2, 2, 2, 2, 2, 2, 2, 2, 2, 2, 2, 2, 2, 2, 2, 2, 2, 2, 2, 2, 2, 2, 2, 2, 2, 2, 2, 2, 2, 2, 2, 2, 2, 2, 2, 2, 2, 2, 2, 2, 2, 2, 2, 2, 2, 2, 2, 2, 2, 2, 2, 2, 2, 2, 2, 2, 2, 2, 2, 2, 2, 2, 2, 2, 2, 2, 2, 2, 2, 2, 2, 2, 2, 2, 2, 2, 2, 2, 2, 2, 2, 2, 2, 2, 2, 2, 2, 2, 2, 2, 2, 2, 2, 2, 2, 2, 2, 2, 2, 2, 2, 2, 2, 2, 2, 2, 2, 2, 2, 2, 2, 2, 2, 2, 2, 2, 2, 2, 2, 2, 2, 2, 2, 2, 2, 2, 2, 2, 2, 2, 2, 2, 2, 2, 2, 2, 2, 2, 2, 2, 2, 2, 2, 2, 2, 2, 2, 2, 2, 2, 2, 2, 2, 2, 2, 2, 2, 2, 2, 2, 2, 2, 2, 2, 2, 2, 2, 2, 2, 2, 2, 2, 2, 2, 2, 2, 2, 2, 2, 2, 2, 2, 2, 2, 2, 2, 2, 2, 2, 2, 2, 2, 2, 2, 2, 2, 2, 2, 2, 2, 2, 2, 2, 2, 2, 2, 2, 2, 2, 2, 2, 2, 2, 2, 2, 2, 2, 2, 2, 2, 2, 2, 2, 2, 2, 2, 2, 2, 2, 2, 2, 2, 2, 2, 2, 2, 2, 2, 2, 2, 2, 2, 2, 2, 2, 2, 2, 2, 2, 2, 2, 2, 2, 2, 2, 2, 2, 2, 2, 2, 2, 2, 2, 2, 2, 2, 2, 2, 2, 2, 2, 2, 2, 2, 2, 2, 2, 2, 2, 2, 2, 2, 2, 2, 2, 2, 2, 2, 2, 2, 2, 2, 2, 2, 2, 2, 2, 2, 2, 2, 2, 2, 2, 2, 2, 2, 2, 2, 2, 2, 2, 2, 2, 2, 2, 2, 2, 2, 2, 2, 2, 2, 2, 2, 2, 2, 2, 2, 2, 2, 2, 2, 2, 2, 2, 2, 2, 2, 2, 2, 2, 2, 2, 2, 2, 2, 2, 2, 2, 2, 2, 2, 2, 2, 2, 2, 2, 2, 2, 2, 2, 2, 2, 2, 2, 2, 2, 2, 2, 2, 2, 2, 2, 2, 2, 2, 2, 2, 2, 2, 2, 2, 2, 2, 2, 2, 2, 2, 2, 2, 2, 2, 2, 2, 2, 2, 2, 2, 2, 2, 2, 2, 2, 2, 2, 2, 2, 2, 2, 2, 2, 2, 2, 2, 2, 2, 2, 2, 2, 2, 2, 2, 2, 2, 2, 2, 2, 2, 2, 2, 2, 2, 2, 2, 2, 2, 2, 2, 2, 2, 2, 2, 2, 2, 3 ),
 ( 0.000000000000000000, 0.001388888888888888942, 0.002777777777777777884, 0.004166666666666666609, 0.005555555555555555768, 0.006944444444444444059, 0.008333333333333333218, 0.009722222222222222376, 0.01111111111111111154, 0.01250000000000000069, 0.01388888888888888812, 0.01527777777777777728, 0.01666666666666666644, 0.01805555555555555386, 0.01944444444444444475, 0.02083333333333333218, 0.02222222222222222307, 0.02361111111111111049, 0.02500000000000000139, 0.02638888888888888881, 0.02777777777777777624, 0.02916666666666666713, 0.03055555555555555455, 0.03194444444444444198, 0.03333333333333333287, 0.03472222222222222376, 0.03611111111111110772, 0.03749999999999999861, 0.03888888888888888951, 0.04027777777777778040, 0.04166666666666666435, 0.04305555555555555525, 0.04444444444444444614, 0.04583333333333333010, 0.04722222222222222099, 0.04861111111111111188, 0.05000000000000000278, 0.05138888888888888673, 0.05277777777777777762, 0.05416666666666666852, 0.05555555555555555247, 0.05694444444444444337, 0.05833333333333333426, 0.05972222222222222515, 0.06111111111111110911, 0.06250000000000000000, 0.06388888888888888395, 0.06527777777777778179, 0.06666666666666666574, 0.06805555555555554970, 0.06944444444444444753, 0.07083333333333333148, 0.07222222222222221544, 0.07361111111111111327, 0.07499999999999999722, 0.07638888888888889506, 0.07777777777777777901, 0.07916666666666666297, 0.08055555555555556080, 0.08194444444444444475, 0.08333333333333332871, 0.08472222222222222654, 0.08611111111111111049, 0.08749999999999999445, 0.08888888888888889228, 0.09027777777777777624, 0.09166666666666666019, 0.09305555555555555802, 0.09444444444444444198, 0.09583333333333333981, 0.09722222222222222376, 0.09861111111111110772, 0.1000000000000000056, 0.1013888888888888895, 0.1027777777777777735, 0.1041666666666666713, 0.1055555555555555552, 0.1069444444444444392, 0.1083333333333333370, 0.1097222222222222210, 0.1111111111111111049, 0.1125000000000000028, 0.1138888888888888867, 0.1152777777777777846, 0.1166666666666666685, 0.1180555555555555525, 0.1194444444444444503, 0.1208333333333333343, 0.1222222222222222182, 0.1236111111111111160, 0.1250000000000000000, 0.1263888888888888840, 0.1277777777777777679, 0.1291666666666666796, 0.1305555555555555636, 0.1319444444444444475, 0.1333333333333333315, 0.1347222222222222154, 0.1361111111111110994, 0.1375000000000000111, 0.1388888888888888951, 0.1402777777777777790, 0.1416666666666666630, 0.1430555555555555469, 0.1444444444444444309, 0.1458333333333333426, 0.1472222222222222265, 0.1486111111111111105, 0.1499999999999999944, 0.1513888888888888784, 0.1527777777777777901, 0.1541666666666666741, 0.1555555555555555580, 0.1569444444444444420, 0.1583333333333333259, 0.1597222222222222099, 0.1611111111111111216, 0.1625000000000000056, 0.1638888888888888895, 0.1652777777777777735, 0.1666666666666666574, 0.1680555555555555691, 0.1694444444444444531, 0.1708333333333333370, 0.1722222222222222210, 0.1736111111111111049, 0.1749999999999999889, 0.1763888888888889006, 0.1777777777777777846, 0.1791666666666666685, 0.1805555555555555525, 0.1819444444444444364, 0.1833333333333333204, 0.1847222222222222321, 0.1861111111111111160, 0.1875000000000000000, 0.1888888888888888840, 0.1902777777777777679, 0.1916666666666666796, 0.1930555555555555636, 0.1944444444444444475, 0.1958333333333333315, 0.1972222222222222154, 0.1986111111111110994, 0.2000000000000000111, 0.2013888888888888951, 0.2027777777777777790, 0.2041666666666666630, 0.2055555555555555469, 0.2069444444444444309, 0.2083333333333333426, 0.2097222222222222265, 0.2111111111111111105, 0.2124999999999999944, 0.2138888888888888784, 0.2152777777777777901, 0.2166666666666666741, 0.2180555555555555580, 0.2194444444444444420, 0.2208333333333333259, 0.2222222222222222099, 0.2236111111111111216, 0.2250000000000000056, 0.2263888888888888895, 0.2277777777777777735, 0.2291666666666666574, 0.2305555555555555691, 0.2319444444444444531, 0.2333333333333333370, 0.2347222222222222210, 0.2361111111111111049, 0.2374999999999999889, 0.2388888888888889006, 0.2402777777777777846, 0.2416666666666666685, 0.2430555555555555525, 0.2444444444444444364, 0.2458333333333333204, 0.2472222222222222321, 0.2486111111111111160, 0.2500000000000000000, 0.2513888888888888840, 0.2527777777777777679, 0.2541666666666666519, 0.2555555555555555358, 0.2569444444444444198, 0.2583333333333333592, 0.2597222222222222432, 0.2611111111111111271, 0.2625000000000000111, 0.2638888888888888951, 0.2652777777777777790, 0.2666666666666666630, 0.2680555555555555469, 0.2694444444444444309, 0.2708333333333333148, 0.2722222222222221988, 0.2736111111111111382, 0.2750000000000000222, 0.2763888888888889062, 0.2777777777777777901, 0.2791666666666666741, 0.2805555555555555580, 0.2819444444444444420, 0.2833333333333333259, 0.2847222222222222099, 0.2861111111111110938, 0.2874999999999999778, 0.2888888888888888618, 0.2902777777777778012, 0.2916666666666666852, 0.2930555555555555691, 0.2944444444444444531, 0.2958333333333333370, 0.2972222222222222210, 0.2986111111111111049, 0.2999999999999999889, 0.3013888888888888729, 0.3027777777777777568, 0.3041666666666666408, 0.3055555555555555802, 0.3069444444444444642, 0.3083333333333333481, 0.3097222222222222321, 0.3111111111111111160, 0.3125000000000000000, 0.3138888888888888840, 0.3152777777777777679, 0.3166666666666666519, 0.3180555555555555358, 0.3194444444444444198, 0.3208333333333333592, 0.3222222222222222432, 0.3236111111111111271, 0.3250000000000000111, 0.3263888888888888951, 0.3277777777777777790, 0.3291666666666666630, 0.3305555555555555469, 0.3319444444444444309, 0.3333333333333333148, 0.3347222222222221988, 0.3361111111111111382, 0.3375000000000000222, 0.3388888888888889062, 0.3402777777777777901, 0.3416666666666666741, 0.3430555555555555580, 0.3444444444444444420, 0.3458333333333333259, 0.3472222222222222099, 0.3486111111111110938, 0.3499999999999999778, 0.3513888888888888618, 0.3527777777777778012, 0.3541666666666666852, 0.3555555555555555691, 0.3569444444444444531, 0.3583333333333333370, 0.3597222222222222210, 0.3611111111111111049, 0.3624999999999999889, 0.3638888888888888729, 0.3652777777777777568, 0.3666666666666666408, 0.3680555555555555802, 0.3694444444444444642, 0.3708333333333333481, 0.3722222222222222321, 0.3736111111111111160, 0.3750000000000000000, 0.3763888888888888840, 0.3777777777777777679, 0.3791666666666666519, 0.3805555555555555358, 0.3819444444444444198, 0.3833333333333333592, 0.3847222222222222432, 0.3861111111111111271, 0.3875000000000000111, 0.3888888888888888951, 0.3902777777777777790, 0.3916666666666666630, 0.3930555555555555469, 0.3944444444444444309, 0.3958333333333333148, 0.3972222222222221988, 0.3986111111111111382, 0.4000000000000000222, 0.4013888888888889062, 0.4027777777777777901, 0.4041666666666666741, 0.4055555555555555580, 0.4069444444444444420, 0.4083333333333333259, 0.4097222222222222099, 0.4111111111111110938, 0.4124999999999999778, 0.4138888888888888618, 0.4152777777777778012, 0.4166666666666666852, 0.4180555555555555691, 0.4194444444444444531, 0.4208333333333333370, 0.4222222222222222210, 0.4236111111111111049, 0.4249999999999999889, 0.4263888888888888729, 0.4277777777777777568, 0.4291666666666666408, 0.4305555555555555802, 0.4319444444444444642, 0.4333333333333333481, 0.4347222222222222321, 0.4361111111111111160, 0.4375000000000000000, 0.4388888888888888840, 0.4402777777777777679, 0.4416666666666666519, 0.4430555555555555358, 0.4444444444444444198, 0.4458333333333333592, 0.4472222222222222432, 0.4486111111111111271, 0.4500000000000000111, 0.4513888888888888951, 0.4527777777777777790, 0.4541666666666666630, 0.4555555555555555469, 0.4569444444444444309, 0.4583333333333333148, 0.4597222222222221988, 0.4611111111111111382, 0.4625000000000000222, 0.4638888888888889062, 0.4652777777777777901, 0.4666666666666666741, 0.4680555555555555580, 0.4694444444444444420, 0.4708333333333333259, 0.4722222222222222099, 0.4736111111111110938, 0.4749999999999999778, 0.4763888888888888618, 0.4777777777777778012, 0.4791666666666666852, 0.4805555555555555691, 0.4819444444444444531, 0.4833333333333333370, 0.4847222222222222210, 0.4861111111111111049, 0.4874999999999999889, 0.4888888888888888729, 0.4902777777777777568, 0.4916666666666666408, 0.4930555555555555802, 0.4944444444444444642, 0.4958333333333333481, 0.4972222222222222321, 0.4986111111111111160, 0.5000000000000000000, 0.5013888888888888840, 0.5027777777777777679, 0.5041666666666666519, 0.5055555555555555358, 0.5069444444444444198, 0.5083333333333333037, 0.5097222222222221877, 0.5111111111111110716, 0.5124999999999999556, 0.5138888888888888395, 0.5152777777777777235, 0.5166666666666667185, 0.5180555555555556024, 0.5194444444444444864, 0.5208333333333333703, 0.5222222222222222543, 0.5236111111111111382, 0.5250000000000000222, 0.5263888888888889062, 0.5277777777777777901, 0.5291666666666666741, 0.5305555555555555580, 0.5319444444444444420, 0.5333333333333333259, 0.5347222222222222099, 0.5361111111111110938, 0.5374999999999999778, 0.5388888888888888618, 0.5402777777777777457, 0.5416666666666666297, 0.5430555555555555136, 0.5444444444444443976, 0.5458333333333332815, 0.5472222222222222765, 0.5486111111111111605, 0.5500000000000000444, 0.5513888888888889284, 0.5527777777777778123, 0.5541666666666666963, 0.5555555555555555802, 0.5569444444444444642, 0.5583333333333333481, 0.5597222222222222321, 0.5611111111111111160, 0.5625000000000000000, 0.5638888888888888840, 0.5652777777777777679, 0.5666666666666666519, 0.5680555555555555358, 0.5694444444444444198, 0.5708333333333333037, 0.5722222222222221877, 0.5736111111111110716, 0.5749999999999999556, 0.5763888888888888395, 0.5777777777777777235, 0.5791666666666667185, 0.5805555555555556024, 0.5819444444444444864, 0.5833333333333333703, 0.5847222222222222543, 0.5861111111111111382, 0.5875000000000000222, 0.5888888888888889062, 0.5902777777777777901, 0.5916666666666666741, 0.5930555555555555580, 0.5944444444444444420, 0.5958333333333333259, 0.5972222222222222099, 0.5986111111111110938, 0.5999999999999999778, 0.6013888888888888618, 0.6027777777777777457, 0.6041666666666666297, 0.6055555555555555136, 0.6069444444444443976, 0.6083333333333332815, 0.6097222222222222765, 0.6111111111111111605, 0.6125000000000000444, 0.6138888888888889284, 0.6152777777777778123, 0.6166666666666666963, 0.6180555555555555802, 0.6194444444444444642, 0.6208333333333333481, 0.6222222222222222321, 0.6236111111111111160, 0.6250000000000000000, 0.6263888888888888840, 0.6277777777777777679, 0.6291666666666666519, 0.6305555555555555358, 0.6319444444444444198, 0.6333333333333333037, 0.6347222222222221877, 0.6361111111111110716, 0.6374999999999999556, 0.6388888888888888395, 0.6402777777777777235, 0.6416666666666667185, 0.6430555555555556024, 0.6444444444444444864, 0.6458333333333333703, 0.6472222222222222543, 0.6486111111111111382, 0.6500000000000000222, 0.6513888888888889062, 0.6527777777777777901, 0.6541666666666666741, 0.6555555555555555580, 0.6569444444444444420, 0.6583333333333333259, 0.6597222222222222099, 0.6611111111111110938, 0.6624999999999999778, 0.6638888888888888618, 0.6652777777777777457, 0.6666666666666666297, 0.6680555555555555136, 0.6694444444444443976, 0.6708333333333332815, 0.6722222222222222765, 0.6736111111111111605, 0.6750000000000000444, 0.6763888888888889284, 0.6777777777777778123, 0.6791666666666666963, 0.6805555555555555802, 0.6819444444444444642, 0.6833333333333333481, 0.6847222222222222321, 0.6861111111111111160, 0.6875000000000000000, 0.6888888888888888840, 0.6902777777777777679, 0.6916666666666666519, 0.6930555555555555358, 0.6944444444444444198, 0.6958333333333333037, 0.6972222222222221877, 0.6986111111111110716, 0.6999999999999999556, 0.7013888888888888395, 0.7027777777777777235, 0.7041666666666667185, 0.7055555555555556024, 0.7069444444444444864, 0.7083333333333333703, 0.7097222222222222543, 0.7111111111111111382, 0.7125000000000000222, 0.7138888888888889062, 0.7152777777777777901, 0.7166666666666666741, 0.7180555555555555580, 0.7194444444444444420, 0.7208333333333333259, 0.7222222222222222099, 0.7236111111111110938, 0.7249999999999999778, 0.7263888888888888618, 0.7277777777777777457, 0.7291666666666666297, 0.7305555555555555136, 0.7319444444444443976, 0.7333333333333332815, 0.7347222222222222765, 0.7361111111111111605, 0.7375000000000000444, 0.7388888888888889284, 0.7402777777777778123, 0.7416666666666666963, 0.7430555555555555802, 0.7444444444444444642, 0.7458333333333333481, 0.7472222222222222321, 0.7486111111111111160, 0.7500000000000000000, 0.7513888888888888840, 0.7527777777777777679, 0.7541666666666666519, 0.7555555555555555358, 0.7569444444444444198, 0.7583333333333333037, 0.7597222222222221877, 0.7611111111111110716, 0.7624999999999999556, 0.7638888888888888395, 0.7652777777777777235, 0.7666666666666667185, 0.7680555555555556024, 0.7694444444444444864, 0.7708333333333333703, 0.7722222222222222543, 0.7736111111111111382, 0.7750000000000000222, 0.7763888888888889062, 0.7777777777777777901, 0.7791666666666666741, 0.7805555555555555580, 0.7819444444444444420, 0.7833333333333333259, 0.7847222222222222099, 0.7861111111111110938, 0.7874999999999999778, 0.7888888888888888618, 0.7902777777777777457, 0.7916666666666666297, 0.7930555555555555136, 0.7944444444444443976, 0.7958333333333332815, 0.7972222222222222765, 0.7986111111111111605, 0.8000000000000000444, 0.8013888888888889284, 0.8027777777777778123, 0.8041666666666666963, 0.8055555555555555802, 0.8069444444444444642, 0.8083333333333333481, 0.8097222222222222321, 0.8111111111111111160, 0.8125000000000000000, 0.8138888888888888840, 0.8152777777777777679, 0.8166666666666666519, 0.8180555555555555358, 0.8194444444444444198, 0.8208333333333333037, 0.8222222222222221877, 0.8236111111111110716, 0.8249999999999999556, 0.8263888888888888395, 0.8277777777777777235, 0.8291666666666667185, 0.8305555555555556024, 0.8319444444444444864, 0.8333333333333333703, 0.8347222222222222543, 0.8361111111111111382, 0.8375000000000000222, 0.8388888888888889062, 0.8402777777777777901, 0.8416666666666666741, 0.8430555555555555580, 0.8444444444444444420, 0.8458333333333333259, 0.8472222222222222099, 0.8486111111111110938, 0.8499999999999999778, 0.8513888888888888618, 0.8527777777777777457, 0.8541666666666666297, 0.8555555555555555136, 0.8569444444444443976, 0.8583333333333332815, 0.8597222222222222765, 0.8611111111111111605, 0.8625000000000000444, 0.8638888888888889284, 0.8652777777777778123, 0.8666666666666666963, 0.8680555555555555802, 0.8694444444444444642, 0.8708333333333333481, 0.8722222222222222321, 0.8736111111111111160, 0.8750000000000000000, 0.8763888888888888840, 0.8777777777777777679, 0.8791666666666666519, 0.8805555555555555358, 0.8819444444444444198, 0.8833333333333333037, 0.8847222222222221877, 0.8861111111111110716, 0.8874999999999999556, 0.8888888888888888395, 0.8902777777777777235, 0.8916666666666667185, 0.8930555555555556024, 0.8944444444444444864, 0.8958333333333333703, 0.8972222222222222543, 0.8986111111111111382, 0.9000000000000000222, 0.9013888888888889062, 0.9027777777777777901, 0.9041666666666666741, 0.9055555555555555580, 0.9069444444444444420, 0.9083333333333333259, 0.9097222222222222099, 0.9111111111111110938, 0.9124999999999999778, 0.9138888888888888618, 0.9152777777777777457, 0.9166666666666666297, 0.9180555555555555136, 0.9194444444444443976, 0.9208333333333332815, 0.9222222222222222765, 0.9236111111111111605, 0.9250000000000000444, 0.9263888888888889284, 0.9277777777777778123, 0.9291666666666666963, 0.9305555555555555802, 0.9319444444444444642, 0.9333333333333333481, 0.9347222222222222321, 0.9361111111111111160, 0.9375000000000000000, 0.9388888888888888840, 0.9402777777777777679, 0.9416666666666666519, 0.9430555555555555358, 0.9444444444444444198, 0.9458333333333333037, 0.9472222222222221877, 0.9486111111111110716, 0.9499999999999999556, 0.9513888888888888395, 0.9527777777777777235, 0.9541666666666667185, 0.9555555555555556024, 0.9569444444444444864, 0.9583333333333333703, 0.9597222222222222543, 0.9611111111111111382, 0.9625000000000000222, 0.9638888888888889062, 0.9652777777777777901, 0.9666666666666666741, 0.9680555555555555580, 0.9694444444444444420, 0.9708333333333333259, 0.9722222222222222099, 0.9736111111111110938, 0.9749999999999999778, 0.9763888888888888618, 0.9777777777777777457, 0.9791666666666666297, 0.9805555555555555136, 0.9819444444444443976, 0.9833333333333332815, 0.9847222222222222765, 0.9861111111111111605, 0.9875000000000000444, 0.9888888888888889284, 0.9902777777777778123, 0.9916666666666666963, 0.9930555555555555802, 0.9944444444444444642, 0.9958333333333333481, 0.9972222222222222321, 0.9986111111111111160, 1.000000000000000000 ),
 .UNSPECIFIED. ) 
 CURVE ( )  GEOMETRIC_REPRESENTATION_ITEM ( )  RATIONAL_B_SPLINE_CURVE ( ( 1.000000000000000000, 0.8660254037844387076, 1.000000000000000000, 0.8660254037844387076, 1.000000000000000000, 0.8660254037844387076, 1.000000000000000000, 0.8660254037844387076, 1.000000000000000000, 0.8660254037844387076, 1.000000000000000000, 0.8660254037844387076, 1.000000000000000000, 0.8660254037844387076, 1.000000000000000000, 0.8660254037844387076, 1.000000000000000000, 0.8660254037844387076, 1.000000000000000000, 0.8660254037844387076, 1.000000000000000000, 0.8660254037844387076, 1.000000000000000000, 0.8660254037844387076, 1.000000000000000000, 0.8660254037844387076, 1.000000000000000000, 0.8660254037844387076, 1.000000000000000000, 0.8660254037844387076, 1.000000000000000000, 0.8660254037844387076, 1.000000000000000000, 0.8660254037844387076, 1.000000000000000000, 0.8660254037844387076, 1.000000000000000000, 0.8660254037844387076, 1.000000000000000000, 0.8660254037844387076, 1.000000000000000000, 0.8660254037844387076, 1.000000000000000000, 0.8660254037844387076, 1.000000000000000000, 0.8660254037844387076, 1.000000000000000000, 0.8660254037844387076, 1.000000000000000000, 0.8660254037844387076, 1.000000000000000000, 0.8660254037844387076, 1.000000000000000000, 0.8660254037844387076, 1.000000000000000000, 0.8660254037844387076, 1.000000000000000000, 0.8660254037844387076, 1.000000000000000000, 0.8660254037844387076, 1.000000000000000000, 0.8660254037844387076, 1.000000000000000000, 0.8660254037844387076, 1.000000000000000000, 0.8660254037844387076, 1.000000000000000000, 0.8660254037844387076, 1.000000000000000000, 0.8660254037844387076, 1.000000000000000000, 0.8660254037844387076, 1.000000000000000000, 0.8660254037844387076, 1.000000000000000000, 0.8660254037844387076, 1.000000000000000000, 0.8660254037844387076, 1.000000000000000000, 0.8660254037844387076, 1.000000000000000000, 0.8660254037844387076, 1.000000000000000000, 0.8660254037844387076, 1.000000000000000000, 0.8660254037844387076, 1.000000000000000000, 0.8660254037844387076, 1.000000000000000000, 0.8660254037844387076, 1.000000000000000000, 0.8660254037844387076, 1.000000000000000000, 0.8660254037844387076, 1.000000000000000000, 0.8660254037844387076, 1.000000000000000000, 0.8660254037844387076, 1.000000000000000000, 0.8660254037844387076, 1.000000000000000000, 0.8660254037844387076, 1.000000000000000000, 0.8660254037844387076, 1.000000000000000000, 0.8660254037844387076, 1.000000000000000000, 0.8660254037844387076, 1.000000000000000000, 0.8660254037844387076, 1.000000000000000000, 0.8660254037844387076, 1.000000000000000000, 0.8660254037844387076, 1.000000000000000000, 0.8660254037844387076, 1.000000000000000000, 0.8660254037844387076, 1.000000000000000000, 0.8660254037844387076, 1.000000000000000000, 0.8660254037844387076, 1.000000000000000000, 0.8660254037844387076, 1.000000000000000000, 0.8660254037844387076, 1.000000000000000000, 0.8660254037844387076, 1.000000000000000000, 0.8660254037844387076, 1.000000000000000000, 0.8660254037844387076, 1.000000000000000000, 0.8660254037844387076, 1.000000000000000000, 0.8660254037844387076, 1.000000000000000000, 0.8660254037844387076, 1.000000000000000000, 0.8660254037844387076, 1.000000000000000000, 0.8660254037844387076, 1.000000000000000000, 0.8660254037844387076, 1.000000000000000000, 0.8660254037844387076, 1.000000000000000000, 0.8660254037844387076, 1.000000000000000000, 0.8660254037844387076, 1.000000000000000000, 0.8660254037844387076, 1.000000000000000000, 0.8660254037844387076, 1.000000000000000000, 0.8660254037844387076, 1.000000000000000000, 0.8660254037844387076, 1.000000000000000000, 0.8660254037844387076, 1.000000000000000000, 0.8660254037844387076, 1.000000000000000000, 0.8660254037844387076, 1.000000000000000000, 0.8660254037844387076, 1.000000000000000000, 0.8660254037844387076, 1.000000000000000000, 0.8660254037844387076, 1.000000000000000000, 0.8660254037844387076, 1.000000000000000000, 0.8660254037844387076, 1.000000000000000000, 0.8660254037844387076, 1.000000000000000000, 0.8660254037844387076, 1.000000000000000000, 0.8660254037844387076, 1.000000000000000000, 0.8660254037844387076, 1.000000000000000000, 0.8660254037844387076, 1.000000000000000000, 0.8660254037844387076, 1.000000000000000000, 0.8660254037844387076, 1.000000000000000000, 0.8660254037844387076, 1.000000000000000000, 0.8660254037844387076, 1.000000000000000000, 0.8660254037844387076, 1.000000000000000000, 0.8660254037844387076, 1.000000000000000000, 0.8660254037844387076, 1.000000000000000000, 0.8660254037844387076, 1.000000000000000000, 0.8660254037844387076, 1.000000000000000000, 0.8660254037844387076, 1.000000000000000000, 0.8660254037844387076, 1.000000000000000000, 0.8660254037844387076, 1.000000000000000000, 0.8660254037844387076, 1.000000000000000000, 0.8660254037844387076, 1.000000000000000000, 0.8660254037844387076, 1.000000000000000000, 0.8660254037844387076, 1.000000000000000000, 0.8660254037844387076, 1.000000000000000000, 0.8660254037844387076, 1.000000000000000000, 0.8660254037844387076, 1.000000000000000000, 0.8660254037844387076, 1.000000000000000000, 0.8660254037844387076, 1.000000000000000000, 0.8660254037844387076, 1.000000000000000000, 0.8660254037844387076, 1.000000000000000000, 0.8660254037844387076, 1.000000000000000000, 0.8660254037844387076, 1.000000000000000000, 0.8660254037844387076, 1.000000000000000000, 0.8660254037844387076, 1.000000000000000000, 0.8660254037844387076, 1.000000000000000000, 0.8660254037844387076, 1.000000000000000000, 0.8660254037844387076, 1.000000000000000000, 0.8660254037844387076, 1.000000000000000000, 0.8660254037844387076, 1.000000000000000000, 0.8660254037844387076, 1.000000000000000000, 0.8660254037844387076, 1.000000000000000000, 0.8660254037844387076, 1.000000000000000000, 0.8660254037844387076, 1.000000000000000000, 0.8660254037844387076, 1.000000000000000000, 0.8660254037844387076, 1.000000000000000000, 0.8660254037844387076, 1.000000000000000000, 0.8660254037844387076, 1.000000000000000000, 0.8660254037844387076, 1.000000000000000000, 0.8660254037844387076, 1.000000000000000000, 0.8660254037844387076, 1.000000000000000000, 0.8660254037844387076, 1.000000000000000000, 0.8660254037844387076, 1.000000000000000000, 0.8660254037844387076, 1.000000000000000000, 0.8660254037844387076, 1.000000000000000000, 0.8660254037844387076, 1.000000000000000000, 0.8660254037844387076, 1.000000000000000000, 0.8660254037844387076, 1.000000000000000000, 0.8660254037844387076, 1.000000000000000000, 0.8660254037844387076, 1.000000000000000000, 0.8660254037844387076, 1.000000000000000000, 0.8660254037844387076, 1.000000000000000000, 0.8660254037844387076, 1.000000000000000000, 0.8660254037844387076, 1.000000000000000000, 0.8660254037844387076, 1.000000000000000000, 0.8660254037844387076, 1.000000000000000000, 0.8660254037844387076, 1.000000000000000000, 0.8660254037844387076, 1.000000000000000000, 0.8660254037844387076, 1.000000000000000000, 0.8660254037844387076, 1.000000000000000000, 0.8660254037844387076, 1.000000000000000000, 0.8660254037844387076, 1.000000000000000000, 0.8660254037844387076, 1.000000000000000000, 0.8660254037844387076, 1.000000000000000000, 0.8660254037844387076, 1.000000000000000000, 0.8660254037844387076, 1.000000000000000000, 0.8660254037844387076, 1.000000000000000000, 0.8660254037844387076, 1.000000000000000000, 0.8660254037844387076, 1.000000000000000000, 0.8660254037844387076, 1.000000000000000000, 0.8660254037844387076, 1.000000000000000000, 0.8660254037844387076, 1.000000000000000000, 0.8660254037844387076, 1.000000000000000000, 0.8660254037844387076, 1.000000000000000000, 0.8660254037844387076, 1.000000000000000000, 0.8660254037844387076, 1.000000000000000000, 0.8660254037844387076, 1.000000000000000000, 0.8660254037844387076, 1.000000000000000000, 0.8660254037844387076, 1.000000000000000000, 0.8660254037844387076, 1.000000000000000000, 0.8660254037844387076, 1.000000000000000000, 0.8660254037844387076, 1.000000000000000000, 0.8660254037844387076, 1.000000000000000000, 0.8660254037844387076, 1.000000000000000000, 0.8660254037844387076, 1.000000000000000000, 0.8660254037844387076, 1.000000000000000000, 0.8660254037844387076, 1.000000000000000000, 0.8660254037844387076, 1.000000000000000000, 0.8660254037844387076, 1.000000000000000000, 0.8660254037844387076, 1.000000000000000000, 0.8660254037844387076, 1.000000000000000000, 0.8660254037844387076, 1.000000000000000000, 0.8660254037844387076, 1.000000000000000000, 0.8660254037844387076, 1.000000000000000000, 0.8660254037844387076, 1.000000000000000000, 0.8660254037844387076, 1.000000000000000000, 0.8660254037844387076, 1.000000000000000000, 0.8660254037844387076, 1.000000000000000000, 0.8660254037844387076, 1.000000000000000000, 0.8660254037844387076, 1.000000000000000000, 0.8660254037844387076, 1.000000000000000000, 0.8660254037844387076, 1.000000000000000000, 0.8660254037844387076, 1.000000000000000000, 0.8660254037844387076, 1.000000000000000000, 0.8660254037844387076, 1.000000000000000000, 0.8660254037844387076, 1.000000000000000000, 0.8660254037844387076, 1.000000000000000000, 0.8660254037844387076, 1.000000000000000000, 0.8660254037844387076, 1.000000000000000000, 0.8660254037844387076, 1.000000000000000000, 0.8660254037844387076, 1.000000000000000000, 0.8660254037844387076, 1.000000000000000000, 0.8660254037844387076, 1.000000000000000000, 0.8660254037844387076, 1.000000000000000000, 0.8660254037844387076, 1.000000000000000000, 0.8660254037844387076, 1.000000000000000000, 0.8660254037844387076, 1.000000000000000000, 0.8660254037844387076, 1.000000000000000000, 0.8660254037844387076, 1.000000000000000000, 0.8660254037844387076, 1.000000000000000000, 0.8660254037844387076, 1.000000000000000000, 0.8660254037844387076, 1.000000000000000000, 0.8660254037844387076, 1.000000000000000000, 0.8660254037844387076, 1.000000000000000000, 0.8660254037844387076, 1.000000000000000000, 0.8660254037844387076, 1.000000000000000000, 0.8660254037844387076, 1.000000000000000000, 0.8660254037844387076, 1.000000000000000000, 0.8660254037844387076, 1.000000000000000000, 0.8660254037844387076, 1.000000000000000000, 0.8660254037844387076, 1.000000000000000000, 0.8660254037844387076, 1.000000000000000000, 0.8660254037844387076, 1.000000000000000000, 0.8660254037844387076, 1.000000000000000000, 0.8660254037844387076, 1.000000000000000000, 0.8660254037844387076, 1.000000000000000000, 0.8660254037844387076, 1.000000000000000000, 0.8660254037844387076, 1.000000000000000000, 0.8660254037844387076, 1.000000000000000000, 0.8660254037844387076, 1.000000000000000000, 0.8660254037844387076, 1.000000000000000000, 0.8660254037844387076, 1.000000000000000000, 0.8660254037844387076, 1.000000000000000000, 0.8660254037844387076, 1.000000000000000000, 0.8660254037844387076, 1.000000000000000000, 0.8660254037844387076, 1.000000000000000000, 0.8660254037844387076, 1.000000000000000000, 0.8660254037844387076, 1.000000000000000000, 0.8660254037844387076, 1.000000000000000000, 0.8660254037844387076, 1.000000000000000000, 0.8660254037844387076, 1.000000000000000000, 0.8660254037844387076, 1.000000000000000000, 0.8660254037844387076, 1.000000000000000000, 0.8660254037844387076, 1.000000000000000000, 0.8660254037844387076, 1.000000000000000000, 0.8660254037844387076, 1.000000000000000000, 0.8660254037844387076, 1.000000000000000000, 0.8660254037844387076, 1.000000000000000000, 0.8660254037844387076, 1.000000000000000000, 0.8660254037844387076, 1.000000000000000000, 0.8660254037844387076, 1.000000000000000000, 0.8660254037844387076, 1.000000000000000000, 0.8660254037844387076, 1.000000000000000000, 0.8660254037844387076, 1.000000000000000000, 0.8660254037844387076, 1.000000000000000000, 0.8660254037844387076, 1.000000000000000000, 0.8660254037844387076, 1.000000000000000000, 0.8660254037844387076, 1.000000000000000000, 0.8660254037844387076, 1.000000000000000000, 0.8660254037844387076, 1.000000000000000000, 0.8660254037844387076, 1.000000000000000000, 0.8660254037844387076, 1.000000000000000000, 0.8660254037844387076, 1.000000000000000000, 0.8660254037844387076, 1.000000000000000000, 0.8660254037844387076, 1.000000000000000000, 0.8660254037844387076, 1.000000000000000000, 0.8660254037844387076, 1.000000000000000000, 0.8660254037844387076, 1.000000000000000000, 0.8660254037844387076, 1.000000000000000000, 0.8660254037844387076, 1.000000000000000000, 0.8660254037844387076, 1.000000000000000000, 0.8660254037844387076, 1.000000000000000000, 0.8660254037844387076, 1.000000000000000000, 0.8660254037844387076, 1.000000000000000000, 0.8660254037844387076, 1.000000000000000000, 0.8660254037844387076, 1.000000000000000000, 0.8660254037844387076, 1.000000000000000000, 0.8660254037844387076, 1.000000000000000000, 0.8660254037844387076, 1.000000000000000000, 0.8660254037844387076, 1.000000000000000000, 0.8660254037844387076, 1.000000000000000000, 0.8660254037844387076, 1.000000000000000000, 0.8660254037844387076, 1.000000000000000000, 0.8660254037844387076, 1.000000000000000000, 0.8660254037844387076, 1.000000000000000000, 0.8660254037844387076, 1.000000000000000000, 0.8660254037844387076, 1.000000000000000000, 0.8660254037844387076, 1.000000000000000000, 0.8660254037844387076, 1.000000000000000000, 0.8660254037844387076, 1.000000000000000000, 0.8660254037844387076, 1.000000000000000000, 0.8660254037844387076, 1.000000000000000000, 0.8660254037844387076, 1.000000000000000000, 0.8660254037844387076, 1.000000000000000000, 0.8660254037844387076, 1.000000000000000000, 0.8660254037844387076, 1.000000000000000000, 0.8660254037844387076, 1.000000000000000000, 0.8660254037844387076, 1.000000000000000000, 0.8660254037844387076, 1.000000000000000000, 0.8660254037844387076, 1.000000000000000000, 0.8660254037844387076, 1.000000000000000000, 0.8660254037844387076, 1.000000000000000000, 0.8660254037844387076, 1.000000000000000000, 0.8660254037844387076, 1.000000000000000000, 0.8660254037844387076, 1.000000000000000000, 0.8660254037844387076, 1.000000000000000000, 0.8660254037844387076, 1.000000000000000000, 0.8660254037844387076, 1.000000000000000000, 0.8660254037844387076, 1.000000000000000000, 0.8660254037844387076, 1.000000000000000000, 0.8660254037844387076, 1.000000000000000000, 0.8660254037844387076, 1.000000000000000000, 0.8660254037844387076, 1.000000000000000000, 0.8660254037844387076, 1.000000000000000000, 0.8660254037844387076, 1.000000000000000000, 0.8660254037844387076, 1.000000000000000000, 0.8660254037844387076, 1.000000000000000000, 0.8660254037844387076, 1.000000000000000000, 0.8660254037844387076, 1.000000000000000000, 0.8660254037844387076, 1.000000000000000000, 0.8660254037844387076, 1.000000000000000000, 0.8660254037844387076, 1.000000000000000000, 0.8660254037844387076, 1.000000000000000000, 0.8660254037844387076, 1.000000000000000000, 0.8660254037844387076, 1.000000000000000000, 0.8660254037844387076, 1.000000000000000000, 0.8660254037844387076, 1.000000000000000000, 0.8660254037844387076, 1.000000000000000000, 0.8660254037844387076, 1.000000000000000000, 0.8660254037844387076, 1.000000000000000000, 0.8660254037844387076, 1.000000000000000000, 0.8660254037844387076, 1.000000000000000000, 0.8660254037844387076, 1.000000000000000000, 0.8660254037844387076, 1.000000000000000000, 0.8660254037844387076, 1.000000000000000000, 0.8660254037844387076, 1.000000000000000000, 0.8660254037844387076, 1.000000000000000000, 0.8660254037844387076, 1.000000000000000000, 0.8660254037844387076, 1.000000000000000000, 0.8660254037844387076, 1.000000000000000000, 0.8660254037844387076, 1.000000000000000000, 0.8660254037844387076, 1.000000000000000000, 0.8660254037844387076, 1.000000000000000000, 0.8660254037844387076, 1.000000000000000000, 0.8660254037844387076, 1.000000000000000000, 0.8660254037844387076, 1.000000000000000000, 0.8660254037844387076, 1.000000000000000000, 0.8660254037844387076, 1.000000000000000000, 0.8660254037844387076, 1.000000000000000000, 0.8660254037844387076, 1.000000000000000000, 0.8660254037844387076, 1.000000000000000000, 0.8660254037844387076, 1.000000000000000000, 0.8660254037844387076, 1.000000000000000000, 0.8660254037844387076, 1.000000000000000000, 0.8660254037844387076, 1.000000000000000000, 0.8660254037844387076, 1.000000000000000000, 0.8660254037844387076, 1.000000000000000000, 0.8660254037844387076, 1.000000000000000000, 0.8660254037844387076, 1.000000000000000000, 0.8660254037844387076, 1.000000000000000000, 0.8660254037844387076, 1.000000000000000000, 0.8660254037844387076, 1.000000000000000000, 0.8660254037844387076, 1.000000000000000000, 0.8660254037844387076, 1.000000000000000000, 0.8660254037844387076, 1.000000000000000000, 0.8660254037844387076, 1.000000000000000000, 0.8660254037844387076, 1.000000000000000000, 0.8660254037844387076, 1.000000000000000000, 0.8660254037844387076, 1.000000000000000000, 0.8660254037844387076, 1.000000000000000000, 0.8660254037844387076, 1.000000000000000000, 0.8660254037844387076, 1.000000000000000000, 0.8660254037844387076, 1.000000000000000000, 0.8660254037844387076, 1.000000000000000000, 0.8660254037844387076, 1.000000000000000000, 0.8660254037844387076, 1.000000000000000000, 0.8660254037844387076, 1.000000000000000000, 0.8660254037844387076, 1.000000000000000000, 0.8660254037844387076, 1.000000000000000000, 0.8660254037844387076, 1.000000000000000000, 0.8660254037844387076, 1.000000000000000000, 0.8660254037844387076, 1.000000000000000000, 0.8660254037844387076, 1.000000000000000000, 0.8660254037844387076, 1.000000000000000000, 0.8660254037844387076, 1.000000000000000000, 0.8660254037844387076, 1.000000000000000000, 0.8660254037844387076, 1.000000000000000000, 0.8660254037844387076, 1.000000000000000000, 0.8660254037844387076, 1.000000000000000000, 0.8660254037844387076, 1.000000000000000000, 0.8660254037844387076, 1.000000000000000000, 0.8660254037844387076, 1.000000000000000000, 0.8660254037844387076, 1.000000000000000000, 0.8660254037844387076, 1.000000000000000000, 0.8660254037844387076, 1.000000000000000000, 0.8660254037844387076, 1.000000000000000000, 0.8660254037844387076, 1.000000000000000000, 0.8660254037844387076, 1.000000000000000000, 0.8660254037844387076, 1.000000000000000000, 0.8660254037844387076, 1.000000000000000000, 0.8660254037844387076, 1.000000000000000000, 0.8660254037844387076, 1.000000000000000000, 0.8660254037844387076, 1.000000000000000000, 0.8660254037844387076, 1.000000000000000000, 0.8660254037844387076, 1.000000000000000000, 0.8660254037844387076, 1.000000000000000000, 0.8660254037844387076, 1.000000000000000000, 0.8660254037844387076, 1.000000000000000000, 0.8660254037844387076, 1.000000000000000000, 0.8660254037844387076, 1.000000000000000000, 0.8660254037844387076, 1.000000000000000000, 0.8660254037844387076, 1.000000000000000000, 0.8660254037844387076, 1.000000000000000000, 0.8660254037844387076, 1.000000000000000000, 0.8660254037844387076, 1.000000000000000000, 0.8660254037844387076, 1.000000000000000000, 0.8660254037844387076, 1.000000000000000000, 0.8660254037844387076, 1.000000000000000000, 0.8660254037844387076, 1.000000000000000000, 0.8660254037844387076, 1.000000000000000000, 0.8660254037844387076, 1.000000000000000000, 0.8660254037844387076, 1.000000000000000000, 0.8660254037844387076, 1.000000000000000000, 0.8660254037844387076, 1.000000000000000000, 0.8660254037844387076, 1.000000000000000000, 0.8660254037844387076, 1.000000000000000000, 0.8660254037844387076, 1.000000000000000000, 0.8660254037844387076, 1.000000000000000000, 0.8660254037844387076, 1.000000000000000000, 0.8660254037844387076, 1.000000000000000000, 0.8660254037844387076, 1.000000000000000000, 0.8660254037844387076, 1.000000000000000000, 0.8660254037844387076, 1.000000000000000000, 0.8660254037844387076, 1.000000000000000000, 0.8660254037844387076, 1.000000000000000000, 0.8660254037844387076, 1.000000000000000000, 0.8660254037844387076, 1.000000000000000000, 0.8660254037844387076, 1.000000000000000000, 0.8660254037844387076, 1.000000000000000000, 0.8660254037844387076, 1.000000000000000000, 0.8660254037844387076, 1.000000000000000000, 0.8660254037844387076, 1.000000000000000000, 0.8660254037844387076, 1.000000000000000000, 0.8660254037844387076, 1.000000000000000000, 0.8660254037844387076, 1.000000000000000000, 0.8660254037844387076, 1.000000000000000000, 0.8660254037844387076, 1.000000000000000000, 0.8660254037844387076, 1.000000000000000000, 0.8660254037844387076, 1.000000000000000000, 0.8660254037844387076, 1.000000000000000000, 0.8660254037844387076, 1.000000000000000000, 0.8660254037844387076, 1.000000000000000000, 0.8660254037844387076, 1.000000000000000000, 0.8660254037844387076, 1.000000000000000000, 0.8660254037844387076, 1.000000000000000000, 0.8660254037844387076, 1.000000000000000000, 0.8660254037844387076, 1.000000000000000000, 0.8660254037844387076, 1.000000000000000000, 0.8660254037844387076, 1.000000000000000000, 0.8660254037844387076, 1.000000000000000000, 0.8660254037844387076, 1.000000000000000000, 0.8660254037844387076, 1.000000000000000000, 0.8660254037844387076, 1.000000000000000000, 0.8660254037844387076, 1.000000000000000000, 0.8660254037844387076, 1.000000000000000000, 0.8660254037844387076, 1.000000000000000000, 0.8660254037844387076, 1.000000000000000000, 0.8660254037844387076, 1.000000000000000000, 0.8660254037844387076, 1.000000000000000000, 0.8660254037844387076, 1.000000000000000000, 0.8660254037844387076, 1.000000000000000000, 0.8660254037844387076, 1.000000000000000000, 0.8660254037844387076, 1.000000000000000000, 0.8660254037844387076, 1.000000000000000000, 0.8660254037844387076, 1.000000000000000000, 0.8660254037844387076, 1.000000000000000000, 0.8660254037844387076, 1.000000000000000000, 0.8660254037844387076, 1.000000000000000000, 0.8660254037844387076, 1.000000000000000000, 0.8660254037844387076, 1.000000000000000000, 0.8660254037844387076, 1.000000000000000000, 0.8660254037844387076, 1.000000000000000000, 0.8660254037844387076, 1.000000000000000000, 0.8660254037844387076, 1.000000000000000000, 0.8660254037844387076, 1.000000000000000000, 0.8660254037844387076, 1.000000000000000000, 0.8660254037844387076, 1.000000000000000000, 0.8660254037844387076, 1.000000000000000000, 0.8660254037844387076, 1.000000000000000000, 0.8660254037844387076, 1.000000000000000000, 0.8660254037844387076, 1.000000000000000000, 0.8660254037844387076, 1.000000000000000000, 0.8660254037844387076, 1.000000000000000000, 0.8660254037844387076, 1.000000000000000000, 0.8660254037844387076, 1.000000000000000000, 0.8660254037844387076, 1.000000000000000000, 0.8660254037844387076, 1.000000000000000000, 0.8660254037844387076, 1.000000000000000000, 0.8660254037844387076, 1.000000000000000000, 0.8660254037844387076, 1.000000000000000000, 0.8660254037844387076, 1.000000000000000000, 0.8660254037844387076, 1.000000000000000000, 0.8660254037844387076, 1.000000000000000000, 0.8660254037844387076, 1.000000000000000000, 0.8660254037844387076, 1.000000000000000000, 0.8660254037844387076, 1.000000000000000000, 0.8660254037844387076, 1.000000000000000000, 0.8660254037844387076, 1.000000000000000000, 0.8660254037844387076, 1.000000000000000000, 0.8660254037844387076, 1.000000000000000000, 0.8660254037844387076, 1.000000000000000000, 0.8660254037844387076, 1.000000000000000000, 0.8660254037844387076, 1.000000000000000000, 0.8660254037844387076, 1.000000000000000000, 0.8660254037844387076, 1.000000000000000000, 0.8660254037844387076, 1.000000000000000000, 0.8660254037844387076, 1.000000000000000000, 0.8660254037844387076, 1.000000000000000000, 0.8660254037844387076, 1.000000000000000000, 0.8660254037844387076, 1.000000000000000000, 0.8660254037844387076, 1.000000000000000000, 0.8660254037844387076, 1.000000000000000000, 0.8660254037844387076, 1.000000000000000000, 0.8660254037844387076, 1.000000000000000000, 0.8660254037844387076, 1.000000000000000000, 0.8660254037844387076, 1.000000000000000000, 0.8660254037844387076, 1.000000000000000000, 0.8660254037844387076, 1.000000000000000000, 0.8660254037844387076, 1.000000000000000000, 0.8660254037844387076, 1.000000000000000000, 0.8660254037844387076, 1.000000000000000000, 0.8660254037844387076, 1.000000000000000000, 0.8660254037844387076, 1.000000000000000000, 0.8660254037844387076, 1.000000000000000000, 0.8660254037844387076, 1.000000000000000000, 0.8660254037844387076, 1.000000000000000000, 0.8660254037844387076, 1.000000000000000000, 0.8660254037844387076, 1.000000000000000000, 0.8660254037844387076, 1.000000000000000000, 0.8660254037844387076, 1.000000000000000000, 0.8660254037844387076, 1.000000000000000000, 0.8660254037844387076, 1.000000000000000000, 0.8660254037844387076, 1.000000000000000000, 0.8660254037844387076, 1.000000000000000000, 0.8660254037844387076, 1.000000000000000000, 0.8660254037844387076, 1.000000000000000000, 0.8660254037844387076, 1.000000000000000000, 0.8660254037844387076, 1.000000000000000000, 0.8660254037844387076, 1.000000000000000000, 0.8660254037844387076, 1.000000000000000000, 0.8660254037844387076, 1.000000000000000000, 0.8660254037844387076, 1.000000000000000000, 0.8660254037844387076, 1.000000000000000000, 0.8660254037844387076, 1.000000000000000000, 0.8660254037844387076, 1.000000000000000000, 0.8660254037844387076, 1.000000000000000000, 0.8660254037844387076, 1.000000000000000000, 0.8660254037844387076, 1.000000000000000000, 0.8660254037844387076, 1.000000000000000000, 0.8660254037844387076, 1.000000000000000000, 0.8660254037844387076, 1.000000000000000000, 0.8660254037844387076, 1.000000000000000000, 0.8660254037844387076, 1.000000000000000000, 0.8660254037844387076, 1.000000000000000000, 0.8660254037844387076, 1.000000000000000000, 0.8660254037844387076, 1.000000000000000000, 0.8660254037844387076, 1.000000000000000000, 0.8660254037844387076, 1.000000000000000000, 0.8660254037844387076, 1.000000000000000000, 0.8660254037844387076, 1.000000000000000000, 0.8660254037844387076, 1.000000000000000000, 0.8660254037844387076, 1.000000000000000000, 0.8660254037844387076, 1.000000000000000000, 0.8660254037844387076, 1.000000000000000000, 0.8660254037844387076, 1.000000000000000000, 0.8660254037844387076, 1.000000000000000000, 0.8660254037844387076, 1.000000000000000000, 0.8660254037844387076, 1.000000000000000000, 0.8660254037844387076, 1.000000000000000000, 0.8660254037844387076, 1.000000000000000000, 0.8660254037844387076, 1.000000000000000000, 0.8660254037844387076, 1.000000000000000000, 0.8660254037844387076, 1.000000000000000000, 0.8660254037844387076, 1.000000000000000000, 0.8660254037844387076, 1.000000000000000000, 0.8660254037844387076, 1.000000000000000000, 0.8660254037844387076, 1.000000000000000000, 0.8660254037844387076, 1.000000000000000000, 0.8660254037844387076, 1.000000000000000000, 0.8660254037844387076, 1.000000000000000000, 0.8660254037844387076, 1.000000000000000000, 0.8660254037844387076, 1.000000000000000000, 0.8660254037844387076, 1.000000000000000000, 0.8660254037844387076, 1.000000000000000000, 0.8660254037844387076, 1.000000000000000000, 0.8660254037844387076, 1.000000000000000000, 0.8660254037844387076, 1.000000000000000000, 0.8660254037844387076, 1.000000000000000000, 0.8660254037844387076, 1.000000000000000000, 0.8660254037844387076, 1.000000000000000000, 0.8660254037844387076, 1.000000000000000000, 0.8660254037844387076, 1.000000000000000000, 0.8660254037844387076, 1.000000000000000000, 0.8660254037844387076, 1.000000000000000000, 0.8660254037844387076, 1.000000000000000000, 0.8660254037844387076, 1.000000000000000000, 0.8660254037844387076, 1.000000000000000000, 0.8660254037844387076, 1.000000000000000000, 0.8660254037844387076, 1.000000000000000000, 0.8660254037844387076, 1.000000000000000000, 0.8660254037844387076, 1.000000000000000000, 0.8660254037844387076, 1.000000000000000000, 0.8660254037844387076, 1.000000000000000000, 0.8660254037844387076, 1.000000000000000000, 0.8660254037844387076, 1.000000000000000000, 0.8660254037844387076, 1.000000000000000000, 0.8660254037844387076, 1.000000000000000000, 0.8660254037844387076, 1.000000000000000000, 0.8660254037844387076, 1.000000000000000000, 0.8660254037844387076, 1.000000000000000000, 0.8660254037844387076, 1.000000000000000000, 0.8660254037844387076, 1.000000000000000000, 0.8660254037844387076, 1.000000000000000000, 0.8660254037844387076, 1.000000000000000000, 0.8660254037844387076, 1.000000000000000000, 0.8660254037844387076, 1.000000000000000000, 0.8660254037844387076, 1.000000000000000000, 0.8660254037844387076, 1.000000000000000000, 0.8660254037844387076, 1.000000000000000000, 0.8660254037844387076, 1.000000000000000000, 0.8660254037844387076, 1.000000000000000000, 0.8660254037844387076, 1.000000000000000000, 0.8660254037844387076, 1.000000000000000000, 0.8660254037844387076, 1.000000000000000000, 0.8660254037844387076, 1.000000000000000000, 0.8660254037844387076, 1.000000000000000000, 0.8660254037844387076, 1.000000000000000000, 0.8660254037844387076, 1.000000000000000000, 0.8660254037844387076, 1.000000000000000000, 0.8660254037844387076, 1.000000000000000000, 0.8660254037844387076, 1.000000000000000000, 0.8660254037844387076, 1.000000000000000000, 0.8660254037844387076, 1.000000000000000000, 0.8660254037844387076, 1.000000000000000000, 0.8660254037844387076, 1.000000000000000000, 0.8660254037844387076, 1.000000000000000000, 0.8660254037844387076, 1.000000000000000000, 0.8660254037844387076, 1.000000000000000000, 0.8660254037844387076, 1.000000000000000000, 0.8660254037844387076, 1.000000000000000000, 0.8660254037844387076, 1.000000000000000000, 0.8660254037844387076, 1.000000000000000000, 0.8660254037844387076, 1.000000000000000000, 0.8660254037844387076, 1.000000000000000000, 0.8660254037844387076, 1.000000000000000000, 0.8660254037844387076, 1.000000000000000000, 0.8660254037844387076, 1.000000000000000000, 0.8660254037844387076, 1.000000000000000000, 0.8660254037844387076, 1.000000000000000000, 0.8660254037844387076, 1.000000000000000000, 0.8660254037844387076, 1.000000000000000000, 0.8660254037844387076, 1.000000000000000000, 0.8660254037844387076, 1.000000000000000000, 0.8660254037844387076, 1.000000000000000000, 0.8660254037844387076, 1.000000000000000000, 0.8660254037844387076, 1.000000000000000000, 0.8660254037844387076, 1.000000000000000000, 0.8660254037844387076, 1.000000000000000000, 0.8660254037844387076, 1.000000000000000000, 0.8660254037844387076, 1.000000000000000000, 0.8660254037844387076, 1.000000000000000000, 0.8660254037844387076, 1.000000000000000000, 0.8660254037844387076, 1.000000000000000000, 0.8660254037844387076, 1.000000000000000000, 0.8660254037844387076, 1.000000000000000000, 0.8660254037844387076, 1.000000000000000000, 0.8660254037844387076, 1.000000000000000000, 0.8660254037844387076, 1.000000000000000000, 0.8660254037844387076, 1.000000000000000000, 0.8660254037844387076, 1.000000000000000000, 0.8660254037844387076, 1.000000000000000000, 0.8660254037844387076, 1.000000000000000000, 0.8660254037844387076, 1.000000000000000000, 0.8660254037844387076, 1.000000000000000000, 0.8660254037844387076, 1.000000000000000000, 0.8660254037844387076, 1.000000000000000000, 0.8660254037844387076, 1.000000000000000000, 0.8660254037844387076, 1.000000000000000000, 0.8660254037844387076, 1.000000000000000000, 0.8660254037844387076, 1.000000000000000000, 0.8660254037844387076, 1.000000000000000000, 0.8660254037844387076, 1.000000000000000000, 0.8660254037844387076, 1.000000000000000000, 0.8660254037844387076, 1.000000000000000000, 0.8660254037844387076, 1.000000000000000000, 0.8660254037844387076, 1.000000000000000000, 0.8660254037844387076, 1.000000000000000000, 0.8660254037844387076, 1.000000000000000000, 0.8660254037844387076, 1.000000000000000000, 0.8660254037844387076, 1.000000000000000000, 0.8660254037844387076, 1.000000000000000000, 0.8660254037844387076, 1.000000000000000000, 0.8660254037844387076, 1.000000000000000000, 0.8660254037844387076, 1.000000000000000000, 0.8660254037844387076, 1.000000000000000000, 0.8660254037844387076, 1.000000000000000000, 0.8660254037844387076, 1.000000000000000000, 0.8660254037844387076, 1.000000000000000000, 0.8660254037844387076, 1.000000000000000000, 0.8660254037844387076, 1.000000000000000000, 0.8660254037844387076, 1.000000000000000000, 0.8660254037844387076, 1.000000000000000000, 0.8660254037844387076, 1.000000000000000000, 0.8660254037844387076, 1.000000000000000000, 0.8660254037844387076, 1.000000000000000000, 0.8660254037844387076, 1.000000000000000000 ) ) 
 REPRESENTATION_ITEM ( '' )  );
#20435=CARTESIAN_POINT ( 'NONE',  ( -2.500000000000000444, -27.16666666666666430, -4.330127018922193649 ) ) ;
#20439=CARTESIAN_POINT ( 'NONE',  ( 4.458734124999999437, -89.06249999863439371, -5.460374474430324690E-16 ) ) ;
#20440=CARTESIAN_POINT ( 'NONE',  ( 6.123233995736766282E-16, -170.0000000000000000, -5.000000000000000000 ) ) ;
#20445=CARTESIAN_POINT ( 'NONE',  ( -3.535533905932738641, -161.5000000027312126, 3.535533905932737309 ) ) ;
#20448=DIRECTION ( 'NONE',  ( -0.000000000000000000, 1.000000000000000000, -0.000000000000000000 ) ) ;
#20451=( BOUNDED_CURVE ( )  B_SPLINE_CURVE ( 2, ( #55885, #7944, #17269, #12122, #46223, #6997, #61978, #2186, #60714 ),
 .UNSPECIFIED., .F., .F. ) 
 B_SPLINE_CURVE_WITH_KNOTS ( ( 3, 2, 2, 2, 3 ),
 ( 0.2770833333333333481, 0.2777777777777777901, 0.2791666666666666741, 0.2805555555555555580, 0.2812500000000000000 ),
 .UNSPECIFIED. ) 
 CURVE ( )  GEOMETRIC_REPRESENTATION_ITEM ( )  RATIONAL_B_SPLINE_CURVE ( ( 0.9330127018922194093, 0.9330127018922194093, 1.000000000000000000, 0.8660254037844387076, 1.000000000000000000, 0.8660254037844387076, 1.000000000000000000, 0.9330127018922194093, 0.9330127018922194093 ) ) 
 REPRESENTATION_ITEM ( '' )  );
#20457=CARTESIAN_POINT ( 'NONE',  ( -2.229367062499996610, -22.14583333196773651, 3.861377020970582219 ) ) ;
#20459=CARTESIAN_POINT ( 'NONE',  ( -5.000000000000000888, -155.4375000000000000, 2.071067811865474617 ) ) ;
#20461=CARTESIAN_POINT ( 'NONE',  ( -8.190561711645485556E-16, -154.6875000013655779, 4.458734124999999437 ) ) ;
#20462=ORIENTED_EDGE ( 'NONE', *, *, #35544, .F. ) ;
#20463=CARTESIAN_POINT ( 'NONE',  ( -2.229367062499996610, -45.39583333196774362, 3.861377020970582219 ) ) ;
#20464=CARTESIAN_POINT ( 'NONE',  ( 1.339745962155612702, -2.294658198738521282, -5.000000000000000000 ) ) ;
#20466=CARTESIAN_POINT ( 'NONE',  ( -2.500000000000000444, 29.83333333333333215, -4.330127018922193649 ) ) ;
#20467=CARTESIAN_POINT ( 'NONE',  ( 4.458734125000001214, 12.10416666803226171, 2.574251347313718519 ) ) ;
#20469=CARTESIAN_POINT ( 'NONE',  ( 2.499999999999998668, -37.20833333060213732, -4.330127018922193649 ) ) ;
#20470=CARTESIAN_POINT ( 'NONE',  ( 1.975475456537005874E-15, -73.75000000000000000, 5.000000000000000000 ) ) ;
#20471=CARTESIAN_POINT ( 'NONE',  ( -4.458734124999999437, 19.43750000136559208, 0.000000000000000000 ) ) ;
#20473=CARTESIAN_POINT ( 'NONE',  ( -4.999999999999999112, 6.208333336064520758, 2.886751345948131764 ) ) ;
#20474=ORIENTED_EDGE ( 'NONE', *, *, #2745, .T. ) ;
#20475=CARTESIAN_POINT ( 'NONE',  ( -2.499999999999996447, 8.166666666666666075, 4.330127018922195425 ) ) ;
#20479=CARTESIAN_POINT ( 'NONE',  ( 4.458734124999998549, -40.72916666530107221, -2.574251347313721627 ) ) ;
#20482=CARTESIAN_POINT ( 'NONE',  ( 5.000000000000000888, -38.45833333060213732, 2.886751345948126879 ) ) ;
#20485=CARTESIAN_POINT ( 'NONE',  ( 4.458734124999998549, -12.72916666530107044, -2.574251347313721627 ) ) ;
#20486=CARTESIAN_POINT ( 'NONE',  ( -2.229367062499996610, -18.39583333196774007, 3.861377020970582219 ) ) ;
#20487=VERTEX_POINT ( 'NONE', #52127 ) ;
#20488=EDGE_CURVE ( 'NONE', #2611, #38204, #8069, .T. ) ;
#20489=CARTESIAN_POINT ( 'NONE',  ( 2.500000000000002220, -80.66666666666665719, 4.330127018922192761 ) ) ;
#20490=CARTESIAN_POINT ( 'NONE',  ( 1.846868145590736310, -166.6250000013656063, 4.458734124999999437 ) ) ;
#20492=CARTESIAN_POINT ( 'NONE',  ( -2.500000000000000444, -88.04166666393548724, -4.330127018922193649 ) ) ;
#20493=CARTESIAN_POINT ( 'NONE',  ( -4.999999999999998224, -17.91666666666666430, 2.886751345948131764 ) ) ;
#20496=CARTESIAN_POINT ( 'NONE',  ( -3.152548672688508926E-16, -24.81249999863440436, -5.148502694627439702 ) ) ;
#20497=EDGE_CURVE ( 'NONE', #16762, #17838, #28526, .T. ) ;
#20500=CARTESIAN_POINT ( 'NONE',  ( -1.846868145590734756, -163.3750000013656347, -4.458734125000000326 ) ) ;
#20501=ADVANCED_FACE ( 'NONE', ( #38274 ), #59336, .T. ) ;
#20503=CARTESIAN_POINT ( 'NONE',  ( 5.000000000000000000, -156.0000000000000000, 0.000000000000000000 ) ) ;
#20506=CARTESIAN_POINT ( 'NONE',  ( 4.458734125000001214, -73.14583333196773651, 2.574251347313718519 ) ) ;
#20509=CARTESIAN_POINT ( 'NONE',  ( 3.152801135295366208, -140.8125000013655779, 3.152801135295367985 ) ) ;
#20510=( BOUNDED_CURVE ( )  B_SPLINE_CURVE ( 2, ( #49706, #14648, #35239, #49389, #5008, #4684, #24628, #44882, #45200 ),
 .UNSPECIFIED., .F., .F. ) 
 B_SPLINE_CURVE_WITH_KNOTS ( ( 3, 2, 2, 2, 3 ),
 ( 0.1916666666666668462, 0.1958333333333334980, 0.2000000000000001776, 0.2041666666666668295, 0.2083333333333335091 ),
 .UNSPECIFIED. ) 
 CURVE ( )  GEOMETRIC_REPRESENTATION_ITEM ( )  RATIONAL_B_SPLINE_CURVE ( ( 0.9999999999999970024, 0.9238795325112897361, 1.000000000000000000, 0.9238795325112867385, 1.000000000000000000, 0.9238795325112867385, 1.000000000000000000, 0.9238795325112837409, 1.000000000000003109 ) ) 
 REPRESENTATION_ITEM ( '' )  );
#20511=ADVANCED_FACE ( 'NONE', ( #25834 ), #45450, .T. ) ;
#20517=CARTESIAN_POINT ( 'NONE',  ( 3.061616997868383141E-16, -152.8750000027311842, -5.000000000000000000 ) ) ;
#20522=CARTESIAN_POINT ( 'NONE',  ( -4.458734124999999437, -76.56249999863440792, 0.000000000000000000 ) ) ;
#20529=CARTESIAN_POINT ( 'NONE',  ( -9.184850993605147944E-16, -146.2500000000000284, 5.000000000000000000 ) ) ;
#20530=CARTESIAN_POINT ( 'NONE',  ( -2.500000000000000444, -60.16666666666665719, -4.330127018922193649 ) ) ;
#20536=CARTESIAN_POINT ( 'NONE',  ( -3.152548672688508926E-16, 16.18750000136559564, -5.148502694627439702 ) ) ;
#20537=CYLINDRICAL_SURFACE ( 'NONE', #44851, 5.000000000000000000 ) ;
#20542=CARTESIAN_POINT ( 'NONE',  ( -6.972266317189433020E-16, -14.24999999999999822, -5.000000000000000000 ) ) ;
#20543=CARTESIAN_POINT ( 'NONE',  ( -3.152548672688508926E-16, -85.56249999863439371, -5.148502694627439702 ) ) ;
#20544=CARTESIAN_POINT ( 'NONE',  ( -4.458734124999999437, -3.395833331967739177, -2.574251347313719407 ) ) ;
#20545=VERTEX_POINT ( 'NONE', #34851 ) ;
#20546=CARTESIAN_POINT ( 'NONE',  ( 4.458734124999999437, -31.06249999863440436, -5.460374474430324690E-16 ) ) ;
#20550=CARTESIAN_POINT ( 'NONE',  ( 2.229367062499998831, 23.35416666803225993, -3.861377020970580887 ) ) ;
#20551=CARTESIAN_POINT ( 'NONE',  ( -4.764381983412779477E-15, 26.37500000273118417, 5.000000000000000000 ) ) ;
#20552=CARTESIAN_POINT ( 'NONE',  ( -4.458734124999997661, -76.47916666530105090, 2.574251347313722516 ) ) ;
#20555=CARTESIAN_POINT ( 'NONE',  ( -2.499999999999996447, 26.29166666939785202, 4.330127018922195425 ) ) ;
#20556=ORIENTED_EDGE ( 'NONE', *, *, #54985, .F. ) ;
#20559=( BOUNDED_CURVE ( )  B_SPLINE_CURVE ( 2, ( #13408, #33028, #16973, #13714, #58092, #33963, #8578, #48124, #8892 ),
 .UNSPECIFIED., .F., .F. ) 
 B_SPLINE_CURVE_WITH_KNOTS ( ( 3, 2, 2, 2, 3 ),
 ( 0.4979166666666666741, 0.4986111111111111160, 0.5000000000000000000, 0.5013888888888888840, 0.5020833333333333259 ),
 .UNSPECIFIED. ) 
 CURVE ( )  GEOMETRIC_REPRESENTATION_ITEM ( )  RATIONAL_B_SPLINE_CURVE ( ( 0.9330127018922194093, 0.9330127018922194093, 1.000000000000000000, 0.8660254037844387076, 1.000000000000000000, 0.8660254037844387076, 1.000000000000000000, 0.9330127018922194093, 0.9330127018922194093 ) ) 
 REPRESENTATION_ITEM ( '' )  );
#20560=DIRECTION ( 'NONE',  ( 0.000000000000000000, 0.000000000000000000, 1.000000000000000000 ) ) ;
#20561=CARTESIAN_POINT ( 'NONE',  ( 1.060575238724906964E-15, -18.75000000000000000, 5.773502691896257311 ) ) ;
#20562=CARTESIAN_POINT ( 'NONE',  ( 4.458734124999998549, -22.72916666530107221, -2.574251347313721627 ) ) ;
#20563=CARTESIAN_POINT ( 'NONE',  ( -3.152548672688508926E-16, -83.56249999863440792, -5.148502694627439702 ) ) ;
#20565=CARTESIAN_POINT ( 'NONE',  ( 5.000000000000000000, -23.37499999726881228, -6.123233995736766282E-16 ) ) ;
#20566=CARTESIAN_POINT ( 'NONE',  ( -2.229367062500000163, -50.47916666530107221, -3.861377020970580443 ) ) ;
#20569=DIRECTION ( 'NONE',  ( -0.000000000000000000, 1.000000000000000000, -0.000000000000000000 ) ) ;
#20570=CARTESIAN_POINT ( 'NONE',  ( -4.458734124999998549, -3.479166665301069994, 2.574251347313722516 ) ) ;
#20571=ORIENTED_EDGE ( 'NONE', *, *, #5537, .T. ) ;
#20573=CARTESIAN_POINT ( 'NONE',  ( 5.000000000000000000, -65.41666666666665719, -2.886751345948129988 ) ) ;
#20574=CARTESIAN_POINT ( 'NONE',  ( 3.152801135295367541, -150.5625000013655779, -3.152801135295367541 ) ) ;
#20577=CARTESIAN_POINT ( 'NONE',  ( 3.061616997868383141E-16, -157.7500000000000000, -5.000000000000000000 ) ) ;
#20581=CARTESIAN_POINT ( 'NONE',  ( 4.458734124999999437, -13.06249999863440259, -5.460374474430324690E-16 ) ) ;
#20582=CARTESIAN_POINT ( 'NONE',  ( -4.458734124999999437, -47.64583333196775072, -2.574251347313719407 ) ) ;
#20584=CARTESIAN_POINT ( 'NONE',  ( -1.846868145590734756, -144.1250000013655779, -4.458734125000000326 ) ) ;
#20586=LINE ( 'NONE', #60145, #36873 ) ;
#20587=ORIENTED_EDGE ( 'NONE', *, *, #63552, .F. ) ;
#20588=ADVANCED_FACE ( 'NONE', ( #24882 ), #35174, .T. ) ;
#20590=CARTESIAN_POINT ( 'NONE',  ( -6.972266317189433020E-16, -64.24999999999998579, -5.000000000000000000 ) ) ;
#20592=ADVANCED_FACE ( 'NONE', ( #5904 ), #442, .T. ) ;
#20593=CARTESIAN_POINT ( 'NONE',  ( 2.499999999999998668, -30.33333333333332860, -4.330127018922193649 ) ) ;
#20597=CARTESIAN_POINT ( 'NONE',  ( -6.972266317189433020E-16, 8.875000002731184168, -5.000000000000000000 ) ) ;
#20600=CARTESIAN_POINT ( 'NONE',  ( 2.229367062499998831, -9.645833331967738289, -3.861377020970580887 ) ) ;
#20601=CARTESIAN_POINT ( 'NONE',  ( 1.975475456537005874E-15, -73.62499999726878741, 5.000000000000000000 ) ) ;
#20602=CARTESIAN_POINT ( 'NONE',  ( -4.458734124999999437, -149.0000000013656063, -1.846868145590735644 ) ) ;
#20604=ORIENTED_EDGE ( 'NONE', *, *, #19666, .F. ) ;
#20608=LINE ( 'NONE', #59848, #32423 ) ;
#20612=CARTESIAN_POINT ( 'NONE',  ( -6.972266317189433020E-16, -74.25000000000000000, -5.000000000000000000 ) ) ;
#20615=CARTESIAN_POINT ( 'NONE',  ( -3.152548672688508926E-16, 12.43750000136559208, -5.148502694627439702 ) ) ;
#20617=ORIENTED_EDGE ( 'NONE', *, *, #51497, .F. ) ;
#20619=CARTESIAN_POINT ( 'NONE',  ( -4.458734124999999437, -12.56249999863440259, 0.000000000000000000 ) ) ;
#20621=CARTESIAN_POINT ( 'NONE',  ( -1.846868145590737420, -162.7500000013655779, 4.458734124999999437 ) ) ;
#20622=LINE ( 'NONE', #36359, #41820 ) ;
#20623=AXIS2_PLACEMENT_3D ( 'NONE', #52825, #49256, #64 ) ;
#20631=CARTESIAN_POINT ( 'NONE',  ( 3.152801135295367541, -150.5625000013655779, -3.152801135295367541 ) ) ;
#20633=CARTESIAN_POINT ( 'NONE',  ( 1.975475456537005874E-15, -57.62499999726880873, 5.000000000000000000 ) ) ;
#20639=CARTESIAN_POINT ( 'NONE',  ( -5.000000000000000000, -2.000000000000001776, 0.000000000000000000 ) ) ;
#20640=CARTESIAN_POINT ( 'NONE',  ( 9.457646018065525792E-16, -65.06249999863440792, 5.148502694627439702 ) ) ;
#20641=( BOUNDED_CURVE ( )  B_SPLINE_CURVE ( 2, ( #11243, #40826, #31817, #31181, #60471, #31487, #50810, #7068, #45661 ),
 .UNSPECIFIED., .F., .F. ) 
 B_SPLINE_CURVE_WITH_KNOTS ( ( 3, 2, 2, 2, 3 ),
 ( 0.6687499999999999556, 0.6694444444444443976, 0.6708333333333332815, 0.6722222222222222765, 0.6729166666666667185 ),
 .UNSPECIFIED. ) 
 CURVE ( )  GEOMETRIC_REPRESENTATION_ITEM ( )  RATIONAL_B_SPLINE_CURVE ( ( 0.9330127018922194093, 0.9330127018922194093, 1.000000000000000000, 0.8660254037844387076, 1.000000000000000000, 0.8660254037844387076, 1.000000000000000000, 0.9330127018922194093, 0.9330127018922194093 ) ) 
 REPRESENTATION_ITEM ( '' )  );
#20642=ADVANCED_FACE ( 'NONE', ( #20049 ), #31281, .T. ) ;
#20643=DIRECTION ( 'NONE',  ( -0.000000000000000000, 1.000000000000000000, -0.000000000000000000 ) ) ;
#20644=CARTESIAN_POINT ( 'NONE',  ( -5.000000000000000000, -9.874999997268815832, 0.000000000000000000 ) ) ;
#20645=CARTESIAN_POINT ( 'NONE',  ( -4.458734124999998549, -34.22916666530107221, 2.574251347313722516 ) ) ;
#20646=VERTEX_POINT ( 'NONE', #20703 ) ;
#20651=CARTESIAN_POINT ( 'NONE',  ( 5.000000000000000888, -52.58333333333332860, 2.886751345948126879 ) ) ;
#20652=CARTESIAN_POINT ( 'NONE',  ( 1.975475456537005874E-15, -46.62499999726880873, 5.000000000000000000 ) ) ;
#20655=CARTESIAN_POINT ( 'NONE',  ( 2.229367062499998831, -73.64583333196773651, -3.861377020970580887 ) ) ;
#20656=CARTESIAN_POINT ( 'NONE',  ( 4.458734125000000326, -141.6250000013656631, -1.846868145590734978 ) ) ;
#20657=CARTESIAN_POINT ( 'NONE',  ( 4.458734124999998549, -82.72916666530106511, -2.574251347313721627 ) ) ;
#20659=CARTESIAN_POINT ( 'NONE',  ( -4.458734124999999437, -32.56249999863440792, 0.000000000000000000 ) ) ;
#20661=FACE_OUTER_BOUND ( 'NONE', #50603, .T. ) ;
#20662=ORIENTED_EDGE ( 'NONE', *, *, #31889, .F. ) ;
#20664=CARTESIAN_POINT ( 'NONE',  ( -1.339745962155613812, 21.91965820146970856, -5.000000000000000000 ) ) ;
#20667=CARTESIAN_POINT ( 'NONE',  ( -6.972266317189433020E-16, -76.12499999726880162, -5.000000000000000000 ) ) ;
#20668=VECTOR ( 'NONE', #3080, 1000.000000000000000 ) ;
#20669=CARTESIAN_POINT ( 'NONE',  ( 2.229367062499998831, -64.89583333196773651, -3.861377020970580887 ) ) ;
#20671=VERTEX_POINT ( 'NONE', #40307 ) ;
#20672=CARTESIAN_POINT ( 'NONE',  ( 1.975475456537005874E-15, 5.375000002731185944, 5.000000000000000000 ) ) ;
#20674=CARTESIAN_POINT ( 'NONE',  ( -2.229367062499996610, 6.854166668032259935, 3.861377020970582219 ) ) ;
#20677=CARTESIAN_POINT ( 'NONE',  ( 4.458734124999999437, -161.3750000013656063, -1.846868145590734978 ) ) ;
#20684=FACE_OUTER_BOUND ( 'NONE', #54169, .T. ) ;
#20687=CARTESIAN_POINT ( 'NONE',  ( 5.000000000000000000, 12.70833333606451809, -2.886751345948130876 ) ) ;
#20688=DIRECTION ( 'NONE',  ( -0.000000000000000000, 1.000000000000000000, -0.000000000000000000 ) ) ;
#20690=( BOUNDED_CURVE ( )  B_SPLINE_CURVE ( 2, ( #25042, #44653, #614, #15400, #10560, #30171, #49802, #25364, #20551 ),
 .UNSPECIFIED., .F., .F. ) 
 B_SPLINE_CURVE_WITH_KNOTS ( ( 3, 2, 2, 2, 3 ),
 ( 0.01874999999999999931, 0.01944444444444444475, 0.02083333333333333218, 0.02222222222222222307, 0.02291666666666666852 ),
 .UNSPECIFIED. ) 
 CURVE ( )  GEOMETRIC_REPRESENTATION_ITEM ( )  RATIONAL_B_SPLINE_CURVE ( ( 0.9330127018922194093, 0.9330127018922194093, 1.000000000000000000, 0.8660254037844387076, 1.000000000000000000, 0.8660254037844387076, 1.000000000000000000, 0.9330127018922191873, 0.9330127018922194093 ) ) 
 REPRESENTATION_ITEM ( '' )  );
#20691=CARTESIAN_POINT ( 'NONE',  ( 1.339745962155612702, -82.16965819600734733, -5.000000000000000000 ) ) ;
#20694=CARTESIAN_POINT ( 'NONE',  ( 2.229367062499998831, -0.8958333319677401763, -3.861377020970580887 ) ) ;
#20695=FACE_OUTER_BOUND ( 'NONE', #44106, .T. ) ;
#20697=CARTESIAN_POINT ( 'NONE',  ( -5.000000000000000888, -144.5625000027311842, 2.071067811865474617 ) ) ;
#20698=CARTESIAN_POINT ( 'NONE',  ( -1.339745962155612480, 28.79465819873852439, -5.000000000000000888 ) ) ;
#20703=CARTESIAN_POINT ( 'NONE',  ( 3.061616997868383141E-16, -161.7500000000000000, -5.000000000000000000 ) ) ;
#20706=CARTESIAN_POINT ( 'NONE',  ( 2.730187237215162345E-16, -165.4375000013655779, -4.458734124999999437 ) ) ;
#20707=CARTESIAN_POINT ( 'NONE',  ( -5.000000000000000000, -160.5000000000000000, -6.123233995736766282E-16 ) ) ;
#20710=CARTESIAN_POINT ( 'NONE',  ( -8.190561711645485556E-16, -139.6875000013656063, 4.458734124999999437 ) ) ;
#20711=ORIENTED_EDGE ( 'NONE', *, *, #41156, .F. ) ;
#20712=CARTESIAN_POINT ( 'NONE',  ( 2.229367062500001939, 20.77083333469892779, 3.861377020970579999 ) ) ;
#20713=ORIENTED_EDGE ( 'NONE', *, *, #22478, .F. ) ;
#20714=CARTESIAN_POINT ( 'NONE',  ( -3.152548672688508926E-16, -64.81249999863440792, -5.148502694627439702 ) ) ;
#20716=CARTESIAN_POINT ( 'NONE',  ( 5.000000000000000888, 2.416666666666667851, 2.886751345948126879 ) ) ;
#20717=CARTESIAN_POINT ( 'NONE',  ( 1.060575238724906964E-15, 12.25000000000000000, 5.773502691896257311 ) ) ;
#20718=CARTESIAN_POINT ( 'NONE',  ( 4.458734124999998549, -50.72916666530106511, -2.574251347313721627 ) ) ;
#20719=CARTESIAN_POINT ( 'NONE',  ( 4.458734124999998549, -11.72916666530107044, -2.574251347313721627 ) ) ;
#20725=CARTESIAN_POINT ( 'NONE',  ( 1.975475456537005874E-15, -79.74999999999998579, 5.000000000000000000 ) ) ;
#20726=CARTESIAN_POINT ( 'NONE',  ( -4.458734124999998549, -57.22916666530107932, 2.574251347313722516 ) ) ;
#20727=CARTESIAN_POINT ( 'NONE',  ( 3.152801135295366208, -155.8125000013656063, 3.152801135295367985 ) ) ;
#20728=CARTESIAN_POINT ( 'NONE',  ( -2.499999999999996447, -56.70833333060214443, 4.330127018922195425 ) ) ;
#20731=CARTESIAN_POINT ( 'NONE',  ( -2.229367062499996610, -0.3958333319677397322, 3.861377020970582219 ) ) ;
#20734=CARTESIAN_POINT ( 'NONE',  ( 4.458734124999999437, -155.4375000013655779, 0.000000000000000000 ) ) ;
#20739=CARTESIAN_POINT ( 'NONE',  ( -9.184850993605147944E-16, -153.2500000000000000, 5.000000000000000000 ) ) ;
#20740=CARTESIAN_POINT ( 'NONE',  ( 4.458734124999998549, -48.97916666530107221, -2.574251347313721627 ) ) ;
#20741=VERTEX_POINT ( 'NONE', #11030 ) ;
#20744=CARTESIAN_POINT ( 'NONE',  ( 2.229367062500001939, 29.02083333469892779, 3.861377020970579999 ) ) ;
#20746=CARTESIAN_POINT ( 'NONE',  ( -3.535533905932738641, -165.3750000000000284, 3.535533905932737309 ) ) ;
#20749=CARTESIAN_POINT ( 'NONE',  ( -2.500000000000000444, 0.8333333333333317050, -4.330127018922193649 ) ) ;
#20751=CYLINDRICAL_SURFACE ( 'NONE', #37014, 5.000000000000000000 ) ;
#20755=CARTESIAN_POINT ( 'NONE',  ( -5.000000000000000000, 24.91666666666666785, -2.886751345948128211 ) ) ;
#20757=CARTESIAN_POINT ( 'NONE',  ( -4.458734124999998549, -90.47916666530106511, 2.574251347313722516 ) ) ;
#20758=LINE ( 'NONE', #60004, #43906 ) ;
#20760=VERTEX_POINT ( 'NONE', #30654 ) ;
#20761=CARTESIAN_POINT ( 'NONE',  ( 1.339745962155612702, -31.29465819873851373, -5.000000000000000000 ) ) ;
#20763=CARTESIAN_POINT ( 'NONE',  ( -2.071067811865478170, -156.4375000027311842, 5.000000000000000000 ) ) ;
#20766=EDGE_CURVE ( 'NONE', #33720, #53313, #6222, .T. ) ;
#20767=CARTESIAN_POINT ( 'NONE',  ( -2.498395430326213474E-14, 22.25000000000000000, 5.000000000000000000 ) ) ;
#20769=CARTESIAN_POINT ( 'NONE',  ( -2.500000000000000444, -67.16666666666667140, -4.330127018922193649 ) ) ;
#20776=CARTESIAN_POINT ( 'NONE',  ( 4.458734124999998549, -17.72916666530106866, -2.574251347313721627 ) ) ;
#20778=CARTESIAN_POINT ( 'NONE',  ( 5.000000000000000888, -152.9375000000000000, -2.071067811865475505 ) ) ;
#20780=CARTESIAN_POINT ( 'NONE',  ( -4.458734125000001214, -156.8750000013655779, 1.846868145590734089 ) ) ;
#20782=CARTESIAN_POINT ( 'NONE',  ( 2.229367062499998831, -46.89583333196774362, -3.861377020970580887 ) ) ;
#20785=CARTESIAN_POINT ( 'NONE',  ( -4.458734124999998549, -90.22916666530106511, 2.574251347313722516 ) ) ;
#20786=CARTESIAN_POINT ( 'NONE',  ( 4.458734125000001214, 5.104166668032261711, 2.574251347313718519 ) ) ;
#20789=EDGE_CURVE ( 'NONE', #41833, #15263, #27730, .T. ) ;
#20790=CYLINDRICAL_SURFACE ( 'NONE', #59461, 5.000000000000000000 ) ;
#20792=CARTESIAN_POINT ( 'NONE',  ( -4.458734124999999437, 18.35416666803225993, -2.574251347313719407 ) ) ;
#20794=CARTESIAN_POINT ( 'NONE',  ( -5.000000000000000000, 11.04166666939785202, -2.886751345948128211 ) ) ;
#20795=ORIENTED_EDGE ( 'NONE', *, *, #18453, .F. ) ;
#20797=ORIENTED_EDGE ( 'NONE', *, *, #27967, .T. ) ;
#20799=CARTESIAN_POINT ( 'NONE',  ( 4.458734124999998549, -44.72916666530106511, -2.574251347313721627 ) ) ;
#20800=ADVANCED_FACE ( 'NONE', ( #47357 ), #32559, .T. ) ;
#20801=CARTESIAN_POINT ( 'NONE',  ( 2.499999999999998668, -41.20833333060214443, -4.330127018922193649 ) ) ;
#20802=EDGE_LOOP ( 'NONE', ( #40445, #17562, #36902, #55721 ) ) ;
#20803=CARTESIAN_POINT ( 'NONE',  ( -4.458734124999999437, -17.31249999863440792, 0.000000000000000000 ) ) ;
#20805=CARTESIAN_POINT ( 'NONE',  ( 5.000000000000000000, -80.41666666666667140, -2.886751345948129988 ) ) ;
#20806=CARTESIAN_POINT ( 'NONE',  ( 3.152801135295366208, -167.5625000013656063, 3.152801135295367985 ) ) ;
#20807=CARTESIAN_POINT ( 'NONE',  ( -2.500000000000000444, -86.04166666393547303, -4.330127018922193649 ) ) ;
#20811=CARTESIAN_POINT ( 'NONE',  ( 2.229367062500001939, -28.22916666530107221, 3.861377020970579999 ) ) ;
#20813=ORIENTED_EDGE ( 'NONE', *, *, #61024, .T. ) ;
#20814=( BOUNDED_CURVE ( )  B_SPLINE_CURVE ( 2, ( #17651, #28231, #37267, #47846, #23741, #18893, #3804, #32435, #23427 ),
 .UNSPECIFIED., .F., .F. ) 
 B_SPLINE_CURVE_WITH_KNOTS ( ( 3, 2, 2, 2, 3 ),
 ( 0.3604166666666666630, 0.3611111111111111049, 0.3624999999999999889, 0.3638888888888888729, 0.3645833333333333148 ),
 .UNSPECIFIED. ) 
 CURVE ( )  GEOMETRIC_REPRESENTATION_ITEM ( )  RATIONAL_B_SPLINE_CURVE ( ( 0.9330127018922194093, 0.9330127018922194093, 1.000000000000000000, 0.8660254037844387076, 1.000000000000000000, 0.8660254037844387076, 1.000000000000000000, 0.9330127018922194093, 0.9330127018922194093 ) ) 
 REPRESENTATION_ITEM ( '' )  );
#20816=CARTESIAN_POINT ( 'NONE',  ( -8.190561711645485556E-16, -163.9375000013655779, 4.458734124999999437 ) ) ;
#20820=ORIENTED_EDGE ( 'NONE', *, *, #33138, .T. ) ;
#20821=CARTESIAN_POINT ( 'NONE',  ( -5.000000000000000000, -26.00000000000000355, 0.000000000000000000 ) ) ;
#20823=CARTESIAN_POINT ( 'NONE',  ( -3.152548672688508926E-16, -72.81249999863439371, -5.148502694627439702 ) ) ;
#20826=CARTESIAN_POINT ( 'NONE',  ( -3.152801135295367096, -142.3125000013655779, -3.152801135295367541 ) ) ;
#20827=CARTESIAN_POINT ( 'NONE',  ( 1.975475456537005874E-15, -57.74999999999999289, 5.000000000000000000 ) ) ;
#20829=CARTESIAN_POINT ( 'NONE',  ( -2.229367062499996610, -48.14583333196772941, 3.861377020970582219 ) ) ;
#20833=( BOUNDED_CURVE ( )  B_SPLINE_CURVE ( 2, ( #54207, #49384, #16256, #10144, #59684, #29751, #35875, #5973, #11418 ),
 .UNSPECIFIED., .F., .F. ) 
 B_SPLINE_CURVE_WITH_KNOTS ( ( 3, 2, 2, 2, 3 ),
 ( 0.8416666666666664520, 0.8458333333333331039, 0.8499999999999997558, 0.8541666666666664076, 0.8583333333333330595 ),
 .UNSPECIFIED. ) 
 CURVE ( )  GEOMETRIC_REPRESENTATION_ITEM ( )  RATIONAL_B_SPLINE_CURVE ( ( 1.000000000000003997, 0.9238795325112826307, 1.000000000000000000, 0.9238795325112867385, 1.000000000000000000, 0.9238795325112867385, 1.000000000000000000, 0.9238795325112908463, 0.9999999999999958922 ) ) 
 REPRESENTATION_ITEM ( '' )  );
#20834=CARTESIAN_POINT ( 'NONE',  ( -5.147856630858197489E-14, 4.249999999999996447, 5.000000000000000000 ) ) ;
#20838=CARTESIAN_POINT ( 'NONE',  ( 4.458734124999999437, -72.06249999863439371, -5.460374474430324690E-16 ) ) ;
#20839=CARTESIAN_POINT ( 'NONE',  ( 0.000000000000000000, -170.0000000000000000, 0.000000000000000000 ) ) ;
#20840=CARTESIAN_POINT ( 'NONE',  ( 1.975475456537005874E-15, -18.74999999999999645, 5.000000000000000000 ) ) ;
#20843=CARTESIAN_POINT ( 'NONE',  ( 5.000000000000000888, -145.9375000000000000, -2.071067811865475505 ) ) ;
#20844=CARTESIAN_POINT ( 'NONE',  ( 1.339745962155618697, 23.83034180399267044, -4.999999999999998224 ) ) ;
#20847=CARTESIAN_POINT ( 'NONE',  ( -5.000000000000000000, -167.6250000027312126, -6.123233995736766282E-16 ) ) ;
#20849=ADVANCED_FACE ( 'NONE', ( #46087 ), #13255, .T. ) ;
#20850=CARTESIAN_POINT ( 'NONE',  ( -2.229367062500000163, 20.27083333469892779, -3.861377020970580443 ) ) ;
#20851=CARTESIAN_POINT ( 'NONE',  ( 0.000000000000000000, -170.0000000000000000, 5.000000000000000000 ) ) ;
#20853=EDGE_CURVE ( 'NONE', #55791, #21047, #2259, .T. ) ;
#20859=CARTESIAN_POINT ( 'NONE',  ( -2.229367062499996610, -83.14583333196773651, 3.861377020970582219 ) ) ;
#20860=CARTESIAN_POINT ( 'NONE',  ( -3.152548672688508926E-16, -2.562499998634407028, -5.148502694627439702 ) ) ;
#20862=CARTESIAN_POINT ( 'NONE',  ( 4.458734125000000326, -32.14583333196773651, 2.574251347313718519 ) ) ;
#20866=CARTESIAN_POINT ( 'NONE',  ( 4.458734125000001214, 19.10416666803225638, 2.574251347313718519 ) ) ;
#20867=DIRECTION ( 'NONE',  ( -0.000000000000000000, 1.000000000000000000, -0.000000000000000000 ) ) ;
#20868=EDGE_CURVE ( 'NONE', #25022, #34977, #56065, .T. ) ;
#20869=CARTESIAN_POINT ( 'NONE',  ( 0.000000000000000000, -170.0000000000000000, 0.000000000000000000 ) ) ;
#20870=CARTESIAN_POINT ( 'NONE',  ( 2.229367062499998831, -79.89583333196773651, -3.861377020970580887 ) ) ;
#20872=CARTESIAN_POINT ( 'NONE',  ( 1.975475456537005874E-15, -80.74999999999998579, 5.000000000000000000 ) ) ;
#20873=CARTESIAN_POINT ( 'NONE',  ( 5.000000000000000888, 26.54166666939785202, 2.886751345948126879 ) ) ;
#20874=EDGE_LOOP ( 'NONE', ( #38596, #62827, #9094, #26243 ) ) ;
#20875=DIRECTION ( 'NONE',  ( -0.000000000000000000, 1.000000000000000000, -0.000000000000000000 ) ) ;
#20877=CARTESIAN_POINT ( 'NONE',  ( -3.535250795749689387E-16, -18.25000000000000355, -5.773502691896257311 ) ) ;
#20878=CARTESIAN_POINT ( 'NONE',  ( -4.458734124999998549, -20.22916666530107221, 2.574251347313722516 ) ) ;
#20879=CARTESIAN_POINT ( 'NONE',  ( 4.458734124999998549, -86.72916666530107932, -2.574251347313721627 ) ) ;
#20880=CARTESIAN_POINT ( 'NONE',  ( 2.499999999999998668, -23.20833333060214443, -4.330127018922193649 ) ) ;
#20881=CARTESIAN_POINT ( 'NONE',  ( -3.152548672688508926E-16, -57.56249999863439371, -5.148502694627439702 ) ) ;
#20883=CARTESIAN_POINT ( 'NONE',  ( 2.500000000000002220, -27.66666666666666430, 4.330127018922192761 ) ) ;
#20885=CARTESIAN_POINT ( 'NONE',  ( 2.229367062500001939, -6.229166665301072214, 3.861377020970579999 ) ) ;
#20886=ORIENTED_EDGE ( 'NONE', *, *, #29530, .F. ) ;
#20888=CARTESIAN_POINT ( 'NONE',  ( -4.999999999999999112, -66.91666666666667140, 2.886751345948131764 ) ) ;
#20889=CARTESIAN_POINT ( 'NONE',  ( -4.458734125000001214, -154.1250000013656063, 1.846868145590734089 ) ) ;
#20893=CARTESIAN_POINT ( 'NONE',  ( -3.535533905932737309, -159.6250000000000284, -3.535533905932738197 ) ) ;
#20896=CARTESIAN_POINT ( 'NONE',  ( -4.458734124999998549, -13.47916666530107221, 2.574251347313722516 ) ) ;
#20897=CARTESIAN_POINT ( 'NONE',  ( -4.458734124999998549, -52.47916666530107221, 2.574251347313722516 ) ) ;
#20899=CARTESIAN_POINT ( 'NONE',  ( -8.190561711645485556E-16, -143.6875000013656063, 4.458734124999999437 ) ) ;
#20904=CARTESIAN_POINT ( 'NONE',  ( -2.229367062499996610, 26.60416666803225993, 3.861377020970582219 ) ) ;
#20906=CARTESIAN_POINT ( 'NONE',  ( 5.000000000000000000, -29.29166666393548013, -2.886751345948130876 ) ) ;
#20912=CARTESIAN_POINT ( 'NONE',  ( -4.458734124999999437, -6.312499998634403475, 0.000000000000000000 ) ) ;
#20913=DIRECTION ( 'NONE',  ( -0.000000000000000000, 1.000000000000000000, -0.000000000000000000 ) ) ;
#20914=CARTESIAN_POINT ( 'NONE',  ( -8.190561711645485556E-16, -148.6875000013656063, 4.458734124999999437 ) ) ;
#20918=CARTESIAN_POINT ( 'NONE',  ( -4.999999999999998224, -62.79166666393546592, 2.886751345948131764 ) ) ;
#20922=CARTESIAN_POINT ( 'NONE',  ( -4.999999999999998224, -5.916666666666666963, 2.886751345948131764 ) ) ;
#20924=EDGE_CURVE ( 'NONE', #48046, #51146, #60892, .T. ) ;
#20929=EDGE_CURVE ( 'NONE', #46416, #36547, #36760, .T. ) ;
#20930=CARTESIAN_POINT ( 'NONE',  ( -4.458734124999997661, 12.77083333469892779, 2.574251347313722516 ) ) ;
#20932=CARTESIAN_POINT ( 'NONE',  ( 4.458734124999999437, -13.06249999863440259, -5.460374474430324690E-16 ) ) ;
#20935=CARTESIAN_POINT ( 'NONE',  ( 3.152801135295367541, -165.3125000013656063, -3.152801135295367541 ) ) ;
#20940=EDGE_CURVE ( 'NONE', #5665, #15117, #61531, .T. ) ;
#20944=CARTESIAN_POINT ( 'NONE',  ( -4.999999999999998224, -88.79166666393548724, 2.886751345948131764 ) ) ;
#20945=CARTESIAN_POINT ( 'NONE',  ( -4.458734124999999437, -38.31249999863439371, 0.000000000000000000 ) ) ;
#20947=CARTESIAN_POINT ( 'NONE',  ( 4.458734124999999437, -148.6875000013656063, 0.000000000000000000 ) ) ;
#20951=VERTEX_POINT ( 'NONE', #29286 ) ;
#20956=CARTESIAN_POINT ( 'NONE',  ( 5.000000000000000888, -3.583333333333333925, 2.886751345948126879 ) ) ;
#20957=CARTESIAN_POINT ( 'NONE',  ( 4.458734125000000326, -67.89583333196773651, 2.574251347313718519 ) ) ;
#20958=CARTESIAN_POINT ( 'NONE',  ( 5.000000000000000888, -22.45833333060214443, 2.886751345948126879 ) ) ;
#20960=CARTESIAN_POINT ( 'NONE',  ( 2.499999999999998668, -10.20833333060214621, -4.330127018922193649 ) ) ;
#20961=CARTESIAN_POINT ( 'NONE',  ( -4.458734124999999437, -37.31249999863440792, 0.000000000000000000 ) ) ;
#20962=ORIENTED_EDGE ( 'NONE', *, *, #11984, .T. ) ;
#20963=CARTESIAN_POINT ( 'NONE',  ( 0.000000000000000000, -170.0000000000000000, 0.000000000000000000 ) ) ;
#20965=CARTESIAN_POINT ( 'NONE',  ( -4.458734124999998549, 11.52083333469892779, 2.574251347313722516 ) ) ;
#20966=ORIENTED_EDGE ( 'NONE', *, *, #57018, .T. ) ;
#20967=DIRECTION ( 'NONE',  ( -0.000000000000000000, 1.000000000000000000, -0.000000000000000000 ) ) ;
#20968=CARTESIAN_POINT ( 'NONE',  ( -4.999999999999999112, -52.91666666666666430, 2.886751345948131764 ) ) ;
#20970=CARTESIAN_POINT ( 'NONE',  ( 9.457646018065525792E-16, -75.06249999863439371, 5.148502694627439702 ) ) ;
#20971=CARTESIAN_POINT ( 'NONE',  ( -8.190561711645485556E-16, -141.9375000013656063, 4.458734124999999437 ) ) ;
#20972=CARTESIAN_POINT ( 'NONE',  ( -4.458734124999999437, -81.39583333196773651, -2.574251347313719407 ) ) ;
#20974=CARTESIAN_POINT ( 'NONE',  ( 9.457646018065525792E-16, -36.31249999863440792, 5.148502694627439702 ) ) ;
#20980=ORIENTED_EDGE ( 'NONE', *, *, #39621, .T. ) ;
#20983=CARTESIAN_POINT ( 'NONE',  ( -2.229367062500000163, -64.72916666530106511, -3.861377020970580443 ) ) ;
#20986=CARTESIAN_POINT ( 'NONE',  ( 2.500000000000002220, -62.66666666666666430, 4.330127018922192761 ) ) ;
#20988=CARTESIAN_POINT ( 'NONE',  ( 9.457646018065525792E-16, 5.937500001365592972, 5.148502694627439702 ) ) ;
#20990=CARTESIAN_POINT ( 'NONE',  ( -1.846868145590737420, -159.7500000013656063, 4.458734124999997661 ) ) ;
#20994=CARTESIAN_POINT ( 'NONE',  ( -6.972266317189433020E-16, -17.12499999726881583, -5.000000000000000000 ) ) ;
#20997=CARTESIAN_POINT ( 'NONE',  ( -4.999999999999998224, -67.91666666666667140, 2.886751345948131764 ) ) ;
#21001=CARTESIAN_POINT ( 'NONE',  ( -6.972266317189433020E-16, -78.12499999726881583, -5.000000000000000000 ) ) ;
#21003=CARTESIAN_POINT ( 'NONE',  ( -4.458734124999999437, 26.68750000136559564, 0.000000000000000000 ) ) ;
#21007=CARTESIAN_POINT ( 'NONE',  ( 4.458734124999998549, 0.02083333469892617584, -2.574251347313721627 ) ) ;
#21009=CARTESIAN_POINT ( 'NONE',  ( -3.535533905932737309, -143.7500000027311842, -3.535533905932738197 ) ) ;
#21018=CARTESIAN_POINT ( 'NONE',  ( 1.846868145590736310, -162.8750000013655779, 4.458734124999997661 ) ) ;
#21022=VERTEX_POINT ( 'NONE', #48916 ) ;
#21023=CARTESIAN_POINT ( 'NONE',  ( 4.458734124999998549, 25.02083333469892423, -2.574251347313721627 ) ) ;
#21024=ORIENTED_EDGE ( 'NONE', *, *, #48019, .T. ) ;
#21025=CARTESIAN_POINT ( 'NONE',  ( 2.229367062499998831, -60.89583333196774362, -3.861377020970580887 ) ) ;
#21028=CARTESIAN_POINT ( 'NONE',  ( -5.000000000000000000, 13.99999999999999822, 0.000000000000000000 ) ) ;
#21029=CARTESIAN_POINT ( 'NONE',  ( -4.458734124999999437, -49.31249999863440792, 0.000000000000000000 ) ) ;
#21030=CARTESIAN_POINT ( 'NONE',  ( 2.229367062499998831, -11.64583333196774007, -3.861377020970580887 ) ) ;
#21031=CYLINDRICAL_SURFACE ( 'NONE', #4094, 5.000000000000000000 ) ;
#21034=CARTESIAN_POINT ( 'NONE',  ( 1.975475456537005874E-15, -63.62499999726880873, 5.000000000000000000 ) ) ;
#21037=CARTESIAN_POINT ( 'NONE',  ( 5.000000000000000000, -35.41666666666667140, -2.886751345948129988 ) ) ;
#21039=CARTESIAN_POINT ( 'NONE',  ( 5.000000000000000888, 21.54166666939785202, 2.886751345948126879 ) ) ;
#21041=CARTESIAN_POINT ( 'NONE',  ( -4.999999999999998224, -31.79166666393548724, 2.886751345948131764 ) ) ;
#21042=CARTESIAN_POINT ( 'NONE',  ( -2.229367062499996610, -61.14583333196774362, 3.861377020970582219 ) ) ;
#21043=CARTESIAN_POINT ( 'NONE',  ( -1.846868145590734756, -153.3750000013656347, -4.458734125000000326 ) ) ;
#21044=CARTESIAN_POINT ( 'NONE',  ( 4.458734124999998549, -65.72916666530106511, -2.574251347313721627 ) ) ;
#21046=CARTESIAN_POINT ( 'NONE',  ( -2.500000000000000444, -57.04166666393548013, -4.330127018922193649 ) ) ;
#21047=VERTEX_POINT ( 'NONE', #4241 ) ;
#21051=CARTESIAN_POINT ( 'NONE',  ( -8.190561711645485556E-16, -152.6875000013656063, 4.458734124999999437 ) ) ;
#21055=CARTESIAN_POINT ( 'NONE',  ( 3.535533905932736864, -153.1250000000000000, 3.535533905932738641 ) ) ;
#21056=CARTESIAN_POINT ( 'NONE',  ( 2.229367062500001939, -49.22916666530107221, 3.861377020970579999 ) ) ;
#21061=CARTESIAN_POINT ( 'NONE',  ( 4.458734124999999437, 26.18750000136559564, -5.460374474430324690E-16 ) ) ;
#21067=CARTESIAN_POINT ( 'NONE',  ( 2.500000000000002220, -28.54166666393548013, 4.330127018922192761 ) ) ;
#21070=CARTESIAN_POINT ( 'NONE',  ( -9.184850993605147944E-16, -161.3750000027311842, 5.000000000000000000 ) ) ;
#21073=DIRECTION ( 'NONE',  ( 0.000000000000000000, 0.000000000000000000, 1.000000000000000000 ) ) ;
#21078=ORIENTED_EDGE ( 'NONE', *, *, #49227, .F. ) ;
#21079=CARTESIAN_POINT ( 'NONE',  ( 3.061616997868383141E-16, -169.7500000000000000, -5.000000000000000000 ) ) ;
#21081=CARTESIAN_POINT ( 'NONE',  ( 3.535533905932736864, -159.2500000027312126, 3.535533905932738641 ) ) ;
#21092=CARTESIAN_POINT ( 'NONE',  ( -2.229367062500000163, -19.47916666530106866, -3.861377020970580443 ) ) ;
#21093=CARTESIAN_POINT ( 'NONE',  ( 5.000000000000000000, -75.41666666666667140, -2.886751345948130876 ) ) ;
#21094=CARTESIAN_POINT ( 'NONE',  ( -5.000000000000000888, -151.5625000000000568, -2.071067811865475949 ) ) ;
#21096=CARTESIAN_POINT ( 'NONE',  ( -3.152801135295367985, -153.8125000013656063, 3.152801135295367096 ) ) ;
#21097=VERTEX_POINT ( 'NONE', #53126 ) ;
#21098=CARTESIAN_POINT ( 'NONE',  ( 2.229367062499998831, -43.89583333196774362, -3.861377020970580887 ) ) ;
#21100=CARTESIAN_POINT ( 'NONE',  ( 2.229367062500001939, -88.97916666530106511, 3.861377020970579999 ) ) ;
#21101=CARTESIAN_POINT ( 'NONE',  ( 4.458734124999998549, 5.270833334698926897, -2.574251347313721627 ) ) ;
#21102=CARTESIAN_POINT ( 'NONE',  ( -3.535533905932737309, -142.6250000000000000, -3.535533905932738197 ) ) ;
#21103=DIRECTION ( 'NONE',  ( -0.000000000000000000, 1.000000000000000000, -0.000000000000000000 ) ) ;
#21105=CARTESIAN_POINT ( 'NONE',  ( 2.229367062499998831, 18.10416666803225993, -3.861377020970580887 ) ) ;
#21107=CARTESIAN_POINT ( 'NONE',  ( 2.500000000000002220, 9.458333336064519870, 4.330127018922192761 ) ) ;
#21108=ORIENTED_EDGE ( 'NONE', *, *, #51078, .T. ) ;
#21110=ORIENTED_EDGE ( 'NONE', *, *, #40828, .T. ) ;
#21111=( BOUNDED_CURVE ( )  B_SPLINE_CURVE ( 2, ( #56061, #31606, #22605, #38015, #57647, #33193, #13575, #62153, #12930 ),
 .UNSPECIFIED., .F., .F. ) 
 B_SPLINE_CURVE_WITH_KNOTS ( ( 3, 2, 2, 2, 3 ),
 ( 0.8687500000000000222, 0.8694444444444444642, 0.8708333333333333481, 0.8722222222222222321, 0.8729166666666666741 ),
 .UNSPECIFIED. ) 
 CURVE ( )  GEOMETRIC_REPRESENTATION_ITEM ( )  RATIONAL_B_SPLINE_CURVE ( ( 0.9330127018922194093, 0.9330127018922194093, 1.000000000000000000, 0.8660254037844387076, 1.000000000000000000, 0.8660254037844387076, 1.000000000000000000, 0.9330127018922194093, 0.9330127018922194093 ) ) 
 REPRESENTATION_ITEM ( '' )  );
#21113=CARTESIAN_POINT ( 'NONE',  ( -3.152548672688508926E-16, -44.56249999863440081, -5.148502694627439702 ) ) ;
#21114=CARTESIAN_POINT ( 'NONE',  ( -3.152801135295367985, -165.0625000013656063, 3.152801135295367096 ) ) ;
#21115=CARTESIAN_POINT ( 'NONE',  ( -5.000000000000000000, -37.87499999726881583, 0.000000000000000000 ) ) ;
#21116=ORIENTED_EDGE ( 'NONE', *, *, #9862, .F. ) ;
#21117=CARTESIAN_POINT ( 'NONE',  ( -4.458734124999999437, -16.39583333196773651, -2.574251347313719407 ) ) ;
#21118=VERTEX_POINT ( 'NONE', #57652 ) ;
#21119=CARTESIAN_POINT ( 'NONE',  ( 5.000000000000000000, -88.41666666666665719, -2.886751345948129988 ) ) ;
#21120=CARTESIAN_POINT ( 'NONE',  ( 2.730187237215162345E-16, -169.1875000013656063, -4.458734124999999437 ) ) ;
#21121=CARTESIAN_POINT ( 'NONE',  ( -5.000000000000000000, -86.95833333060214443, -2.886751345948128211 ) ) ;
#21122=CARTESIAN_POINT ( 'NONE',  ( -5.000000000000000000, -19.08333333333333570, -2.886751345948128211 ) ) ;
#21123=ORIENTED_EDGE ( 'NONE', *, *, #12668, .F. ) ;
#21126=CARTESIAN_POINT ( 'NONE',  ( 4.458734124999998549, -34.97916666530107221, -2.574251347313721627 ) ) ;
#21127=CARTESIAN_POINT ( 'NONE',  ( 2.500000000000002220, -29.66666666666666785, 4.330127018922192761 ) ) ;
#21134=CARTESIAN_POINT ( 'NONE',  ( -9.184850993605147944E-16, -166.3750000027312126, 5.000000000000000000 ) ) ;
#21136=CARTESIAN_POINT ( 'NONE',  ( -2.229367062499996610, -81.39583333196773651, 3.861377020970582219 ) ) ;
#21139=CARTESIAN_POINT ( 'NONE',  ( -8.190561711645485556E-16, -143.9375000013656063, 4.458734124999999437 ) ) ;
#21140=CARTESIAN_POINT ( 'NONE',  ( -5.000000000000000000, -58.08333333333333570, -2.886751345948128211 ) ) ;
#21142=CARTESIAN_POINT ( 'NONE',  ( 4.458734125000000326, -46.89583333196773651, 2.574251347313718519 ) ) ;
#21143=CARTESIAN_POINT ( 'NONE',  ( -1.339745962155613812, 27.79465819873851729, -5.000000000000000000 ) ) ;
#21147=CARTESIAN_POINT ( 'NONE',  ( -8.190561711645485556E-16, -139.9375000013656063, 4.458734124999999437 ) ) ;
#21152=CARTESIAN_POINT ( 'NONE',  ( 4.458734124999998549, -72.97916666530107932, -2.574251347313721627 ) ) ;
#21153=CARTESIAN_POINT ( 'NONE',  ( 5.000000000000000000, -34.41666666666666430, -2.886751345948130876 ) ) ;
#21155=VERTEX_POINT ( 'NONE', #28980 ) ;
#21160=CARTESIAN_POINT ( 'NONE',  ( -4.999999999999998224, -4.916666666666666075, 2.886751345948131764 ) ) ;
#21162=CARTESIAN_POINT ( 'NONE',  ( -3.152548672688508926E-16, 15.18750000136559564, -5.148502694627439702 ) ) ;
#21168=CARTESIAN_POINT ( 'NONE',  ( -2.229367062500000163, -86.47916666530107932, -3.861377020970580443 ) ) ;
#21169=CARTESIAN_POINT ( 'NONE',  ( -2.229367062500000163, -4.479166665301070438, -3.861377020970580443 ) ) ;
#21171=EDGE_LOOP ( 'NONE', ( #34323, #26057, #60964 ) ) ;
#21172=CARTESIAN_POINT ( 'NONE',  ( 4.458734124999999437, -29.06249999863440436, -5.460374474430324690E-16 ) ) ;
#21176=AXIS2_PLACEMENT_3D ( 'NONE', #2107, #50969, #5954 ) ;
#21178=CARTESIAN_POINT ( 'NONE',  ( -3.152548672688508926E-16, 21.43750000136559564, -5.148502694627439702 ) ) ;
#21179=CARTESIAN_POINT ( 'NONE',  ( 1.339745962155615144, 1.294658198738520172, 4.999999999999999112 ) ) ;
#21180=CARTESIAN_POINT ( 'NONE',  ( 9.457646018065525792E-16, -79.31249999863440792, 5.148502694627439702 ) ) ;
#21183=CARTESIAN_POINT ( 'NONE',  ( 5.000000000000000000, 22.70833333606451632, -2.886751345948129988 ) ) ;
#21185=CARTESIAN_POINT ( 'NONE',  ( -5.000000000000000000, -66.00000000000000000, 0.000000000000000000 ) ) ;
#21186=DIRECTION ( 'NONE',  ( -0.000000000000000000, 1.000000000000000000, -0.000000000000000000 ) ) ;
#21188=CARTESIAN_POINT ( 'NONE',  ( -2.499999999999996447, -21.83333333333332860, 4.330127018922195425 ) ) ;
#21189=CARTESIAN_POINT ( 'NONE',  ( 2.229367062499998831, -28.64583333196774007, -3.861377020970580887 ) ) ;
#21190=CARTESIAN_POINT ( 'NONE',  ( 2.229367062500001939, -86.97916666530107932, 3.861377020970579999 ) ) ;
#21191=( BOUNDED_CURVE ( )  B_SPLINE_CURVE ( 2, ( #29166, #25946, #1519, #6973, #16932, #21122, #41674, #21769, #46202 ),
 .UNSPECIFIED., .F., .F. ) 
 B_SPLINE_CURVE_WITH_KNOTS ( ( 3, 2, 2, 2, 3 ),
 ( 0.4062500000000000000, 0.4069444444444444420, 0.4083333333333333259, 0.4097222222222222099, 0.4104166666666666519 ),
 .UNSPECIFIED. ) 
 CURVE ( )  GEOMETRIC_REPRESENTATION_ITEM ( )  RATIONAL_B_SPLINE_CURVE ( ( 0.9330127018922194093, 0.9330127018922194093, 1.000000000000000000, 0.8660254037844387076, 1.000000000000000000, 0.8660254037844387076, 1.000000000000000000, 0.9330127018922194093, 0.9330127018922194093 ) ) 
 REPRESENTATION_ITEM ( '' )  );
#21192=CARTESIAN_POINT ( 'NONE',  ( 5.000000000000000000, -24.37499999726881228, -6.123233995736766282E-16 ) ) ;
#21193=CARTESIAN_POINT ( 'NONE',  ( 9.457646018065525792E-16, -57.06249999863440081, 5.148502694627439702 ) ) ;
#21196=CYLINDRICAL_SURFACE ( 'NONE', #36467, 5.000000000000000000 ) ;
#21197=CARTESIAN_POINT ( 'NONE',  ( -2.229367062500000163, -4.729166665301071326, -3.861377020970580443 ) ) ;
#21199=CARTESIAN_POINT ( 'NONE',  ( -5.000000000000000000, -72.00000000000000000, 0.000000000000000000 ) ) ;
#21200=CARTESIAN_POINT ( 'NONE',  ( -3.152801135295367096, -152.3125000013655779, -3.152801135295367541 ) ) ;
#21203=CARTESIAN_POINT ( 'NONE',  ( 3.535533905932736864, -158.1250000000000284, 3.535533905932738641 ) ) ;
#21207=CARTESIAN_POINT ( 'NONE',  ( 2.229367062499998831, -14.89583333196773474, -3.861377020970580887 ) ) ;
#21208=CARTESIAN_POINT ( 'NONE',  ( 2.229367062499998831, -52.89583333196773651, -3.861377020970580887 ) ) ;
#21209=( BOUNDED_CURVE ( )  B_SPLINE_CURVE ( 2, ( #391, #43480, #4884, #24185, #53766, #58291, #15170, #19993, #72 ),
 .UNSPECIFIED., .F., .F. ) 
 B_SPLINE_CURVE_WITH_KNOTS ( ( 3, 2, 2, 2, 3 ),
 ( 0.2020833333333333370, 0.2027777777777777790, 0.2041666666666666630, 0.2055555555555555469, 0.2062499999999999889 ),
 .UNSPECIFIED. ) 
 CURVE ( )  GEOMETRIC_REPRESENTATION_ITEM ( )  RATIONAL_B_SPLINE_CURVE ( ( 0.9330127018922194093, 0.9330127018922194093, 1.000000000000000000, 0.8660254037844387076, 1.000000000000000000, 0.8660254037844387076, 1.000000000000000000, 0.9330127018922194093, 0.9330127018922194093 ) ) 
 REPRESENTATION_ITEM ( '' )  );
#21211=CARTESIAN_POINT ( 'NONE',  ( -1.846868145590734756, -143.1250000013656063, -4.458734125000000326 ) ) ;
#21213=ORIENTED_EDGE ( 'NONE', *, *, #37851, .F. ) ;
#21215=CARTESIAN_POINT ( 'NONE',  ( 2.229367062499998831, 26.10416666803225993, -3.861377020970580887 ) ) ;
#21226=DIRECTION ( 'NONE',  ( -0.000000000000000000, 1.000000000000000000, -0.000000000000000000 ) ) ;
#21227=CARTESIAN_POINT ( 'NONE',  ( 4.458734125000001214, -6.895833331967734736, 2.574251347313718519 ) ) ;
#21229=CARTESIAN_POINT ( 'NONE',  ( 1.846868145590735200, -150.2500000013656347, -4.458734124999999437 ) ) ;
#21231=ORIENTED_EDGE ( 'NONE', *, *, #36622, .F. ) ;
#21232=CARTESIAN_POINT ( 'NONE',  ( -5.000000000000000000, -62.87499999726880873, 0.000000000000000000 ) ) ;
#21233=CARTESIAN_POINT ( 'NONE',  ( -6.972266317189433020E-16, 26.87500000273118417, -5.000000000000000000 ) ) ;
#21235=CARTESIAN_POINT ( 'NONE',  ( 2.500000000000002220, -85.54166666393547303, 4.330127018922192761 ) ) ;
#21236=CARTESIAN_POINT ( 'NONE',  ( -2.500000000000000444, -6.166666666666667851, -4.330127018922193649 ) ) ;
#21243=CARTESIAN_POINT ( 'NONE',  ( 4.458734125000000326, 11.10416666803225993, 2.574251347313718519 ) ) ;
#21245=CARTESIAN_POINT ( 'NONE',  ( -2.229367062500000163, -12.72916666530107044, -3.861377020970580443 ) ) ;
#21247=CARTESIAN_POINT ( 'NONE',  ( -1.846868145590737420, -164.7500000013656063, 4.458734124999999437 ) ) ;
#21251=EDGE_CURVE ( 'NONE', #11078, #58699, #21474, .T. ) ;
#21253=CARTESIAN_POINT ( 'NONE',  ( -9.184850993605147944E-16, -165.3750000027312126, 5.000000000000000000 ) ) ;
#21254=CARTESIAN_POINT ( 'NONE',  ( 5.000000000000000000, -139.1875000027312126, 2.071067811865478614 ) ) ;
#21255=CARTESIAN_POINT ( 'NONE',  ( -2.229367062499996610, -34.14583333196772941, 3.861377020970582219 ) ) ;
#21262=( BOUNDED_CURVE ( )  B_SPLINE_CURVE ( 2, ( #20767, #5650, #24307, #54541, #43912, #33961, #15622, #49062, #14340 ),
 .UNSPECIFIED., .F., .F. ) 
 B_SPLINE_CURVE_WITH_KNOTS ( ( 3, 2, 2, 2, 3 ),
 ( 0.06458333333333333981, 0.06527777777777778179, 0.06666666666666666574, 0.06805555555555554970, 0.06875000000000000555 ),
 .UNSPECIFIED. ) 
 CURVE ( )  GEOMETRIC_REPRESENTATION_ITEM ( )  RATIONAL_B_SPLINE_CURVE ( ( 0.9330127018922194093, 0.9330127018922200755, 1.000000000000000000, 0.8660254037844387076, 1.000000000000000000, 0.8660254037844387076, 1.000000000000000000, 0.9330127018922187432, 0.9330127018922194093 ) ) 
 REPRESENTATION_ITEM ( '' )  );
#21265=CARTESIAN_POINT ( 'NONE',  ( -3.535250795749689387E-16, -6.249999999999998224, -5.773502691896257311 ) ) ;
#21266=CARTESIAN_POINT ( 'NONE',  ( -2.229367062500000163, -73.47916666530106511, -3.861377020970580443 ) ) ;
#21268=LINE ( 'NONE', #40873, #5136 ) ;
#21269=CARTESIAN_POINT ( 'NONE',  ( 5.000000000000000000, -5.374999997268811391, -6.123233995736766282E-16 ) ) ;
#21270=CARTESIAN_POINT ( 'NONE',  ( -2.229367062500000163, -37.47916666530107221, -3.861377020970580443 ) ) ;
#21271=ORIENTED_EDGE ( 'NONE', *, *, #6302, .T. ) ;
#21273=CARTESIAN_POINT ( 'NONE',  ( 4.458734125000001214, 9.854166668032263487, 2.574251347313718519 ) ) ;
#21276=CARTESIAN_POINT ( 'NONE',  ( -2.499999999999996447, -48.83333333333332860, 4.330127018922195425 ) ) ;
#21278=CARTESIAN_POINT ( 'NONE',  ( -5.000000000000000000, 14.12500000273118594, 0.000000000000000000 ) ) ;
#21279=CARTESIAN_POINT ( 'NONE',  ( -4.458734124999998549, -77.22916666530106511, 2.574251347313722516 ) ) ;
#21280=CARTESIAN_POINT ( 'NONE',  ( -3.152801135295367985, -140.0625000013655779, 3.152801135295367096 ) ) ;
#21281=CARTESIAN_POINT ( 'NONE',  ( 9.457646018065525792E-16, -87.06249999863440792, 5.148502694627439702 ) ) ;
#21283=CARTESIAN_POINT ( 'NONE',  ( -3.152548672688508926E-16, -37.81249999863440792, -5.148502694627439702 ) ) ;
#21284=EDGE_CURVE ( 'NONE', #23096, #46264, #34587, .T. ) ;
#21290=EDGE_CURVE ( 'NONE', #61986, #56964, #30899, .T. ) ;
#21291=ORIENTED_EDGE ( 'NONE', *, *, #39010, .T. ) ;
#21292=CARTESIAN_POINT ( 'NONE',  ( -1.339745962155660663, -3.669658196007337558, 4.999999999999972466 ) ) ;
#21294=DIRECTION ( 'NONE',  ( -0.000000000000000000, 1.000000000000000000, -0.000000000000000000 ) ) ;
#21295=CARTESIAN_POINT ( 'NONE',  ( -4.458734124999998549, -65.47916666530107932, 2.574251347313722516 ) ) ;
#21297=VERTEX_POINT ( 'NONE', #54396 ) ;
#21299=CARTESIAN_POINT ( 'NONE',  ( -5.000000000000000000, 5.041666669397853795, -2.886751345948128211 ) ) ;
#21300=ORIENTED_EDGE ( 'NONE', *, *, #6436, .F. ) ;
#21304=CARTESIAN_POINT ( 'NONE',  ( 2.229367062500001939, 10.02083333469892779, 3.861377020970579999 ) ) ;
#21305=CARTESIAN_POINT ( 'NONE',  ( -3.152801135295367096, -163.0625000013656063, -3.152801135295367541 ) ) ;
#21313=VECTOR ( 'NONE', #48219, 1000.000000000000000 ) ;
#21314=CARTESIAN_POINT ( 'NONE',  ( 2.499999999999998668, 25.79166666939785202, -4.330127018922193649 ) ) ;
#21318=CARTESIAN_POINT ( 'NONE',  ( -1.339745962155610925, -28.79465819873852084, 5.000000000000000000 ) ) ;
#21320=CARTESIAN_POINT ( 'NONE',  ( -6.972266317189433020E-16, -0.1249999972688142225, -5.000000000000000000 ) ) ;
#21321=CARTESIAN_POINT ( 'NONE',  ( 4.458734125000000326, 26.10416666803225993, 2.574251347313718519 ) ) ;
#21324=CARTESIAN_POINT ( 'NONE',  ( -2.229367062500000163, 0.2708333346989263979, -3.861377020970580443 ) ) ;
#21325=CARTESIAN_POINT ( 'NONE',  ( -3.535533905932737309, -149.7500000027312126, -3.535533905932738197 ) ) ;
#21327=CARTESIAN_POINT ( 'NONE',  ( -3.535533905932738641, -145.5000000027311842, 3.535533905932737309 ) ) ;
#21328=CARTESIAN_POINT ( 'NONE',  ( 3.061616997868383141E-16, -158.7500000000000000, -5.000000000000000000 ) ) ;
#21332=CARTESIAN_POINT ( 'NONE',  ( -5.000000000000000000, -140.5000000000000000, -6.123233995736766282E-16 ) ) ;
#21333=CARTESIAN_POINT ( 'NONE',  ( 1.975475456537005874E-15, -88.74999999999998579, 5.000000000000000000 ) ) ;
#21335=CARTESIAN_POINT ( 'NONE',  ( -4.458734125000000326, -163.1250000013656347, 1.846868145590734089 ) ) ;
#21338=CARTESIAN_POINT ( 'NONE',  ( -4.458734124999999437, -139.9375000013656063, -5.460374474430324690E-16 ) ) ;
#21339=EDGE_LOOP ( 'NONE', ( #13889, #33305, #29804, #17942 ) ) ;
#21340=CARTESIAN_POINT ( 'NONE',  ( -4.458734124999999437, 24.43750000136559208, 0.000000000000000000 ) ) ;
#21345=CARTESIAN_POINT ( 'NONE',  ( 5.000000000000000000, 11.50000000000000000, -6.123233995736766282E-16 ) ) ;
#21346=CARTESIAN_POINT ( 'NONE',  ( 2.229367062499998831, -53.64583333196773651, -3.861377020970580887 ) ) ;
#21347=CARTESIAN_POINT ( 'NONE',  ( -2.229367062500000163, -11.47916666530107044, -3.861377020970580443 ) ) ;
#21348=CARTESIAN_POINT ( 'NONE',  ( 3.061616997868383141E-16, -165.8750000027312126, -5.000000000000000000 ) ) ;
#21351=CARTESIAN_POINT ( 'NONE',  ( -5.000000000000000000, -64.08333333333332860, -2.886751345948128211 ) ) ;
#21353=CARTESIAN_POINT ( 'NONE',  ( 2.499999999999998668, -36.33333333333332860, -4.330127018922193649 ) ) ;
#21355=LINE ( 'NONE', #10743, #44950 ) ;
#21358=CARTESIAN_POINT ( 'NONE',  ( -2.500000000000000444, -32.04166666393548724, -4.330127018922193649 ) ) ;
#21359=CARTESIAN_POINT ( 'NONE',  ( 4.458734124999999437, -57.81249999863440081, -5.460374474430324690E-16 ) ) ;
#21360=CARTESIAN_POINT ( 'NONE',  ( 3.152801135295366208, -150.8125000013655779, 3.152801135295367985 ) ) ;
#21361=CARTESIAN_POINT ( 'NONE',  ( -4.458734124999999437, -72.31249999863439371, 0.000000000000000000 ) ) ;
#21364=CARTESIAN_POINT ( 'NONE',  ( 5.000000000000000888, -59.45833333060214443, 2.886751345948126879 ) ) ;
#21368=DIRECTION ( 'NONE',  ( -0.000000000000000000, 1.000000000000000000, -0.000000000000000000 ) ) ;
#21370=CARTESIAN_POINT ( 'NONE',  ( 4.458734124999999437, -151.4375000013655779, 0.000000000000000000 ) ) ;
#21371=ORIENTED_EDGE ( 'NONE', *, *, #2715, .F. ) ;
#21375=CARTESIAN_POINT ( 'NONE',  ( 4.458734124999999437, -50.06249999863440792, -5.460374474430324690E-16 ) ) ;
#21380=CARTESIAN_POINT ( 'NONE',  ( -3.152548672688508926E-16, 24.43750000136559564, -5.148502694627439702 ) ) ;
#21382=CARTESIAN_POINT ( 'NONE',  ( 2.500000000000002220, -13.54166666393548013, 4.330127018922192761 ) ) ;
#21383=CARTESIAN_POINT ( 'NONE',  ( -6.972266317189433020E-16, -61.12499999726880162, -5.000000000000000000 ) ) ;
#21384=ORIENTED_EDGE ( 'NONE', *, *, #39262, .T. ) ;
#21389=( BOUNDED_CURVE ( )  B_SPLINE_CURVE ( 2, ( #1376, #24838, #59906, #48948, #44761, #59580, #15514, #25467, #4897 ),
 .UNSPECIFIED., .F., .F. ) 
 B_SPLINE_CURVE_WITH_KNOTS ( ( 3, 2, 2, 2, 3 ),
 ( 0.6770833333333333703, 0.6777777777777778123, 0.6791666666666666963, 0.6805555555555555802, 0.6812500000000000222 ),
 .UNSPECIFIED. ) 
 CURVE ( )  GEOMETRIC_REPRESENTATION_ITEM ( )  RATIONAL_B_SPLINE_CURVE ( ( 0.9330127018922194093, 0.9330127018922194093, 1.000000000000000000, 0.8660254037844387076, 1.000000000000000000, 0.8660254037844387076, 1.000000000000000000, 0.9330127018922194093, 0.9330127018922194093 ) ) 
 REPRESENTATION_ITEM ( '' )  );
#21390=CARTESIAN_POINT ( 'NONE',  ( -6.972266317189433020E-16, -63.25000000000000000, -5.000000000000000000 ) ) ;
#21392=CARTESIAN_POINT ( 'NONE',  ( -5.000000000000000888, -157.4375000000000000, 2.071067811865474617 ) ) ;
#21397=DIRECTION ( 'NONE',  ( 0.000000000000000000, 0.000000000000000000, 1.000000000000000000 ) ) ;
#21399=ORIENTED_EDGE ( 'NONE', *, *, #8292, .T. ) ;
#21403=CARTESIAN_POINT ( 'NONE',  ( 5.000000000000000000, -159.1250000027311842, 0.000000000000000000 ) ) ;
#21404=ORIENTED_EDGE ( 'NONE', *, *, #18453, .T. ) ;
#21406=VECTOR ( 'NONE', #3463, 1000.000000000000000 ) ;
#21414=CARTESIAN_POINT ( 'NONE',  ( -3.152548672688508926E-16, -19.56249999863440081, -5.148502694627439702 ) ) ;
#21416=CARTESIAN_POINT ( 'NONE',  ( 3.535533905932738197, -151.8750000000000000, -3.535533905932738197 ) ) ;
#21418=CARTESIAN_POINT ( 'NONE',  ( 4.458734125000000326, -153.3750000013656347, -1.846868145590734978 ) ) ;
#21419=ORIENTED_EDGE ( 'NONE', *, *, #58890, .T. ) ;
#21420=CARTESIAN_POINT ( 'NONE',  ( 9.457646018065525792E-16, -51.31249999863440792, 5.148502694627439702 ) ) ;
#21423=CARTESIAN_POINT ( 'NONE',  ( -2.229367062500000163, -89.47916666530106511, -3.861377020970580443 ) ) ;
#21424=AXIS2_PLACEMENT_3D ( 'NONE', #39083, #28495, #19789 ) ;
#21425=CARTESIAN_POINT ( 'NONE',  ( 2.229367062500001939, 2.020833334698927786, 3.861377020970579999 ) ) ;
#21427=CARTESIAN_POINT ( 'NONE',  ( 1.339745962155612702, -17.29465819873852084, -5.000000000000000000 ) ) ;
#21428=CARTESIAN_POINT ( 'NONE',  ( 4.458734125000001214, 14.85416666803225993, 2.574251347313718519 ) ) ;
#21429=CARTESIAN_POINT ( 'NONE',  ( 1.060575238724906964E-15, 2.375000002731185500, 5.773502691896257311 ) ) ;
#21431=CARTESIAN_POINT ( 'NONE',  ( -1.339745962155613812, 7.794658198738521726, -5.000000000000000000 ) ) ;
#21432=ORIENTED_EDGE ( 'NONE', *, *, #38998, .T. ) ;
#21434=CARTESIAN_POINT ( 'NONE',  ( 2.229367062500001939, -45.97916666530106511, 3.861377020970579999 ) ) ;
#21435=CARTESIAN_POINT ( 'NONE',  ( -3.152801135295367985, -164.0625000013656063, 3.152801135295367096 ) ) ;
#21436=EDGE_CURVE ( 'NONE', #28232, #8173, #56551, .T. ) ;
#21437=CARTESIAN_POINT ( 'NONE',  ( -2.500000000000000444, -40.04166666393548013, -4.330127018922193649 ) ) ;
#21438=ORIENTED_EDGE ( 'NONE', *, *, #63327, .F. ) ;
#21439=CARTESIAN_POINT ( 'NONE',  ( -2.229367062500000163, -16.47916666530107577, -3.861377020970580443 ) ) ;
#21443=CARTESIAN_POINT ( 'NONE',  ( -3.152801135295367096, -164.0625000013656063, -3.152801135295367541 ) ) ;
#21444=( BOUNDED_CURVE ( )  B_SPLINE_CURVE ( 2, ( #18807, #13680, #13369, #42315, #61955 ),
 .UNSPECIFIED., .F., .F. ) 
 B_SPLINE_CURVE_WITH_KNOTS ( ( 3, 2, 3 ),
 ( 0.000000000000000000, 0.004166666666666670078, 0.008333333333333340157 ),
 .UNSPECIFIED. ) 
 CURVE ( )  GEOMETRIC_REPRESENTATION_ITEM ( )  RATIONAL_B_SPLINE_CURVE ( ( 1.000000000000000000, 0.9238795325112867385, 1.000000000000000000, 0.9238795325112866275, 1.000000000000000222 ) ) 
 REPRESENTATION_ITEM ( '' )  );
#21446=CARTESIAN_POINT ( 'NONE',  ( -5.000000000000000000, -84.95833333060215864, -2.886751345948128211 ) ) ;
#21447=CARTESIAN_POINT ( 'NONE',  ( -6.972266317189433020E-16, -61.12499999726880162, -5.000000000000000000 ) ) ;
#21450=AXIS2_PLACEMENT_3D ( 'NONE', #56730, #21993, #8465 ) ;
#21451=CARTESIAN_POINT ( 'NONE',  ( -4.458734124999998549, -31.47916666530107221, 2.574251347313722516 ) ) ;
#21452=CARTESIAN_POINT ( 'NONE',  ( -1.339745962155613812, 19.91965820146970501, -5.000000000000000000 ) ) ;
#21453=ORIENTED_EDGE ( 'NONE', *, *, #22568, .T. ) ;
#21456=CARTESIAN_POINT ( 'NONE',  ( -1.127183054612291972E-14, 24.37500000273118417, 4.999999999999999112 ) ) ;
#21460=CARTESIAN_POINT ( 'NONE',  ( -2.229367062499996610, -82.39583333196773651, 3.861377020970582219 ) ) ;
#21463=CARTESIAN_POINT ( 'NONE',  ( 1.846868145590736310, -142.8750000013656063, 4.458734124999997661 ) ) ;
#21464=CARTESIAN_POINT ( 'NONE',  ( -9.184850993605147944E-16, -145.3750000027312126, 5.000000000000000000 ) ) ;
#21466=CARTESIAN_POINT ( 'NONE',  ( -4.458734124999999437, -46.39583333196774362, -2.574251347313719407 ) ) ;
#21469=CARTESIAN_POINT ( 'NONE',  ( -6.972266317189433020E-16, 18.74999999999999645, -5.000000000000000000 ) ) ;
#21474=( BOUNDED_CURVE ( )  B_SPLINE_CURVE ( 2, ( #38947, #34434, #10324, #59544, #5187, #6469, #16106, #54062, #24803 ),
 .UNSPECIFIED., .F., .F. ) 
 B_SPLINE_CURVE_WITH_KNOTS ( ( 3, 2, 2, 2, 3 ),
 ( 0.5687499999999999778, 0.5694444444444444198, 0.5708333333333333037, 0.5722222222222221877, 0.5729166666666666297 ),
 .UNSPECIFIED. ) 
 CURVE ( )  GEOMETRIC_REPRESENTATION_ITEM ( )  RATIONAL_B_SPLINE_CURVE ( ( 0.9330127018922194093, 0.9330127018922194093, 1.000000000000000000, 0.8660254037844387076, 1.000000000000000000, 0.8660254037844387076, 1.000000000000000000, 0.9330127018922194093, 0.9330127018922194093 ) ) 
 REPRESENTATION_ITEM ( '' )  );
#21475=CARTESIAN_POINT ( 'NONE',  ( 4.458734124999998549, -80.97916666530106511, -2.574251347313721627 ) ) ;
#21478=FACE_OUTER_BOUND ( 'NONE', #880, .T. ) ;
#21481=CARTESIAN_POINT ( 'NONE',  ( 0.000000000000000000, -170.0000000000000000, 5.000000000000000000 ) ) ;
#21482=CARTESIAN_POINT ( 'NONE',  ( 2.500000000000002220, -47.66666666666666430, 4.330127018922192761 ) ) ;
#21484=CARTESIAN_POINT ( 'NONE',  ( -3.535533905932737309, -167.7500000027312126, -3.535533905932738197 ) ) ;
#21486=CARTESIAN_POINT ( 'NONE',  ( -4.458734124999999437, 14.35416666803226171, -2.574251347313719407 ) ) ;
#21487=CARTESIAN_POINT ( 'NONE',  ( 5.000000000000000000, -77.37499999726881583, -6.123233995736766282E-16 ) ) ;
#21493=CARTESIAN_POINT ( 'NONE',  ( -4.458734124999999437, -84.39583333196773651, -2.574251347313719407 ) ) ;
#21494=CARTESIAN_POINT ( 'NONE',  ( -4.458734124999997661, -2.229166665301068662, 2.574251347313722516 ) ) ;
#21497=CARTESIAN_POINT ( 'NONE',  ( -4.458734124999997661, -28.47916666530107221, 2.574251347313722516 ) ) ;
#21504=AXIS2_PLACEMENT_3D ( 'NONE', #1220, #34976, #45254 ) ;
#21505=CARTESIAN_POINT ( 'NONE',  ( 4.458734125000001214, 21.10416666803226349, 2.574251347313718519 ) ) ;
#21506=CARTESIAN_POINT ( 'NONE',  ( -5.000000000000000000, -43.95833333060214443, -2.886751345948128211 ) ) ;
#21507=CARTESIAN_POINT ( 'NONE',  ( 4.458734124999999437, -77.06249999863440792, -5.460374474430324690E-16 ) ) ;
#21510=CARTESIAN_POINT ( 'NONE',  ( -3.535250795749689387E-16, 23.87500000273118417, -5.773502691896257311 ) ) ;
#21511=VERTEX_POINT ( 'NONE', #27573 ) ;
#21514=CARTESIAN_POINT ( 'NONE',  ( 2.500000000000002220, -0.6666666666666660745, 4.330127018922192761 ) ) ;
#21515=CARTESIAN_POINT ( 'NONE',  ( -3.535250795749689387E-16, -21.24999999999999645, -5.773502691896257311 ) ) ;
#21516=CARTESIAN_POINT ( 'NONE',  ( 2.229367062500001939, -26.97916666530106866, 3.861377020970579999 ) ) ;
#21517=CARTESIAN_POINT ( 'NONE',  ( 2.229367062499998831, -87.64583333196773651, -3.861377020970580887 ) ) ;
#21518=CARTESIAN_POINT ( 'NONE',  ( 5.000000000000000000, -25.37499999726881583, -6.123233995736766282E-16 ) ) ;
#21519=CARTESIAN_POINT ( 'NONE',  ( -3.152548672688508926E-16, -54.56249999863439371, -5.148502694627439702 ) ) ;
#21521=DIRECTION ( 'NONE',  ( -0.000000000000000000, 1.000000000000000000, -0.000000000000000000 ) ) ;
#21523=CARTESIAN_POINT ( 'NONE',  ( 4.458734124999999437, -2.062499998634406584, -5.460374474430324690E-16 ) ) ;
#21524=VERTEX_POINT ( 'NONE', #61375 ) ;
#21525=CARTESIAN_POINT ( 'NONE',  ( 5.000000000000000000, -72.50000000000000000, -6.123233995736766282E-16 ) ) ;
#21529=CARTESIAN_POINT ( 'NONE',  ( 2.071067811865476394, -160.1875000000000000, 5.000000000000000000 ) ) ;
#21530=CARTESIAN_POINT ( 'NONE',  ( -5.000000000000000000, -70.95833333060214443, -2.886751345948128211 ) ) ;
#21533=CARTESIAN_POINT ( 'NONE',  ( -2.229367062499996610, -15.39583333196773651, 3.861377020970582219 ) ) ;
#21534=CARTESIAN_POINT ( 'NONE',  ( -3.152548672688508926E-16, -52.81249999863440792, -5.148502694627439702 ) ) ;
#21535=CARTESIAN_POINT ( 'NONE',  ( 1.975475456537005874E-15, -65.62499999726881583, 5.000000000000000000 ) ) ;
#21537=CARTESIAN_POINT ( 'NONE',  ( -1.846868145590734756, -145.1250000013655779, -4.458734125000000326 ) ) ;
#21541=CARTESIAN_POINT ( 'NONE',  ( -3.535533905932738641, -155.3750000000000000, 3.535533905932737309 ) ) ;
#21542=CARTESIAN_POINT ( 'NONE',  ( 9.457646018065525792E-16, 26.68750000136559564, 5.148502694627439702 ) ) ;
#21547=CARTESIAN_POINT ( 'NONE',  ( 2.730187237215162345E-16, -149.4375000013656063, -4.458734124999999437 ) ) ;
#21549=CARTESIAN_POINT ( 'NONE',  ( 4.458734125000001214, -65.14583333196773651, 2.574251347313718519 ) ) ;
#21550=CARTESIAN_POINT ( 'NONE',  ( -5.000000000000000000, -83.87499999726880162, 0.000000000000000000 ) ) ;
#21551=CARTESIAN_POINT ( 'NONE',  ( -4.458734124999998549, -9.229166665301068662, 2.574251347313722516 ) ) ;
#21552=CARTESIAN_POINT ( 'NONE',  ( 2.500000000000002220, 6.458333336064519870, 4.330127018922192761 ) ) ;
#21553=CARTESIAN_POINT ( 'NONE',  ( -1.846868145590734756, -144.1250000013655779, -4.458734124999999437 ) ) ;
#21556=CARTESIAN_POINT ( 'NONE',  ( 0.000000000000000000, -170.0000000000000000, 0.000000000000000000 ) ) ;
#21567=CARTESIAN_POINT ( 'NONE',  ( -6.972266317189433020E-16, -15.25000000000000000, -5.000000000000000000 ) ) ;
#21568=CARTESIAN_POINT ( 'NONE',  ( -4.458734124999999437, 12.60416666803226349, -2.574251347313719407 ) ) ;
#21570=CARTESIAN_POINT ( 'NONE',  ( 4.458734124999999437, -15.06249999863440436, -5.460374474430324690E-16 ) ) ;
#21572=CARTESIAN_POINT ( 'NONE',  ( 1.846868145590735200, -162.2500000013656347, -4.458734125000000326 ) ) ;
#21575=EDGE_CURVE ( 'NONE', #7616, #1762, #10754, .T. ) ;
#21576=( BOUNDED_CURVE ( )  B_SPLINE_CURVE ( 2, ( #23264, #18432, #63137, #48635, #57989, #48323, #38053, #4574, #43805 ),
 .UNSPECIFIED., .F., .F. ) 
 B_SPLINE_CURVE_WITH_KNOTS ( ( 3, 2, 2, 2, 3 ),
 ( 0.5416666666666671848, 0.5458333333333338366, 0.5500000000000004885, 0.5541666666666671404, 0.5583333333333337922 ),
 .UNSPECIFIED. ) 
 CURVE ( )  GEOMETRIC_REPRESENTATION_ITEM ( )  RATIONAL_B_SPLINE_CURVE ( ( 0.9999999999999898970, 0.9238795325112968415, 1.000000000000000000, 0.9238795325112867385, 1.000000000000000000, 0.9238795325112867385, 1.000000000000000000, 0.9238795325112786339, 1.000000000000008216 ) ) 
 REPRESENTATION_ITEM ( '' )  );
#21577=CARTESIAN_POINT ( 'NONE',  ( -1.339745962155613812, -28.20534180126147916, -5.000000000000000000 ) ) ;
#21578=CARTESIAN_POINT ( 'NONE',  ( -5.000000000000000000, -88.95833333060214443, -2.886751345948128211 ) ) ;
#21579=CARTESIAN_POINT ( 'NONE',  ( -3.152548672688508926E-16, -34.56249999863440792, -5.148502694627439702 ) ) ;
#21580=CARTESIAN_POINT ( 'NONE',  ( 5.000000000000000888, -60.58333333333332860, 2.886751345948126879 ) ) ;
#21582=CARTESIAN_POINT ( 'NONE',  ( 6.123233995736766282E-16, -170.0000000000000000, -5.000000000000000000 ) ) ;
#21587=CARTESIAN_POINT ( 'NONE',  ( 5.000000000000000000, -89.29166666393547303, -2.886751345948130876 ) ) ;
#21588=CARTESIAN_POINT ( 'NONE',  ( -3.535250795749689387E-16, -8.250000000000000000, -5.773502691896257311 ) ) ;
#21590=CARTESIAN_POINT ( 'NONE',  ( 9.457646018065525792E-16, -74.06249999863440792, 5.148502694627439702 ) ) ;
#21592=DIRECTION ( 'NONE',  ( 0.000000000000000000, 0.000000000000000000, 1.000000000000000000 ) ) ;
#21594=CARTESIAN_POINT ( 'NONE',  ( -2.499999999999996447, -9.708333330602146205, 4.330127018922195425 ) ) ;
#21595=CARTESIAN_POINT ( 'NONE',  ( 2.229367062499998831, -40.64583333196773651, -3.861377020970580887 ) ) ;
#21596=ORIENTED_EDGE ( 'NONE', *, *, #62196, .T. ) ;
#21599=CARTESIAN_POINT ( 'NONE',  ( 4.458734124999999437, 13.93750000136559386, -5.460374474430324690E-16 ) ) ;
#21600=ORIENTED_EDGE ( 'NONE', *, *, #16225, .T. ) ;
#21602=CARTESIAN_POINT ( 'NONE',  ( -4.999999999999999112, -54.91666666666667140, 2.886751345948131764 ) ) ;
#21605=CARTESIAN_POINT ( 'NONE',  ( 4.458734124999999437, -75.81249999863440792, -5.460374474430324690E-16 ) ) ;
#21606=CARTESIAN_POINT ( 'NONE',  ( 4.458734125000000326, -140.6250000013656063, -1.846868145590734978 ) ) ;
#21607=CARTESIAN_POINT ( 'NONE',  ( 4.458734125000001214, -86.89583333196773651, 2.574251347313718519 ) ) ;
#21610=CARTESIAN_POINT ( 'NONE',  ( -3.152548672688508926E-16, -33.81249999863440792, -5.148502694627439702 ) ) ;
#21611=CARTESIAN_POINT ( 'NONE',  ( 5.000000000000000000, -16.37499999726881228, -6.123233995736766282E-16 ) ) ;
#21614=CARTESIAN_POINT ( 'NONE',  ( -5.000000000000000000, 22.04166666939785202, -2.886751345948128211 ) ) ;
#21616=CARTESIAN_POINT ( 'NONE',  ( -1.049326080737009628E-13, -3.624999997268818053, 5.000000000000000000 ) ) ;
#21617=CARTESIAN_POINT ( 'NONE',  ( -2.499999999999996447, -11.70833333060214798, 4.330127018922195425 ) ) ;
#21618=CARTESIAN_POINT ( 'NONE',  ( 4.458734124999999437, -66.06249999863440792, -5.460374474430324690E-16 ) ) ;
#21623=VERTEX_POINT ( 'NONE', #23075 ) ;
#21626=CARTESIAN_POINT ( 'NONE',  ( 2.229367062500001939, 8.020833334698926009, 3.861377020970579999 ) ) ;
#21629=CARTESIAN_POINT ( 'NONE',  ( 1.846868145590735200, -157.2500000013656063, -4.458734124999999437 ) ) ;
#21633=CYLINDRICAL_SURFACE ( 'NONE', #9952, 5.000000000000000000 ) ;
#21635=LINE ( 'NONE', #26134, #40638 ) ;
#21640=CARTESIAN_POINT ( 'NONE',  ( -3.152548672688508926E-16, 29.43750000136559564, -5.148502694627439702 ) ) ;
#21643=CARTESIAN_POINT ( 'NONE',  ( 9.457646018065525792E-16, 2.687500001365593860, 5.148502694627439702 ) ) ;
#21644=( BOUNDED_CURVE ( )  B_SPLINE_CURVE ( 2, ( #35032, #50464, #40159, #55923, #7035, #59802, #30834, #35342, #21828 ),
 .UNSPECIFIED., .F., .F. ) 
 B_SPLINE_CURVE_WITH_KNOTS ( ( 3, 2, 2, 2, 3 ),
 ( 0.2520833333333333259, 0.2527777777777777679, 0.2541666666666666519, 0.2555555555555555358, 0.2562499999999999778 ),
 .UNSPECIFIED. ) 
 CURVE ( )  GEOMETRIC_REPRESENTATION_ITEM ( )  RATIONAL_B_SPLINE_CURVE ( ( 0.9330127018922194093, 0.9330127018922194093, 1.000000000000000000, 0.8660254037844387076, 1.000000000000000000, 0.8660254037844387076, 1.000000000000000000, 0.9330127018922194093, 0.9330127018922194093 ) ) 
 REPRESENTATION_ITEM ( '' )  );
#21647=CARTESIAN_POINT ( 'NONE',  ( 5.000000000000000000, -145.1250000027312126, 0.000000000000000000 ) ) ;
#21648=CARTESIAN_POINT ( 'NONE',  ( 5.000000000000000888, -33.45833333060215153, 2.886751345948126879 ) ) ;
#21653=DIRECTION ( 'NONE',  ( -0.000000000000000000, 1.000000000000000000, -0.000000000000000000 ) ) ;
#21656=EDGE_CURVE ( 'NONE', #21511, #30690, #15386, .T. ) ;
#21658=CARTESIAN_POINT ( 'NONE',  ( 4.458734124999999437, -161.6250000013656063, -1.846868145590734978 ) ) ;
#21659=CARTESIAN_POINT ( 'NONE',  ( 2.499999999999998668, 7.666666666666665186, -4.330127018922193649 ) ) ;
#21661=CARTESIAN_POINT ( 'NONE',  ( 4.458734124999999437, -140.5000000013656347, 1.846868145590737864 ) ) ;
#21663=CARTESIAN_POINT ( 'NONE',  ( 4.458734124999999437, 21.93750000136559208, -5.460374474430324690E-16 ) ) ;
#21669=CARTESIAN_POINT ( 'NONE',  ( -5.000000000000000000, 7.916666666666665186, -2.886751345948128211 ) ) ;
#21671=CARTESIAN_POINT ( 'NONE',  ( -4.458734124999999437, -58.39583333196773651, -2.574251347313719407 ) ) ;
#21672=CARTESIAN_POINT ( 'NONE',  ( 4.458734125000001214, -10.89583333196773651, 2.574251347313718519 ) ) ;
#21678=CARTESIAN_POINT ( 'NONE',  ( -4.999999999999999112, -40.91666666666667140, 2.886751345948131764 ) ) ;
#21683=CARTESIAN_POINT ( 'NONE',  ( 0.000000000000000000, -170.0000000000000000, 0.000000000000000000 ) ) ;
#21684=CARTESIAN_POINT ( 'NONE',  ( 4.458734125000001214, -60.89583333196774362, 2.574251347313718519 ) ) ;
#21685=CARTESIAN_POINT ( 'NONE',  ( -4.458734125000000326, -153.2500000013655779, -1.846868145590735644 ) ) ;
#21686=CARTESIAN_POINT ( 'NONE',  ( -3.152548672688508926E-16, -69.56249999863439371, -5.148502694627439702 ) ) ;
#21688=CARTESIAN_POINT ( 'NONE',  ( -4.458734124999998549, -17.47916666530106866, 2.574251347313722516 ) ) ;
#21689=CARTESIAN_POINT ( 'NONE',  ( 2.500000000000002220, -62.54166666393547303, 4.330127018922192761 ) ) ;
#21690=ORIENTED_EDGE ( 'NONE', *, *, #47647, .T. ) ;
#21692=VERTEX_POINT ( 'NONE', #9218 ) ;
#21694=CARTESIAN_POINT ( 'NONE',  ( -9.184850993605147944E-16, -157.3750000027311842, 5.000000000000000000 ) ) ;
#21696=CARTESIAN_POINT ( 'NONE',  ( -1.846868145590737420, -150.7500000013655779, 4.458734124999999437 ) ) ;
#21698=CARTESIAN_POINT ( 'NONE',  ( -6.972266317189433020E-16, -24.12499999726881228, -5.000000000000000000 ) ) ;
#21700=DIRECTION ( 'NONE',  ( 0.000000000000000000, 0.000000000000000000, 1.000000000000000000 ) ) ;
#21701=CARTESIAN_POINT ( 'NONE',  ( 9.457646018065525792E-16, -46.31249999863440792, 5.148502694627439702 ) ) ;
#21705=CARTESIAN_POINT ( 'NONE',  ( 4.458734124999998549, 23.27083333469892423, -2.574251347313721627 ) ) ;
#21711=CARTESIAN_POINT ( 'NONE',  ( 3.061616997868383141E-16, -169.7500000000000000, -5.000000000000000000 ) ) ;
#21717=DIRECTION ( 'NONE',  ( -0.000000000000000000, 1.000000000000000000, -0.000000000000000000 ) ) ;
#21721=EDGE_LOOP ( 'NONE', ( #60147, #13752, #34778, #12468 ) ) ;
#21724=CARTESIAN_POINT ( 'NONE',  ( -5.000000000000000888, -157.6875000027312126, -2.071067811865475949 ) ) ;
#21735=CARTESIAN_POINT ( 'NONE',  ( 4.458734124999998549, -26.72916666530106866, -2.574251347313721627 ) ) ;
#21736=CARTESIAN_POINT ( 'NONE',  ( 2.071067811865560326, -146.8125000000000000, -4.999999999999914735 ) ) ;
#21737=CARTESIAN_POINT ( 'NONE',  ( -2.071067811865475061, -149.6875000000000000, -5.000000000000000888 ) ) ;
#21739=CARTESIAN_POINT ( 'NONE',  ( 2.730187237215162345E-16, -153.1875000013656063, -4.458734124999999437 ) ) ;
#21741=CARTESIAN_POINT ( 'NONE',  ( -4.458734124999999437, -50.64583333196773651, -2.574251347313719407 ) ) ;
#21743=FACE_OUTER_BOUND ( 'NONE', #1375, .T. ) ;
#21744=DIRECTION ( 'NONE',  ( 0.000000000000000000, 0.000000000000000000, 1.000000000000000000 ) ) ;
#21745=CARTESIAN_POINT ( 'NONE',  ( 1.060575238724906964E-15, 25.25000000000000355, 5.773502691896257311 ) ) ;
#21748=CARTESIAN_POINT ( 'NONE',  ( 4.458734124999999437, 3.187500001365594304, -5.460374474430324690E-16 ) ) ;
#21749=CARTESIAN_POINT ( 'NONE',  ( -5.000000000000000000, -142.5000000000000284, -6.123233995736766282E-16 ) ) ;
#21750=CARTESIAN_POINT ( 'NONE',  ( 1.339745962155612702, -41.16965819600732601, -5.000000000000000000 ) ) ;
#21751=DIRECTION ( 'NONE',  ( -0.000000000000000000, 1.000000000000000000, -0.000000000000000000 ) ) ;
#21752=CARTESIAN_POINT ( 'NONE',  ( 2.229367062499998831, 14.10416666803226171, -3.861377020970580887 ) ) ;
#21753=CARTESIAN_POINT ( 'NONE',  ( -2.499999999999996447, 2.291666669397850686, 4.330127018922195425 ) ) ;
#21755=EDGE_LOOP ( 'NONE', ( #59184, #44605, #8780, #57994 ) ) ;
#21757=VERTEX_POINT ( 'NONE', #60351 ) ;
#21759=CARTESIAN_POINT ( 'NONE',  ( -3.152548672688508926E-16, -43.56249999863440081, -5.148502694627439702 ) ) ;
#21761=CARTESIAN_POINT ( 'NONE',  ( 3.152801135295367541, -162.5625000013656063, -3.152801135295367541 ) ) ;
#21763=CARTESIAN_POINT ( 'NONE',  ( 5.000000000000000888, -45.45833333060214443, 2.886751345948126879 ) ) ;
#21765=CARTESIAN_POINT ( 'NONE',  ( -4.458734124999998549, -18.22916666530107221, 2.574251347313722516 ) ) ;
#21766=ORIENTED_EDGE ( 'NONE', *, *, #51519, .T. ) ;
#21767=CARTESIAN_POINT ( 'NONE',  ( -2.499999999999996447, -87.83333333333332860, 4.330127018922195425 ) ) ;
#21768=CARTESIAN_POINT ( 'NONE',  ( 3.152801135295367541, -165.3125000013656063, -3.152801135295367541 ) ) ;
#21769=CARTESIAN_POINT ( 'NONE',  ( -1.339745962155613812, -19.20534180126147916, -5.000000000000000000 ) ) ;
#21772=CARTESIAN_POINT ( 'NONE',  ( -2.229367062500000163, -33.72916666530107221, -3.861377020970580443 ) ) ;
#21773=CARTESIAN_POINT ( 'NONE',  ( -4.999999999999998224, -38.91666666666667140, 2.886751345948131764 ) ) ;
#21774=EDGE_LOOP ( 'NONE', ( #15112, #52162, #44595, #56960, #61007, #10595, #60510, #13627, #8705, #31538, #47624, #12358, #11775, #53630, #23620, #7564, #12349, #26578, #55307, #3402, #23891, #39737, #55894, #36228, #1704, #20886, #56037, #386, #17945, #49234, #36066, #5040, #4176, #12023, #48801, #3716, #61857, #5123, #11771, #5217, #31646, #38879, #43155, #24301, #22326, #36793, #35753, #20711, #23168, #4736, #17738, #6714, #51977, #8711, #41595, #27514, #37494, #30758, #18655, #60589, #15671, #2421, #39830, #33175, #53735, #44346, #2121, #8757, #37580, #56774, #40653, #13117, #43501, #5272, #60591, #54826, #18166, #56609, #49268, #20604, #60116, #18437, #10758, #12103, #15125, #7063, #53624, #37674, #8943, #50885, #32759, #24569, #45239, #24056, #35776, #35819, #39770, #27535, #8614, #50649, #25956, #63361, #41349, #51984, #47049, #9791, #6117, #43873, #25083, #41411, #23972, #13452, #58809, #61083, #3656, #56338, #15693, #31334, #28904, #34400, #37576, #46922, #2108, #843, #11449, #54101, #11698, #47322, #39546, #22552, #20090, #5939, #16153, #38851, #29156, #12739, #19186, #2406, #4189, #43021, #35557, #41094, #8197, #37543, #33055, #45736, #7400, #5764, #9900, #1030, #26571, #109, #8090, #22088, #60055, #19368, #8133, #28222, #63205, #33099, #12501, #20462, #54356, #3974, #44426, #6417, #48619, #40041, #35786, #1600, #19492, #33675, #9644, #40177, #1982, #48720, #55846, #57168, #17278, #20713, #56805, #705, #56000, #35400, #36414, #19979, #28517, #46295, #45562, #42139, #22993, #53177, #11437, #55855, #22801, #4506, #37492, #18433, #47080, #13515, #60370, #40664, #16646, #42702, #5554, #38982, #4041, #39384, #41604, #15344, #20662, #29604, #3965, #30434, #46666, #63573, #56812, #56368, #38458, #25077, #34167, #8790, #54259, #14061, #53294, #46418, #1954, #19520, #1283, #53223, #54509, #48906, #58865, #31323, #35430, #620, #15985, #57058, #61630, #34534, #31070, #46585, #52692, #22494 ) ) ;
#21779=ORIENTED_EDGE ( 'NONE', *, *, #22892, .F. ) ;
#21782=CARTESIAN_POINT ( 'NONE',  ( 2.229367062500001939, -80.22916666530106511, 3.861377020970579999 ) ) ;
#21784=CARTESIAN_POINT ( 'NONE',  ( -9.184850993605147944E-16, -143.2500000000000284, 5.000000000000000000 ) ) ;
#21785=CARTESIAN_POINT ( 'NONE',  ( -3.152801135295367985, -142.0625000013655779, 3.152801135295367096 ) ) ;
#21787=CARTESIAN_POINT ( 'NONE',  ( -2.229367062499996610, -47.14583333196774362, 3.861377020970582219 ) ) ;
#21790=CARTESIAN_POINT ( 'NONE',  ( 1.975475456537005874E-15, 16.37500000273118417, 5.000000000000000000 ) ) ;
#21793=CARTESIAN_POINT ( 'NONE',  ( 3.061616997868383141E-16, -153.8750000027311842, -5.000000000000000000 ) ) ;
#21795=CARTESIAN_POINT ( 'NONE',  ( -4.458734124999999437, -78.64583333196773651, -2.574251347313719407 ) ) ;
#21800=DIRECTION ( 'NONE',  ( 0.000000000000000000, 0.000000000000000000, 1.000000000000000000 ) ) ;
#21803=CARTESIAN_POINT ( 'NONE',  ( -5.000000000000000888, -168.6875000027311842, -2.071067811865475949 ) ) ;
#21805=CARTESIAN_POINT ( 'NONE',  ( 4.458734124999999437, 13.93750000136559386, -5.460374474430324690E-16 ) ) ;
#21812=CARTESIAN_POINT ( 'NONE',  ( -4.458734124999999437, -87.39583333196773651, -2.574251347313719407 ) ) ;
#21813=CARTESIAN_POINT ( 'NONE',  ( 4.458734125000000326, -8.895833331967736513, 2.574251347313718519 ) ) ;
#21815=CARTESIAN_POINT ( 'NONE',  ( -4.458734124999997661, -36.47916666530107221, 2.574251347313722516 ) ) ;
#21819=CARTESIAN_POINT ( 'NONE',  ( -2.229367062499996610, 17.85416666803225993, 3.861377020970582219 ) ) ;
#21821=FACE_OUTER_BOUND ( 'NONE', #24746, .T. ) ;
#21822=CARTESIAN_POINT ( 'NONE',  ( -4.458734124999999437, -83.56249999863439371, 0.000000000000000000 ) ) ;
#21826=CARTESIAN_POINT ( 'NONE',  ( 5.000000000000000000, 17.62500000273118417, -6.123233995736766282E-16 ) ) ;
#21828=CARTESIAN_POINT ( 'NONE',  ( 1.975475456537005874E-15, -1.624999997268813834, 5.000000000000000000 ) ) ;
#21829=( BOUNDED_CURVE ( )  B_SPLINE_CURVE ( 2, ( #62321, #55993, #50842, #13107, #11907, #6784, #26393, #27891, #42680 ),
 .UNSPECIFIED., .F., .F. ) 
 B_SPLINE_CURVE_WITH_KNOTS ( ( 3, 2, 2, 2, 3 ),
 ( 0.1645833333333333315, 0.1652777777777777735, 0.1666666666666666574, 0.1680555555555555691, 0.1687500000000000111 ),
 .UNSPECIFIED. ) 
 CURVE ( )  GEOMETRIC_REPRESENTATION_ITEM ( )  RATIONAL_B_SPLINE_CURVE ( ( 0.9330127018922194093, 0.9330127018922194093, 1.000000000000000000, 0.8660254037844387076, 1.000000000000000000, 0.8660254037844387076, 1.000000000000000000, 0.9330127018922194093, 0.9330127018922194093 ) ) 
 REPRESENTATION_ITEM ( '' )  );
#21832=CARTESIAN_POINT ( 'NONE',  ( -2.500000000000000444, -26.16666666666666430, -4.330127018922193649 ) ) ;
#21833=CARTESIAN_POINT ( 'NONE',  ( 4.458734124999998549, -26.72916666530106866, -2.574251347313721627 ) ) ;
#21834=CARTESIAN_POINT ( 'NONE',  ( 9.457646018065525792E-16, -88.06249999863439371, 5.148502694627439702 ) ) ;
#21835=CARTESIAN_POINT ( 'NONE',  ( -5.000000000000000000, -26.87499999726881583, 0.000000000000000000 ) ) ;
#21836=CARTESIAN_POINT ( 'NONE',  ( 4.458734124999999437, -54.81249999863440081, -5.460374474430324690E-16 ) ) ;
#21837=ORIENTED_EDGE ( 'NONE', *, *, #61761, .T. ) ;
#21840=CARTESIAN_POINT ( 'NONE',  ( 2.229367062500001939, -1.229166665301071548, 3.861377020970579999 ) ) ;
#21841=ORIENTED_EDGE ( 'NONE', *, *, #42224, .T. ) ;
#21842=CARTESIAN_POINT ( 'NONE',  ( -3.535250795749689387E-16, -73.25000000000000000, -5.773502691896257311 ) ) ;
#21846=CARTESIAN_POINT ( 'NONE',  ( 2.499999999999998668, -71.20833333060214443, -4.330127018922193649 ) ) ;
#21849=CARTESIAN_POINT ( 'NONE',  ( 2.229367062500001939, -17.22916666530106866, 3.861377020970579999 ) ) ;
#21850=CARTESIAN_POINT ( 'NONE',  ( 2.229367062500001939, -49.22916666530107221, 3.861377020970579999 ) ) ;
#21853=CARTESIAN_POINT ( 'NONE',  ( 1.846868145590735200, -140.2500000013656063, -4.458734125000000326 ) ) ;
#21855=CARTESIAN_POINT ( 'NONE',  ( 5.000000000000000888, -157.9375000000000000, -2.071067811865475505 ) ) ;
#21858=CARTESIAN_POINT ( 'NONE',  ( 2.229367062500001939, 26.77083333469892423, 3.861377020970579999 ) ) ;
#21860=DIRECTION ( 'NONE',  ( 0.000000000000000000, 0.000000000000000000, 1.000000000000000000 ) ) ;
#21863=CARTESIAN_POINT ( 'NONE',  ( -1.846868145590737420, -150.0000000013655779, 4.458734124999999437 ) ) ;
#21866=CARTESIAN_POINT ( 'NONE',  ( -3.152548672688508926E-16, -65.81249999863440792, -5.148502694627439702 ) ) ;
#21867=CARTESIAN_POINT ( 'NONE',  ( -2.499999999999996447, -83.70833333060214443, 4.330127018922195425 ) ) ;
#21869=CARTESIAN_POINT ( 'NONE',  ( -1.846868145590734756, -146.1250000013655779, -4.458734124999999437 ) ) ;
#21870=( BOUNDED_CURVE ( )  B_SPLINE_CURVE ( 2, ( #39922, #10660, #711, #74, #45079, #59570, #1046, #15503, #20652 ),
 .UNSPECIFIED., .F., .F. ) 
 B_SPLINE_CURVE_WITH_KNOTS ( ( 3, 2, 2, 2, 3 ),
 ( 0.6270833333333333259, 0.6277777777777777679, 0.6291666666666666519, 0.6305555555555555358, 0.6312499999999999778 ),
 .UNSPECIFIED. ) 
 CURVE ( )  GEOMETRIC_REPRESENTATION_ITEM ( )  RATIONAL_B_SPLINE_CURVE ( ( 0.9330127018922194093, 0.9330127018922194093, 1.000000000000000000, 0.8660254037844387076, 1.000000000000000000, 0.8660254037844387076, 1.000000000000000000, 0.9330127018922194093, 0.9330127018922194093 ) ) 
 REPRESENTATION_ITEM ( '' )  );
#21872=VERTEX_POINT ( 'NONE', #55528 ) ;
#21874=CARTESIAN_POINT ( 'NONE',  ( -5.000000000000000888, -144.5625000000000000, -2.071067811865475949 ) ) ;
#21877=CARTESIAN_POINT ( 'NONE',  ( 4.458734124999998549, 26.02083333469892779, -2.574251347313721627 ) ) ;
#21878=CARTESIAN_POINT ( 'NONE',  ( -2.499999999999996447, -5.833333333333336590, 4.330127018922195425 ) ) ;
#21883=DIRECTION ( 'NONE',  ( -0.000000000000000000, 1.000000000000000000, -0.000000000000000000 ) ) ;
#21884=CARTESIAN_POINT ( 'NONE',  ( -6.972266317189433020E-16, -60.12499999726880873, -5.000000000000000000 ) ) ;
#21885=CARTESIAN_POINT ( 'NONE',  ( -2.229367062500000163, 10.52083333469892779, -3.861377020970580443 ) ) ;
#21887=CARTESIAN_POINT ( 'NONE',  ( 4.458734124999998549, -20.97916666530107221, -2.574251347313721627 ) ) ;
#21889=CARTESIAN_POINT ( 'NONE',  ( 3.152801135295366208, -159.5625000013656063, 3.152801135295367985 ) ) ;
#21894=CARTESIAN_POINT ( 'NONE',  ( -4.458734124999999437, -34.39583333196772941, -2.574251347313719407 ) ) ;
#21895=CYLINDRICAL_SURFACE ( 'NONE', #16352, 5.000000000000000000 ) ;
#21897=CARTESIAN_POINT ( 'NONE',  ( 1.975475456537005874E-15, -13.75000000000000000, 5.000000000000000000 ) ) ;
#21898=CARTESIAN_POINT ( 'NONE',  ( -6.972266317189433020E-16, -89.24999999999998579, -5.000000000000000000 ) ) ;
#21899=ORIENTED_EDGE ( 'NONE', *, *, #50975, .F. ) ;
#21902=CARTESIAN_POINT ( 'NONE',  ( 2.071067811865560326, -143.9375000027311842, -4.999999999999914735 ) ) ;
#21903=CARTESIAN_POINT ( 'NONE',  ( -2.499999999999996447, -8.833333333333332149, 4.330127018922195425 ) ) ;
#21904=CARTESIAN_POINT ( 'NONE',  ( 4.458734124999999437, -74.81249999863440792, -5.460374474430324690E-16 ) ) ;
#21905=CARTESIAN_POINT ( 'NONE',  ( -2.499999999999996447, -16.83333333333333215, 4.330127018922195425 ) ) ;
#21906=CARTESIAN_POINT ( 'NONE',  ( -2.500000000000000444, -8.041666663935481907, -4.330127018922193649 ) ) ;
#21907=CARTESIAN_POINT ( 'NONE',  ( -3.152548672688508926E-16, -38.56249999863439371, -5.148502694627439702 ) ) ;
#21908=ORIENTED_EDGE ( 'NONE', *, *, #654, .F. ) ;
#21910=CARTESIAN_POINT ( 'NONE',  ( 2.229367062499998831, 14.10416666803226171, -3.861377020970580887 ) ) ;
#21912=CARTESIAN_POINT ( 'NONE',  ( 2.499999999999998668, -81.20833333060213022, -4.330127018922193649 ) ) ;
#21913=CARTESIAN_POINT ( 'NONE',  ( 5.000000000000000000, -57.41666666666667140, -2.886751345948129988 ) ) ;
#21914=CARTESIAN_POINT ( 'NONE',  ( 3.152801135295366208, -159.8125000013656063, 3.152801135295367985 ) ) ;
#21916=CARTESIAN_POINT ( 'NONE',  ( -1.339745962155613812, -35.20534180126148271, -5.000000000000000000 ) ) ;
#21917=CARTESIAN_POINT ( 'NONE',  ( 2.229367062500001939, -80.97916666530106511, 3.861377020970579999 ) ) ;
#21918=CARTESIAN_POINT ( 'NONE',  ( 2.730187237215162345E-16, -141.4375000013656063, -4.458734124999999437 ) ) ;
#21919=CARTESIAN_POINT ( 'NONE',  ( -4.458734124999998549, -85.22916666530107932, 2.574251347313722516 ) ) ;
#21921=CARTESIAN_POINT ( 'NONE',  ( -4.458734124999998549, -0.4791666653010707710, 2.574251347313722516 ) ) ;
#21922=CARTESIAN_POINT ( 'NONE',  ( -2.229367062499996610, -35.39583333196772941, 3.861377020970582219 ) ) ;
#21926=ORIENTED_EDGE ( 'NONE', *, *, #37737, .T. ) ;
#21928=CARTESIAN_POINT ( 'NONE',  ( 5.000000000000000888, -151.9375000000000000, -2.071067811865475505 ) ) ;
#21929=CARTESIAN_POINT ( 'NONE',  ( -3.152548672688508926E-16, -66.81249999863442213, -5.148502694627439702 ) ) ;
#21930=ADVANCED_FACE ( 'NONE', ( #10806 ), #6623, .T. ) ;
#21932=VERTEX_POINT ( 'NONE', #11119 ) ;
#21937=CARTESIAN_POINT ( 'NONE',  ( -4.458734124999998549, 8.770833334698927786, 2.574251347313722516 ) ) ;
#21938=CARTESIAN_POINT ( 'NONE',  ( -5.000000000000000000, -76.00000000000000000, 0.000000000000000000 ) ) ;
#21939=CARTESIAN_POINT ( 'NONE',  ( -4.458734124999999437, -159.0000000013656063, -1.846868145590735644 ) ) ;
#21953=CARTESIAN_POINT ( 'NONE',  ( -4.458734124999999437, 27.60416666803226349, -2.574251347313719407 ) ) ;
#21956=CARTESIAN_POINT ( 'NONE',  ( 4.458734124999998549, 4.020833334698926009, -2.574251347313721627 ) ) ;
#21957=CARTESIAN_POINT ( 'NONE',  ( -6.972266317189433020E-16, -0.1249999972688142363, -5.000000000000000000 ) ) ;
#21959=CARTESIAN_POINT ( 'NONE',  ( -9.184850993605147944E-16, -141.3750000027312126, 5.000000000000000000 ) ) ;
#21960=CARTESIAN_POINT ( 'NONE',  ( -6.972266317189433020E-16, -33.12499999726880873, -5.000000000000000000 ) ) ;
#21966=CARTESIAN_POINT ( 'NONE',  ( 0.000000000000000000, -170.0000000000000000, 0.000000000000000000 ) ) ;
#21970=CARTESIAN_POINT ( 'NONE',  ( -3.152801135295367096, -161.3125000013656063, -3.152801135295367541 ) ) ;
#21974=ORIENTED_EDGE ( 'NONE', *, *, #62146, .F. ) ;
#21975=CARTESIAN_POINT ( 'NONE',  ( -2.229367062499996610, 17.60416666803225993, 3.861377020970582219 ) ) ;
#21981=CARTESIAN_POINT ( 'NONE',  ( -5.000000000000000000, 8.000000000000000000, 0.000000000000000000 ) ) ;
#21982=CARTESIAN_POINT ( 'NONE',  ( -2.229367062500000163, -58.47916666530106511, -3.861377020970580443 ) ) ;
#21986=CARTESIAN_POINT ( 'NONE',  ( -2.499999999999996447, -37.70833333060213732, 4.330127018922195425 ) ) ;
#21987=CARTESIAN_POINT ( 'NONE',  ( -2.499999999999996447, -63.83333333333332860, 4.330127018922195425 ) ) ;
#21988=CARTESIAN_POINT ( 'NONE',  ( -1.339745962155610925, -24.66965819600733667, 5.000000000000000000 ) ) ;
#21989=CARTESIAN_POINT ( 'NONE',  ( -4.999999999999999112, -37.91666666666666430, 2.886751345948131764 ) ) ;
#21991=CARTESIAN_POINT ( 'NONE',  ( -5.000000000000000000, -45.00000000000000000, 0.000000000000000000 ) ) ;
#21993=DIRECTION ( 'NONE',  ( -0.000000000000000000, 1.000000000000000000, -0.000000000000000000 ) ) ;
#21994=CARTESIAN_POINT ( 'NONE',  ( -2.229367062500000163, -57.47916666530107932, -3.861377020970580443 ) ) ;
#21995=CARTESIAN_POINT ( 'NONE',  ( 1.846868145590736310, -151.8750000013655779, 4.458734124999999437 ) ) ;
#21996=CARTESIAN_POINT ( 'NONE',  ( -2.229367062499996610, -72.14583333196773651, 3.861377020970582219 ) ) ;
#21998=CARTESIAN_POINT ( 'NONE',  ( 4.458734124999998549, -21.97916666530107221, -2.574251347313721627 ) ) ;
#21999=CARTESIAN_POINT ( 'NONE',  ( -2.499999999999996447, -60.70833333060214443, 4.330127018922195425 ) ) ;
#22001=CARTESIAN_POINT ( 'NONE',  ( -2.499999999999996447, -48.83333333333332860, 4.330127018922195425 ) ) ;
#22004=CARTESIAN_POINT ( 'NONE',  ( 1.975475456537005874E-15, -64.74999999999998579, 5.000000000000000000 ) ) ;
#22005=CARTESIAN_POINT ( 'NONE',  ( -1.846868145590737420, -152.7500000013656063, 4.458734124999999437 ) ) ;
#22006=ORIENTED_EDGE ( 'NONE', *, *, #50294, .F. ) ;
#22007=CARTESIAN_POINT ( 'NONE',  ( 2.500000000000002220, 25.33333333333333215, 4.330127018922192761 ) ) ;
#22010=CARTESIAN_POINT ( 'NONE',  ( 2.229367062500001939, -50.22916666530107221, 3.861377020970579999 ) ) ;
#22011=EDGE_CURVE ( 'NONE', #25520, #5760, #8525, .T. ) ;
#22013=CARTESIAN_POINT ( 'NONE',  ( 2.626220312808019583E-14, 15.74999999999999645, -5.000000000000000000 ) ) ;
#22015=CARTESIAN_POINT ( 'NONE',  ( -2.229367062500000163, 24.52083333469892779, -3.861377020970580443 ) ) ;
#22017=CARTESIAN_POINT ( 'NONE',  ( 2.499999999999998668, -13.20833333060214976, -4.330127018922193649 ) ) ;
#22018=CARTESIAN_POINT ( 'NONE',  ( 5.000000000000000888, -164.9375000000000284, -2.071067811865475505 ) ) ;
#22019=( BOUNDED_CURVE ( )  B_SPLINE_CURVE ( 2, ( #55190, #54220, #4692, #58730, #24314, #43921, #63568, #14656, #10158 ),
 .UNSPECIFIED., .F., .F. ) 
 B_SPLINE_CURVE_WITH_KNOTS ( ( 3, 2, 2, 2, 3 ),
 ( 0.6979166666666666297, 0.6986111111111110716, 0.6999999999999999556, 0.7013888888888888395, 0.7020833333333332815 ),
 .UNSPECIFIED. ) 
 CURVE ( )  GEOMETRIC_REPRESENTATION_ITEM ( )  RATIONAL_B_SPLINE_CURVE ( ( 0.9330127018922194093, 0.9330127018922194093, 1.000000000000000000, 0.8660254037844387076, 1.000000000000000000, 0.8660254037844387076, 1.000000000000000000, 0.9330127018922194093, 0.9330127018922194093 ) ) 
 REPRESENTATION_ITEM ( '' )  );
#22022=CARTESIAN_POINT ( 'NONE',  ( -5.000000000000000000, 0.9166666666666664076, -2.886751345948128211 ) ) ;
#22030=CARTESIAN_POINT ( 'NONE',  ( -3.535533905932738641, -139.5000000027311842, 3.535533905932737309 ) ) ;
#22033=ORIENTED_EDGE ( 'NONE', *, *, #25556, .F. ) ;
#22036=CARTESIAN_POINT ( 'NONE',  ( -9.184850993605147944E-16, -156.3750000027311842, 5.000000000000000000 ) ) ;
#22042=CARTESIAN_POINT ( 'NONE',  ( 5.000000000000000000, -147.0625000000000000, 2.071067811865478614 ) ) ;
#22046=CARTESIAN_POINT ( 'NONE',  ( -3.152548672688508926E-16, -23.56249999863440436, -5.148502694627439702 ) ) ;
#22048=CARTESIAN_POINT ( 'NONE',  ( -2.071067811865478170, -151.3125000000000284, 5.000000000000000000 ) ) ;
#22050=CARTESIAN_POINT ( 'NONE',  ( 4.458734124999999437, -150.4375000013656063, 0.000000000000000000 ) ) ;
#22053=CARTESIAN_POINT ( 'NONE',  ( 2.229367062499998831, -51.89583333196773651, -3.861377020970580887 ) ) ;
#22054=( BOUNDED_CURVE ( )  B_SPLINE_CURVE ( 2, ( #20113, #39717, #59354, #1474, #25579, #15289, #10454, #30069, #49698 ),
 .UNSPECIFIED., .F., .F. ) 
 B_SPLINE_CURVE_WITH_KNOTS ( ( 3, 2, 2, 2, 3 ),
 ( 0.1479166666666666685, 0.1486111111111111105, 0.1499999999999999944, 0.1513888888888888784, 0.1520833333333333481 ),
 .UNSPECIFIED. ) 
 CURVE ( )  GEOMETRIC_REPRESENTATION_ITEM ( )  RATIONAL_B_SPLINE_CURVE ( ( 0.9330127018922194093, 0.9330127018922194093, 1.000000000000000000, 0.8660254037844387076, 1.000000000000000000, 0.8660254037844387076, 1.000000000000000000, 0.9330127018922180770, 0.9330127018922194093 ) ) 
 REPRESENTATION_ITEM ( '' )  );
#22055=CARTESIAN_POINT ( 'NONE',  ( 0.000000000000000000, -170.0000000000000000, 0.000000000000000000 ) ) ;
#22057=CARTESIAN_POINT ( 'NONE',  ( 5.000000000000000000, 23.58333333333333215, -2.886751345948129988 ) ) ;
#22061=CARTESIAN_POINT ( 'NONE',  ( -4.458734124999998549, -3.229166665301069994, 2.574251347313722516 ) ) ;
#22062=CARTESIAN_POINT ( 'NONE',  ( 0.000000000000000000, -170.0000000000000000, 0.000000000000000000 ) ) ;
#22064=CARTESIAN_POINT ( 'NONE',  ( 2.229367062500001939, 15.77083333469892601, 3.861377020970579999 ) ) ;
#22065=CARTESIAN_POINT ( 'NONE',  ( 2.499999999999998668, 0.7916666693978530178, -4.330127018922193649 ) ) ;
#22069=CARTESIAN_POINT ( 'NONE',  ( -6.972266317189433020E-16, -24.12499999726881228, -5.000000000000000000 ) ) ;
#22070=CARTESIAN_POINT ( 'NONE',  ( 2.229367062500001939, -42.97916666530107932, 3.861377020970579999 ) ) ;
#22071=CARTESIAN_POINT ( 'NONE',  ( 3.152801135295367541, -164.5625000013656063, -3.152801135295367541 ) ) ;
#22072=CARTESIAN_POINT ( 'NONE',  ( 1.060575238724906964E-15, -42.62499999726880162, 5.773502691896257311 ) ) ;
#22074=CARTESIAN_POINT ( 'NONE',  ( 4.458734124999999437, -19.81249999863440081, -5.460374474430324690E-16 ) ) ;
#22075=ORIENTED_EDGE ( 'NONE', *, *, #19321, .T. ) ;
#22076=CARTESIAN_POINT ( 'NONE',  ( 5.000000000000000888, -87.58333333333332860, 2.886751345948126879 ) ) ;
#22077=CARTESIAN_POINT ( 'NONE',  ( -4.458734124999999437, -163.9375000013655779, -5.460374474430324690E-16 ) ) ;
#22080=CARTESIAN_POINT ( 'NONE',  ( 4.458734125000001214, -33.14583333196774362, 2.574251347313718519 ) ) ;
#22084=ADVANCED_FACE ( 'NONE', ( #47752 ), #47132, .T. ) ;
#22088=ORIENTED_EDGE ( 'NONE', *, *, #812, .F. ) ;
#22089=CARTESIAN_POINT ( 'NONE',  ( 1.975475456537005874E-15, -83.74999999999998579, 5.000000000000000000 ) ) ;
#22091=CARTESIAN_POINT ( 'NONE',  ( 2.229367062500001939, -78.22916666530106511, 3.861377020970579999 ) ) ;
#22098=CARTESIAN_POINT ( 'NONE',  ( -2.229367062500000163, -45.47916666530106511, -3.861377020970580443 ) ) ;
#22103=AXIS2_PLACEMENT_3D ( 'NONE', #60137, #16058, #55315 ) ;
#22104=CARTESIAN_POINT ( 'NONE',  ( 5.000000000000000000, -169.5625000013656063, 0.000000000000000000 ) ) ;
#22108=EDGE_CURVE ( 'NONE', #57819, #19872, #17341, .T. ) ;
#22110=CARTESIAN_POINT ( 'NONE',  ( -4.458734124999999437, -78.56249999863440792, 0.000000000000000000 ) ) ;
#22115=EDGE_CURVE ( 'NONE', #50115, #39210, #23902, .T. ) ;
#22117=EDGE_CURVE ( 'NONE', #32533, #30611, #19099, .T. ) ;
#22118=CARTESIAN_POINT ( 'NONE',  ( 0.000000000000000000, -170.0000000000000000, 0.000000000000000000 ) ) ;
#22120=CARTESIAN_POINT ( 'NONE',  ( 2.229367062499998831, 11.10416666803225993, -3.861377020970580887 ) ) ;
#22126=CARTESIAN_POINT ( 'NONE',  ( -5.000000000000000000, -15.95833333060214443, -2.886751345948128211 ) ) ;
#22127=CARTESIAN_POINT ( 'NONE',  ( -2.229367062499996610, -7.145833331967735624, 3.861377020970582219 ) ) ;
#22129=ORIENTED_EDGE ( 'NONE', *, *, #25509, .T. ) ;
#22130=CARTESIAN_POINT ( 'NONE',  ( -4.458734124999999437, -34.56249999863440792, 0.000000000000000000 ) ) ;
#22135=CARTESIAN_POINT ( 'NONE',  ( -1.846868145590734756, -148.3750000013655779, -4.458734124999999437 ) ) ;
#22136=CARTESIAN_POINT ( 'NONE',  ( 2.229367062500001939, 22.02083333469892779, 3.861377020970579999 ) ) ;
#22138=CARTESIAN_POINT ( 'NONE',  ( 1.975475456537005874E-15, -66.74999999999998579, 5.000000000000000000 ) ) ;
#22139=CARTESIAN_POINT ( 'NONE',  ( -4.458734124999999437, -84.64583333196773651, -2.574251347313719407 ) ) ;
#22142=CARTESIAN_POINT ( 'NONE',  ( 5.000000000000000000, 21.62500000273118417, -6.123233995736766282E-16 ) ) ;
#22147=CARTESIAN_POINT ( 'NONE',  ( -5.000000000000000000, -23.00000000000000000, 0.000000000000000000 ) ) ;
#22148=CARTESIAN_POINT ( 'NONE',  ( -4.458734124999999437, -26.39583333196773651, -2.574251347313719407 ) ) ;
#22149=CARTESIAN_POINT ( 'NONE',  ( 4.458734125000000326, -85.89583333196775072, 2.574251347313718519 ) ) ;
#22152=CARTESIAN_POINT ( 'NONE',  ( 5.000000000000000000, -31.29166666393548368, -2.886751345948129988 ) ) ;
#22153=CARTESIAN_POINT ( 'NONE',  ( -4.458734124999999437, -55.31249999863440081, 0.000000000000000000 ) ) ;
#22154=ORIENTED_EDGE ( 'NONE', *, *, #30741, .T. ) ;
#22156=CARTESIAN_POINT ( 'NONE',  ( -4.458734124999998549, -9.479166665301070438, 2.574251347313722516 ) ) ;
#22158=CARTESIAN_POINT ( 'NONE',  ( -5.000000000000000000, -74.00000000000000000, 0.000000000000000000 ) ) ;
#22161=CARTESIAN_POINT ( 'NONE',  ( -4.999999999999999112, -78.79166666393547303, 2.886751345948131764 ) ) ;
#22165=CARTESIAN_POINT ( 'NONE',  ( -2.229367062500000163, -18.72916666530106866, -3.861377020970580443 ) ) ;
#22166=CARTESIAN_POINT ( 'NONE',  ( -2.229367062500000163, -51.72916666530107221, -3.861377020970580443 ) ) ;
#22168=CARTESIAN_POINT ( 'NONE',  ( -1.846868145590737420, -140.7500000013655779, 4.458734124999999437 ) ) ;
#22170=CARTESIAN_POINT ( 'NONE',  ( 1.975475456537005874E-15, 10.24999999999999822, 5.000000000000000000 ) ) ;
#22174=CARTESIAN_POINT ( 'NONE',  ( 5.000000000000000000, 18.58333333333333215, -2.886751345948130876 ) ) ;
#22177=CARTESIAN_POINT ( 'NONE',  ( 3.152801135295366208, -147.8125000013655779, 3.152801135295367985 ) ) ;
#22181=CARTESIAN_POINT ( 'NONE',  ( -4.458734124999999437, -61.56249999863440081, 0.000000000000000000 ) ) ;
#22182=AXIS2_PLACEMENT_3D ( 'NONE', #49517, #29887, #35364 ) ;
#22186=CARTESIAN_POINT ( 'NONE',  ( -3.152801135295367985, -144.8125000013655779, 3.152801135295367096 ) ) ;
#22188=EDGE_LOOP ( 'NONE', ( #54024, #60044, #44780, #36737 ) ) ;
#22196=CARTESIAN_POINT ( 'NONE',  ( -1.339745962155610925, -17.66965819600733312, 5.000000000000000000 ) ) ;
#22199=EDGE_CURVE ( 'NONE', #6259, #20545, #6260, .T. ) ;
#22204=CARTESIAN_POINT ( 'NONE',  ( 5.000000000000000000, 21.58333333333333215, -2.886751345948130876 ) ) ;
#22205=CARTESIAN_POINT ( 'NONE',  ( 9.457646018065525792E-16, 8.937500001365595637, 5.148502694627439702 ) ) ;
#22207=CARTESIAN_POINT ( 'NONE',  ( 2.229367062499998831, -17.89583333196773651, -3.861377020970580887 ) ) ;
#22210=CARTESIAN_POINT ( 'NONE',  ( 4.458734124999999437, -159.4375000013655779, 0.000000000000000000 ) ) ;
#22215=CARTESIAN_POINT ( 'NONE',  ( 4.458734124999999437, -42.81249999863440081, -5.460374474430324690E-16 ) ) ;
#22216=CARTESIAN_POINT ( 'NONE',  ( 1.339745962155615144, 19.41965820146970501, 4.999999999999999112 ) ) ;
#22217=CARTESIAN_POINT ( 'NONE',  ( -4.458734124999999437, -68.64583333196773651, -2.574251347313719407 ) ) ;
#22219=CARTESIAN_POINT ( 'NONE',  ( -6.972266317189433020E-16, -57.12499999726879452, -5.000000000000000000 ) ) ;
#22220=CARTESIAN_POINT ( 'NONE',  ( -6.972266317189433020E-16, -41.24999999999999289, -5.000000000000000000 ) ) ;
#22223=DIRECTION ( 'NONE',  ( -0.000000000000000000, 1.000000000000000000, -0.000000000000000000 ) ) ;
#22224=CARTESIAN_POINT ( 'NONE',  ( 5.000000000000000000, -7.500000000000000000, -6.123233995736766282E-16 ) ) ;
#22225=CARTESIAN_POINT ( 'NONE',  ( -3.152548672688508926E-16, -71.56249999863439371, -5.148502694627439702 ) ) ;
#22227=CARTESIAN_POINT ( 'NONE',  ( -5.000000000000000000, -13.95833333060215153, -2.886751345948128211 ) ) ;
#22228=CARTESIAN_POINT ( 'NONE',  ( -2.229367062500000163, -39.47916666530107221, -3.861377020970580443 ) ) ;
#22231=CARTESIAN_POINT ( 'NONE',  ( 2.229367062500001939, 9.770833334698927786, 3.861377020970579999 ) ) ;
#22233=CARTESIAN_POINT ( 'NONE',  ( -3.535533905932737309, -151.6250000000000000, -3.535533905932738197 ) ) ;
#22234=CARTESIAN_POINT ( 'NONE',  ( 5.000000000000000888, -56.58333333333332860, 2.886751345948126879 ) ) ;
#22235=CARTESIAN_POINT ( 'NONE',  ( -3.152801135295367096, -160.3125000013656063, -3.152801135295367541 ) ) ;
#22237=CARTESIAN_POINT ( 'NONE',  ( 0.000000000000000000, -170.0000000000000000, 5.000000000000000000 ) ) ;
#22238=CARTESIAN_POINT ( 'NONE',  ( 4.458734125000001214, -80.89583333196773651, 2.574251347313718519 ) ) ;
#22239=CARTESIAN_POINT ( 'NONE',  ( 3.535533905932738197, -164.8750000000000284, -3.535533905932738197 ) ) ;
#22240=CARTESIAN_POINT ( 'NONE',  ( 4.458734124999998549, -84.72916666530106511, -2.574251347313721627 ) ) ;
#22242=VECTOR ( 'NONE', #47904, 1000.000000000000000 ) ;
#22243=CARTESIAN_POINT ( 'NONE',  ( 4.458734124999998549, -0.9791666653010713262, -2.574251347313721627 ) ) ;
#22244=AXIS2_PLACEMENT_3D ( 'NONE', #37845, #43283, #53572 ) ;
#22245=CARTESIAN_POINT ( 'NONE',  ( 4.458734125000001214, -37.14583333196773651, 2.574251347313718519 ) ) ;
#22246=EDGE_CURVE ( 'NONE', #11915, #27774, #52901, .T. ) ;
#22247=CARTESIAN_POINT ( 'NONE',  ( 2.499999999999998668, -16.20833333060214443, -4.330127018922193649 ) ) ;
#22251=( BOUNDED_CURVE ( )  B_SPLINE_CURVE ( 2, ( #20529, #31118, #26291, #1243, #35000, #20843, #50740, #15055, #10540 ),
 .UNSPECIFIED., .F., .F. ) 
 B_SPLINE_CURVE_WITH_KNOTS ( ( 3, 2, 2, 2, 3 ),
 ( 0.7916666666666664076, 0.7958333333333330595, 0.7999999999999998224, 0.8041666666666664742, 0.8083333333333331261 ),
 .UNSPECIFIED. ) 
 CURVE ( )  GEOMETRIC_REPRESENTATION_ITEM ( )  RATIONAL_B_SPLINE_CURVE ( ( 1.000000000000003997, 0.9238795325112826307, 1.000000000000000000, 0.9238795325112867385, 1.000000000000000000, 0.9238795325112867385, 1.000000000000000000, 0.9238795325112908463, 0.9999999999999958922 ) ) 
 REPRESENTATION_ITEM ( '' )  );
#22252=CARTESIAN_POINT ( 'NONE',  ( -5.000000000000000000, -11.87499999726881761, 0.000000000000000000 ) ) ;
#22253=CARTESIAN_POINT ( 'NONE',  ( 2.229367062500001939, -67.22916666530106511, 3.861377020970579999 ) ) ;
#22255=ORIENTED_EDGE ( 'NONE', *, *, #29108, .F. ) ;
#22260=CARTESIAN_POINT ( 'NONE',  ( 9.457646018065525792E-16, 3.937500001365595192, 5.148502694627439702 ) ) ;
#22261=CARTESIAN_POINT ( 'NONE',  ( -5.000000000000000000, -76.08333333333334281, -2.886751345948128211 ) ) ;
#22262=CARTESIAN_POINT ( 'NONE',  ( 1.846868145590736310, -157.6250000013655779, 4.458734124999997661 ) ) ;
#22266=CARTESIAN_POINT ( 'NONE',  ( 0.000000000000000000, -170.0000000000000000, 0.000000000000000000 ) ) ;
#22274=CARTESIAN_POINT ( 'NONE',  ( 2.229367062500001939, 22.02083333469892779, 3.861377020970579999 ) ) ;
#22276=CARTESIAN_POINT ( 'NONE',  ( 4.458734124999999437, -1.062499998634405696, -5.460374474430324690E-16 ) ) ;
#22277=VECTOR ( 'NONE', #6313, 1000.000000000000000 ) ;
#22278=CARTESIAN_POINT ( 'NONE',  ( 2.071067811865561215, -160.3125000027312126, 4.999999999999913847 ) ) ;
#22280=CARTESIAN_POINT ( 'NONE',  ( 5.000000000000000000, -142.1875000027312126, 2.071067811865478614 ) ) ;
#22281=CYLINDRICAL_SURFACE ( 'NONE', #48964, 5.000000000000000000 ) ;
#22284=AXIS2_PLACEMENT_3D ( 'NONE', #43242, #4960, #18500 ) ;
#22287=CARTESIAN_POINT ( 'NONE',  ( 5.000000000000000888, -22.58333333333332860, 2.886751345948126879 ) ) ;
#22288=AXIS2_PLACEMENT_3D ( 'NONE', #19957, #34759, #29601 ) ;
#22290=CARTESIAN_POINT ( 'NONE',  ( 4.458734124999999437, -157.6250000013655779, -1.846868145590734978 ) ) ;
#22294=CARTESIAN_POINT ( 'NONE',  ( -3.152548672688508926E-16, 20.18750000136559208, -5.148502694627439702 ) ) ;
#22299=CARTESIAN_POINT ( 'NONE',  ( -5.000000000000000000, 6.999999999999999112, 0.000000000000000000 ) ) ;
#22301=CARTESIAN_POINT ( 'NONE',  ( -2.229367062500000163, -57.47916666530107932, -3.861377020970580443 ) ) ;
#22302=CARTESIAN_POINT ( 'NONE',  ( -1.339745962155613812, -8.205341801261480938, -5.000000000000000000 ) ) ;
#22305=CARTESIAN_POINT ( 'NONE',  ( 1.975475456537005874E-15, 7.375000002731186832, 5.000000000000000000 ) ) ;
#22306=CARTESIAN_POINT ( 'NONE',  ( 0.000000000000000000, -170.0000000000000000, 0.000000000000000000 ) ) ;
#22307=DIRECTION ( 'NONE',  ( 0.000000000000000000, 0.000000000000000000, 1.000000000000000000 ) ) ;
#22308=CARTESIAN_POINT ( 'NONE',  ( 5.000000000000000000, -41.41666666666667140, -2.886751345948129988 ) ) ;
#22309=CARTESIAN_POINT ( 'NONE',  ( 1.975475456537005874E-15, 13.37500000273118417, 5.000000000000000000 ) ) ;
#22312=LINE ( 'NONE', #31637, #6028 ) ;
#22313=CARTESIAN_POINT ( 'NONE',  ( -4.458734124999999437, -64.39583333196772230, -2.574251347313719407 ) ) ;
#22314=CARTESIAN_POINT ( 'NONE',  ( 1.846868145590735200, -150.5000000013656347, -4.458734125000000326 ) ) ;
#22315=CARTESIAN_POINT ( 'NONE',  ( 2.229367062500001939, -68.97916666530107932, 3.861377020970579999 ) ) ;
#22317=CARTESIAN_POINT ( 'NONE',  ( 9.457646018065525792E-16, -18.31249999863440436, 5.148502694627439702 ) ) ;
#22318=CARTESIAN_POINT ( 'NONE',  ( 5.000000000000000000, -61.29166666393548013, -2.886751345948129988 ) ) ;
#22319=ORIENTED_EDGE ( 'NONE', *, *, #29322, .F. ) ;
#22323=FACE_OUTER_BOUND ( 'NONE', #57075, .T. ) ;
#22324=CARTESIAN_POINT ( 'NONE',  ( 6.123233995736766282E-16, -170.0000000000000000, -5.000000000000000000 ) ) ;
#22325=CARTESIAN_POINT ( 'NONE',  ( 3.152801135295367541, -151.3125000013655779, -3.152801135295367541 ) ) ;
#22326=ORIENTED_EDGE ( 'NONE', *, *, #6001, .F. ) ;
#22327=VECTOR ( 'NONE', #48986, 1000.000000000000000 ) ;
#22330=CARTESIAN_POINT ( 'NONE',  ( -6.972266317189433020E-16, -8.249999999999998224, -5.000000000000000000 ) ) ;
#22331=CARTESIAN_POINT ( 'NONE',  ( 2.229367062500001939, -53.22916666530107221, 3.861377020970579999 ) ) ;
#22333=VECTOR ( 'NONE', #58944, 1000.000000000000000 ) ;
#22334=( BOUNDED_CURVE ( )  B_SPLINE_CURVE ( 2, ( #12198, #26995, #46614, #22174, #61421, #14078, #24063, #56908, #37587 ),
 .UNSPECIFIED., .F., .F. ) 
 B_SPLINE_CURVE_WITH_KNOTS ( ( 3, 2, 2, 2, 3 ),
 ( 0.09375000000000000000, 0.09444444444444444198, 0.09583333333333333981, 0.09722222222222222376, 0.09791666666666666574 ),
 .UNSPECIFIED. ) 
 CURVE ( )  GEOMETRIC_REPRESENTATION_ITEM ( )  RATIONAL_B_SPLINE_CURVE ( ( 0.9330127018922194093, 0.9330127018922194093, 1.000000000000000000, 0.8660254037844387076, 1.000000000000000000, 0.8660254037844387076, 1.000000000000000000, 0.9330127018922194093, 0.9330127018922194093 ) ) 
 REPRESENTATION_ITEM ( '' )  );
#22335=DIRECTION ( 'NONE',  ( 0.000000000000000000, 0.000000000000000000, 1.000000000000000000 ) ) ;
#22336=VECTOR ( 'NONE', #38404, 1000.000000000000000 ) ;
#22339=CARTESIAN_POINT ( 'NONE',  ( 2.229367062499998831, 21.35416666803226349, -3.861377020970580887 ) ) ;
#22342=CARTESIAN_POINT ( 'NONE',  ( 4.458734124999997661, -168.5000000013655779, 1.846868145590737864 ) ) ;
#22347=CARTESIAN_POINT ( 'NONE',  ( 5.000000000000000888, -69.45833333060214443, 2.886751345948126879 ) ) ;
#22351=CARTESIAN_POINT ( 'NONE',  ( 4.729367062499999719, -169.8437500006828031, 0.000000000000000000 ) ) ;
#22352=CARTESIAN_POINT ( 'NONE',  ( 0.000000000000000000, -170.0000000000000000, 0.000000000000000000 ) ) ;
#22355=ORIENTED_EDGE ( 'NONE', *, *, #57552, .T. ) ;
#22356=CARTESIAN_POINT ( 'NONE',  ( -6.972266317189433020E-16, -48.24999999999999289, -5.000000000000000000 ) ) ;
#22358=CARTESIAN_POINT ( 'NONE',  ( 5.000000000000000000, -155.1250000027311842, 0.000000000000000000 ) ) ;
#22359=ORIENTED_EDGE ( 'NONE', *, *, #16199, .T. ) ;
#22364=CARTESIAN_POINT ( 'NONE',  ( -2.071067811865478170, -147.3125000000000000, 5.000000000000000000 ) ) ;
#22368=CARTESIAN_POINT ( 'NONE',  ( -4.458734124999997661, -25.22916666530106866, 2.574251347313722516 ) ) ;
#22372=CARTESIAN_POINT ( 'NONE',  ( -3.152801135295367985, -148.8125000013655779, 3.152801135295367096 ) ) ;
#22374=CARTESIAN_POINT ( 'NONE',  ( 5.000000000000000000, -150.0000000000000284, 0.000000000000000000 ) ) ;
#22375=CARTESIAN_POINT ( 'NONE',  ( -4.458734124999999437, -51.56249999863440792, 0.000000000000000000 ) ) ;
#22377=LINE ( 'NONE', #13030, #55098 ) ;
#22379=CARTESIAN_POINT ( 'NONE',  ( 2.499999999999998668, 23.66666666666666430, -4.330127018922193649 ) ) ;
#22381=AXIS2_PLACEMENT_3D ( 'NONE', #49246, #29937, #14505 ) ;
#22382=CARTESIAN_POINT ( 'NONE',  ( 2.229367062499998831, -0.6458333319677399542, -3.861377020970580887 ) ) ;
#22383=CARTESIAN_POINT ( 'NONE',  ( 1.975475456537005874E-15, 4.375000002731185056, 5.000000000000000000 ) ) ;
#22385=CARTESIAN_POINT ( 'NONE',  ( -5.000000000000000000, -74.08333333333330017, -2.886751345948128211 ) ) ;
#22386=CARTESIAN_POINT ( 'NONE',  ( 4.458734124999999437, 14.93750000136559386, -5.460374474430324690E-16 ) ) ;
#22387=CARTESIAN_POINT ( 'NONE',  ( -4.999999999999999112, 3.208333336064520758, 2.886751345948131764 ) ) ;
#22389=CARTESIAN_POINT ( 'NONE',  ( 5.000000000000000000, 26.50000000000000000, -6.123233995736766282E-16 ) ) ;
#22391=CARTESIAN_POINT ( 'NONE',  ( 1.975475456537005874E-15, -70.75000000000000000, 5.000000000000000000 ) ) ;
#22392=CARTESIAN_POINT ( 'NONE',  ( 4.458734124999998549, -50.72916666530107932, -2.574251347313721627 ) ) ;
#22393=CARTESIAN_POINT ( 'NONE',  ( 4.458734124999999437, -162.6875000013655779, 0.000000000000000000 ) ) ;
#22394=EDGE_CURVE ( 'NONE', #5037, #43748, #26486, .T. ) ;
#22395=CARTESIAN_POINT ( 'NONE',  ( 5.000000000000000888, -47.45833333060214443, 2.886751345948126879 ) ) ;
#22396=ORIENTED_EDGE ( 'NONE', *, *, #58946, .F. ) ;
#22397=CARTESIAN_POINT ( 'NONE',  ( -2.229367062499996610, -25.14583333196773651, 3.861377020970582219 ) ) ;
#22400=CARTESIAN_POINT ( 'NONE',  ( -5.000000000000000000, -87.00000000000000000, 0.000000000000000000 ) ) ;
#22401=CARTESIAN_POINT ( 'NONE',  ( -1.846868145590734756, -166.1250000013655779, -4.458734125000000326 ) ) ;
#22402=( BOUNDED_CURVE ( )  B_SPLINE_CURVE ( 2, ( #35311, #49139, #5723, #5082, #24704, #59444, #35630, #6053, #6371 ),
 .UNSPECIFIED., .F., .F. ) 
 B_SPLINE_CURVE_WITH_KNOTS ( ( 3, 2, 2, 2, 3 ),
 ( 0.1187500000000000083, 0.1194444444444444503, 0.1208333333333333343, 0.1222222222222222182, 0.1229166666666666741 ),
 .UNSPECIFIED. ) 
 CURVE ( )  GEOMETRIC_REPRESENTATION_ITEM ( )  RATIONAL_B_SPLINE_CURVE ( ( 0.9330127018922194093, 0.9330127018922200755, 1.000000000000000000, 0.8660254037844387076, 1.000000000000000000, 0.8660254037844387076, 1.000000000000000000, 0.9330127018922187432, 0.9330127018922194093 ) ) 
 REPRESENTATION_ITEM ( '' )  );
#22405=CARTESIAN_POINT ( 'NONE',  ( 4.458734124999999437, -31.06249999863440436, -5.460374474430324690E-16 ) ) ;
#22406=FACE_OUTER_BOUND ( 'NONE', #46029, .T. ) ;
#22410=CARTESIAN_POINT ( 'NONE',  ( -1.339745962155613812, -29.08034179853029144, -5.000000000000000000 ) ) ;
#22412=CARTESIAN_POINT ( 'NONE',  ( -6.972266317189433020E-16, -23.12499999726880873, -5.000000000000000000 ) ) ;
#22414=CARTESIAN_POINT ( 'NONE',  ( 2.229367062499998831, -79.89583333196773651, -3.861377020970580887 ) ) ;
#22417=CARTESIAN_POINT ( 'NONE',  ( 1.975475456537005874E-15, -9.750000000000000000, 5.000000000000000000 ) ) ;
#22421=DIRECTION ( 'NONE',  ( -0.000000000000000000, 1.000000000000000000, -0.000000000000000000 ) ) ;
#22425=CARTESIAN_POINT ( 'NONE',  ( -1.339745962155613812, 3.794658198738521282, -5.000000000000000000 ) ) ;
#22430=CARTESIAN_POINT ( 'NONE',  ( 1.255007937094098239E-14, 24.75000000000000000, -4.999999999999999112 ) ) ;
#22431=CARTESIAN_POINT ( 'NONE',  ( 9.457646018065525792E-16, -80.31249999863440792, 5.148502694627439702 ) ) ;
#22433=( BOUNDED_CURVE ( )  B_SPLINE_CURVE ( 2, ( #20022, #39947, #14553, #54111, #5235, #39628, #4914, #54764, #25483 ),
 .UNSPECIFIED., .F., .F. ) 
 B_SPLINE_CURVE_WITH_KNOTS ( ( 3, 2, 2, 2, 3 ),
 ( 0.4520833333333333370, 0.4527777777777777790, 0.4541666666666666630, 0.4555555555555555469, 0.4562499999999999889 ),
 .UNSPECIFIED. ) 
 CURVE ( )  GEOMETRIC_REPRESENTATION_ITEM ( )  RATIONAL_B_SPLINE_CURVE ( ( 0.9330127018922194093, 0.9330127018922194093, 1.000000000000000000, 0.8660254037844387076, 1.000000000000000000, 0.8660254037844387076, 1.000000000000000000, 0.9330127018922194093, 0.9330127018922194093 ) ) 
 REPRESENTATION_ITEM ( '' )  );
#22436=CARTESIAN_POINT ( 'NONE',  ( 1.975475456537005874E-15, -82.74999999999998579, 5.000000000000000000 ) ) ;
#22438=CARTESIAN_POINT ( 'NONE',  ( 3.061616997868383141E-16, -163.8750000027311842, -5.000000000000000000 ) ) ;
#22440=CARTESIAN_POINT ( 'NONE',  ( -4.458734124999999437, 14.43750000136559386, 0.000000000000000000 ) ) ;
#22446=CARTESIAN_POINT ( 'NONE',  ( -5.000000000000000000, -15.87499999726881406, 0.000000000000000000 ) ) ;
#22447=CARTESIAN_POINT ( 'NONE',  ( -2.229367062499996610, -8.145833331967736513, 3.861377020970582219 ) ) ;
#22449=ORIENTED_EDGE ( 'NONE', *, *, #25496, .T. ) ;
#22450=CARTESIAN_POINT ( 'NONE',  ( -4.458734124999997661, -34.47916666530107221, 2.574251347313722516 ) ) ;
#22455=CARTESIAN_POINT ( 'NONE',  ( 4.458734124999999437, -151.6250000013655779, -1.846868145590734978 ) ) ;
#22456=CARTESIAN_POINT ( 'NONE',  ( 4.458734124999998549, 17.27083333469892779, -2.574251347313721627 ) ) ;
#22457=EDGE_CURVE ( 'NONE', #7439, #12164, #49820, .T. ) ;
#22459=CARTESIAN_POINT ( 'NONE',  ( -4.999999999999998224, -43.79166666393546592, 2.886751345948131764 ) ) ;
#22460=DIRECTION ( 'NONE',  ( -0.000000000000000000, 1.000000000000000000, -0.000000000000000000 ) ) ;
#22461=CARTESIAN_POINT ( 'NONE',  ( 4.458734125000000326, -83.14583333196773651, 2.574251347313718519 ) ) ;
#22464=CARTESIAN_POINT ( 'NONE',  ( 5.000000000000000000, 16.62500000273118417, -6.123233995736766282E-16 ) ) ;
#22465=ORIENTED_EDGE ( 'NONE', *, *, #48881, .T. ) ;
#22467=VECTOR ( 'NONE', #17433, 1000.000000000000000 ) ;
#22470=CARTESIAN_POINT ( 'NONE',  ( 2.499999999999998668, -25.33333333333333215, -4.330127018922193649 ) ) ;
#22471=CARTESIAN_POINT ( 'NONE',  ( 2.229367062499998831, -25.64583333196773651, -3.861377020970580887 ) ) ;
#22472=VECTOR ( 'NONE', #51195, 1000.000000000000000 ) ;
#22473=ADVANCED_FACE ( 'NONE', ( #41259 ), #40945, .T. ) ;
#22474=CARTESIAN_POINT ( 'NONE',  ( -2.500000000000000444, -30.04166666393548013, -4.330127018922193649 ) ) ;
#22476=CARTESIAN_POINT ( 'NONE',  ( -2.229367062499996610, -62.14583333196774362, 3.861377020970582219 ) ) ;
#22477=VERTEX_POINT ( 'NONE', #35187 ) ;
#22478=EDGE_CURVE ( 'NONE', #37963, #14479, #62991, .T. ) ;
#22479=CARTESIAN_POINT ( 'NONE',  ( 2.229367062499998831, -10.89583333196773829, -3.861377020970580887 ) ) ;
#22480=ORIENTED_EDGE ( 'NONE', *, *, #61048, .T. ) ;
#22481=CARTESIAN_POINT ( 'NONE',  ( 2.500000000000002220, -69.66666666666667140, 4.330127018922192761 ) ) ;
#22484=CARTESIAN_POINT ( 'NONE',  ( 2.499999999999998668, -76.20833333060214443, -4.330127018922193649 ) ) ;
#22485=CARTESIAN_POINT ( 'NONE',  ( 1.975475456537005874E-15, -65.62499999726881583, 5.000000000000000000 ) ) ;
#22486=ORIENTED_EDGE ( 'NONE', *, *, #16075, .F. ) ;
#22488=CARTESIAN_POINT ( 'NONE',  ( 4.458734125000001214, -15.14583333196773651, 2.574251347313718519 ) ) ;
#22489=CARTESIAN_POINT ( 'NONE',  ( -2.229367062499996610, -58.39583333196773651, 3.861377020970582219 ) ) ;
#22490=CARTESIAN_POINT ( 'NONE',  ( -1.339745962155610925, -23.79465819873851729, 5.000000000000000000 ) ) ;
#22491=CARTESIAN_POINT ( 'NONE',  ( 2.730187237215162345E-16, -141.1875000013656063, -4.458734124999999437 ) ) ;
#22494=ORIENTED_EDGE ( 'NONE', *, *, #54891, .F. ) ;
#22500=CARTESIAN_POINT ( 'NONE',  ( 4.458734124999999437, -149.7500000013656063, 1.846868145590737864 ) ) ;
#22504=CARTESIAN_POINT ( 'NONE',  ( 2.229367062499998831, -63.89583333196772941, -3.861377020970580887 ) ) ;
#22506=CARTESIAN_POINT ( 'NONE',  ( -2.500000000000000444, -43.04166666393548013, -4.330127018922193649 ) ) ;
#22507=CARTESIAN_POINT ( 'NONE',  ( 4.458734124999999437, -146.4375000013656063, 0.000000000000000000 ) ) ;
#22510=ORIENTED_EDGE ( 'NONE', *, *, #47211, .T. ) ;
#22515=CARTESIAN_POINT ( 'NONE',  ( 0.000000000000000000, -170.0000000000000000, 0.000000000000000000 ) ) ;
#22518=CARTESIAN_POINT ( 'NONE',  ( -2.229367062499996610, 27.60416666803225993, 3.861377020970582219 ) ) ;
#22524=CARTESIAN_POINT ( 'NONE',  ( 6.123233995736766282E-16, -170.0000000000000000, -5.000000000000000000 ) ) ;
#22525=CARTESIAN_POINT ( 'NONE',  ( 2.229367062500001939, 8.020833334698926009, 3.861377020970579999 ) ) ;
#22527=CARTESIAN_POINT ( 'NONE',  ( -4.458734124999999437, -20.64583333196774007, -2.574251347313719407 ) ) ;
#22529=CARTESIAN_POINT ( 'NONE',  ( 3.152801135295366208, -158.5625000013656063, 3.152801135295367985 ) ) ;
#22530=CARTESIAN_POINT ( 'NONE',  ( -5.000000000000000000, 29.12500000273118417, 0.000000000000000000 ) ) ;
#22535=CARTESIAN_POINT ( 'NONE',  ( -4.458734124999999437, -38.39583333196773651, -2.574251347313719407 ) ) ;
#22536=EDGE_CURVE ( 'NONE', #7188, #54337, #26164, .T. ) ;
#22538=CARTESIAN_POINT ( 'NONE',  ( 9.457646018065525792E-16, -65.31249999863440792, 5.148502694627439702 ) ) ;
#22541=CARTESIAN_POINT ( 'NONE',  ( 3.535533905932736864, -152.2500000027312126, 3.535533905932738641 ) ) ;
#22543=CARTESIAN_POINT ( 'NONE',  ( -1.339745962155613812, -68.08034179853028434, -5.000000000000000000 ) ) ;
#22544=CARTESIAN_POINT ( 'NONE',  ( 2.499999999999998668, -6.333333333333336590, -4.330127018922193649 ) ) ;
#22545=CARTESIAN_POINT ( 'NONE',  ( 4.458734124999998549, -72.72916666530107932, -2.574251347313721627 ) ) ;
#22547=CARTESIAN_POINT ( 'NONE',  ( -5.000000000000000000, -14.95833333060214265, -2.886751345948128211 ) ) ;
#22548=CARTESIAN_POINT ( 'NONE',  ( -4.458734124999999437, -47.31249999863440792, 0.000000000000000000 ) ) ;
#22550=CARTESIAN_POINT ( 'NONE',  ( -5.000000000000000000, 30.00000000000000000, 0.000000000000000000 ) ) ;
#22551=CARTESIAN_POINT ( 'NONE',  ( 4.458734124999998549, 5.020833334698926897, -2.574251347313721627 ) ) ;
#22552=ORIENTED_EDGE ( 'NONE', *, *, #40483, .F. ) ;
#22553=CARTESIAN_POINT ( 'NONE',  ( 5.000000000000000888, -34.45833333060213732, 2.886751345948126879 ) ) ;
#22554=CARTESIAN_POINT ( 'NONE',  ( -2.500000000000000444, -58.16666666666665719, -4.330127018922193649 ) ) ;
#22555=ADVANCED_FACE ( 'NONE', ( #36137 ), #54485, .T. ) ;
#22556=CARTESIAN_POINT ( 'NONE',  ( -4.458734125000001214, -161.1250000013656063, 1.846868145590734089 ) ) ;
#22560=CARTESIAN_POINT ( 'NONE',  ( 4.458734124999999437, -78.81249999863440792, -5.460374474430324690E-16 ) ) ;
#22561=CARTESIAN_POINT ( 'NONE',  ( -9.184850993605147944E-16, -167.2500000000000000, 5.000000000000000000 ) ) ;
#22563=CARTESIAN_POINT ( 'NONE',  ( 2.229367062499998831, -89.64583333196773651, -3.861377020970580887 ) ) ;
#22566=CARTESIAN_POINT ( 'NONE',  ( 2.229367062499998831, -1.895833331967737623, -3.861377020970580887 ) ) ;
#22567=CARTESIAN_POINT ( 'NONE',  ( 4.458734125000001214, -40.14583333196772941, 2.574251347313718519 ) ) ;
#22568=EDGE_CURVE ( 'NONE', #5292, #48949, #49930, .T. ) ;
#22571=CARTESIAN_POINT ( 'NONE',  ( 1.339745962155615144, -84.70534180126146850, 4.999999999999999112 ) ) ;
#22573=CARTESIAN_POINT ( 'NONE',  ( 3.061616997868383141E-16, -148.8750000027312126, -5.000000000000000000 ) ) ;
#22575=CARTESIAN_POINT ( 'NONE',  ( -4.458734124999998549, -70.47916666530107932, 2.574251347313722516 ) ) ;
#22578=ORIENTED_EDGE ( 'NONE', *, *, #62482, .F. ) ;
#22579=FACE_OUTER_BOUND ( 'NONE', #10817, .T. ) ;
#22582=CARTESIAN_POINT ( 'NONE',  ( -1.339745962155613812, 2.794658198738520394, -5.000000000000000000 ) ) ;
#22583=CARTESIAN_POINT ( 'NONE',  ( -3.152548672688508926E-16, 2.437500001365594304, -5.148502694627439702 ) ) ;
#22584=DIRECTION ( 'NONE',  ( -0.000000000000000000, 1.000000000000000000, -0.000000000000000000 ) ) ;
#22585=CARTESIAN_POINT ( 'NONE',  ( -1.846868145590737420, -158.7500000013656063, 4.458734124999997661 ) ) ;
#22586=( BOUNDED_CURVE ( )  B_SPLINE_CURVE ( 2, ( #59041, #59363, #14971, #54212, #3985, #19710, #38686, #19067, #53492 ),
 .UNSPECIFIED., .F., .F. ) 
 B_SPLINE_CURVE_WITH_KNOTS ( ( 3, 2, 2, 2, 3 ),
 ( 0.4020833333333333481, 0.4027777777777777901, 0.4041666666666666741, 0.4055555555555555580, 0.4062500000000000000 ),
 .UNSPECIFIED. ) 
 CURVE ( )  GEOMETRIC_REPRESENTATION_ITEM ( )  RATIONAL_B_SPLINE_CURVE ( ( 0.9330127018922194093, 0.9330127018922194093, 1.000000000000000000, 0.8660254037844387076, 1.000000000000000000, 0.8660254037844387076, 1.000000000000000000, 0.9330127018922194093, 0.9330127018922194093 ) ) 
 REPRESENTATION_ITEM ( '' )  );
#22593=CARTESIAN_POINT ( 'NONE',  ( -9.184850993605147944E-16, -142.3750000027312126, 5.000000000000000000 ) ) ;
#22594=CARTESIAN_POINT ( 'NONE',  ( 5.000000000000000888, -67.58333333333332860, 2.886751345948126879 ) ) ;
#22596=CARTESIAN_POINT ( 'NONE',  ( -6.972266317189433020E-16, 5.875000002731185056, -5.000000000000000000 ) ) ;
#22599=CARTESIAN_POINT ( 'NONE',  ( 4.458734124999999437, 21.18750000136559208, -5.460374474430324690E-16 ) ) ;
#22601=CARTESIAN_POINT ( 'NONE',  ( -2.229367062500000163, -1.729166665301071992, -3.861377020970580443 ) ) ;
#22604=CARTESIAN_POINT ( 'NONE',  ( 3.535533905932736864, -140.2500000027311842, 3.535533905932738641 ) ) ;
#22605=CARTESIAN_POINT ( 'NONE',  ( 2.499999999999998668, -75.20833333060214443, -4.330127018922193649 ) ) ;
#22613=CARTESIAN_POINT ( 'NONE',  ( -1.846868145590734756, -158.3750000013655779, -4.458734124999999437 ) ) ;
#22616=EDGE_LOOP ( 'NONE', ( #570, #21291, #56738, #49647 ) ) ;
#22617=CARTESIAN_POINT ( 'NONE',  ( -2.229367062499996610, 19.60416666803225993, 3.861377020970582219 ) ) ;
#22623=CARTESIAN_POINT ( 'NONE',  ( 5.000000000000000888, 6.416666666666666963, 2.886751345948126879 ) ) ;
#22624=CARTESIAN_POINT ( 'NONE',  ( 2.229367062499998831, -54.64583333196773651, -3.861377020970580887 ) ) ;
#22627=CARTESIAN_POINT ( 'NONE',  ( 0.000000000000000000, -170.0000000000000000, 0.000000000000000000 ) ) ;
#22628=CARTESIAN_POINT ( 'NONE',  ( -9.184850993605147944E-16, -153.3750000027311842, 5.000000000000000000 ) ) ;
#22629=DIRECTION ( 'NONE',  ( 0.000000000000000000, 0.000000000000000000, 1.000000000000000000 ) ) ;
#22630=CARTESIAN_POINT ( 'NONE',  ( -5.000000000000000000, -37.08333333333332860, -2.886751345948128211 ) ) ;
#22631=CARTESIAN_POINT ( 'NONE',  ( -2.500000000000000444, 12.95833333606451809, -4.330127018922193649 ) ) ;
#22634=CARTESIAN_POINT ( 'NONE',  ( -5.000000000000000888, -143.4375000000000284, 2.071067811865474617 ) ) ;
#22635=CARTESIAN_POINT ( 'NONE',  ( 2.229367062500001939, -62.97916666530106511, 3.861377020970579999 ) ) ;
#22636=( BOUNDED_CURVE ( )  B_SPLINE_CURVE ( 2, ( #34483, #19707, #14874, #20026, #43509, #53180, #54117, #33558, #9113 ),
 .UNSPECIFIED., .F., .F. ) 
 B_SPLINE_CURVE_WITH_KNOTS ( ( 3, 2, 2, 2, 3 ),
 ( 0.5770833333333332815, 0.5777777777777777235, 0.5791666666666667185, 0.5805555555555556024, 0.5812500000000000444 ),
 .UNSPECIFIED. ) 
 CURVE ( )  GEOMETRIC_REPRESENTATION_ITEM ( )  RATIONAL_B_SPLINE_CURVE ( ( 0.9330127018922194093, 0.9330127018922194093, 1.000000000000000000, 0.8660254037844387076, 1.000000000000000000, 0.8660254037844387076, 1.000000000000000000, 0.9330127018922194093, 0.9330127018922194093 ) ) 
 REPRESENTATION_ITEM ( '' )  );
#22637=CARTESIAN_POINT ( 'NONE',  ( 4.458734124999999437, -146.6875000013656063, 0.000000000000000000 ) ) ;
#22638=CARTESIAN_POINT ( 'NONE',  ( 4.458734124999998549, -71.72916666530107932, -2.574251347313721627 ) ) ;
#22640=CARTESIAN_POINT ( 'NONE',  ( -4.458734124999999437, -18.64583333196774007, -2.574251347313719407 ) ) ;
#22641=CARTESIAN_POINT ( 'NONE',  ( -5.000000000000000000, -62.87499999726880873, 0.000000000000000000 ) ) ;
#22643=CARTESIAN_POINT ( 'NONE',  ( -3.535533905932738641, -150.3750000000000000, 3.535533905932737309 ) ) ;
#22644=ORIENTED_EDGE ( 'NONE', *, *, #26730, .T. ) ;
#22646=CARTESIAN_POINT ( 'NONE',  ( 2.499999999999998668, -21.20833333060214798, -4.330127018922193649 ) ) ;
#22648=ORIENTED_EDGE ( 'NONE', *, *, #48778, .T. ) ;
#22652=CARTESIAN_POINT ( 'NONE',  ( 5.000000000000000000, -8.500000000000000000, -6.123233995736766282E-16 ) ) ;
#22653=VECTOR ( 'NONE', #27106, 1000.000000000000000 ) ;
#22654=CARTESIAN_POINT ( 'NONE',  ( -3.152548672688508926E-16, -51.81249999863440792, -5.148502694627439702 ) ) ;
#22658=CARTESIAN_POINT ( 'NONE',  ( 9.457646018065525792E-16, 18.93750000136559208, 5.148502694627439702 ) ) ;
#22661=CARTESIAN_POINT ( 'NONE',  ( 2.071067811865412445, -164.8125000000000284, -5.000000000000063949 ) ) ;
#22662=VERTEX_POINT ( 'NONE', #61544 ) ;
#22664=CARTESIAN_POINT ( 'NONE',  ( -5.000000000000000000, -39.99999999999999289, 0.000000000000000000 ) ) ;
#22671=CARTESIAN_POINT ( 'NONE',  ( 0.000000000000000000, -170.0000000000000000, 5.000000000000000000 ) ) ;
#22676=CARTESIAN_POINT ( 'NONE',  ( 0.000000000000000000, -170.0000000000000000, 0.000000000000000000 ) ) ;
#22678=CARTESIAN_POINT ( 'NONE',  ( -2.071067811865475061, -154.8125000027312126, -5.000000000000000888 ) ) ;
#22684=CARTESIAN_POINT ( 'NONE',  ( -2.071067811865478170, -145.3125000000000000, 5.000000000000000000 ) ) ;
#22687=CARTESIAN_POINT ( 'NONE',  ( 1.339745962155609149, 22.41965820146970501, 5.000000000000003553 ) ) ;
#22688=CARTESIAN_POINT ( 'NONE',  ( 4.458734124999999437, -25.81249999863440792, -5.460374474430324690E-16 ) ) ;
#22689=CARTESIAN_POINT ( 'NONE',  ( 5.000000000000000888, -146.9375000000000000, -2.071067811865475505 ) ) ;
#22692=CARTESIAN_POINT ( 'NONE',  ( 4.458734125000000326, -147.3750000013656063, -1.846868145590734978 ) ) ;
#22693=VERTEX_POINT ( 'NONE', #51568 ) ;
#22696=CARTESIAN_POINT ( 'NONE',  ( 4.458734124999998549, -53.97916666530107221, -2.574251347313721627 ) ) ;
#22697=EDGE_CURVE ( 'NONE', #52288, #18740, #3629, .T. ) ;
#22699=CARTESIAN_POINT ( 'NONE',  ( 0.000000000000000000, -170.0000000000000000, 0.000000000000000000 ) ) ;
#22700=CARTESIAN_POINT ( 'NONE',  ( 2.499999999999998668, 22.66666666666666430, -4.330127018922193649 ) ) ;
#22701=VECTOR ( 'NONE', #48065, 1000.000000000000000 ) ;
#22702=CARTESIAN_POINT ( 'NONE',  ( 1.339745962155615144, -17.58034179853029499, 4.999999999999999112 ) ) ;
#22703=CARTESIAN_POINT ( 'NONE',  ( 4.458734125000001214, -2.895833331967738289, 2.574251347313718519 ) ) ;
#22706=CARTESIAN_POINT ( 'NONE',  ( -2.229367062499996610, 7.604166668032260823, 3.861377020970582219 ) ) ;
#22708=CARTESIAN_POINT ( 'NONE',  ( 2.499999999999998668, -42.33333333333333570, -4.330127018922193649 ) ) ;
#22709=ORIENTED_EDGE ( 'NONE', *, *, #56962, .F. ) ;
#22710=CARTESIAN_POINT ( 'NONE',  ( -5.000000000000000000, -23.95833333060214443, -2.886751345948128211 ) ) ;
#22711=CARTESIAN_POINT ( 'NONE',  ( -4.458734124999999437, -47.39583333196774362, -2.574251347313719407 ) ) ;
#22712=CARTESIAN_POINT ( 'NONE',  ( 3.152801135295366208, -158.8125000013656063, 3.152801135295367985 ) ) ;
#22713=( BOUNDED_CURVE ( )  B_SPLINE_CURVE ( 2, ( #24767, #14785, #5783, #29577, #45343, #35063, #44371, #34734, #25403 ),
 .UNSPECIFIED., .F., .F. ) 
 B_SPLINE_CURVE_WITH_KNOTS ( ( 3, 2, 2, 2, 3 ),
 ( 0.7645833333333332815, 0.7652777777777777235, 0.7666666666666667185, 0.7680555555555556024, 0.7687500000000000444 ),
 .UNSPECIFIED. ) 
 CURVE ( )  GEOMETRIC_REPRESENTATION_ITEM ( )  RATIONAL_B_SPLINE_CURVE ( ( 0.9330127018922194093, 0.9330127018922194093, 1.000000000000000000, 0.8660254037844387076, 1.000000000000000000, 0.8660254037844387076, 1.000000000000000000, 0.9330127018922194093, 0.9330127018922194093 ) ) 
 REPRESENTATION_ITEM ( '' )  );
#22714=CARTESIAN_POINT ( 'NONE',  ( 1.060575238724906964E-15, -43.62499999726880873, 5.773502691896257311 ) ) ;
#22716=CARTESIAN_POINT ( 'NONE',  ( -2.229367062499996610, -21.14583333196774007, 3.861377020970582219 ) ) ;
#22717=EDGE_LOOP ( 'NONE', ( #61787, #11042, #61191, #47903 ) ) ;
#22718=CARTESIAN_POINT ( 'NONE',  ( 1.975475456537005874E-15, -13.62499999726881228, 5.000000000000000000 ) ) ;
#22719=CARTESIAN_POINT ( 'NONE',  ( -8.190561711645485556E-16, -164.6875000013655779, 4.458734124999999437 ) ) ;
#22722=CARTESIAN_POINT ( 'NONE',  ( 9.457646018065525792E-16, -36.31249999863440792, 5.148502694627439702 ) ) ;
#22724=ORIENTED_EDGE ( 'NONE', *, *, #53156, .F. ) ;
#22727=CARTESIAN_POINT ( 'NONE',  ( 3.061616997868383141E-16, -155.7500000000000000, -5.000000000000000000 ) ) ;
#22728=ORIENTED_EDGE ( 'NONE', *, *, #58256, .T. ) ;
#22729=CARTESIAN_POINT ( 'NONE',  ( -2.499999999999996447, -22.70833333060214443, 4.330127018922195425 ) ) ;
#22731=CARTESIAN_POINT ( 'NONE',  ( -2.229367062499996610, -84.39583333196773651, 3.861377020970582219 ) ) ;
#22735=CARTESIAN_POINT ( 'NONE',  ( 3.535533905932738197, -145.0000000027311842, -3.535533905932738197 ) ) ;
#22737=CARTESIAN_POINT ( 'NONE',  ( -1.339745962155610925, -84.66965819600731891, 5.000000000000000000 ) ) ;
#22738=AXIS2_PLACEMENT_3D ( 'NONE', #46546, #45903, #1865 ) ;
#22742=CARTESIAN_POINT ( 'NONE',  ( 3.535533905932736864, -159.2500000027312126, 3.535533905932738641 ) ) ;
#22745=CARTESIAN_POINT ( 'NONE',  ( -5.000000000000000000, -153.6250000027312126, -6.123233995736766282E-16 ) ) ;
#22747=CARTESIAN_POINT ( 'NONE',  ( -2.229367062499996610, -78.39583333196773651, 3.861377020970582219 ) ) ;
#22753=CARTESIAN_POINT ( 'NONE',  ( 5.000000000000000000, -166.1875000027311842, 2.071067811865478614 ) ) ;
#22755=CARTESIAN_POINT ( 'NONE',  ( 2.229367062499998831, 10.10416666803225993, -3.861377020970580887 ) ) ;
#22763=( BOUNDED_CURVE ( )  B_SPLINE_CURVE ( 2, ( #31062, #7591, #51654, #12406, #41028, #50370, #46184, #27199, #11443 ),
 .UNSPECIFIED., .F., .F. ) 
 B_SPLINE_CURVE_WITH_KNOTS ( ( 3, 2, 2, 2, 3 ),
 ( 0.2750000000000002442, 0.2791666666666668961, 0.2833333333333335480, 0.2875000000000001998, 0.2916666666666669072 ),
 .UNSPECIFIED. ) 
 CURVE ( )  GEOMETRIC_REPRESENTATION_ITEM ( )  RATIONAL_B_SPLINE_CURVE ( ( 0.9999999999999958922, 0.9238795325112908463, 1.000000000000000000, 0.9238795325112867385, 1.000000000000000000, 0.9238795325112867385, 1.000000000000000000, 0.9238795325112826307, 1.000000000000003997 ) ) 
 REPRESENTATION_ITEM ( '' )  );
#22765=CARTESIAN_POINT ( 'NONE',  ( -4.999999999999998224, -21.79166666393548368, 2.886751345948131764 ) ) ;
#22766=CARTESIAN_POINT ( 'NONE',  ( 4.458734124999999437, -6.812499998634404363, -5.460374474430324690E-16 ) ) ;
#22768=CARTESIAN_POINT ( 'NONE',  ( 4.458734124999998549, -35.97916666530107221, -2.574251347313721627 ) ) ;
#22770=CARTESIAN_POINT ( 'NONE',  ( 6.123233995736766282E-16, -170.0000000000000000, -5.000000000000000000 ) ) ;
#22774=CARTESIAN_POINT ( 'NONE',  ( -4.458734124999999437, 13.68750000136559386, 0.000000000000000000 ) ) ;
#22776=CARTESIAN_POINT ( 'NONE',  ( 1.975475456537005874E-15, -87.75000000000001421, 5.000000000000000000 ) ) ;
#22777=CARTESIAN_POINT ( 'NONE',  ( 9.457646018065525792E-16, -83.31249999863440792, 5.148502694627439702 ) ) ;
#22779=CARTESIAN_POINT ( 'NONE',  ( 5.000000000000000000, -72.37499999726880162, -6.123233995736766282E-16 ) ) ;
#22780=CARTESIAN_POINT ( 'NONE',  ( 1.060575238724906964E-15, 17.37500000273118417, 5.773502691896257311 ) ) ;
#22785=CARTESIAN_POINT ( 'NONE',  ( -4.999999999999999112, -27.91666666666666430, 2.886751345948131764 ) ) ;
#22786=CARTESIAN_POINT ( 'NONE',  ( -2.229367062500000163, -30.47916666530107221, -3.861377020970580443 ) ) ;
#22789=CARTESIAN_POINT ( 'NONE',  ( 2.500000000000002220, -29.54166666393548013, 4.330127018922192761 ) ) ;
#22791=CARTESIAN_POINT ( 'NONE',  ( -2.229367062499996610, -61.14583333196774362, 3.861377020970582219 ) ) ;
#22792=ORIENTED_EDGE ( 'NONE', *, *, #25492, .T. ) ;
#22793=CARTESIAN_POINT ( 'NONE',  ( 5.000000000000000888, -62.45833333060213732, 2.886751345948126879 ) ) ;
#22794=CARTESIAN_POINT ( 'NONE',  ( -2.229367062499996610, -9.395833331967736513, 3.861377020970582219 ) ) ;
#22795=ORIENTED_EDGE ( 'NONE', *, *, #57754, .T. ) ;
#22796=CARTESIAN_POINT ( 'NONE',  ( -3.535250795749689387E-16, -78.25000000000001421, -5.773502691896257311 ) ) ;
#22799=CARTESIAN_POINT ( 'NONE',  ( -5.000000000000000000, -76.87499999726880162, 0.000000000000000000 ) ) ;
#22801=ORIENTED_EDGE ( 'NONE', *, *, #6782, .F. ) ;
#22803=CARTESIAN_POINT ( 'NONE',  ( 9.457646018065525792E-16, -19.31249999863440792, 5.148502694627439702 ) ) ;
#22804=CARTESIAN_POINT ( 'NONE',  ( 9.457646018065525792E-16, -55.31249999863439371, 5.148502694627439702 ) ) ;
#22806=SHAPE_REPRESENTATION_RELATIONSHIP ( 'NONE' , 'NONE' ,  #25037, #3382 ) ;
#22807=CARTESIAN_POINT ( 'NONE',  ( -1.846868145590737420, -169.0000000013655779, 4.458734124999999437 ) ) ;
#22809=CARTESIAN_POINT ( 'NONE',  ( 5.000000000000000888, -148.0625000027312126, -2.071067811865475505 ) ) ;
#22813=( BOUNDED_CURVE ( )  B_SPLINE_CURVE ( 2, ( #20348, #15528, #44137, #48962, #35461, #14870, #35148, #49295, #30626 ),
 .UNSPECIFIED., .F., .F. ) 
 B_SPLINE_CURVE_WITH_KNOTS ( ( 3, 2, 2, 2, 3 ),
 ( 0.4687500000000000000, 0.4694444444444444420, 0.4708333333333333259, 0.4722222222222222099, 0.4729166666666666519 ),
 .UNSPECIFIED. ) 
 CURVE ( )  GEOMETRIC_REPRESENTATION_ITEM ( )  RATIONAL_B_SPLINE_CURVE ( ( 0.9330127018922194093, 0.9330127018922194093, 1.000000000000000000, 0.8660254037844387076, 1.000000000000000000, 0.8660254037844387076, 1.000000000000000000, 0.9330127018922194093, 0.9330127018922194093 ) ) 
 REPRESENTATION_ITEM ( '' )  );
#22814=CARTESIAN_POINT ( 'NONE',  ( 1.975475456537005874E-15, -29.74999999999999645, 5.000000000000000000 ) ) ;
#22820=CARTESIAN_POINT ( 'NONE',  ( 3.152801135295367541, -149.5625000013655779, -3.152801135295367541 ) ) ;
#22822=DIRECTION ( 'NONE',  ( -0.000000000000000000, 1.000000000000000000, -0.000000000000000000 ) ) ;
#22824=CARTESIAN_POINT ( 'NONE',  ( -3.152548672688508926E-16, -61.81249999863440081, -5.148502694627439702 ) ) ;
#22826=CARTESIAN_POINT ( 'NONE',  ( 1.975475456537005874E-15, -42.62499999726880873, 5.000000000000000000 ) ) ;
#22827=CARTESIAN_POINT ( 'NONE',  ( -4.458734124999999437, -147.0000000013656063, -1.846868145590735644 ) ) ;
#22836=CARTESIAN_POINT ( 'NONE',  ( -4.458734124999999437, 26.43750000136559564, 0.000000000000000000 ) ) ;
#22837=DIRECTION ( 'NONE',  ( 0.000000000000000000, 0.000000000000000000, 1.000000000000000000 ) ) ;
#22840=DIRECTION ( 'NONE',  ( -0.000000000000000000, 1.000000000000000000, -0.000000000000000000 ) ) ;
#22841=EDGE_CURVE ( 'NONE', #15636, #44762, #26092, .T. ) ;
#22843=CARTESIAN_POINT ( 'NONE',  ( -2.229367062500000163, 9.520833334698927786, -3.861377020970580443 ) ) ;
#22845=CARTESIAN_POINT ( 'NONE',  ( -2.229367062500000163, -19.72916666530107221, -3.861377020970580443 ) ) ;
#22847=CARTESIAN_POINT ( 'NONE',  ( -3.152801135295367096, -160.0625000013656063, -3.152801135295367541 ) ) ;
#22848=CARTESIAN_POINT ( 'NONE',  ( 1.975475456537005874E-15, -67.62499999726881583, 5.000000000000000000 ) ) ;
#22852=CARTESIAN_POINT ( 'NONE',  ( -4.458734124999999437, -42.31249999863440081, 0.000000000000000000 ) ) ;
#22854=CARTESIAN_POINT ( 'NONE',  ( 2.229367062500001939, -65.22916666530106511, 3.861377020970579999 ) ) ;
#22858=VERTEX_POINT ( 'NONE', #48300 ) ;
#22861=CARTESIAN_POINT ( 'NONE',  ( -5.000000000000000000, -11.08333333333333393, -2.886751345948128211 ) ) ;
#22862=CARTESIAN_POINT ( 'NONE',  ( -4.458734124999999437, -16.39583333196773651, -2.574251347313719407 ) ) ;
#22863=CARTESIAN_POINT ( 'NONE',  ( -4.458734124999999437, -78.39583333196772230, -2.574251347313719407 ) ) ;
#22865=CARTESIAN_POINT ( 'NONE',  ( 2.500000000000002220, -11.54166666393547835, 4.330127018922192761 ) ) ;
#22866=CARTESIAN_POINT ( 'NONE',  ( 2.229367062499998831, -42.64583333196773651, -3.861377020970580887 ) ) ;
#22867=ORIENTED_EDGE ( 'NONE', *, *, #59743, .F. ) ;
#22868=CARTESIAN_POINT ( 'NONE',  ( 2.229367062499998831, 9.104166668032261711, -3.861377020970580887 ) ) ;
#22871=CARTESIAN_POINT ( 'NONE',  ( 5.000000000000000000, -55.49999999999999289, -6.123233995736766282E-16 ) ) ;
#22872=CARTESIAN_POINT ( 'NONE',  ( -8.190561711645485556E-16, -159.9375000013655779, 4.458734124999999437 ) ) ;
#22875=CARTESIAN_POINT ( 'NONE',  ( -3.152548672688508926E-16, -81.56249999863440792, -5.148502694627439702 ) ) ;
#22876=CARTESIAN_POINT ( 'NONE',  ( 2.071067811865476394, -165.1875000000000000, 5.000000000000000000 ) ) ;
#22877=CARTESIAN_POINT ( 'NONE',  ( 5.000000000000000888, 5.541666669397853795, 2.886751345948126879 ) ) ;
#22879=CARTESIAN_POINT ( 'NONE',  ( -2.229367062500000163, -1.729166665301071992, -3.861377020970580443 ) ) ;
#22880=CARTESIAN_POINT ( 'NONE',  ( -3.152548672688508926E-16, -42.81249999863440081, -5.148502694627439702 ) ) ;
#22883=CARTESIAN_POINT ( 'NONE',  ( 2.499999999999998668, -84.33333333333332860, -4.330127018922193649 ) ) ;
#22884=ORIENTED_EDGE ( 'NONE', *, *, #8025, .T. ) ;
#22885=CARTESIAN_POINT ( 'NONE',  ( -9.184850993605147944E-16, -141.2500000000000284, 5.000000000000000000 ) ) ;
#22887=CARTESIAN_POINT ( 'NONE',  ( 2.229367062500001939, -71.22916666530107932, 3.861377020970579999 ) ) ;
#22889=VERTEX_POINT ( 'NONE', #8761 ) ;
#22890=( BOUNDED_CURVE ( )  B_SPLINE_CURVE ( 2, ( #745, #45754, #31593, #44785, #56048, #25818, #60561, #31264, #16800 ),
 .UNSPECIFIED., .F., .F. ) 
 B_SPLINE_CURVE_WITH_KNOTS ( ( 3, 2, 2, 2, 3 ),
 ( 0.8354166666666666963, 0.8361111111111111382, 0.8375000000000000222, 0.8388888888888889062, 0.8395833333333333481 ),
 .UNSPECIFIED. ) 
 CURVE ( )  GEOMETRIC_REPRESENTATION_ITEM ( )  RATIONAL_B_SPLINE_CURVE ( ( 0.9330127018922194093, 0.9330127018922194093, 1.000000000000000000, 0.8660254037844387076, 1.000000000000000000, 0.8660254037844387076, 1.000000000000000000, 0.9330127018922194093, 0.9330127018922194093 ) ) 
 REPRESENTATION_ITEM ( '' )  );
#22891=CARTESIAN_POINT ( 'NONE',  ( 2.499999999999998668, -5.333333333333335702, -4.330127018922193649 ) ) ;
#22892=EDGE_CURVE ( 'NONE', #24529, #31402, #10013, .T. ) ;
#22893=EDGE_CURVE ( 'NONE', #16274, #48010, #28680, .T. ) ;
#22894=CARTESIAN_POINT ( 'NONE',  ( 5.000000000000000000, -3.374999997268816276, -6.123233995736766282E-16 ) ) ;
#22898=CARTESIAN_POINT ( 'NONE',  ( 9.457646018065525792E-16, 1.937500001365593416, 5.148502694627439702 ) ) ;
#22899=CARTESIAN_POINT ( 'NONE',  ( -2.500000000000000444, -80.16666666666665719, -4.330127018922193649 ) ) ;
#22900=CARTESIAN_POINT ( 'NONE',  ( 2.730187237215162345E-16, -158.1875000013655779, -4.458734124999999437 ) ) ;
#22906=ADVANCED_FACE ( 'NONE', ( #34135 ), #43470, .T. ) ;
#22907=FACE_OUTER_BOUND ( 'NONE', #38534, .T. ) ;
#22908=ADVANCED_FACE ( 'NONE', ( #23867 ), #43159, .T. ) ;
#22916=CARTESIAN_POINT ( 'NONE',  ( -3.152548672688508926E-16, 21.43750000136559208, -5.148502694627439702 ) ) ;
#22917=EDGE_CURVE ( 'NONE', #19872, #20646, #52020, .T. ) ;
#22919=CARTESIAN_POINT ( 'NONE',  ( 4.458734124999999437, -6.062499998634403475, -5.460374474430324690E-16 ) ) ;
#22922=EDGE_CURVE ( 'NONE', #39751, #27115, #47498, .T. ) ;
#22923=CARTESIAN_POINT ( 'NONE',  ( 3.535533905932738197, -143.0000000027311842, -3.535533905932738197 ) ) ;
#22924=CARTESIAN_POINT ( 'NONE',  ( -2.499999999999996447, -51.83333333333332860, 4.330127018922195425 ) ) ;
#22928=LINE ( 'NONE', #53437, #37801 ) ;
#22930=CARTESIAN_POINT ( 'NONE',  ( 4.458734124999999437, -157.6875000013655779, 0.000000000000000000 ) ) ;
#22932=( LENGTH_UNIT ( ) NAMED_UNIT ( * ) SI_UNIT ( .MILLI., .METRE. ) );
#22933=ORIENTED_EDGE ( 'NONE', *, *, #10676, .F. ) ;
#22934=CARTESIAN_POINT ( 'NONE',  ( -4.458734124999999437, 17.35416666803225993, -2.574251347313719407 ) ) ;
#22939=CARTESIAN_POINT ( 'NONE',  ( 0.000000000000000000, -170.0000000000000000, 5.000000000000000000 ) ) ;
#22940=CARTESIAN_POINT ( 'NONE',  ( 2.499999999999998668, 3.666666666666665186, -4.330127018922193649 ) ) ;
#22941=CARTESIAN_POINT ( 'NONE',  ( 4.458734125000000326, -61.89583333196774362, 2.574251347313718519 ) ) ;
#22942=CARTESIAN_POINT ( 'NONE',  ( -2.500000000000000444, -8.166666666666669627, -4.330127018922193649 ) ) ;
#22944=CARTESIAN_POINT ( 'NONE',  ( -4.458734124999998549, -31.22916666530107221, 2.574251347313722516 ) ) ;
#22945=CARTESIAN_POINT ( 'NONE',  ( 1.339745962155615144, 7.419658201469705894, 4.999999999999999112 ) ) ;
#22946=CARTESIAN_POINT ( 'NONE',  ( -5.000000000000000888, -151.5625000027311842, 2.071067811865474617 ) ) ;
#22947=CARTESIAN_POINT ( 'NONE',  ( 5.000000000000000000, -37.50000000000000711, -6.123233995736766282E-16 ) ) ;
#22951=CARTESIAN_POINT ( 'NONE',  ( -2.229367062499996610, -63.14583333196774362, 3.861377020970582219 ) ) ;
#22952=CARTESIAN_POINT ( 'NONE',  ( 2.730187237215162345E-16, -148.4375000013656063, -4.458734124999999437 ) ) ;
#22953=CARTESIAN_POINT ( 'NONE',  ( -4.458734124999999437, -77.39583333196772230, -2.574251347313719407 ) ) ;
#22955=CARTESIAN_POINT ( 'NONE',  ( -2.229367062499996610, -26.39583333196774007, 3.861377020970582219 ) ) ;
#22956=CARTESIAN_POINT ( 'NONE',  ( 5.000000000000000000, -65.37499999726881583, -6.123233995736766282E-16 ) ) ;
#22962=EDGE_LOOP ( 'NONE', ( #23409, #31003, #21766, #23490 ) ) ;
#22965=CARTESIAN_POINT ( 'NONE',  ( -2.500000000000000444, -56.04166666393548013, -4.330127018922193649 ) ) ;
#22966=CARTESIAN_POINT ( 'NONE',  ( 2.229367062500001939, -51.22916666530107221, 3.861377020970579999 ) ) ;
#22970=CARTESIAN_POINT ( 'NONE',  ( 4.458734124999998549, 19.27083333469893134, -2.574251347313721627 ) ) ;
#22978=CARTESIAN_POINT ( 'NONE',  ( -6.972266317189433020E-16, -69.12499999726880162, -5.000000000000000000 ) ) ;
#22985=CYLINDRICAL_SURFACE ( 'NONE', #26407, 5.000000000000000000 ) ;
#22992=CARTESIAN_POINT ( 'NONE',  ( -5.000000000000000888, -152.5625000027312126, 2.071067811865474617 ) ) ;
#22993=ORIENTED_EDGE ( 'NONE', *, *, #23566, .F. ) ;
#22998=CARTESIAN_POINT ( 'NONE',  ( 5.000000000000000000, -145.0625000000000284, 2.071067811865478614 ) ) ;
#23002=CARTESIAN_POINT ( 'NONE',  ( 1.846868145590735200, -168.5000000013655779, -4.458734124999999437 ) ) ;
#23003=CARTESIAN_POINT ( 'NONE',  ( 2.229367062500001939, -26.97916666530106866, 3.861377020970579999 ) ) ;
#23007=CARTESIAN_POINT ( 'NONE',  ( -4.458734124999999437, -148.9375000013656063, -5.460374474430324690E-16 ) ) ;
#23009=CARTESIAN_POINT ( 'NONE',  ( 3.535533905932738197, -149.8750000000000000, -3.535533905932738197 ) ) ;
#23010=CARTESIAN_POINT ( 'NONE',  ( 2.229367062500001939, -57.22916666530107932, 3.861377020970579999 ) ) ;
#23013=CARTESIAN_POINT ( 'NONE',  ( -4.999999999999999112, 26.08333333333333215, 2.886751345948131764 ) ) ;
#23014=DIRECTION ( 'NONE',  ( -0.000000000000000000, 1.000000000000000000, -0.000000000000000000 ) ) ;
#23015=CARTESIAN_POINT ( 'NONE',  ( -2.229367062500000163, 1.520833334698927564, -3.861377020970580443 ) ) ;
#23016=CARTESIAN_POINT ( 'NONE',  ( -5.000000000000000888, -164.4375000000000284, 2.071067811865474617 ) ) ;
#23017=CARTESIAN_POINT ( 'NONE',  ( -2.229367062500000163, 11.27083333469892601, -3.861377020970580443 ) ) ;
#23019=CARTESIAN_POINT ( 'NONE',  ( -6.972266317189433020E-16, -16.25000000000000000, -5.000000000000000000 ) ) ;
#23020=VERTEX_POINT ( 'NONE', #34782 ) ;
#23021=CARTESIAN_POINT ( 'NONE',  ( 5.000000000000000888, 27.54166666939785557, 2.886751345948126879 ) ) ;
#23022=CARTESIAN_POINT ( 'NONE',  ( -2.229367062499996610, -51.14583333196772941, 3.861377020970582219 ) ) ;
#23023=CARTESIAN_POINT ( 'NONE',  ( -4.458734125000000326, -158.2500000013656063, -1.846868145590735644 ) ) ;
#23024=CARTESIAN_POINT ( 'NONE',  ( -2.499999999999996447, -45.70833333060214443, 4.330127018922195425 ) ) ;
#23026=CARTESIAN_POINT ( 'NONE',  ( 2.229367062500001939, -20.97916666530107221, 3.861377020970579999 ) ) ;
#23027=ORIENTED_EDGE ( 'NONE', *, *, #4580, .T. ) ;
#23030=CARTESIAN_POINT ( 'NONE',  ( 2.730187237215162345E-16, -160.1875000013655779, -4.458734124999999437 ) ) ;
#23031=DIRECTION ( 'NONE',  ( 0.000000000000000000, 0.000000000000000000, 1.000000000000000000 ) ) ;
#23033=CARTESIAN_POINT ( 'NONE',  ( 2.229367062499998831, -35.89583333196773651, -3.861377020970580887 ) ) ;
#23034=CARTESIAN_POINT ( 'NONE',  ( -4.999999999999998224, 17.08333333333333215, 2.886751345948131764 ) ) ;
#23035=EDGE_LOOP ( 'NONE', ( #42574, #44528, #25585, #57600 ) ) ;
#23038=CARTESIAN_POINT ( 'NONE',  ( 5.000000000000000000, -59.50000000000000000, -6.123233995736766282E-16 ) ) ;
#23039=ORIENTED_EDGE ( 'NONE', *, *, #53434, .T. ) ;
#23042=CARTESIAN_POINT ( 'NONE',  ( 2.229367062499998831, -83.89583333196773651, -3.861377020970580887 ) ) ;
#23045=CARTESIAN_POINT ( 'NONE',  ( 0.000000000000000000, -170.0000000000000000, 0.000000000000000000 ) ) ;
#23050=CARTESIAN_POINT ( 'NONE',  ( -4.999999999999998224, -81.91666666666667140, 2.886751345948131764 ) ) ;
#23053=CYLINDRICAL_SURFACE ( 'NONE', #22244, 5.000000000000000000 ) ;
#23055=CARTESIAN_POINT ( 'NONE',  ( -2.229367062499996610, -82.39583333196773651, 3.861377020970582219 ) ) ;
#23058=ORIENTED_EDGE ( 'NONE', *, *, #1366, .F. ) ;
#23059=CARTESIAN_POINT ( 'NONE',  ( -5.000000000000000000, -155.6250000027311842, -6.123233995736766282E-16 ) ) ;
#23061=CARTESIAN_POINT ( 'NONE',  ( -5.000000000000000888, -163.5625000027312126, 2.071067811865474617 ) ) ;
#23063=CARTESIAN_POINT ( 'NONE',  ( -5.000000000000000000, -16.08333333333333215, -2.886751345948128211 ) ) ;
#23068=CARTESIAN_POINT ( 'NONE',  ( -2.499999999999996447, -19.83333333333333570, 4.330127018922195425 ) ) ;
#23069=CARTESIAN_POINT ( 'NONE',  ( -5.000000000000000888, -152.4375000000000000, 2.071067811865474617 ) ) ;
#23070=CARTESIAN_POINT ( 'NONE',  ( 4.458734124999998549, -10.72916666530106866, -2.574251347313721627 ) ) ;
#23073=CARTESIAN_POINT ( 'NONE',  ( 4.458734124999999437, -34.06249999863440792, -5.460374474430324690E-16 ) ) ;
#23075=CARTESIAN_POINT ( 'NONE',  ( 1.062108568985190270E-13, -26.12499999726881583, -4.999999999999999112 ) ) ;
#23079=( BOUNDED_CURVE ( )  B_SPLINE_CURVE ( 2, ( #2874, #22490, #42086, #38434, #61728, #17657, #37273, #56900, #12819 ),
 .UNSPECIFIED., .F., .F. ) 
 B_SPLINE_CURVE_WITH_KNOTS ( ( 3, 2, 2, 2, 3 ),
 ( 0.4479166666666666852, 0.4486111111111111271, 0.4500000000000000111, 0.4513888888888888951, 0.4520833333333333370 ),
 .UNSPECIFIED. ) 
 CURVE ( )  GEOMETRIC_REPRESENTATION_ITEM ( )  RATIONAL_B_SPLINE_CURVE ( ( 0.9330127018922194093, 0.9330127018922194093, 1.000000000000000000, 0.8660254037844387076, 1.000000000000000000, 0.8660254037844387076, 1.000000000000000000, 0.9330127018922194093, 0.9330127018922194093 ) ) 
 REPRESENTATION_ITEM ( '' )  );
#23080=CARTESIAN_POINT ( 'NONE',  ( 4.458734124999999437, 13.18750000136559208, -5.460374474430324690E-16 ) ) ;
#23081=DIRECTION ( 'NONE',  ( -0.000000000000000000, 1.000000000000000000, -0.000000000000000000 ) ) ;
#23082=CARTESIAN_POINT ( 'NONE',  ( 1.339745962155612702, -55.29465819873852439, -5.000000000000000000 ) ) ;
#23083=CARTESIAN_POINT ( 'NONE',  ( -4.458734124999997661, -84.47916666530107932, 2.574251347313722516 ) ) ;
#23085=CARTESIAN_POINT ( 'NONE',  ( -2.500000000000000444, 12.95833333606451809, -4.330127018922193649 ) ) ;
#23087=CARTESIAN_POINT ( 'NONE',  ( 5.000000000000000888, -25.58333333333333215, 2.886751345948126879 ) ) ;
#23089=CARTESIAN_POINT ( 'NONE',  ( 1.339745962155615144, -52.70534180126147561, 4.999999999999999112 ) ) ;
#23090=CARTESIAN_POINT ( 'NONE',  ( -2.499999999999996447, -26.83333333333333570, 4.330127018922195425 ) ) ;
#23091=CARTESIAN_POINT ( 'NONE',  ( -4.458734124999999437, -31.31249999863440436, 0.000000000000000000 ) ) ;
#23094=CARTESIAN_POINT ( 'NONE',  ( 2.500000000000002220, -30.54166666393548013, 4.330127018922192761 ) ) ;
#23095=CARTESIAN_POINT ( 'NONE',  ( 4.458734124999998549, -59.72916666530106511, -2.574251347313721627 ) ) ;
#23096=VERTEX_POINT ( 'NONE', #39591 ) ;
#23098=CARTESIAN_POINT ( 'NONE',  ( -4.458734124999999437, -7.645833331967735624, -2.574251347313719407 ) ) ;
#23100=CARTESIAN_POINT ( 'NONE',  ( 5.000000000000000000, -74.41666666666665719, -2.886751345948129988 ) ) ;
#23103=CARTESIAN_POINT ( 'NONE',  ( 5.000000000000000000, -76.37499999726880162, -6.123233995736766282E-16 ) ) ;
#23105=ORIENTED_EDGE ( 'NONE', *, *, #1264, .F. ) ;
#23107=CARTESIAN_POINT ( 'NONE',  ( 4.458734124999998549, -22.97916666530107221, -2.574251347313721627 ) ) ;
#23108=CARTESIAN_POINT ( 'NONE',  ( -4.458734124999998549, -59.47916666530106511, 2.574251347313722516 ) ) ;
#23111=CARTESIAN_POINT ( 'NONE',  ( -1.846868145590734756, -140.1250000013655779, -4.458734125000000326 ) ) ;
#23114=ORIENTED_EDGE ( 'NONE', *, *, #23349, .T. ) ;
#23120=CARTESIAN_POINT ( 'NONE',  ( 4.458734124999999437, -145.7500000013655779, 1.846868145590737864 ) ) ;
#23124=( BOUNDED_CURVE ( )  B_SPLINE_CURVE ( 2, ( #48177, #8942, #42717, #24365, #52393, #14390, #19212, #8630, #24055 ),
 .UNSPECIFIED., .F., .F. ) 
 B_SPLINE_CURVE_WITH_KNOTS ( ( 3, 2, 2, 2, 3 ),
 ( 0.04166666666666670599, 0.04583333333333337173, 0.05000000000000004441, 0.05416666666666671709, 0.05833333333333338283 ),
 .UNSPECIFIED. ) 
 CURVE ( )  GEOMETRIC_REPRESENTATION_ITEM ( )  RATIONAL_B_SPLINE_CURVE ( ( 0.9999999999999992228, 0.9238795325112875156, 1.000000000000000000, 0.9238795325112867385, 1.000000000000000000, 0.9238795325112867385, 1.000000000000000000, 0.9238795325112858503, 1.000000000000000888 ) ) 
 REPRESENTATION_ITEM ( '' )  );
#23125=CARTESIAN_POINT ( 'NONE',  ( -4.458734124999999437, -67.56249999863440792, 0.000000000000000000 ) ) ;
#23127=CARTESIAN_POINT ( 'NONE',  ( 4.458734124999997661, -142.5000000013656063, 1.846868145590737864 ) ) ;
#23135=CARTESIAN_POINT ( 'NONE',  ( 4.458734125000000326, 25.85416666803225993, 2.574251347313718519 ) ) ;
#23136=CARTESIAN_POINT ( 'NONE',  ( -5.000000000000000000, -17.95833333060214798, -2.886751345948128211 ) ) ;
#23142=CARTESIAN_POINT ( 'NONE',  ( 4.458734124999999437, 7.187500001365594748, -5.460374474430324690E-16 ) ) ;
#23144=CARTESIAN_POINT ( 'NONE',  ( 2.229367062499998831, -21.89583333196774007, -3.861377020970580887 ) ) ;
#23146=CARTESIAN_POINT ( 'NONE',  ( -4.458734124999999437, -160.9375000013655779, -5.460374474430324690E-16 ) ) ;
#23147=CARTESIAN_POINT ( 'NONE',  ( -2.071067811865351604, -158.3125000000000284, 5.000000000000126121 ) ) ;
#23150=CARTESIAN_POINT ( 'NONE',  ( 2.229367062499998831, 29.35416666803225993, -3.861377020970580887 ) ) ;
#23151=CARTESIAN_POINT ( 'NONE',  ( -4.458734124999997661, -42.22916666530107932, 2.574251347313722516 ) ) ;
#23152=LINE ( 'NONE', #29216, #59558 ) ;
#23154=CARTESIAN_POINT ( 'NONE',  ( -2.229367062500000163, -66.72916666530106511, -3.861377020970580443 ) ) ;
#23157=CARTESIAN_POINT ( 'NONE',  ( 1.339745962155615144, -89.70534180126146850, 4.999999999999999112 ) ) ;
#23160=CARTESIAN_POINT ( 'NONE',  ( 1.339745962155612702, -6.169658196007334894, -5.000000000000000000 ) ) ;
#23161=CARTESIAN_POINT ( 'NONE',  ( -4.999999999999999112, -13.91666666666666785, 2.886751345948131764 ) ) ;
#23162=CARTESIAN_POINT ( 'NONE',  ( 9.457646018065525792E-16, -18.06249999863440436, 5.148502694627439702 ) ) ;
#23164=CARTESIAN_POINT ( 'NONE',  ( -2.229367062500000163, -77.47916666530106511, -3.861377020970580443 ) ) ;
#23166=CARTESIAN_POINT ( 'NONE',  ( 5.000000000000000000, -11.37499999726881583, -6.123233995736766282E-16 ) ) ;
#23167=CARTESIAN_POINT ( 'NONE',  ( -2.229367062499996610, -43.14583333196773651, 3.861377020970582219 ) ) ;
#23168=ORIENTED_EDGE ( 'NONE', *, *, #52386, .F. ) ;
#23170=CARTESIAN_POINT ( 'NONE',  ( -2.229367062499996610, 4.604166668032261711, 3.861377020970582219 ) ) ;
#23172=CARTESIAN_POINT ( 'NONE',  ( -5.000000000000000000, -63.08333333333332860, -2.886751345948128211 ) ) ;
#23173=CARTESIAN_POINT ( 'NONE',  ( -1.846868145590737420, -159.0000000013656063, 4.458734124999999437 ) ) ;
#23176=( BOUNDED_CURVE ( )  B_SPLINE_CURVE ( 2, ( #5815, #45372, #35727, #55356, #15788, #46008, #55989, #41486, #60817 ),
 .UNSPECIFIED., .F., .F. ) 
 B_SPLINE_CURVE_WITH_KNOTS ( ( 3, 2, 2, 2, 3 ),
 ( 0.5812500000000000444, 0.5819444444444444864, 0.5833333333333333703, 0.5847222222222222543, 0.5854166666666666963 ),
 .UNSPECIFIED. ) 
 CURVE ( )  GEOMETRIC_REPRESENTATION_ITEM ( )  RATIONAL_B_SPLINE_CURVE ( ( 0.9330127018922194093, 0.9330127018922194093, 1.000000000000000000, 0.8660254037844387076, 1.000000000000000000, 0.8660254037844387076, 1.000000000000000000, 0.9330127018922194093, 0.9330127018922194093 ) ) 
 REPRESENTATION_ITEM ( '' )  );
#23177=CARTESIAN_POINT ( 'NONE',  ( 3.061616997868383141E-16, -165.7500000000000000, -5.000000000000000000 ) ) ;
#23178=EDGE_CURVE ( 'NONE', #1738, #31328, #8443, .T. ) ;
#23179=LINE ( 'NONE', #42789, #32336 ) ;
#23181=CARTESIAN_POINT ( 'NONE',  ( 4.458734125000001214, -7.145833331967734736, 2.574251347313718519 ) ) ;
#23182=CARTESIAN_POINT ( 'NONE',  ( 2.229367062499998831, -42.89583333196773651, -3.861377020970580887 ) ) ;
#23183=CARTESIAN_POINT ( 'NONE',  ( 5.000000000000000000, -67.29166666393547303, -2.886751345948130876 ) ) ;
#23184=ADVANCED_FACE ( 'NONE', ( #10647 ), #45067, .T. ) ;
#23186=CARTESIAN_POINT ( 'NONE',  ( 2.500000000000002220, 8.333333333333332149, 4.330127018922192761 ) ) ;
#23190=CARTESIAN_POINT ( 'NONE',  ( -4.458734124999999437, -69.56249999863439371, 0.000000000000000000 ) ) ;
#23191=CARTESIAN_POINT ( 'NONE',  ( -4.458734124999999437, -148.1875000013656063, -5.460374474430324690E-16 ) ) ;
#23192=ORIENTED_EDGE ( 'NONE', *, *, #39697, .T. ) ;
#23196=CARTESIAN_POINT ( 'NONE',  ( 4.458734124999998549, 2.270833334698928230, -2.574251347313721627 ) ) ;
#23198=CARTESIAN_POINT ( 'NONE',  ( -1.846868145590737420, -154.7500000013656063, 4.458734124999997661 ) ) ;
#23200=ORIENTED_EDGE ( 'NONE', *, *, #33487, .T. ) ;
#23203=CARTESIAN_POINT ( 'NONE',  ( 2.499999999999998668, -63.33333333333332149, -4.330127018922193649 ) ) ;
#23205=ADVANCED_FACE ( 'NONE', ( #30587 ), #55040, .T. ) ;
#23206=CARTESIAN_POINT ( 'NONE',  ( -6.972266317189433020E-16, -34.25000000000000000, -5.000000000000000000 ) ) ;
#23207=CARTESIAN_POINT ( 'NONE',  ( 2.500000000000002220, -23.54166666393548368, 4.330127018922192761 ) ) ;
#23208=CARTESIAN_POINT ( 'NONE',  ( 2.499999999999998668, -87.33333333333332860, -4.330127018922193649 ) ) ;
#23210=CARTESIAN_POINT ( 'NONE',  ( 1.339745962155615144, -64.58034179853029855, 4.999999999999999112 ) ) ;
#23212=CARTESIAN_POINT ( 'NONE',  ( 5.000000000000000888, -10.58333333333333393, 2.886751345948126879 ) ) ;
#23214=CARTESIAN_POINT ( 'NONE',  ( -2.229367062499996610, 23.85416666803225993, 3.861377020970582219 ) ) ;
#23216=CARTESIAN_POINT ( 'NONE',  ( 4.458734124999998549, -4.979166665301071326, -2.574251347313721627 ) ) ;
#23219=CARTESIAN_POINT ( 'NONE',  ( -5.000000000000000888, -139.6875000027312126, -2.071067811865475949 ) ) ;
#23220=CARTESIAN_POINT ( 'NONE',  ( -1.049326080737009628E-13, -20.62499999726881583, 5.000000000000000000 ) ) ;
#23227=CARTESIAN_POINT ( 'NONE',  ( 3.152801135295366208, -157.8125000013656063, 3.152801135295367985 ) ) ;
#23231=CARTESIAN_POINT ( 'NONE',  ( -4.458734124999999437, 19.35416666803225993, -2.574251347313719407 ) ) ;
#23232=ORIENTED_EDGE ( 'NONE', *, *, #20051, .T. ) ;
#23236=AXIS2_PLACEMENT_3D ( 'NONE', #33569, #8810, #52567 ) ;
#23237=CARTESIAN_POINT ( 'NONE',  ( -5.000000000000000000, 0.9166666666666664076, -2.886751345948128211 ) ) ;
#23238=AXIS2_PLACEMENT_3D ( 'NONE', #44713, #40219, #6136 ) ;
#23239=CARTESIAN_POINT ( 'NONE',  ( 2.229367062499998831, -63.64583333196772941, -3.861377020970580887 ) ) ;
#23240=VECTOR ( 'NONE', #33639, 1000.000000000000000 ) ;
#23242=EDGE_CURVE ( 'NONE', #12417, #26245, #40556, .T. ) ;
#23244=CARTESIAN_POINT ( 'NONE',  ( 4.458734124999999437, -29.81249999863440436, -5.460374474430324690E-16 ) ) ;
#23246=CYLINDRICAL_SURFACE ( 'NONE', #10748, 5.000000000000000000 ) ;
#23247=ADVANCED_FACE ( 'NONE', ( #51181 ), #27666, .T. ) ;
#23249=CARTESIAN_POINT ( 'NONE',  ( 2.500000000000002220, -44.66666666666665719, 4.330127018922192761 ) ) ;
#23251=CARTESIAN_POINT ( 'NONE',  ( -2.500000000000000444, -45.16666666666665719, -4.330127018922193649 ) ) ;
#23253=CARTESIAN_POINT ( 'NONE',  ( 5.000000000000000000, -4.374999997268816720, -6.123233995736766282E-16 ) ) ;
#23254=CARTESIAN_POINT ( 'NONE',  ( 4.458734125000001214, -63.89583333196772941, 2.574251347313718519 ) ) ;
#23255=CARTESIAN_POINT ( 'NONE',  ( -8.190561711645485556E-16, -146.9375000013656063, 4.458734124999999437 ) ) ;
#23257=CARTESIAN_POINT ( 'NONE',  ( -4.458734124999999437, -75.31249999863440792, 0.000000000000000000 ) ) ;
#23260=( BOUNDED_CURVE ( )  B_SPLINE_CURVE ( 2, ( #55551, #36233, #61006, #26906, #12099, #7295, #40729, #26256, #21447 ),
 .UNSPECIFIED., .F., .F. ) 
 B_SPLINE_CURVE_WITH_KNOTS ( ( 3, 2, 2, 2, 3 ),
 ( 0.7479166666666666741, 0.7486111111111111160, 0.7500000000000000000, 0.7513888888888888840, 0.7520833333333333259 ),
 .UNSPECIFIED. ) 
 CURVE ( )  GEOMETRIC_REPRESENTATION_ITEM ( )  RATIONAL_B_SPLINE_CURVE ( ( 0.9330127018922194093, 0.9330127018922194093, 1.000000000000000000, 0.8660254037844387076, 1.000000000000000000, 0.8660254037844387076, 1.000000000000000000, 0.9330127018922194093, 0.9330127018922194093 ) ) 
 REPRESENTATION_ITEM ( '' )  );
#23261=CARTESIAN_POINT ( 'NONE',  ( 4.458734125000001214, -27.14583333196774717, 2.574251347313718519 ) ) ;
#23262=CARTESIAN_POINT ( 'NONE',  ( -5.000000000000000000, -64.87499999726881583, 0.000000000000000000 ) ) ;
#23263=ORIENTED_EDGE ( 'NONE', *, *, #814, .T. ) ;
#23264=CARTESIAN_POINT ( 'NONE',  ( 3.061616997868383141E-16, -152.8750000027311842, -5.000000000000000000 ) ) ;
#23265=ADVANCED_FACE ( 'NONE', ( #61152 ), #27348, .T. ) ;
#23266=ORIENTED_EDGE ( 'NONE', *, *, #29190, .T. ) ;
#23268=DIRECTION ( 'NONE',  ( -0.000000000000000000, 1.000000000000000000, -0.000000000000000000 ) ) ;
#23272=CARTESIAN_POINT ( 'NONE',  ( 1.975475456537005874E-15, -25.75000000000000355, 5.000000000000000000 ) ) ;
#23273=CARTESIAN_POINT ( 'NONE',  ( 2.229367062499998831, -53.89583333196773651, -3.861377020970580887 ) ) ;
#23275=ORIENTED_EDGE ( 'NONE', *, *, #57116, .T. ) ;
#23276=( BOUNDED_CURVE ( )  B_SPLINE_CURVE ( 2, ( #46982, #37322, #32815, #21587, #16756, #36372, #9617, #4479, #27979 ),
 .UNSPECIFIED., .F., .F. ) 
 B_SPLINE_CURVE_WITH_KNOTS ( ( 3, 2, 2, 2, 3 ),
 ( 0.9854166666666667185, 0.9861111111111111605, 0.9875000000000000444, 0.9888888888888889284, 0.9895833333333333703 ),
 .UNSPECIFIED. ) 
 CURVE ( )  GEOMETRIC_REPRESENTATION_ITEM ( )  RATIONAL_B_SPLINE_CURVE ( ( 0.9330127018922194093, 0.9330127018922194093, 1.000000000000000000, 0.8660254037844387076, 1.000000000000000000, 0.8660254037844387076, 1.000000000000000000, 0.9330127018922194093, 0.9330127018922194093 ) ) 
 REPRESENTATION_ITEM ( '' )  );
#23279=CARTESIAN_POINT ( 'NONE',  ( 4.458734124999998549, 20.27083333469892779, -2.574251347313721627 ) ) ;
#23281=DIRECTION ( 'NONE',  ( -0.000000000000000000, 1.000000000000000000, -0.000000000000000000 ) ) ;
#23282=CARTESIAN_POINT ( 'NONE',  ( 3.152801135295367541, -167.3125000013656063, -3.152801135295367541 ) ) ;
#23284=EDGE_LOOP ( 'NONE', ( #10477, #55278, #46197, #58005 ) ) ;
#23286=CARTESIAN_POINT ( 'NONE',  ( -4.999999999999998224, -85.79166666393547303, 2.886751345948131764 ) ) ;
#23289=AXIS2_PLACEMENT_3D ( 'NONE', #57703, #47409, #48032 ) ;
#23290=CARTESIAN_POINT ( 'NONE',  ( 1.975475456537005874E-15, -69.62499999726880162, 5.000000000000000000 ) ) ;
#23293=CARTESIAN_POINT ( 'NONE',  ( 2.499999999999998668, -20.33333333333333570, -4.330127018922193649 ) ) ;
#23295=CARTESIAN_POINT ( 'NONE',  ( 5.000000000000000888, -76.58333333333335702, 2.886751345948126879 ) ) ;
#23296=CARTESIAN_POINT ( 'NONE',  ( -5.000000000000000000, -156.5000000000000000, -6.123233995736766282E-16 ) ) ;
#23297=CARTESIAN_POINT ( 'NONE',  ( -6.972266317189433020E-16, -89.12499999726880162, -5.000000000000000000 ) ) ;
#23300=CARTESIAN_POINT ( 'NONE',  ( 5.000000000000000000, 11.58333333333333393, -2.886751345948130876 ) ) ;
#23302=CARTESIAN_POINT ( 'NONE',  ( -5.000000000000000000, -152.6250000027312126, -6.123233995736766282E-16 ) ) ;
#23308=CARTESIAN_POINT ( 'NONE',  ( 5.000000000000000000, -143.0000000000000284, 0.000000000000000000 ) ) ;
#23314=CARTESIAN_POINT ( 'NONE',  ( -2.229367062499996610, -30.14583333196773651, 3.861377020970582219 ) ) ;
#23318=CARTESIAN_POINT ( 'NONE',  ( 3.152801135295367541, -147.3125000013655779, -3.152801135295367541 ) ) ;
#23319=ORIENTED_EDGE ( 'NONE', *, *, #23242, .F. ) ;
#23320=CARTESIAN_POINT ( 'NONE',  ( 0.000000000000000000, -170.0000000000000000, 0.000000000000000000 ) ) ;
#23321=CARTESIAN_POINT ( 'NONE',  ( 4.458734124999998549, -57.97916666530107932, -2.574251347313721627 ) ) ;
#23324=CARTESIAN_POINT ( 'NONE',  ( -5.000000000000000000, 18.00000000000000000, 0.000000000000000000 ) ) ;
#23326=CARTESIAN_POINT ( 'NONE',  ( 9.457646018065525792E-16, -0.06249999863440491854, 5.148502694627439702 ) ) ;
#23328=EDGE_CURVE ( 'NONE', #26895, #48046, #34723, .T. ) ;
#23330=CARTESIAN_POINT ( 'NONE',  ( -4.458734124999999437, 11.43750000136559564, 0.000000000000000000 ) ) ;
#23334=VECTOR ( 'NONE', #5572, 1000.000000000000000 ) ;
#23335=CARTESIAN_POINT ( 'NONE',  ( 1.975475456537005874E-15, -23.62499999726880873, 5.000000000000000000 ) ) ;
#23336=CARTESIAN_POINT ( 'NONE',  ( -4.458734124999999437, -46.31249999863440792, 0.000000000000000000 ) ) ;
#23337=CARTESIAN_POINT ( 'NONE',  ( 4.458734124999999437, -158.7500000013656063, 1.846868145590737864 ) ) ;
#23340=CARTESIAN_POINT ( 'NONE',  ( -4.999999999999999112, -51.79166666393548013, 2.886751345948131764 ) ) ;
#23342=VECTOR ( 'NONE', #355, 1000.000000000000000 ) ;
#23343=CARTESIAN_POINT ( 'NONE',  ( 4.458734124999998549, -22.72916666530107221, -2.574251347313721627 ) ) ;
#23347=CARTESIAN_POINT ( 'NONE',  ( -8.190561711645485556E-16, -160.6875000013655779, 4.458734124999999437 ) ) ;
#23348=EDGE_CURVE ( 'NONE', #46264, #57843, #12873, .T. ) ;
#23349=EDGE_CURVE ( 'NONE', #54895, #61565, #45432, .T. ) ;
#23352=CARTESIAN_POINT ( 'NONE',  ( 4.458734124999999437, -39.06249999863440081, -5.460374474430324690E-16 ) ) ;
#23357=CARTESIAN_POINT ( 'NONE',  ( 1.975475456537005874E-15, -24.62499999726881583, 5.000000000000000000 ) ) ;
#23360=CARTESIAN_POINT ( 'NONE',  ( 4.458734124999998549, -83.97916666530107932, -2.574251347313721627 ) ) ;
#23362=CARTESIAN_POINT ( 'NONE',  ( 5.000000000000000000, -35.37499999726881583, -6.123233995736766282E-16 ) ) ;
#23363=CARTESIAN_POINT ( 'NONE',  ( -3.535533905932737309, -158.7500000027312126, -3.535533905932738197 ) ) ;
#23364=( BOUNDED_CURVE ( )  B_SPLINE_CURVE ( 2, ( #2145, #21750, #41345, #12082, #25923, #35580, #51339, #60033, #30751 ),
 .UNSPECIFIED., .F., .F. ) 
 B_SPLINE_CURVE_WITH_KNOTS ( ( 3, 2, 2, 2, 3 ),
 ( 0.5854166666666666963, 0.5861111111111111382, 0.5875000000000000222, 0.5888888888888889062, 0.5895833333333333481 ),
 .UNSPECIFIED. ) 
 CURVE ( )  GEOMETRIC_REPRESENTATION_ITEM ( )  RATIONAL_B_SPLINE_CURVE ( ( 0.9330127018922194093, 0.9330127018922194093, 1.000000000000000000, 0.8660254037844387076, 1.000000000000000000, 0.8660254037844387076, 1.000000000000000000, 0.9330127018922194093, 0.9330127018922194093 ) ) 
 REPRESENTATION_ITEM ( '' )  );
#23365=CARTESIAN_POINT ( 'NONE',  ( 1.339745962155615144, -57.70534180126147561, 4.999999999999999112 ) ) ;
#23367=CARTESIAN_POINT ( 'NONE',  ( 2.500000000000002220, -37.66666666666666430, 4.330127018922192761 ) ) ;
#23370=CARTESIAN_POINT ( 'NONE',  ( -6.972266317189433020E-16, -18.12499999726881228, -5.000000000000000000 ) ) ;
#23375=CARTESIAN_POINT ( 'NONE',  ( -2.229367062500000163, -82.72916666530106511, -3.861377020970580443 ) ) ;
#23382=CARTESIAN_POINT ( 'NONE',  ( 5.000000000000000000, -165.1250000027311842, 0.000000000000000000 ) ) ;
#23392=CARTESIAN_POINT ( 'NONE',  ( 5.000000000000000000, 17.58333333333333215, -2.886751345948130876 ) ) ;
#23393=CARTESIAN_POINT ( 'NONE',  ( 9.457646018065525792E-16, -12.06249999863440081, 5.148502694627439702 ) ) ;
#23396=CARTESIAN_POINT ( 'NONE',  ( -4.458734124999999437, -40.64583333196773651, -2.574251347313719407 ) ) ;
#23397=CARTESIAN_POINT ( 'NONE',  ( 2.500000000000002220, -77.66666666666665719, 4.330127018922192761 ) ) ;
#23402=CARTESIAN_POINT ( 'NONE',  ( 4.458734124999999437, 16.18750000136559564, -5.460374474430324690E-16 ) ) ;
#23403=EDGE_CURVE ( 'NONE', #50575, #57905, #23276, .T. ) ;
#23406=CARTESIAN_POINT ( 'NONE',  ( 4.458734124999999437, -89.06249999863439371, -5.460374474430324690E-16 ) ) ;
#23408=CARTESIAN_POINT ( 'NONE',  ( 5.000000000000000888, 15.54166666939785024, 2.886751345948126879 ) ) ;
#23409=ORIENTED_EDGE ( 'NONE', *, *, #38635, .F. ) ;
#23413=CARTESIAN_POINT ( 'NONE',  ( -5.000000000000000000, -31.00000000000000000, 0.000000000000000000 ) ) ;
#23414=CARTESIAN_POINT ( 'NONE',  ( -3.152548672688508926E-16, -34.56249999863440792, -5.148502694627439702 ) ) ;
#23416=CARTESIAN_POINT ( 'NONE',  ( -5.000000000000000000, -34.95833333060213732, -2.886751345948128211 ) ) ;
#23417=CARTESIAN_POINT ( 'NONE',  ( -2.229367062500000163, -62.47916666530106511, -3.861377020970580443 ) ) ;
#23420=CARTESIAN_POINT ( 'NONE',  ( -2.229367062499996610, -7.395833331967735624, 3.861377020970582219 ) ) ;
#23421=ORIENTED_EDGE ( 'NONE', *, *, #17283, .F. ) ;
#23422=CARTESIAN_POINT ( 'NONE',  ( 5.000000000000000000, -78.41666666666667140, -2.886751345948129988 ) ) ;
#23426=CARTESIAN_POINT ( 'NONE',  ( 5.000000000000000888, -76.45833333060215864, 2.886751345948126879 ) ) ;
#23427=CARTESIAN_POINT ( 'NONE',  ( 1.975475456537005874E-15, -13.75000000000000000, 5.000000000000000000 ) ) ;
#23428=ORIENTED_EDGE ( 'NONE', *, *, #38231, .T. ) ;
#23431=CARTESIAN_POINT ( 'NONE',  ( 4.458734124999998549, -19.97916666530106866, -2.574251347313721627 ) ) ;
#23432=CARTESIAN_POINT ( 'NONE',  ( -2.229367062500000163, -55.72916666530107221, -3.861377020970580443 ) ) ;
#23433=ORIENTED_EDGE ( 'NONE', *, *, #17283, .T. ) ;
#23435=CARTESIAN_POINT ( 'NONE',  ( 3.152801135295367541, -165.5625000013656063, -3.152801135295367541 ) ) ;
#23437=CARTESIAN_POINT ( 'NONE',  ( 1.339745962155612702, -50.16965819600732601, -5.000000000000000000 ) ) ;
#23438=ORIENTED_EDGE ( 'NONE', *, *, #43261, .T. ) ;
#23444=CARTESIAN_POINT ( 'NONE',  ( -1.846868145590737420, -146.0000000013655779, 4.458734124999999437 ) ) ;
#23447=CARTESIAN_POINT ( 'NONE',  ( -4.458734124999998549, -67.47916666530106511, 2.574251347313722516 ) ) ;
#23449=CARTESIAN_POINT ( 'NONE',  ( 4.458734124999999437, -140.3750000013656063, -1.846868145590734978 ) ) ;
#23452=CARTESIAN_POINT ( 'NONE',  ( -5.000000000000000000, -70.87499999726880162, 0.000000000000000000 ) ) ;
#23453=CYLINDRICAL_SURFACE ( 'NONE', #38059, 5.000000000000000000 ) ;
#23459=CARTESIAN_POINT ( 'NONE',  ( 2.229367062500001939, 20.77083333469892779, 3.861377020970579999 ) ) ;
#23467=CARTESIAN_POINT ( 'NONE',  ( 2.229367062499998831, 7.354166668032259935, -3.861377020970580887 ) ) ;
#23468=CARTESIAN_POINT ( 'NONE',  ( -2.229367062499996610, -22.39583333196773651, 3.861377020970582219 ) ) ;
#23469=CARTESIAN_POINT ( 'NONE',  ( 4.458734125000000326, -155.3750000013656347, -1.846868145590734978 ) ) ;
#23472=AXIS2_PLACEMENT_3D ( 'NONE', #9546, #29151, #48772 ) ;
#23476=CARTESIAN_POINT ( 'NONE',  ( -4.458734124999999437, -69.56249999863439371, 0.000000000000000000 ) ) ;
#23478=CARTESIAN_POINT ( 'NONE',  ( 1.339745962155615144, -73.70534180126146850, 4.999999999999999112 ) ) ;
#23479=CARTESIAN_POINT ( 'NONE',  ( 5.000000000000000888, 27.54166666939785557, 2.886751345948126879 ) ) ;
#23480=VERTEX_POINT ( 'NONE', #24418 ) ;
#23481=CARTESIAN_POINT ( 'NONE',  ( -1.339745962155601378, 14.91965820146970501, -5.000000000000007105 ) ) ;
#23482=CARTESIAN_POINT ( 'NONE',  ( -4.999999999999998224, 12.20833333606451632, 2.886751345948131764 ) ) ;
#23483=CARTESIAN_POINT ( 'NONE',  ( 2.500000000000002220, -12.66666666666666607, 4.330127018922192761 ) ) ;
#23484=CARTESIAN_POINT ( 'NONE',  ( -4.458734124999999437, -18.39583333196774007, -2.574251347313719407 ) ) ;
#23485=CARTESIAN_POINT ( 'NONE',  ( 4.458734125000000326, -79.89583333196773651, 2.574251347313718519 ) ) ;
#23487=CARTESIAN_POINT ( 'NONE',  ( 1.846868145590735200, -168.5000000013656063, -4.458734125000000326 ) ) ;
#23488=CARTESIAN_POINT ( 'NONE',  ( 5.000000000000000888, -15.45833333060214265, 2.886751345948126879 ) ) ;
#23489=CARTESIAN_POINT ( 'NONE',  ( 4.458734124999999437, -42.81249999863440081, -5.460374474430324690E-16 ) ) ;
#23490=ORIENTED_EDGE ( 'NONE', *, *, #9223, .F. ) ;
#23492=CARTESIAN_POINT ( 'NONE',  ( 4.458734125000001214, 7.854166668032260823, 2.574251347313718519 ) ) ;
#23493=VERTEX_POINT ( 'NONE', #33135 ) ;
#23495=CARTESIAN_POINT ( 'NONE',  ( 5.000000000000000000, -61.50000000000000000, -6.123233995736766282E-16 ) ) ;
#23496=CARTESIAN_POINT ( 'NONE',  ( 1.846868145590736310, -155.8750000013655779, 4.458734124999999437 ) ) ;
#23499=CARTESIAN_POINT ( 'NONE',  ( -5.000000000000000888, -166.5625000000000000, -2.071067811865475949 ) ) ;
#23500=CARTESIAN_POINT ( 'NONE',  ( 2.071067811865495045, -168.1875000000000284, 4.999999999999981348 ) ) ;
#23502=CARTESIAN_POINT ( 'NONE',  ( 9.457646018065525792E-16, -8.312499998634406140, 5.148502694627439702 ) ) ;
#23503=CARTESIAN_POINT ( 'NONE',  ( 2.229367062499998831, -38.89583333196773651, -3.861377020970580887 ) ) ;
#23504=CARTESIAN_POINT ( 'NONE',  ( -6.972266317189433020E-16, -67.12499999726881583, -5.000000000000000000 ) ) ;
#23505=CARTESIAN_POINT ( 'NONE',  ( -4.458734125000000326, -150.0000000013655779, -1.846868145590735644 ) ) ;
#23507=( BOUNDED_CURVE ( )  B_SPLINE_CURVE ( 2, ( #40570, #30922, #50549, #56656, #12264, #37336, #26743, #21916, #7127 ),
 .UNSPECIFIED., .F., .F. ) 
 B_SPLINE_CURVE_WITH_KNOTS ( ( 3, 2, 2, 2, 3 ),
 ( 0.5395833333333333037, 0.5402777777777777457, 0.5416666666666666297, 0.5430555555555555136, 0.5437499999999999556 ),
 .UNSPECIFIED. ) 
 CURVE ( )  GEOMETRIC_REPRESENTATION_ITEM ( )  RATIONAL_B_SPLINE_CURVE ( ( 0.9330127018922194093, 0.9330127018922194093, 1.000000000000000000, 0.8660254037844387076, 1.000000000000000000, 0.8660254037844387076, 1.000000000000000000, 0.9330127018922194093, 0.9330127018922194093 ) ) 
 REPRESENTATION_ITEM ( '' )  );
#23510=CARTESIAN_POINT ( 'NONE',  ( -5.000000000000000888, -141.4375000000000284, 2.071067811865474617 ) ) ;
#23513=CARTESIAN_POINT ( 'NONE',  ( -2.229367062499996610, -70.39583333196773651, 3.861377020970582219 ) ) ;
#23515=CARTESIAN_POINT ( 'NONE',  ( 3.152801135295367541, -146.5625000013655779, -3.152801135295367541 ) ) ;
#23519=CARTESIAN_POINT ( 'NONE',  ( -4.458734124999998549, 1.770833334698927786, 2.574251347313722516 ) ) ;
#23521=CARTESIAN_POINT ( 'NONE',  ( 3.152801135295366208, -151.5625000013655779, 3.152801135295367985 ) ) ;
#23525=CARTESIAN_POINT ( 'NONE',  ( 1.975475456537005874E-15, -74.75000000000000000, 5.000000000000000000 ) ) ;
#23526=CARTESIAN_POINT ( 'NONE',  ( 1.339745962155615144, -12.58034179853029144, 4.999999999999999112 ) ) ;
#23528=EDGE_CURVE ( 'NONE', #14852, #26724, #1885, .T. ) ;
#23529=CARTESIAN_POINT ( 'NONE',  ( 0.000000000000000000, -170.0000000000000000, 5.000000000000000000 ) ) ;
#23537=CARTESIAN_POINT ( 'NONE',  ( -2.229367062500000163, 24.52083333469892779, -3.861377020970580443 ) ) ;
#23539=CARTESIAN_POINT ( 'NONE',  ( 4.458734124999998549, -5.979166665301071326, -2.574251347313721627 ) ) ;
#23540=CARTESIAN_POINT ( 'NONE',  ( -1.339745962155610925, -62.79465819873851729, 5.000000000000000000 ) ) ;
#23542=CARTESIAN_POINT ( 'NONE',  ( -3.152801135295367985, -167.8125000013656063, 3.152801135295367096 ) ) ;
#23543=CARTESIAN_POINT ( 'NONE',  ( -5.000000000000000000, -52.00000000000000711, 0.000000000000000000 ) ) ;
#23548=EDGE_CURVE ( 'NONE', #30305, #59122, #28149, .T. ) ;
#23549=DIRECTION ( 'NONE',  ( -0.000000000000000000, 1.000000000000000000, -0.000000000000000000 ) ) ;
#23552=CARTESIAN_POINT ( 'NONE',  ( 1.846868145590736310, -157.8750000013655779, 4.458734124999997661 ) ) ;
#23556=CARTESIAN_POINT ( 'NONE',  ( 0.000000000000000000, -170.0000000000000000, 0.000000000000000000 ) ) ;
#23562=( BOUNDED_CURVE ( )  B_SPLINE_CURVE ( 2, ( #21898, #51491, #3549, #51176, #8375, #32167, #18330, #23157, #18007 ),
 .UNSPECIFIED., .F., .F. ) 
 B_SPLINE_CURVE_WITH_KNOTS ( ( 3, 2, 2, 2, 3 ),
 ( 0.9937500000000000222, 0.9944444444444444642, 0.9958333333333333481, 0.9972222222222222321, 0.9979166666666666741 ),
 .UNSPECIFIED. ) 
 CURVE ( )  GEOMETRIC_REPRESENTATION_ITEM ( )  RATIONAL_B_SPLINE_CURVE ( ( 0.9330127018922194093, 0.9330127018922194093, 1.000000000000000000, 0.8660254037844387076, 1.000000000000000000, 0.8660254037844387076, 1.000000000000000000, 0.9330127018922194093, 0.9330127018922194093 ) ) 
 REPRESENTATION_ITEM ( '' )  );
#23563=CARTESIAN_POINT ( 'NONE',  ( -1.339745962155613812, -88.08034179853028434, -5.000000000000000000 ) ) ;
#23564=CARTESIAN_POINT ( 'NONE',  ( -2.499999999999996447, 2.166666666666667407, 4.330127018922195425 ) ) ;
#23566=EDGE_CURVE ( 'NONE', #12840, #7641, #23652, .T. ) ;
#23567=CARTESIAN_POINT ( 'NONE',  ( 2.229367062500001939, -63.97916666530106511, 3.861377020970579999 ) ) ;
#23568=CARTESIAN_POINT ( 'NONE',  ( -1.339745962155610925, -7.794658198738519950, 5.000000000000000000 ) ) ;
#23569=CARTESIAN_POINT ( 'NONE',  ( 5.000000000000000888, 1.541666669397853573, 2.886751345948126879 ) ) ;
#23570=CARTESIAN_POINT ( 'NONE',  ( -2.229367062500000163, -27.47916666530107221, -3.861377020970580443 ) ) ;
#23571=CARTESIAN_POINT ( 'NONE',  ( -1.339745962155613812, -42.20534180126148271, -5.000000000000000000 ) ) ;
#23572=CARTESIAN_POINT ( 'NONE',  ( 0.000000000000000000, -170.0000000000000000, 0.000000000000000000 ) ) ;
#23573=CARTESIAN_POINT ( 'NONE',  ( -6.972266317189433020E-16, -19.25000000000000000, -5.000000000000000000 ) ) ;
#23574=CARTESIAN_POINT ( 'NONE',  ( -2.499999999999996447, -44.83333333333333570, 4.330127018922195425 ) ) ;
#23575=CARTESIAN_POINT ( 'NONE',  ( -6.972266317189433020E-16, -45.24999999999999289, -5.000000000000000000 ) ) ;
#23577=CARTESIAN_POINT ( 'NONE',  ( -4.458734124999998549, -64.22916666530107932, 2.574251347313722516 ) ) ;
#23578=CARTESIAN_POINT ( 'NONE',  ( 4.458734125000000326, -146.6250000013655779, -1.846868145590734978 ) ) ;
#23579=CARTESIAN_POINT ( 'NONE',  ( -3.152548672688508926E-16, -77.56249999863440792, -5.148502694627439702 ) ) ;
#23581=CARTESIAN_POINT ( 'NONE',  ( -4.458734124999999437, -27.56249999863440081, 0.000000000000000000 ) ) ;
#23582=CARTESIAN_POINT ( 'NONE',  ( -5.000000000000000000, -64.95833333060214443, -2.886751345948128211 ) ) ;
#23586=ORIENTED_EDGE ( 'NONE', *, *, #3867, .F. ) ;
#23590=ORIENTED_EDGE ( 'NONE', *, *, #25667, .T. ) ;
#23592=CARTESIAN_POINT ( 'NONE',  ( 4.458734125000001214, -55.14583333196772941, 2.574251347313718519 ) ) ;
#23594=ORIENTED_EDGE ( 'NONE', *, *, #40432, .F. ) ;
#23596=CARTESIAN_POINT ( 'NONE',  ( 4.458734124999998549, 17.27083333469892779, -2.574251347313721627 ) ) ;
#23598=LINE ( 'NONE', #62837, #26444 ) ;
#23599=CARTESIAN_POINT ( 'NONE',  ( -4.458734125000000326, -165.8750000013656063, 1.846868145590734089 ) ) ;
#23602=DIRECTION ( 'NONE',  ( -0.000000000000000000, 1.000000000000000000, -0.000000000000000000 ) ) ;
#23606=EDGE_CURVE ( 'NONE', #44494, #8541, #19264, .T. ) ;
#23607=CARTESIAN_POINT ( 'NONE',  ( -2.071067811865404451, -162.4375000027311557, 5.000000000000073719 ) ) ;
#23612=CYLINDRICAL_SURFACE ( 'NONE', #24237, 5.000000000000000000 ) ;
#23613=CARTESIAN_POINT ( 'NONE',  ( 2.499999999999998668, -18.20833333060214798, -4.330127018922193649 ) ) ;
#23614=CARTESIAN_POINT ( 'NONE',  ( -9.184850993605147944E-16, -159.2500000000000000, 5.000000000000000000 ) ) ;
#23617=DIRECTION ( 'NONE',  ( -0.000000000000000000, 1.000000000000000000, -0.000000000000000000 ) ) ;
#23619=CARTESIAN_POINT ( 'NONE',  ( -3.535533905932738641, -151.5000000027312126, 3.535533905932737309 ) ) ;
#23620=ORIENTED_EDGE ( 'NONE', *, *, #44076, .F. ) ;
#23624=ADVANCED_FACE ( 'NONE', ( #29541 ), #59803, .T. ) ;
#23626=CARTESIAN_POINT ( 'NONE',  ( -3.535533905932737309, -144.6250000000000000, -3.535533905932738197 ) ) ;
#23627=ADVANCED_FACE ( 'NONE', ( #45631 ), #54324, .T. ) ;
#23629=CARTESIAN_POINT ( 'NONE',  ( -2.500000000000000444, -55.16666666666667140, -4.330127018922193649 ) ) ;
#23630=CARTESIAN_POINT ( 'NONE',  ( 2.229367062499998831, -29.64583333196773296, -3.861377020970580887 ) ) ;
#23631=DIRECTION ( 'NONE',  ( 0.000000000000000000, 0.000000000000000000, 1.000000000000000000 ) ) ;
#23632=CARTESIAN_POINT ( 'NONE',  ( 5.000000000000000000, 18.62500000273118772, -6.123233995736766282E-16 ) ) ;
#23634=CARTESIAN_POINT ( 'NONE',  ( -4.458734124999999437, -145.9375000013656063, -5.460374474430324690E-16 ) ) ;
#23635=ORIENTED_EDGE ( 'NONE', *, *, #9707, .T. ) ;
#23637=CARTESIAN_POINT ( 'NONE',  ( 9.457646018065525792E-16, -57.31249999863440081, 5.148502694627439702 ) ) ;
#23640=CARTESIAN_POINT ( 'NONE',  ( 5.000000000000000000, 17.58333333333333215, -2.886751345948129988 ) ) ;
#23641=( BOUNDED_CURVE ( )  B_SPLINE_CURVE ( 2, ( #49206, #29254, #52545, #24445, #39228, #10288, #25079, #30212, #14469 ),
 .UNSPECIFIED., .F., .F. ) 
 B_SPLINE_CURVE_WITH_KNOTS ( ( 3, 2, 2, 2, 3 ),
 ( 0.2895833333333333592, 0.2902777777777778012, 0.2916666666666666852, 0.2930555555555555691, 0.2937500000000000111 ),
 .UNSPECIFIED. ) 
 CURVE ( )  GEOMETRIC_REPRESENTATION_ITEM ( )  RATIONAL_B_SPLINE_CURVE ( ( 0.9330127018922194093, 0.9330127018922220739, 1.000000000000000000, 0.8660254037844387076, 1.000000000000000000, 0.8660254037844387076, 1.000000000000000000, 0.9330127018922194093, 0.9330127018922194093 ) ) 
 REPRESENTATION_ITEM ( '' )  );
#23642=CARTESIAN_POINT ( 'NONE',  ( -2.229367062500000163, -7.479166665301073991, -3.861377020970580443 ) ) ;
#23645=CARTESIAN_POINT ( 'NONE',  ( 9.457646018065525792E-16, 8.687500001365595637, 5.148502694627439702 ) ) ;
#23646=CARTESIAN_POINT ( 'NONE',  ( 2.499999999999998668, -53.20833333060213732, -4.330127018922193649 ) ) ;
#23649=CARTESIAN_POINT ( 'NONE',  ( -4.458734124999999437, -48.39583333196772941, -2.574251347313719407 ) ) ;
#23650=CARTESIAN_POINT ( 'NONE',  ( -3.152801135295367096, -160.3125000013656063, -3.152801135295367541 ) ) ;
#23652=( BOUNDED_CURVE ( )  B_SPLINE_CURVE ( 2, ( #14753, #38881, #47905, #34370, #28293, #18333, #57590, #13518, #8679 ),
 .UNSPECIFIED., .F., .F. ) 
 B_SPLINE_CURVE_WITH_KNOTS ( ( 3, 2, 2, 2, 3 ),
 ( 0.2187500000000000000, 0.2194444444444444420, 0.2208333333333333259, 0.2222222222222222099, 0.2229166666666666796 ),
 .UNSPECIFIED. ) 
 CURVE ( )  GEOMETRIC_REPRESENTATION_ITEM ( )  RATIONAL_B_SPLINE_CURVE ( ( 0.9330127018922194093, 0.9330127018922194093, 1.000000000000000000, 0.8660254037844387076, 1.000000000000000000, 0.8660254037844387076, 1.000000000000000000, 0.9330127018922180770, 0.9330127018922194093 ) ) 
 REPRESENTATION_ITEM ( '' )  );
#23653=CARTESIAN_POINT ( 'NONE',  ( 5.000000000000000888, -52.45833333060213732, 2.886751345948126879 ) ) ;
#23654=VERTEX_POINT ( 'NONE', #16039 ) ;
#23655=CARTESIAN_POINT ( 'NONE',  ( -4.458734124999999437, -23.39583333196773296, -2.574251347313719407 ) ) ;
#23659=CARTESIAN_POINT ( 'NONE',  ( 4.458734124999999437, -161.5000000013656063, 1.846868145590737864 ) ) ;
#23660=ORIENTED_EDGE ( 'NONE', *, *, #36892, .T. ) ;
#23663=CARTESIAN_POINT ( 'NONE',  ( 2.229367062500001939, -35.22916666530107221, 3.861377020970579999 ) ) ;
#23665=VERTEX_POINT ( 'NONE', #25050 ) ;
#23668=LINE ( 'NONE', #38142, #19409 ) ;
#23671=CARTESIAN_POINT ( 'NONE',  ( 4.458734124999999437, -87.06249999863439371, -5.460374474430324690E-16 ) ) ;
#23674=LINE ( 'NONE', #15275, #16167 ) ;
#23677=CARTESIAN_POINT ( 'NONE',  ( 1.975475456537005874E-15, -37.74999999999999289, 5.000000000000000000 ) ) ;
#23680=CARTESIAN_POINT ( 'NONE',  ( -6.972266317189433020E-16, -82.24999999999998579, -5.000000000000000000 ) ) ;
#23681=EDGE_CURVE ( 'NONE', #49893, #551, #15410, .T. ) ;
#23685=CARTESIAN_POINT ( 'NONE',  ( -6.972266317189433020E-16, -61.25000000000000000, -5.000000000000000000 ) ) ;
#23686=CARTESIAN_POINT ( 'NONE',  ( -2.229367062499996610, -85.39583333196773651, 3.861377020970582219 ) ) ;
#23689=EDGE_CURVE ( 'NONE', #14909, #51364, #35344, .T. ) ;
#23693=CARTESIAN_POINT ( 'NONE',  ( 2.071067811865476394, -165.3125000027312126, 5.000000000000000000 ) ) ;
#23695=AXIS2_PLACEMENT_3D ( 'NONE', #5261, #1094, #10399 ) ;
#23697=EDGE_CURVE ( 'NONE', #34811, #23480, #53999, .T. ) ;
#23699=EDGE_CURVE ( 'NONE', #7768, #58694, #58585, .T. ) ;
#23707=CARTESIAN_POINT ( 'NONE',  ( -2.229367062500000163, -14.47916666530107221, -3.861377020970580443 ) ) ;
#23708=CARTESIAN_POINT ( 'NONE',  ( 5.000000000000000888, -71.58333333333332860, 2.886751345948126879 ) ) ;
#23711=CARTESIAN_POINT ( 'NONE',  ( 9.457646018065525792E-16, -41.31249999863440792, 5.148502694627439702 ) ) ;
#23712=( BOUNDED_CURVE ( )  B_SPLINE_CURVE ( 2, ( #35195, #54811, #20398, #5283, #54493, #24903, #5926, #45793, #29708 ),
 .UNSPECIFIED., .F., .F. ) 
 B_SPLINE_CURVE_WITH_KNOTS ( ( 3, 2, 2, 2, 3 ),
 ( 0.3312499999999999889, 0.3319444444444444309, 0.3333333333333333148, 0.3347222222222221988, 0.3354166666666666963 ),
 .UNSPECIFIED. ) 
 CURVE ( )  GEOMETRIC_REPRESENTATION_ITEM ( )  RATIONAL_B_SPLINE_CURVE ( ( 0.9330127018922194093, 0.9330127018922194093, 1.000000000000000000, 0.8660254037844387076, 1.000000000000000000, 0.8660254037844387076, 1.000000000000000000, 0.9330127018922167448, 0.9330127018922194093 ) ) 
 REPRESENTATION_ITEM ( '' )  );
#23717=CARTESIAN_POINT ( 'NONE',  ( -2.229367062499996610, 12.85416666803226171, 3.861377020970582219 ) ) ;
#23719=CARTESIAN_POINT ( 'NONE',  ( 3.061616997868383141E-16, -155.7500000000000000, -5.000000000000000000 ) ) ;
#23721=CARTESIAN_POINT ( 'NONE',  ( -4.458734124999999437, -88.64583333196773651, -2.574251347313719407 ) ) ;
#23723=CARTESIAN_POINT ( 'NONE',  ( 5.000000000000000888, 14.54166666939785024, 2.886751345948126879 ) ) ;
#23728=CARTESIAN_POINT ( 'NONE',  ( -3.535250795749689387E-16, -30.24999999999999645, -5.773502691896257311 ) ) ;
#23729=CARTESIAN_POINT ( 'NONE',  ( -3.152548672688508926E-16, -31.56249999863440436, -5.148502694627439702 ) ) ;
#23730=CARTESIAN_POINT ( 'NONE',  ( 5.000000000000000000, -36.29166666393547303, -2.886751345948129988 ) ) ;
#23731=CARTESIAN_POINT ( 'NONE',  ( -2.229367062499996610, -63.14583333196774362, 3.861377020970582219 ) ) ;
#23734=CARTESIAN_POINT ( 'NONE',  ( 2.229367062500001939, -14.22916666530107221, 3.861377020970579999 ) ) ;
#23735=ORIENTED_EDGE ( 'NONE', *, *, #42929, .F. ) ;
#23736=CARTESIAN_POINT ( 'NONE',  ( -2.499999999999996447, -76.83333333333334281, 4.330127018922195425 ) ) ;
#23739=( BOUNDED_CURVE ( )  B_SPLINE_CURVE ( 2, ( #27477, #47105, #31674, #61911, #61275, #17196, #41949, #36823, #56454 ),
 .UNSPECIFIED., .F., .F. ) 
 B_SPLINE_CURVE_WITH_KNOTS ( ( 3, 2, 2, 2, 3 ),
 ( 0.08958333333333333426, 0.09027777777777777624, 0.09166666666666666019, 0.09305555555555555802, 0.09375000000000000000 ),
 .UNSPECIFIED. ) 
 CURVE ( )  GEOMETRIC_REPRESENTATION_ITEM ( )  RATIONAL_B_SPLINE_CURVE ( ( 0.9330127018922194093, 0.9330127018922194093, 1.000000000000000000, 0.8660254037844387076, 1.000000000000000000, 0.8660254037844387076, 1.000000000000000000, 0.9330127018922194093, 0.9330127018922194093 ) ) 
 REPRESENTATION_ITEM ( '' )  );
#23740=CARTESIAN_POINT ( 'NONE',  ( 5.000000000000000000, -80.29166666393545881, -2.886751345948129988 ) ) ;
#23741=CARTESIAN_POINT ( 'NONE',  ( 5.000000000000000000, -13.49999999999999822, -6.123233995736766282E-16 ) ) ;
#23743=AXIS2_PLACEMENT_3D ( 'NONE', #44661, #21186, #50465 ) ;
#23745=CARTESIAN_POINT ( 'NONE',  ( -4.458734124999999437, -22.64583333196773296, -2.574251347313719407 ) ) ;
#23746=CARTESIAN_POINT ( 'NONE',  ( -4.458734124999999437, -55.64583333196773651, -2.574251347313719407 ) ) ;
#23747=ORIENTED_EDGE ( 'NONE', *, *, #48346, .T. ) ;
#23749=CARTESIAN_POINT ( 'NONE',  ( 3.152801135295366208, -168.8125000013656063, 3.152801135295367985 ) ) ;
#23752=EDGE_LOOP ( 'NONE', ( #36299, #33699, #3409, #36700 ) ) ;
#23756=CARTESIAN_POINT ( 'NONE',  ( 0.000000000000000000, -170.0000000000000000, 0.000000000000000000 ) ) ;
#23759=CARTESIAN_POINT ( 'NONE',  ( 3.152801135295367541, -144.5625000013655779, -3.152801135295367541 ) ) ;
#23762=CARTESIAN_POINT ( 'NONE',  ( -2.229367062499996610, -67.39583333196773651, 3.861377020970582219 ) ) ;
#23763=DIRECTION ( 'NONE',  ( -0.000000000000000000, 1.000000000000000000, -0.000000000000000000 ) ) ;
#23764=CARTESIAN_POINT ( 'NONE',  ( 4.458734124999999437, -142.3750000013656063, -1.846868145590734978 ) ) ;
#23767=CARTESIAN_POINT ( 'NONE',  ( -4.999999999999998224, -70.79166666393547303, 2.886751345948131764 ) ) ;
#23772=CARTESIAN_POINT ( 'NONE',  ( 9.457646018065525792E-16, 23.68750000136559564, 5.148502694627439702 ) ) ;
#23778=CARTESIAN_POINT ( 'NONE',  ( 2.499999999999998668, -43.20833333060214443, -4.330127018922193649 ) ) ;
#23779=CARTESIAN_POINT ( 'NONE',  ( -2.229367062499996610, 1.854166668032262377, 3.861377020970582219 ) ) ;
#23780=CARTESIAN_POINT ( 'NONE',  ( -3.152548672688508926E-16, -26.81249999863440436, -5.148502694627439702 ) ) ;
#23781=CARTESIAN_POINT ( 'NONE',  ( 1.846868145590735200, -155.2500000013656063, -4.458734125000000326 ) ) ;
#23784=CARTESIAN_POINT ( 'NONE',  ( 5.000000000000000000, 15.58333333333332860, -2.886751345948130876 ) ) ;
#23787=CARTESIAN_POINT ( 'NONE',  ( 4.458734125000000326, -75.14583333196775072, 2.574251347313718519 ) ) ;
#23790=CARTESIAN_POINT ( 'NONE',  ( -2.500000000000000444, 28.95833333606451987, -4.330127018922193649 ) ) ;
#23794=CARTESIAN_POINT ( 'NONE',  ( 1.060575238724906964E-15, -13.75000000000000000, 5.773502691896257311 ) ) ;
#23795=CARTESIAN_POINT ( 'NONE',  ( -2.229367062500000163, -15.47916666530107399, -3.861377020970580443 ) ) ;
#23796=CARTESIAN_POINT ( 'NONE',  ( -4.458734124999999437, -78.31249999863440792, 0.000000000000000000 ) ) ;
#23797=CARTESIAN_POINT ( 'NONE',  ( -1.846868145590734756, -169.3750000013656347, -4.458734125000000326 ) ) ;
#23798=CARTESIAN_POINT ( 'NONE',  ( -5.000000000000000000, -18.87499999726881583, 0.000000000000000000 ) ) ;
#23799=CARTESIAN_POINT ( 'NONE',  ( -2.229367062499996610, -47.14583333196774362, 3.861377020970582219 ) ) ;
#23801=CARTESIAN_POINT ( 'NONE',  ( -1.339745962155610925, -27.66965819600733667, 5.000000000000000000 ) ) ;
#23802=CARTESIAN_POINT ( 'NONE',  ( 4.458734124999998549, 2.020833334698927786, -2.574251347313721627 ) ) ;
#23803=VERTEX_POINT ( 'NONE', #32097 ) ;
#23805=CARTESIAN_POINT ( 'NONE',  ( -2.500000000000000444, -63.16666666666666430, -4.330127018922193649 ) ) ;
#23806=CARTESIAN_POINT ( 'NONE',  ( 3.152801135295367541, -156.5625000013656063, -3.152801135295367541 ) ) ;
#23808=CARTESIAN_POINT ( 'NONE',  ( -5.000000000000000000, -79.00000000000000000, 0.000000000000000000 ) ) ;
#23809=CARTESIAN_POINT ( 'NONE',  ( -2.071067811865478170, -161.3125000000000284, 5.000000000000000000 ) ) ;
#23810=CARTESIAN_POINT ( 'NONE',  ( 0.000000000000000000, -170.0000000000000000, 0.000000000000000000 ) ) ;
#23812=CARTESIAN_POINT ( 'NONE',  ( 4.458734125000001214, -4.145833331967740065, 2.574251347313718519 ) ) ;
#23813=CARTESIAN_POINT ( 'NONE',  ( -4.458734124999998549, -41.47916666530107221, 2.574251347313722516 ) ) ;
#23815=CARTESIAN_POINT ( 'NONE',  ( -1.846868145590737420, -149.7500000013656063, 4.458734124999999437 ) ) ;
#23817=CARTESIAN_POINT ( 'NONE',  ( 1.339745962155615144, 8.294658198738519062, 4.999999999999999112 ) ) ;
#23822=CARTESIAN_POINT ( 'NONE',  ( -2.229367062500000163, -77.72916666530106511, -3.861377020970580443 ) ) ;
#23823=ORIENTED_EDGE ( 'NONE', *, *, #50790, .T. ) ;
#23827=PRODUCT_DEFINITION_CONTEXT ( 'detailed design', #38816, 'design' ) ;
#23829=CARTESIAN_POINT ( 'NONE',  ( -4.458734124999999437, -2.312499998634407028, 0.000000000000000000 ) ) ;
#23831=CARTESIAN_POINT ( 'NONE',  ( -4.458734124999999437, -151.9375000013655779, -5.460374474430324690E-16 ) ) ;
#23834=ORIENTED_EDGE ( 'NONE', *, *, #46844, .T. ) ;
#23837=CARTESIAN_POINT ( 'NONE',  ( 2.499999999999998668, -12.20833333060214798, -4.330127018922193649 ) ) ;
#23840=CYLINDRICAL_SURFACE ( 'NONE', #35593, 5.000000000000000000 ) ;
#23843=CARTESIAN_POINT ( 'NONE',  ( 2.499999999999998668, -64.20833333060213022, -4.330127018922193649 ) ) ;
#23846=CARTESIAN_POINT ( 'NONE',  ( 9.457646018065525792E-16, 15.93750000136559564, 5.148502694627439702 ) ) ;
#23848=CARTESIAN_POINT ( 'NONE',  ( 4.458734125000000326, -7.145833331967736513, 2.574251347313718519 ) ) ;
#23851=CARTESIAN_POINT ( 'NONE',  ( 4.458734125000000326, -167.3750000013656347, -1.846868145590734978 ) ) ;
#23857=LINE ( 'NONE', #43460, #41868 ) ;
#23859=CARTESIAN_POINT ( 'NONE',  ( -4.458734124999999437, -155.1875000013655779, -5.460374474430324690E-16 ) ) ;
#23863=ORIENTED_EDGE ( 'NONE', *, *, #5603, .F. ) ;
#23867=FACE_OUTER_BOUND ( 'NONE', #28915, .T. ) ;
#23868=CARTESIAN_POINT ( 'NONE',  ( -5.000000000000000000, 2.916666666666668739, -2.886751345948128211 ) ) ;
#23869=CARTESIAN_POINT ( 'NONE',  ( 2.229367062499998831, -59.64583333196774362, -3.861377020970580887 ) ) ;
#23871=CARTESIAN_POINT ( 'NONE',  ( 5.000000000000000000, -0.3749999972688135008, -6.123233995736766282E-16 ) ) ;
#23872=CARTESIAN_POINT ( 'NONE',  ( -4.458734124999998549, -28.22916666530106866, 2.574251347313722516 ) ) ;
#23873=CARTESIAN_POINT ( 'NONE',  ( 3.061616997868383141E-16, -152.8750000027311842, -5.000000000000000000 ) ) ;
#23875=( BOUNDED_CURVE ( )  B_SPLINE_CURVE ( 2, ( #3967, #406, #48951, #44447, #14228, #63140, #48014, #20009, #48326 ),
 .UNSPECIFIED., .F., .F. ) 
 B_SPLINE_CURVE_WITH_KNOTS ( ( 3, 2, 2, 2, 3 ),
 ( 0.01041666666666666782, 0.01111111111111111154, 0.01250000000000000069, 0.01388888888888888812, 0.01458333333333333356 ),
 .UNSPECIFIED. ) 
 CURVE ( )  GEOMETRIC_REPRESENTATION_ITEM ( )  RATIONAL_B_SPLINE_CURVE ( ( 0.9330127018922192983, 0.9330127018922194093, 1.000000000000000000, 0.8660254037844387076, 1.000000000000000000, 0.8660254037844387076, 1.000000000000000000, 0.9330127018922191873, 0.9330127018922192983 ) ) 
 REPRESENTATION_ITEM ( '' )  );
#23876=DIRECTION ( 'NONE',  ( 0.000000000000000000, 0.000000000000000000, 1.000000000000000000 ) ) ;
#23877=CARTESIAN_POINT ( 'NONE',  ( 5.000000000000000000, -45.41666666666666430, -2.886751345948129988 ) ) ;
#23878=CARTESIAN_POINT ( 'NONE',  ( 3.061616997868383141E-16, -141.8750000027312126, -5.000000000000000000 ) ) ;
#23879=( BOUNDED_CURVE ( )  B_SPLINE_CURVE ( 2, ( #44727, #58891, #14821, #369, #19973, #689, #39582, #45057, #59545 ),
 .UNSPECIFIED., .F., .F. ) 
 B_SPLINE_CURVE_WITH_KNOTS ( ( 3, 2, 2, 2, 3 ),
 ( 0.8916666666666664964, 0.8958333333333331483, 0.8999999999999999112, 0.9041666666666665630, 0.9083333333333332149 ),
 .UNSPECIFIED. ) 
 CURVE ( )  GEOMETRIC_REPRESENTATION_ITEM ( )  RATIONAL_B_SPLINE_CURVE ( ( 1.000000000000003997, 0.9238795325112826307, 1.000000000000000000, 0.9238795325112867385, 1.000000000000000000, 0.9238795325112867385, 1.000000000000000000, 0.9238795325112887369, 0.9999999999999980016 ) ) 
 REPRESENTATION_ITEM ( '' )  );
#23882=CARTESIAN_POINT ( 'NONE',  ( 9.457646018065525792E-16, -71.06249999863440792, 5.148502694627439702 ) ) ;
#23883=CARTESIAN_POINT ( 'NONE',  ( 1.846868145590736310, -146.8750000013656063, 4.458734124999999437 ) ) ;
#23884=CARTESIAN_POINT ( 'NONE',  ( 4.458734125000001214, -74.89583333196773651, 2.574251347313718519 ) ) ;
#23887=CARTESIAN_POINT ( 'NONE',  ( -2.229367062500000163, -24.72916666530106866, -3.861377020970580443 ) ) ;
#23888=CARTESIAN_POINT ( 'NONE',  ( -4.999999999999999112, -65.79166666393547303, 2.886751345948131764 ) ) ;
#23890=CARTESIAN_POINT ( 'NONE',  ( -4.999999999999998224, -21.91666666666666785, 2.886751345948131764 ) ) ;
#23891=ORIENTED_EDGE ( 'NONE', *, *, #50769, .F. ) ;
#23893=CARTESIAN_POINT ( 'NONE',  ( -9.184850993605147944E-16, -166.2500000000000000, 5.000000000000000000 ) ) ;
#23896=CARTESIAN_POINT ( 'NONE',  ( 4.458734124999999437, -57.06249999863440081, -5.460374474430324690E-16 ) ) ;
#23899=ADVANCED_FACE ( 'NONE', ( #12799 ), #50774, .T. ) ;
#23902=( BOUNDED_CURVE ( )  B_SPLINE_CURVE ( 2, ( #14590, #9455, #43544, #23943, #59304, #62875, #44179, #63189, #29701 ),
 .UNSPECIFIED., .F., .F. ) 
 B_SPLINE_CURVE_WITH_KNOTS ( ( 3, 2, 2, 2, 3 ),
 ( 0.1270833333333333259, 0.1277777777777777679, 0.1291666666666666796, 0.1305555555555555636, 0.1312500000000000056 ),
 .UNSPECIFIED. ) 
 CURVE ( )  GEOMETRIC_REPRESENTATION_ITEM ( )  RATIONAL_B_SPLINE_CURVE ( ( 0.9330127018922194093, 0.9330127018922194093, 1.000000000000000000, 0.8660254037844387076, 1.000000000000000000, 0.8660254037844387076, 1.000000000000000000, 0.9330127018922194093, 0.9330127018922194093 ) ) 
 REPRESENTATION_ITEM ( '' )  );
#23903=CARTESIAN_POINT ( 'NONE',  ( -2.229367062499996610, 17.85416666803225993, 3.861377020970582219 ) ) ;
#23905=CARTESIAN_POINT ( 'NONE',  ( -8.190561711645485556E-16, -163.6875000013655779, 4.458734124999999437 ) ) ;
#23906=VERTEX_POINT ( 'NONE', #17634 ) ;
#23908=CARTESIAN_POINT ( 'NONE',  ( -2.499999999999996447, -69.70833333060214443, 4.330127018922195425 ) ) ;
#23913=CARTESIAN_POINT ( 'NONE',  ( -2.499999999999996447, 6.166666666666667851, 4.330127018922195425 ) ) ;
#23915=DIRECTION ( 'NONE',  ( -0.000000000000000000, 1.000000000000000000, -0.000000000000000000 ) ) ;
#23920=CARTESIAN_POINT ( 'NONE',  ( -4.458734124999999437, 7.354166668032259047, -2.574251347313719407 ) ) ;
#23921=( BOUNDED_CURVE ( )  B_SPLINE_CURVE ( 2, ( #11159, #41688, #25640, #45256, #20821, #16312, #35933, #11476, #50717 ),
 .UNSPECIFIED., .F., .F. ) 
 B_SPLINE_CURVE_WITH_KNOTS ( ( 3, 2, 2, 2, 3 ),
 ( 0.4645833333333333481, 0.4652777777777777901, 0.4666666666666666741, 0.4680555555555555580, 0.4687500000000000000 ),
 .UNSPECIFIED. ) 
 CURVE ( )  GEOMETRIC_REPRESENTATION_ITEM ( )  RATIONAL_B_SPLINE_CURVE ( ( 0.9330127018922194093, 0.9330127018922194093, 1.000000000000000000, 0.8660254037844387076, 1.000000000000000000, 0.8660254037844387076, 1.000000000000000000, 0.9330127018922194093, 0.9330127018922194093 ) ) 
 REPRESENTATION_ITEM ( '' )  );
#23924=CARTESIAN_POINT ( 'NONE',  ( -3.535533905932737309, -147.7500000027311842, -3.535533905932738197 ) ) ;
#23929=CARTESIAN_POINT ( 'NONE',  ( 5.000000000000000888, -142.9375000000000284, -2.071067811865475505 ) ) ;
#23930=EDGE_CURVE ( 'NONE', #26541, #40520, #63472, .T. ) ;
#23932=CARTESIAN_POINT ( 'NONE',  ( 4.458734124999999437, -167.6875000013655779, 0.000000000000000000 ) ) ;
#23933=CARTESIAN_POINT ( 'NONE',  ( -3.152548672688508926E-16, -29.56249999863440436, -5.148502694627439702 ) ) ;
#23935=FACE_OUTER_BOUND ( 'NONE', #10407, .T. ) ;
#23937=CARTESIAN_POINT ( 'NONE',  ( 4.458734124999999437, -144.5000000013656063, 1.846868145590737864 ) ) ;
#23939=CARTESIAN_POINT ( 'NONE',  ( -4.458734124999998549, 28.52083333469892423, 2.574251347313722516 ) ) ;
#23941=CARTESIAN_POINT ( 'NONE',  ( 2.229367062499998831, -54.89583333196773651, -3.861377020970580887 ) ) ;
#23943=CARTESIAN_POINT ( 'NONE',  ( 5.000000000000000000, 13.70833333606451987, -2.886751345948130876 ) ) ;
#23944=CARTESIAN_POINT ( 'NONE',  ( -5.000000000000000000, 17.00000000000000000, 0.000000000000000000 ) ) ;
#23946=CARTESIAN_POINT ( 'NONE',  ( 4.458734125000001214, -3.895833331967739621, 2.574251347313718519 ) ) ;
#23947=CARTESIAN_POINT ( 'NONE',  ( -2.499999999999996447, 4.291666669397852907, 4.330127018922195425 ) ) ;
#23948=CARTESIAN_POINT ( 'NONE',  ( -2.229367062500000163, 10.27083333469892779, -3.861377020970580443 ) ) ;
#23950=CARTESIAN_POINT ( 'NONE',  ( 4.458734125000001214, -53.89583333196773651, 2.574251347313718519 ) ) ;
#23951=CARTESIAN_POINT ( 'NONE',  ( -8.190561711645485556E-16, -159.9375000013655779, 4.458734124999999437 ) ) ;
#23953=CARTESIAN_POINT ( 'NONE',  ( 2.500000000000002220, -52.54166666393548013, 4.330127018922192761 ) ) ;
#23954=VERTEX_POINT ( 'NONE', #13431 ) ;
#23955=CARTESIAN_POINT ( 'NONE',  ( -4.458734124999999437, 2.437500001365593860, 0.000000000000000000 ) ) ;
#23956=ORIENTED_EDGE ( 'NONE', *, *, #42064, .F. ) ;
#23959=CARTESIAN_POINT ( 'NONE',  ( 3.152801135295367541, -160.3125000013656063, -3.152801135295367541 ) ) ;
#23960=ORIENTED_EDGE ( 'NONE', *, *, #4725, .T. ) ;
#23962=CARTESIAN_POINT ( 'NONE',  ( 1.975475456537005874E-15, -83.74999999999998579, 5.000000000000000000 ) ) ;
#23965=CARTESIAN_POINT ( 'NONE',  ( -4.458734124999999437, -38.56249999863440081, 0.000000000000000000 ) ) ;
#23967=VECTOR ( 'NONE', #44946, 1000.000000000000114 ) ;
#23968=CARTESIAN_POINT ( 'NONE',  ( 3.535533905932738197, -143.0000000027311842, -3.535533905932738197 ) ) ;
#23971=CARTESIAN_POINT ( 'NONE',  ( 1.339745962155615144, -24.58034179853029499, 4.999999999999999112 ) ) ;
#23972=ORIENTED_EDGE ( 'NONE', *, *, #61683, .F. ) ;
#23973=EDGE_CURVE ( 'NONE', #55402, #59225, #14993, .T. ) ;
#23974=CARTESIAN_POINT ( 'NONE',  ( -4.458734124999999437, -83.56249999863439371, 0.000000000000000000 ) ) ;
#23976=CARTESIAN_POINT ( 'NONE',  ( 1.975475456537005874E-15, -40.74999999999999289, 5.000000000000000000 ) ) ;
#23985=CARTESIAN_POINT ( 'NONE',  ( 0.000000000000000000, -170.0000000000000000, 0.000000000000000000 ) ) ;
#23987=CARTESIAN_POINT ( 'NONE',  ( -4.458734124999998549, -82.47916666530106511, 2.574251347313722516 ) ) ;
#23991=CARTESIAN_POINT ( 'NONE',  ( -1.339745962155610925, -16.66965819600733312, 5.000000000000000000 ) ) ;
#23993=CARTESIAN_POINT ( 'NONE',  ( -5.000000000000000888, -161.6875000027312126, -2.071067811865475949 ) ) ;
#23998=( BOUNDED_CURVE ( )  B_SPLINE_CURVE ( 2, ( #62102, #47301, #52452, #47607, #2937, #42778, #33144, #18019, #56336 ),
 .UNSPECIFIED., .F., .F. ) 
 B_SPLINE_CURVE_WITH_KNOTS ( ( 3, 2, 2, 2, 3 ),
 ( 0.5937500000000000000, 0.5944444444444444420, 0.5958333333333333259, 0.5972222222222222099, 0.5979166666666666519 ),
 .UNSPECIFIED. ) 
 CURVE ( )  GEOMETRIC_REPRESENTATION_ITEM ( )  RATIONAL_B_SPLINE_CURVE ( ( 0.9330127018922194093, 0.9330127018922194093, 1.000000000000000000, 0.8660254037844387076, 1.000000000000000000, 0.8660254037844387076, 1.000000000000000000, 0.9330127018922194093, 0.9330127018922194093 ) ) 
 REPRESENTATION_ITEM ( '' )  );
#24005=CARTESIAN_POINT ( 'NONE',  ( -3.152548672688508926E-16, -15.56249999863440614, -5.148502694627439702 ) ) ;
#24007=CARTESIAN_POINT ( 'NONE',  ( 2.071067811865476394, -155.1875000000000000, 5.000000000000000000 ) ) ;
#24008=ORIENTED_EDGE ( 'NONE', *, *, #6348, .T. ) ;
#24009=CARTESIAN_POINT ( 'NONE',  ( -2.229367062500000163, -42.72916666530107932, -3.861377020970580443 ) ) ;
#24010=CARTESIAN_POINT ( 'NONE',  ( 5.000000000000000000, -77.50000000000000000, -6.123233995736766282E-16 ) ) ;
#24012=CARTESIAN_POINT ( 'NONE',  ( -5.000000000000000000, 27.04166666939785202, -2.886751345948128211 ) ) ;
#24015=AXIS2_PLACEMENT_3D ( 'NONE', #20839, #11176, #30799 ) ;
#24016=CARTESIAN_POINT ( 'NONE',  ( -3.152548672688508926E-16, 8.437500001365595637, -5.148502694627439702 ) ) ;
#24019=CARTESIAN_POINT ( 'NONE',  ( -5.000000000000000000, 11.91666666666666607, -2.886751345948128211 ) ) ;
#24021=CARTESIAN_POINT ( 'NONE',  ( 2.500000000000002220, 15.45833333606451987, 4.330127018922192761 ) ) ;
#24028=CARTESIAN_POINT ( 'NONE',  ( -5.000000000000000000, -36.00000000000000711, 0.000000000000000000 ) ) ;
#24029=CARTESIAN_POINT ( 'NONE',  ( 9.457646018065525792E-16, -38.06249999863441502, 5.148502694627439702 ) ) ;
#24030=ADVANCED_FACE ( 'NONE', ( #52979 ), #8920, .T. ) ;
#24031=CARTESIAN_POINT ( 'NONE',  ( -5.000000000000000000, -34.87499999726881583, 0.000000000000000000 ) ) ;
#24032=EDGE_CURVE ( 'NONE', #18740, #43422, #32664, .T. ) ;
#24033=CARTESIAN_POINT ( 'NONE',  ( -2.229367062499996610, -65.14583333196773651, 3.861377020970582219 ) ) ;
#24036=CARTESIAN_POINT ( 'NONE',  ( 2.229367062499998831, -13.64583333196774184, -3.861377020970580887 ) ) ;
#24037=CARTESIAN_POINT ( 'NONE',  ( -4.458734124999998549, -12.47916666530107221, 2.574251347313722516 ) ) ;
#24038=ORIENTED_EDGE ( 'NONE', *, *, #1270, .T. ) ;
#24040=CARTESIAN_POINT ( 'NONE',  ( 5.000000000000000000, -77.41666666666665719, -2.886751345948129988 ) ) ;
#24043=CARTESIAN_POINT ( 'NONE',  ( -4.999999999999999112, -82.79166666393547303, 2.886751345948131764 ) ) ;
#24048=CARTESIAN_POINT ( 'NONE',  ( 4.458734125000001214, -24.14583333196773651, 2.574251347313718519 ) ) ;
#24050=CARTESIAN_POINT ( 'NONE',  ( -2.229367062499996610, -60.39583333196774362, 3.861377020970582219 ) ) ;
#24052=CARTESIAN_POINT ( 'NONE',  ( 2.730187237215162345E-16, -165.4375000013655779, -4.458734124999999437 ) ) ;
#24053=ADVANCED_FACE ( 'NONE', ( #20397 ), #789, .T. ) ;
#24055=CARTESIAN_POINT ( 'NONE',  ( -9.184850993605147944E-16, -167.3750000027312126, 5.000000000000000000 ) ) ;
#24056=ORIENTED_EDGE ( 'NONE', *, *, #31015, .F. ) ;
#24063=CARTESIAN_POINT ( 'NONE',  ( 2.500000000000002220, 18.33333333333333215, 4.330127018922192761 ) ) ;
#24067=CARTESIAN_POINT ( 'NONE',  ( -1.846868145590734756, -145.3750000013656347, -4.458734125000000326 ) ) ;
#24071=CARTESIAN_POINT ( 'NONE',  ( -2.229367062499996610, -68.39583333196773651, 3.861377020970582219 ) ) ;
#24072=CARTESIAN_POINT ( 'NONE',  ( 2.500000000000002220, -43.66666666666665719, 4.330127018922192761 ) ) ;
#24073=CARTESIAN_POINT ( 'NONE',  ( -5.000000000000000000, -0.8749999972688139449, 0.000000000000000000 ) ) ;
#24074=CARTESIAN_POINT ( 'NONE',  ( 4.458734124999999437, -140.4375000013656063, 0.000000000000000000 ) ) ;
#24077=VERTEX_POINT ( 'NONE', #1435 ) ;
#24084=CARTESIAN_POINT ( 'NONE',  ( -4.458734124999997661, 20.52083333469892423, 2.574251347313722516 ) ) ;
#24091=CARTESIAN_POINT ( 'NONE',  ( -2.229367062500000163, 1.520833334698927564, -3.861377020970580443 ) ) ;
#24093=CARTESIAN_POINT ( 'NONE',  ( -2.229367062499996610, -27.39583333196774007, 3.861377020970582219 ) ) ;
#24094=CARTESIAN_POINT ( 'NONE',  ( -3.152801135295367096, -157.0625000013656063, -3.152801135295367541 ) ) ;
#24097=CARTESIAN_POINT ( 'NONE',  ( 4.458734124999998549, 27.27083333469892423, -2.574251347313721627 ) ) ;
#24100=CARTESIAN_POINT ( 'NONE',  ( 9.457646018065525792E-16, -70.31249999863439371, 5.148502694627439702 ) ) ;
#24103=CARTESIAN_POINT ( 'NONE',  ( -5.000000000000000000, 29.04166666939784847, -2.886751345948128211 ) ) ;
#24105=CARTESIAN_POINT ( 'NONE',  ( 4.458734124999999437, -169.5625000013655779, 0.000000000000000000 ) ) ;
#24107=CARTESIAN_POINT ( 'NONE',  ( 2.499999999999998668, -6.208333330602149758, -4.330127018922193649 ) ) ;
#24108=CARTESIAN_POINT ( 'NONE',  ( -2.499999999999996447, -12.83333333333333570, 4.330127018922195425 ) ) ;
#24109=CARTESIAN_POINT ( 'NONE',  ( 4.458734124999998549, -16.72916666530107577, -2.574251347313721627 ) ) ;
#24110=CARTESIAN_POINT ( 'NONE',  ( -2.229367062500000163, -76.47916666530106511, -3.861377020970580443 ) ) ;
#24111=AXIS2_PLACEMENT_3D ( 'NONE', #23810, #19285, #38287 ) ;
#24112=CARTESIAN_POINT ( 'NONE',  ( 3.152801135295366208, -168.8125000013656063, 3.152801135295367985 ) ) ;
#24113=CARTESIAN_POINT ( 'NONE',  ( 2.499999999999998668, -17.20833333060214443, -4.330127018922193649 ) ) ;
#24114=CARTESIAN_POINT ( 'NONE',  ( -4.458734124999999437, -49.39583333196773651, -2.574251347313719407 ) ) ;
#24116=CARTESIAN_POINT ( 'NONE',  ( -3.152548672688508926E-16, 2.187500001365593416, -5.148502694627439702 ) ) ;
#24119=CARTESIAN_POINT ( 'NONE',  ( 5.000000000000000888, -58.58333333333333570, 2.886751345948126879 ) ) ;
#24120=CARTESIAN_POINT ( 'NONE',  ( -4.458734124999999437, -158.1875000013655779, -5.460374474430324690E-16 ) ) ;
#24122=CARTESIAN_POINT ( 'NONE',  ( -2.499999999999996447, -64.83333333333332860, 4.330127018922195425 ) ) ;
#24123=CARTESIAN_POINT ( 'NONE',  ( 3.061616997868383141E-16, -160.7500000000000000, -5.000000000000000000 ) ) ;
#24124=CARTESIAN_POINT ( 'NONE',  ( 1.339745962155615144, 5.419658201469705894, 4.999999999999999112 ) ) ;
#24126=CARTESIAN_POINT ( 'NONE',  ( -4.458734124999998549, -3.479166665301069994, 2.574251347313722516 ) ) ;
#24127=CARTESIAN_POINT ( 'NONE',  ( -4.458734124999999437, -45.64583333196774362, -2.574251347313719407 ) ) ;
#24128=DIRECTION ( 'NONE',  ( -0.000000000000000000, 1.000000000000000000, -0.000000000000000000 ) ) ;
#24129=CARTESIAN_POINT ( 'NONE',  ( -8.190561711645485556E-16, -148.6875000013656063, 4.458734124999999437 ) ) ;
#24132=VERTEX_POINT ( 'NONE', #5925 ) ;
#24133=EDGE_CURVE ( 'NONE', #51592, #39210, #6244, .T. ) ;
#24136=VERTEX_POINT ( 'NONE', #16204 ) ;
#24137=EDGE_CURVE ( 'NONE', #55402, #25522, #36146, .T. ) ;
#24141=CARTESIAN_POINT ( 'NONE',  ( 2.229367062500001939, -2.979166665301069550, 3.861377020970579999 ) ) ;
#24143=CARTESIAN_POINT ( 'NONE',  ( 4.458734124999999437, -152.4375000013655779, 0.000000000000000000 ) ) ;
#24150=LINE ( 'NONE', #9042, #12863 ) ;
#24158=CARTESIAN_POINT ( 'NONE',  ( 2.229367062500001939, 15.02083333469892779, 3.861377020970579999 ) ) ;
#24160=CARTESIAN_POINT ( 'NONE',  ( -2.229367062499996610, -10.39583333196773829, 3.861377020970582219 ) ) ;
#24163=CARTESIAN_POINT ( 'NONE',  ( -1.846868145590737420, -167.7500000013655779, 4.458734124999999437 ) ) ;
#24170=CARTESIAN_POINT ( 'NONE',  ( -1.846868145590737420, -155.0000000013656063, 4.458734124999997661 ) ) ;
#24174=ORIENTED_EDGE ( 'NONE', *, *, #54198, .T. ) ;
#24177=CARTESIAN_POINT ( 'NONE',  ( -3.535250795749689387E-16, 3.750000000000000000, -5.773502691896257311 ) ) ;
#24178=CARTESIAN_POINT ( 'NONE',  ( 4.458734124999999437, -61.81249999863440081, -5.460374474430324690E-16 ) ) ;
#24180=CARTESIAN_POINT ( 'NONE',  ( -5.000000000000000000, 19.91666666666666430, -2.886751345948128211 ) ) ;
#24181=CARTESIAN_POINT ( 'NONE',  ( 2.500000000000002220, -1.541666663935480130, 4.330127018922192761 ) ) ;
#24182=CARTESIAN_POINT ( 'NONE',  ( 2.229367062499998831, -30.64583333196773651, -3.861377020970580887 ) ) ;
#24185=CARTESIAN_POINT ( 'NONE',  ( 5.000000000000000000, 5.583333333333332149, -2.886751345948130876 ) ) ;
#24186=CARTESIAN_POINT ( 'NONE',  ( -5.000000000000000000, -43.00000000000000000, 0.000000000000000000 ) ) ;
#24187=CARTESIAN_POINT ( 'NONE',  ( 6.123233995736766282E-16, -170.0000000000000000, -5.000000000000000000 ) ) ;
#24190=CARTESIAN_POINT ( 'NONE',  ( 2.229367062500001939, -70.97916666530107932, 3.861377020970579999 ) ) ;
#24191=CARTESIAN_POINT ( 'NONE',  ( 4.458734124999999437, -144.6875000013656063, 0.000000000000000000 ) ) ;
#24192=CARTESIAN_POINT ( 'NONE',  ( 2.229367062500001939, -78.97916666530106511, 3.861377020970579999 ) ) ;
#24195=CARTESIAN_POINT ( 'NONE',  ( 2.229367062499998831, -23.89583333196773651, -3.861377020970580887 ) ) ;
#24196=( BOUNDED_CURVE ( )  B_SPLINE_CURVE ( 2, ( #55329, #1623, #11246, #54366, #10294, #44694, #59514, #15448, #35066 ),
 .UNSPECIFIED., .F., .F. ) 
 B_SPLINE_CURVE_WITH_KNOTS ( ( 3, 2, 2, 2, 3 ),
 ( 0.4104166666666666519, 0.4111111111111110938, 0.4124999999999999778, 0.4138888888888888618, 0.4145833333333333592 ),
 .UNSPECIFIED. ) 
 CURVE ( )  GEOMETRIC_REPRESENTATION_ITEM ( )  RATIONAL_B_SPLINE_CURVE ( ( 0.9330127018922194093, 0.9330127018922194093, 1.000000000000000000, 0.8660254037844387076, 1.000000000000000000, 0.8660254037844387076, 1.000000000000000000, 0.9330127018922167448, 0.9330127018922194093 ) ) 
 REPRESENTATION_ITEM ( '' )  );
#24197=CARTESIAN_POINT ( 'NONE',  ( -4.999999999999999112, -67.79166666393547303, 2.886751345948131764 ) ) ;
#24200=ORIENTED_EDGE ( 'NONE', *, *, #7932, .T. ) ;
#24206=LINE ( 'NONE', #48954, #36332 ) ;
#24207=CARTESIAN_POINT ( 'NONE',  ( 4.458734124999998549, -59.97916666530107221, -2.574251347313721627 ) ) ;
#24209=ORIENTED_EDGE ( 'NONE', *, *, #62983, .F. ) ;
#24211=CYLINDRICAL_SURFACE ( 'NONE', #8947, 5.000000000000000000 ) ;
#24212=CARTESIAN_POINT ( 'NONE',  ( -4.458734124999999437, 10.68750000136559386, 0.000000000000000000 ) ) ;
#24215=CARTESIAN_POINT ( 'NONE',  ( 2.730187237215162345E-16, -164.1875000013655779, -4.458734124999999437 ) ) ;
#24225=CARTESIAN_POINT ( 'NONE',  ( 1.975475456537005874E-15, -82.62499999726878741, 5.000000000000000000 ) ) ;
#24229=CARTESIAN_POINT ( 'NONE',  ( -4.458734124999997661, 6.520833334698930450, 2.574251347313722516 ) ) ;
#24232=CARTESIAN_POINT ( 'NONE',  ( -3.535533905932738641, -149.5000000027311842, 3.535533905932737309 ) ) ;
#24237=AXIS2_PLACEMENT_3D ( 'NONE', #48038, #23915, #62849 ) ;
#24239=CARTESIAN_POINT ( 'NONE',  ( -3.535533905932738641, -144.3750000000000000, 3.535533905932737309 ) ) ;
#24241=CARTESIAN_POINT ( 'NONE',  ( -3.152801135295367985, -164.0625000013656063, 3.152801135295367096 ) ) ;
#24242=CARTESIAN_POINT ( 'NONE',  ( -4.458734124999999437, -31.39583333196773296, -2.574251347313719407 ) ) ;
#24246=CARTESIAN_POINT ( 'NONE',  ( 1.846868145590735200, -144.2500000013656063, -4.458734125000000326 ) ) ;
#24248=CARTESIAN_POINT ( 'NONE',  ( -4.458734124999999437, 26.35416666803226349, -2.574251347313719407 ) ) ;
#24250=CARTESIAN_POINT ( 'NONE',  ( 4.458734124999998549, -56.97916666530107932, -2.574251347313721627 ) ) ;
#24251=( BOUNDED_CURVE ( )  B_SPLINE_CURVE ( 2, ( #56546, #42044, #32399, #22765, #61686, #37233, #37540, #42360, #61999 ),
 .UNSPECIFIED., .F., .F. ) 
 B_SPLINE_CURVE_WITH_KNOTS ( ( 3, 2, 2, 2, 3 ),
 ( 0.4229166666666666630, 0.4236111111111111049, 0.4249999999999999889, 0.4263888888888888729, 0.4270833333333333148 ),
 .UNSPECIFIED. ) 
 CURVE ( )  GEOMETRIC_REPRESENTATION_ITEM ( )  RATIONAL_B_SPLINE_CURVE ( ( 0.9330127018922194093, 0.9330127018922194093, 1.000000000000000000, 0.8660254037844387076, 1.000000000000000000, 0.8660254037844387076, 1.000000000000000000, 0.9330127018922194093, 0.9330127018922194093 ) ) 
 REPRESENTATION_ITEM ( '' )  );
#24254=CARTESIAN_POINT ( 'NONE',  ( -3.535250795749689387E-16, 20.74999999999999645, -5.773502691896257311 ) ) ;
#24256=CARTESIAN_POINT ( 'NONE',  ( -3.152548672688508926E-16, -5.562499998634402587, -5.148502694627439702 ) ) ;
#24262=CARTESIAN_POINT ( 'NONE',  ( -3.152548672688508926E-16, -55.56249999863440081, -5.148502694627439702 ) ) ;
#24263=CARTESIAN_POINT ( 'NONE',  ( 2.730187237215162345E-16, -156.4375000013655779, -4.458734124999999437 ) ) ;
#24264=CARTESIAN_POINT ( 'NONE',  ( -2.500000000000000444, -51.04166666393547303, -4.330127018922193649 ) ) ;
#24266=CARTESIAN_POINT ( 'NONE',  ( -2.229367062500000163, 5.270833334698927786, -3.861377020970580443 ) ) ;
#24270=CARTESIAN_POINT ( 'NONE',  ( -3.152801135295367096, -159.0625000013656063, -3.152801135295367541 ) ) ;
#24274=CARTESIAN_POINT ( 'NONE',  ( -6.972266317189433020E-16, -87.12499999726880162, -5.000000000000000000 ) ) ;
#24276=DIRECTION ( 'NONE',  ( -0.000000000000000000, 1.000000000000000000, -0.000000000000000000 ) ) ;
#24277=CARTESIAN_POINT ( 'NONE',  ( -3.152548672688508926E-16, -45.81249999863440081, -5.148502694627439702 ) ) ;
#24278=AXIS2_PLACEMENT_3D ( 'NONE', #3222, #21883, #12853 ) ;
#24281=CARTESIAN_POINT ( 'NONE',  ( 1.975475456537005874E-15, -45.74999999999999289, 5.000000000000000000 ) ) ;
#24284=CARTESIAN_POINT ( 'NONE',  ( -4.458734124999998549, 26.77083333469893134, 2.574251347313722516 ) ) ;
#24288=( BOUNDED_CURVE ( )  B_SPLINE_CURVE ( 2, ( #37726, #8463, #28071, #47688, #57674, #33219, #52837, #59239, #15172 ),
 .UNSPECIFIED., .F., .F. ) 
 B_SPLINE_CURVE_WITH_KNOTS ( ( 3, 2, 2, 2, 3 ),
 ( 0.4604166666666666963, 0.4611111111111111382, 0.4625000000000000222, 0.4638888888888889062, 0.4645833333333333481 ),
 .UNSPECIFIED. ) 
 CURVE ( )  GEOMETRIC_REPRESENTATION_ITEM ( )  RATIONAL_B_SPLINE_CURVE ( ( 0.9330127018922194093, 0.9330127018922220739, 1.000000000000000000, 0.8660254037844387076, 1.000000000000000000, 0.8660254037844387076, 1.000000000000000000, 0.9330127018922194093, 0.9330127018922194093 ) ) 
 REPRESENTATION_ITEM ( '' )  );
#24289=CARTESIAN_POINT ( 'NONE',  ( 1.339745962155612702, -52.16965819600733312, -5.000000000000000000 ) ) ;
#24291=CARTESIAN_POINT ( 'NONE',  ( -2.500000000000000444, 9.958333336064519870, -4.330127018922193649 ) ) ;
#24296=CYLINDRICAL_SURFACE ( 'NONE', #32468, 5.000000000000000000 ) ;
#24297=CARTESIAN_POINT ( 'NONE',  ( -1.339745962155610925, -19.66965819600733667, 5.000000000000000000 ) ) ;
#24298=CARTESIAN_POINT ( 'NONE',  ( -4.458734124999999437, -89.56249999863440792, 0.000000000000000000 ) ) ;
#24301=ORIENTED_EDGE ( 'NONE', *, *, #49967, .F. ) ;
#24302=CARTESIAN_POINT ( 'NONE',  ( -1.339745962155610925, -80.79465819873850307, 5.000000000000000000 ) ) ;
#24304=CARTESIAN_POINT ( 'NONE',  ( 5.000000000000000000, -161.1250000027311842, 0.000000000000000000 ) ) ;
#24307=CARTESIAN_POINT ( 'NONE',  ( -2.499999999999996447, 22.16666666666666785, 4.330127018922195425 ) ) ;
#24314=CARTESIAN_POINT ( 'NONE',  ( -5.000000000000000000, -53.99999999999999289, 0.000000000000000000 ) ) ;
#24315=CARTESIAN_POINT ( 'NONE',  ( -4.458734124999999437, -15.39583333196773651, -2.574251347313719407 ) ) ;
#24316=CARTESIAN_POINT ( 'NONE',  ( 6.123233995736766282E-16, -170.0000000000000000, -5.000000000000000000 ) ) ;
#24317=CARTESIAN_POINT ( 'NONE',  ( -2.071067811865478170, -156.3125000000000284, 5.000000000000000000 ) ) ;
#24320=CARTESIAN_POINT ( 'NONE',  ( -2.229367062500000163, -40.72916666530107221, -3.861377020970580443 ) ) ;
#24321=VECTOR ( 'NONE', #34194, 1000.000000000000000 ) ;
#24328=VECTOR ( 'NONE', #52528, 1000.000000000000000 ) ;
#24330=CARTESIAN_POINT ( 'NONE',  ( 9.457646018065525792E-16, 8.937500001365597413, 5.148502694627439702 ) ) ;
#24332=CARTESIAN_POINT ( 'NONE',  ( -6.972266317189433020E-16, -44.25000000000000000, -5.000000000000000000 ) ) ;
#24333=ADVANCED_FACE ( 'NONE', ( #42856 ), #17485, .T. ) ;
#24335=CARTESIAN_POINT ( 'NONE',  ( -3.152548672688508926E-16, -88.81249999863439371, -5.148502694627439702 ) ) ;
#24336=CARTESIAN_POINT ( 'NONE',  ( 4.458734124999999437, 22.93750000136559564, -5.460374474430324690E-16 ) ) ;
#24338=CARTESIAN_POINT ( 'NONE',  ( -2.499999999999996447, 14.29166666939785202, 4.330127018922195425 ) ) ;
#24340=CARTESIAN_POINT ( 'NONE',  ( 0.000000000000000000, -170.0000000000000000, 0.000000000000000000 ) ) ;
#24341=ORIENTED_EDGE ( 'NONE', *, *, #50324, .F. ) ;
#24342=CARTESIAN_POINT ( 'NONE',  ( 5.000000000000000000, -85.41666666666665719, -2.886751345948130876 ) ) ;
#24343=CARTESIAN_POINT ( 'NONE',  ( 5.000000000000000000, -32.50000000000000000, -6.123233995736766282E-16 ) ) ;
#24344=CARTESIAN_POINT ( 'NONE',  ( -4.458734124999999437, -36.39583333196772941, -2.574251347313719407 ) ) ;
#24346=CARTESIAN_POINT ( 'NONE',  ( -3.535250795749689387E-16, -33.12499999726881583, -5.773502691896257311 ) ) ;
#24347=CARTESIAN_POINT ( 'NONE',  ( 2.229367062500001939, -67.97916666530106511, 3.861377020970579999 ) ) ;
#24350=CARTESIAN_POINT ( 'NONE',  ( -2.229367062500000163, -14.47916666530107221, -3.861377020970580443 ) ) ;
#24351=CARTESIAN_POINT ( 'NONE',  ( 4.458734125000001214, -14.14583333196774184, 2.574251347313718519 ) ) ;
#24353=CARTESIAN_POINT ( 'NONE',  ( 2.500000000000002220, -81.66666666666667140, 4.330127018922192761 ) ) ;
#24356=CARTESIAN_POINT ( 'NONE',  ( -2.499999999999996447, -84.70833333060214443, 4.330127018922195425 ) ) ;
#24360=CARTESIAN_POINT ( 'NONE',  ( -4.458734124999999437, -28.56249999863440081, 0.000000000000000000 ) ) ;
#24362=CARTESIAN_POINT ( 'NONE',  ( 2.730187237215162345E-16, -168.4375000013656063, -4.458734124999999437 ) ) ;
#24363=EDGE_CURVE ( 'NONE', #33925, #15736, #10485, .T. ) ;
#24365=CARTESIAN_POINT ( 'NONE',  ( -5.000000000000000888, -167.6875000027311842, -2.071067811865475949 ) ) ;
#24366=ORIENTED_EDGE ( 'NONE', *, *, #55953, .T. ) ;
#24372=VECTOR ( 'NONE', #13188, 1000.000000000000000 ) ;
#24378=CARTESIAN_POINT ( 'NONE',  ( -3.152801135295367985, -144.0625000013655779, 3.152801135295367096 ) ) ;
#24382=CARTESIAN_POINT ( 'NONE',  ( 2.229367062500001939, -66.22916666530106511, 3.861377020970579999 ) ) ;
#24384=CYLINDRICAL_SURFACE ( 'NONE', #60392, 5.000000000000000000 ) ;
#24385=CARTESIAN_POINT ( 'NONE',  ( -4.458734124999999437, -139.9375000013656063, -5.460374474430324690E-16 ) ) ;
#24387=ORIENTED_EDGE ( 'NONE', *, *, #22917, .F. ) ;
#24393=CARTESIAN_POINT ( 'NONE',  ( -2.229367062499996610, 25.60416666803225993, 3.861377020970582219 ) ) ;
#24394=CARTESIAN_POINT ( 'NONE',  ( -5.000000000000000000, 26.91666666666666430, -2.886751345948128211 ) ) ;
#24396=EDGE_CURVE ( 'NONE', #44687, #30129, #60674, .T. ) ;
#24397=ADVANCED_FACE ( 'NONE', ( #37723 ), #2687, .T. ) ;
#24401=CYLINDRICAL_SURFACE ( 'NONE', #28420, 5.000000000000000000 ) ;
#24402=CARTESIAN_POINT ( 'NONE',  ( 4.458734124999999437, 0.1875000013655953035, -5.460374474430324690E-16 ) ) ;
#24404=CARTESIAN_POINT ( 'NONE',  ( 4.458734124999999437, -23.06249999863440436, -5.460374474430324690E-16 ) ) ;
#24408=CARTESIAN_POINT ( 'NONE',  ( -4.458734124999999437, 26.68750000136559564, 0.000000000000000000 ) ) ;
#24412=CARTESIAN_POINT ( 'NONE',  ( -4.458734124999997661, -74.47916666530106511, 2.574251347313722516 ) ) ;
#24415=CARTESIAN_POINT ( 'NONE',  ( 3.061616997868383141E-16, -155.8750000027311842, -5.000000000000000000 ) ) ;
#24416=ORIENTED_EDGE ( 'NONE', *, *, #42491, .F. ) ;
#24418=CARTESIAN_POINT ( 'NONE',  ( -6.972266317189433020E-16, -43.12499999726880873, -5.000000000000000000 ) ) ;
#24419=CARTESIAN_POINT ( 'NONE',  ( -5.000000000000000000, -17.00000000000000000, 0.000000000000000000 ) ) ;
#24420=CARTESIAN_POINT ( 'NONE',  ( -4.458734124999998549, -21.22916666530107221, 2.574251347313722516 ) ) ;
#24421=CARTESIAN_POINT ( 'NONE',  ( -4.458734124999997661, -84.22916666530107932, 2.574251347313722516 ) ) ;
#24422=CARTESIAN_POINT ( 'NONE',  ( -4.458734125000001214, -169.1250000013656347, 1.846868145590734089 ) ) ;
#24423=CARTESIAN_POINT ( 'NONE',  ( -5.000000000000000000, -16.95833333060214443, -2.886751345948128211 ) ) ;
#24424=CARTESIAN_POINT ( 'NONE',  ( -2.229367062499996610, -50.14583333196772941, 3.861377020970582219 ) ) ;
#24427=CARTESIAN_POINT ( 'NONE',  ( 3.061616997868383141E-16, -164.8750000027311842, -5.000000000000000000 ) ) ;
#24428=CARTESIAN_POINT ( 'NONE',  ( -4.458734124999999437, -0.5624999986344053626, 0.000000000000000000 ) ) ;
#24429=ORIENTED_EDGE ( 'NONE', *, *, #59887, .T. ) ;
#24431=CARTESIAN_POINT ( 'NONE',  ( -4.999999999999999112, -60.91666666666666430, 2.886751345948131764 ) ) ;
#24432=CARTESIAN_POINT ( 'NONE',  ( 4.458734124999999437, -157.7500000013656063, 1.846868145590737864 ) ) ;
#24434=CARTESIAN_POINT ( 'NONE',  ( -5.000000000000000000, -65.00000000000000000, 0.000000000000000000 ) ) ;
#24435=CARTESIAN_POINT ( 'NONE',  ( -5.000000000000000888, -160.5625000000000284, -2.071067811865475949 ) ) ;
#24437=CARTESIAN_POINT ( 'NONE',  ( -4.458734124999999437, -9.562499998634406140, 0.000000000000000000 ) ) ;
#24438=CARTESIAN_POINT ( 'NONE',  ( 2.229367062499998831, -48.89583333196772941, -3.861377020970580887 ) ) ;
#24440=CARTESIAN_POINT ( 'NONE',  ( 1.846868145590735200, -148.2500000013656063, -4.458734125000000326 ) ) ;
#24443=ORIENTED_EDGE ( 'NONE', *, *, #50294, .T. ) ;
#24445=CARTESIAN_POINT ( 'NONE',  ( -4.999999999999998224, -5.791666663935480130, 2.886751345948131764 ) ) ;
#24447=CARTESIAN_POINT ( 'NONE',  ( 2.499999999999998668, -29.20833333060214798, -4.330127018922193649 ) ) ;
#24452=CARTESIAN_POINT ( 'NONE',  ( -4.999999999999998224, -50.91666666666666430, 2.886751345948131764 ) ) ;
#24453=CARTESIAN_POINT ( 'NONE',  ( -4.458734124999999437, -2.395833331967737845, -2.574251347313719407 ) ) ;
#24455=CARTESIAN_POINT ( 'NONE',  ( -1.846868145590734756, -152.1250000013655779, -4.458734124999999437 ) ) ;
#24456=AXIS2_PLACEMENT_3D ( 'NONE', #41538, #6198, #16795 ) ;
#24458=ORIENTED_EDGE ( 'NONE', *, *, #27271, .F. ) ;
#24460=CARTESIAN_POINT ( 'NONE',  ( 0.000000000000000000, -170.0000000000000000, 5.000000000000000000 ) ) ;
#24461=CARTESIAN_POINT ( 'NONE',  ( 2.500000000000002220, -12.54166666393548013, 4.330127018922192761 ) ) ;
#24463=CARTESIAN_POINT ( 'NONE',  ( -2.500000000000000444, 27.95833333606451987, -4.330127018922193649 ) ) ;
#24464=LINE ( 'NONE', #54044, #27368 ) ;
#24472=CARTESIAN_POINT ( 'NONE',  ( -2.229367062499996610, 18.85416666803225993, 3.861377020970582219 ) ) ;
#24474=CARTESIAN_POINT ( 'NONE',  ( -2.229367062499996610, -9.395833331967736513, 3.861377020970582219 ) ) ;
#24478=CARTESIAN_POINT ( 'NONE',  ( -1.846868145590734756, -167.1250000013656063, -4.458734125000000326 ) ) ;
#24479=CARTESIAN_POINT ( 'NONE',  ( -5.000000000000000000, -20.95833333060214798, -2.886751345948128211 ) ) ;
#24483=VECTOR ( 'NONE', #24544, 1000.000000000000000 ) ;
#24485=CARTESIAN_POINT ( 'NONE',  ( -2.500000000000000444, -55.04166666393548013, -4.330127018922193649 ) ) ;
#24486=CARTESIAN_POINT ( 'NONE',  ( 5.000000000000000888, -69.58333333333332860, 2.886751345948126879 ) ) ;
#24487=CARTESIAN_POINT ( 'NONE',  ( 3.152801135295367541, -155.5625000013656063, -3.152801135295367541 ) ) ;
#24489=DIRECTION ( 'NONE',  ( 0.000000000000000000, 0.000000000000000000, 1.000000000000000000 ) ) ;
#24490=ADVANCED_FACE ( 'NONE', ( #19673 ), #47999, .T. ) ;
#24491=CARTESIAN_POINT ( 'NONE',  ( -9.184850993605147944E-16, -148.3750000027312126, 5.000000000000000000 ) ) ;
#24492=ORIENTED_EDGE ( 'NONE', *, *, #31896, .T. ) ;
#24496=EDGE_CURVE ( 'NONE', #20741, #62531, #21209, .T. ) ;
#24497=CARTESIAN_POINT ( 'NONE',  ( -5.000000000000000000, 0.000000000000000000, 0.000000000000000000 ) ) ;
#24498=CARTESIAN_POINT ( 'NONE',  ( 2.229367062500001939, -64.97916666530106511, 3.861377020970579999 ) ) ;
#24499=CARTESIAN_POINT ( 'NONE',  ( -2.500000000000000444, -31.04166666393548368, -4.330127018922193649 ) ) ;
#24500=EDGE_CURVE ( 'NONE', #14071, #39231, #39601, .T. ) ;
#24501=CARTESIAN_POINT ( 'NONE',  ( -5.000000000000000000, -2.874999997268815832, 0.000000000000000000 ) ) ;
#24502=CARTESIAN_POINT ( 'NONE',  ( -2.229367062499996610, -34.14583333196772941, 3.861377020970582219 ) ) ;
#24504=CARTESIAN_POINT ( 'NONE',  ( 1.339745962155615144, 17.41965820146970145, 4.999999999999999112 ) ) ;
#24507=CARTESIAN_POINT ( 'NONE',  ( 5.000000000000000888, -46.58333333333334991, 2.886751345948126879 ) ) ;
#24508=CARTESIAN_POINT ( 'NONE',  ( 3.061616997868383141E-16, -147.7500000000000284, -5.000000000000000000 ) ) ;
#24511=CARTESIAN_POINT ( 'NONE',  ( 2.499999999999998668, -4.208333330602147981, -4.330127018922193649 ) ) ;
#24512=CARTESIAN_POINT ( 'NONE',  ( 2.229367062499998831, -70.64583333196773651, -3.861377020970580887 ) ) ;
#24513=CARTESIAN_POINT ( 'NONE',  ( -4.458734125000000326, -145.2500000013655779, -1.846868145590735644 ) ) ;
#24514=CARTESIAN_POINT ( 'NONE',  ( 2.229367062499998831, -84.64583333196773651, -3.861377020970580887 ) ) ;
#24517=CARTESIAN_POINT ( 'NONE',  ( -3.152548672688508926E-16, -32.81249999863440792, -5.148502694627439702 ) ) ;
#24518=CARTESIAN_POINT ( 'NONE',  ( 5.000000000000000888, -70.45833333060214443, 2.886751345948126879 ) ) ;
#24523=CARTESIAN_POINT ( 'NONE',  ( 5.000000000000000000, -166.0000000000000000, 0.000000000000000000 ) ) ;
#24527=CARTESIAN_POINT ( 'NONE',  ( -4.458734124999999437, -56.64583333196773651, -2.574251347313719407 ) ) ;
#24529=VERTEX_POINT ( 'NONE', #54416 ) ;
#24530=CARTESIAN_POINT ( 'NONE',  ( 3.061616997868383141E-16, -146.7500000000000284, -5.000000000000000000 ) ) ;
#24532=CARTESIAN_POINT ( 'NONE',  ( -2.229367062500000163, 14.52083333469892779, -3.861377020970580443 ) ) ;
#24535=CARTESIAN_POINT ( 'NONE',  ( -4.458734124999999437, -166.0000000013656063, -1.846868145590735644 ) ) ;
#24538=CARTESIAN_POINT ( 'NONE',  ( -3.535533905932738641, -153.3750000000000000, 3.535533905932737309 ) ) ;
#24541=CARTESIAN_POINT ( 'NONE',  ( -1.339745962155610925, 2.205341801261479606, 5.000000000000000000 ) ) ;
#24544=DIRECTION ( 'NONE',  ( -0.000000000000000000, 1.000000000000000000, -0.000000000000000000 ) ) ;
#24548=PRODUCT ( 'pulling arm', 'pulling arm', '', ( #15349 ) ) ;
#24550=CARTESIAN_POINT ( 'NONE',  ( 9.457646018065525792E-16, 8.687500001365595637, 5.148502694627439702 ) ) ;
#24552=CARTESIAN_POINT ( 'NONE',  ( -6.972266317189433020E-16, -13.25000000000000000, -5.000000000000000000 ) ) ;
#24554=CARTESIAN_POINT ( 'NONE',  ( 3.061616997868383141E-16, -149.8750000027312126, -5.000000000000000000 ) ) ;
#24561=CARTESIAN_POINT ( 'NONE',  ( -5.000000000000000888, -141.4375000000000284, 2.071067811865474617 ) ) ;
#24563=CARTESIAN_POINT ( 'NONE',  ( -4.458734124999999437, -167.1875000013655779, -5.460374474430324690E-16 ) ) ;
#24564=CARTESIAN_POINT ( 'NONE',  ( 9.457646018065525792E-16, -28.06249999863440081, 5.148502694627439702 ) ) ;
#24565=CARTESIAN_POINT ( 'NONE',  ( -1.339745962155610925, -32.79465819873851729, 5.000000000000000000 ) ) ;
#24566=LINE ( 'NONE', #44812, #27687 ) ;
#24568=CARTESIAN_POINT ( 'NONE',  ( -1.846868145590737420, -143.7500000013655779, 4.458734124999999437 ) ) ;
#24569=ORIENTED_EDGE ( 'NONE', *, *, #36971, .F. ) ;
#24570=CARTESIAN_POINT ( 'NONE',  ( 1.060575238724906964E-15, -90.62499999726880162, 5.773502691896257311 ) ) ;
#24572=CARTESIAN_POINT ( 'NONE',  ( -4.458734124999997661, -64.47916666530106511, 2.574251347313722516 ) ) ;
#24575=CARTESIAN_POINT ( 'NONE',  ( -4.999999999999999112, 19.08333333333333570, 2.886751345948131764 ) ) ;
#24576=CARTESIAN_POINT ( 'NONE',  ( -4.458734124999999437, -49.39583333196772230, -2.574251347313719407 ) ) ;
#24577=CARTESIAN_POINT ( 'NONE',  ( -4.458734124999999437, -7.395833331967734736, -2.574251347313719407 ) ) ;
#24578=( BOUNDED_CURVE ( )  B_SPLINE_CURVE ( 2, ( #45185, #6283, #35543, #29414, #11088, #185, #25249, #827, #10136 ),
 .UNSPECIFIED., .F., .F. ) 
 B_SPLINE_CURVE_WITH_KNOTS ( ( 3, 2, 2, 2, 3 ),
 ( 0.8979166666666666963, 0.8986111111111111382, 0.9000000000000000222, 0.9013888888888889062, 0.9020833333333333481 ),
 .UNSPECIFIED. ) 
 CURVE ( )  GEOMETRIC_REPRESENTATION_ITEM ( )  RATIONAL_B_SPLINE_CURVE ( ( 0.9330127018922194093, 0.9330127018922194093, 1.000000000000000000, 0.8660254037844387076, 1.000000000000000000, 0.8660254037844387076, 1.000000000000000000, 0.9330127018922194093, 0.9330127018922194093 ) ) 
 REPRESENTATION_ITEM ( '' )  );
#24580=DIRECTION ( 'NONE',  ( 0.000000000000000000, 0.000000000000000000, 1.000000000000000000 ) ) ;
#24586=CARTESIAN_POINT ( 'NONE',  ( -2.229367062500000163, -55.47916666530107221, -3.861377020970580443 ) ) ;
#24587=CARTESIAN_POINT ( 'NONE',  ( 4.458734125000000326, -157.6250000013655779, -1.846868145590734978 ) ) ;
#24588=CARTESIAN_POINT ( 'NONE',  ( -4.999999999999999112, -47.79166666393548013, 2.886751345948131764 ) ) ;
#24590=CARTESIAN_POINT ( 'NONE',  ( 9.457646018065525792E-16, 6.687500001365594748, 5.148502694627439702 ) ) ;
#24591=VERTEX_POINT ( 'NONE', #9080 ) ;
#24594=CARTESIAN_POINT ( 'NONE',  ( -3.152801135295367985, -155.8125000013656063, 3.152801135295367096 ) ) ;
#24600=CARTESIAN_POINT ( 'NONE',  ( -2.229367062500000163, -44.72916666530106511, -3.861377020970580443 ) ) ;
#24604=DIRECTION ( 'NONE',  ( -0.000000000000000000, 1.000000000000000000, -0.000000000000000000 ) ) ;
#24605=ORIENTED_EDGE ( 'NONE', *, *, #46782, .T. ) ;
#24606=CARTESIAN_POINT ( 'NONE',  ( 2.229367062499998831, -88.89583333196773651, -3.861377020970580887 ) ) ;
#24610=CARTESIAN_POINT ( 'NONE',  ( 2.071067811865459962, -168.8124999999999716, -5.000000000000015987 ) ) ;
#24612=CARTESIAN_POINT ( 'NONE',  ( -4.999999999999998224, 10.20833333606451987, 2.886751345948131764 ) ) ;
#24614=FACE_OUTER_BOUND ( 'NONE', #7609, .T. ) ;
#24617=DIRECTION ( 'NONE',  ( 0.000000000000000000, 0.000000000000000000, 1.000000000000000000 ) ) ;
#24619=CARTESIAN_POINT ( 'NONE',  ( 2.229367062500001939, -90.22916666530106511, 3.861377020970579999 ) ) ;
#24624=CARTESIAN_POINT ( 'NONE',  ( -9.184850993605147944E-16, -169.2500000000000000, 5.000000000000000000 ) ) ;
#24626=CARTESIAN_POINT ( 'NONE',  ( -5.000000000000000888, -159.5625000027311842, 2.071067811865474617 ) ) ;
#24628=CARTESIAN_POINT ( 'NONE',  ( 3.535533905932738197, -163.0000000027312126, -3.535533905932738197 ) ) ;
#24636=DIRECTION ( 'NONE',  ( 0.000000000000000000, 0.000000000000000000, 1.000000000000000000 ) ) ;
#24637=CARTESIAN_POINT ( 'NONE',  ( 9.457646018065525792E-16, -13.06249999863440259, 5.148502694627439702 ) ) ;
#24639=CARTESIAN_POINT ( 'NONE',  ( 5.000000000000000000, -154.0000000000000284, 0.000000000000000000 ) ) ;
#24641=ORIENTED_EDGE ( 'NONE', *, *, #57552, .F. ) ;
#24642=CARTESIAN_POINT ( 'NONE',  ( 4.458734124999999437, -40.06249999863440081, -5.460374474430324690E-16 ) ) ;
#24643=CARTESIAN_POINT ( 'NONE',  ( 0.000000000000000000, -170.0000000000000000, 0.000000000000000000 ) ) ;
#24649=CARTESIAN_POINT ( 'NONE',  ( 4.458734125000001214, 10.10416666803226171, 2.574251347313718519 ) ) ;
#24651=CARTESIAN_POINT ( 'NONE',  ( -4.999999999999998224, 12.08333333333333215, 2.886751345948131764 ) ) ;
#24653=CARTESIAN_POINT ( 'NONE',  ( -4.458734124999999437, 23.35416666803226349, -2.574251347313719407 ) ) ;
#24655=CARTESIAN_POINT ( 'NONE',  ( 5.000000000000000000, 10.62500000273118594, -6.123233995736766282E-16 ) ) ;
#24656=ORIENTED_EDGE ( 'NONE', *, *, #44166, .T. ) ;
#24658=ORIENTED_EDGE ( 'NONE', *, *, #9525, .F. ) ;
#24660=CARTESIAN_POINT ( 'NONE',  ( 5.000000000000000888, -36.58333333333332149, 2.886751345948126879 ) ) ;
#24661=CARTESIAN_POINT ( 'NONE',  ( -3.152548672688508926E-16, -39.56249999863440081, -5.148502694627439702 ) ) ;
#24662=CARTESIAN_POINT ( 'NONE',  ( -5.000000000000000000, -32.87499999726880873, 0.000000000000000000 ) ) ;
#24663=CARTESIAN_POINT ( 'NONE',  ( 4.458734124999998549, -67.72916666530107932, -2.574251347313721627 ) ) ;
#24664=VERTEX_POINT ( 'NONE', #23573 ) ;
#24666=CARTESIAN_POINT ( 'NONE',  ( -4.458734124999999437, -15.31249999863440436, 0.000000000000000000 ) ) ;
#24667=CARTESIAN_POINT ( 'NONE',  ( -2.229367062500000163, -16.72916666530107577, -3.861377020970580443 ) ) ;
#24669=CARTESIAN_POINT ( 'NONE',  ( 2.499999999999998668, -82.33333333333332860, -4.330127018922193649 ) ) ;
#24670=CARTESIAN_POINT ( 'NONE',  ( 1.846868145590736310, -167.6250000013655779, 4.458734124999999437 ) ) ;
#24672=( BOUNDED_CURVE ( )  B_SPLINE_CURVE ( 2, ( #25857, #30351, #26175, #10101, #11373, #21039, #49976, #44506, #40646 ),
 .UNSPECIFIED., .F., .F. ) 
 B_SPLINE_CURVE_WITH_KNOTS ( ( 3, 2, 2, 2, 3 ),
 ( 0.06041666666666666713, 0.06111111111111110911, 0.06250000000000000000, 0.06388888888888888395, 0.06458333333333333981 ),
 .UNSPECIFIED. ) 
 CURVE ( )  GEOMETRIC_REPRESENTATION_ITEM ( )  RATIONAL_B_SPLINE_CURVE ( ( 0.9330127018922194093, 0.9330127018922194093, 1.000000000000000000, 0.8660254037844387076, 1.000000000000000000, 0.8660254037844387076, 1.000000000000000000, 0.9330127018922187432, 0.9330127018922194093 ) ) 
 REPRESENTATION_ITEM ( '' )  );
#24673=CARTESIAN_POINT ( 'NONE',  ( 2.499999999999998668, -80.20833333060213022, -4.330127018922193649 ) ) ;
#24674=CARTESIAN_POINT ( 'NONE',  ( -5.000000000000000000, -48.87499999726880873, 0.000000000000000000 ) ) ;
#24678=CARTESIAN_POINT ( 'NONE',  ( 2.229367062500001939, -26.22916666530106866, 3.861377020970579999 ) ) ;
#24679=ORIENTED_EDGE ( 'NONE', *, *, #45606, .F. ) ;
#24680=CARTESIAN_POINT ( 'NONE',  ( -4.458734124999999437, -165.1875000013655779, -5.460374474430324690E-16 ) ) ;
#24684=AXIS2_PLACEMENT_3D ( 'NONE', #54844, #10775, #30386 ) ;
#24687=CARTESIAN_POINT ( 'NONE',  ( 1.846868145590735200, -144.5000000013656063, -4.458734124999999437 ) ) ;
#24695=CARTESIAN_POINT ( 'NONE',  ( -5.000000000000000888, -167.4375000000000284, 2.071067811865474617 ) ) ;
#24701=CARTESIAN_POINT ( 'NONE',  ( 2.229367062499998831, -72.89583333196773651, -3.861377020970580887 ) ) ;
#24702=CARTESIAN_POINT ( 'NONE',  ( -3.535533905932738641, -144.5000000027311842, 3.535533905932737309 ) ) ;
#24703=DIRECTION ( 'NONE',  ( -0.000000000000000000, 1.000000000000000000, -0.000000000000000000 ) ) ;
#24704=CARTESIAN_POINT ( 'NONE',  ( 5.000000000000000000, 14.62500000273118594, -6.123233995736766282E-16 ) ) ;
#24706=ORIENTED_EDGE ( 'NONE', *, *, #29108, .T. ) ;
#24712=CARTESIAN_POINT ( 'NONE',  ( -4.458734124999999437, 17.43750000136559208, 0.000000000000000000 ) ) ;
#24714=EDGE_CURVE ( 'NONE', #9036, #39802, #41195, .T. ) ;
#24720=CARTESIAN_POINT ( 'NONE',  ( -4.458734124999997661, 1.770833334698928008, 2.574251347313722516 ) ) ;
#24722=CARTESIAN_POINT ( 'NONE',  ( -2.229367062499996610, -25.39583333196773651, 3.861377020970582219 ) ) ;
#24725=CARTESIAN_POINT ( 'NONE',  ( 2.229367062499998831, 27.35416666803225993, -3.861377020970580887 ) ) ;
#24729=CARTESIAN_POINT ( 'NONE',  ( -4.458734124999999437, -72.56249999863439371, 0.000000000000000000 ) ) ;
#24732=CARTESIAN_POINT ( 'NONE',  ( -5.000000000000000000, 28.04166666939785202, -2.886751345948128211 ) ) ;
#24733=ORIENTED_EDGE ( 'NONE', *, *, #53095, .F. ) ;
#24734=FACE_OUTER_BOUND ( 'NONE', #13041, .T. ) ;
#24735=DIRECTION ( 'NONE',  ( -0.000000000000000000, 1.000000000000000000, -0.000000000000000000 ) ) ;
#24736=CARTESIAN_POINT ( 'NONE',  ( -4.999999999999999112, -17.91666666666666430, 2.886751345948131764 ) ) ;
#24737=CARTESIAN_POINT ( 'NONE',  ( 4.458734124999998549, -19.72916666530107221, -2.574251347313721627 ) ) ;
#24739=CARTESIAN_POINT ( 'NONE',  ( -4.458734124999999437, -81.39583333196773651, -2.574251347313719407 ) ) ;
#24740=CARTESIAN_POINT ( 'NONE',  ( -3.152801135295367096, -169.3125000013656063, -3.152801135295367541 ) ) ;
#24741=CARTESIAN_POINT ( 'NONE',  ( -5.000000000000000000, -18.95833333060214443, -2.886751345948128211 ) ) ;
#24742=CARTESIAN_POINT ( 'NONE',  ( -4.458734124999998549, -50.22916666530107221, 2.574251347313722516 ) ) ;
#24745=CARTESIAN_POINT ( 'NONE',  ( -3.152548672688508926E-16, 0.1875000013655953035, -5.148502694627439702 ) ) ;
#24746=EDGE_LOOP ( 'NONE', ( #16479, #24443, #48135, #34235 ) ) ;
#24747=CARTESIAN_POINT ( 'NONE',  ( 2.500000000000002220, -65.66666666666667140, 4.330127018922192761 ) ) ;
#24748=CARTESIAN_POINT ( 'NONE',  ( -1.846868145590737420, -158.0000000013655779, 4.458734124999999437 ) ) ;
#24751=CARTESIAN_POINT ( 'NONE',  ( 5.000000000000000000, -162.0625000000000000, 2.071067811865478614 ) ) ;
#24755=CARTESIAN_POINT ( 'NONE',  ( 4.458734124999998549, -9.979166665301068662, -2.574251347313721627 ) ) ;
#24756=CARTESIAN_POINT ( 'NONE',  ( 9.457646018065525792E-16, -45.31249999863440081, 5.148502694627439702 ) ) ;
#24757=( BOUNDED_CURVE ( )  B_SPLINE_CURVE ( 2, ( #39798, #49775, #50098, #21153, #26286, #46229, #41391, #16643, #1871 ),
 .UNSPECIFIED., .F., .F. ) 
 B_SPLINE_CURVE_WITH_KNOTS ( ( 3, 2, 2, 2, 3 ),
 ( 0.5354166666666666519, 0.5361111111111110938, 0.5374999999999999778, 0.5388888888888888618, 0.5395833333333333037 ),
 .UNSPECIFIED. ) 
 CURVE ( )  GEOMETRIC_REPRESENTATION_ITEM ( )  RATIONAL_B_SPLINE_CURVE ( ( 0.9330127018922194093, 0.9330127018922194093, 1.000000000000000000, 0.8660254037844387076, 1.000000000000000000, 0.8660254037844387076, 1.000000000000000000, 0.9330127018922194093, 0.9330127018922194093 ) ) 
 REPRESENTATION_ITEM ( '' )  );
#24759=DIRECTION ( 'NONE',  ( -0.000000000000000000, 1.000000000000000000, -0.000000000000000000 ) ) ;
#24760=CARTESIAN_POINT ( 'NONE',  ( -1.846868145590734756, -150.1250000013655779, -4.458734125000000326 ) ) ;
#24765=CARTESIAN_POINT ( 'NONE',  ( -2.499999999999996447, -68.70833333060214443, 4.330127018922195425 ) ) ;
#24767=CARTESIAN_POINT ( 'NONE',  ( 1.975475456537005874E-15, -61.74999999999999289, 5.000000000000000000 ) ) ;
#24775=CARTESIAN_POINT ( 'NONE',  ( 4.458734125000001214, -3.895833331967739621, 2.574251347313718519 ) ) ;
#24777=CARTESIAN_POINT ( 'NONE',  ( -4.458734124999999437, -151.0000000013656063, -1.846868145590735644 ) ) ;
#24779=EDGE_LOOP ( 'NONE', ( #62015, #51283, #31288, #62378 ) ) ;
#24781=CARTESIAN_POINT ( 'NONE',  ( -4.999999999999998224, -74.91666666666665719, 2.886751345948131764 ) ) ;
#24783=AXIS2_PLACEMENT_3D ( 'NONE', #50618, #26493, #15889 ) ;
#24784=CARTESIAN_POINT ( 'NONE',  ( 1.339745962155612702, 8.830341803992666883, -5.000000000000000000 ) ) ;
#24790=CARTESIAN_POINT ( 'NONE',  ( 1.339745962155615144, 9.294658198738520838, 4.999999999999999112 ) ) ;
#24791=CARTESIAN_POINT ( 'NONE',  ( 4.458734124999999437, 17.18750000136559564, -5.460374474430324690E-16 ) ) ;
#24795=CARTESIAN_POINT ( 'NONE',  ( -4.458734124999999437, -9.562499998634406140, 0.000000000000000000 ) ) ;
#24796=CARTESIAN_POINT ( 'NONE',  ( 2.071067811865472841, -168.9375000027311842, -5.000000000000002665 ) ) ;
#24798=CARTESIAN_POINT ( 'NONE',  ( -3.152801135295367985, -166.8125000013656063, 3.152801135295367096 ) ) ;
#24803=CARTESIAN_POINT ( 'NONE',  ( 1.975475456537005874E-15, -38.75000000000000000, 5.000000000000000000 ) ) ;
#24805=CARTESIAN_POINT ( 'NONE',  ( 0.000000000000000000, -170.0000000000000000, 5.000000000000000000 ) ) ;
#24806=CARTESIAN_POINT ( 'NONE',  ( 4.458734124999997661, -153.7500000013656063, 1.846868145590737864 ) ) ;
#24810=CARTESIAN_POINT ( 'NONE',  ( 3.535533905932738197, -162.8750000000000284, -3.535533905932738197 ) ) ;
#24811=ORIENTED_EDGE ( 'NONE', *, *, #22011, .T. ) ;
#24814=CARTESIAN_POINT ( 'NONE',  ( -9.184850993605147944E-16, -162.2500000000000000, 5.000000000000000000 ) ) ;
#24815=CARTESIAN_POINT ( 'NONE',  ( -5.000000000000000000, -2.083333333333333037, -2.886751345948128211 ) ) ;
#24816=CARTESIAN_POINT ( 'NONE',  ( -4.458734124999997661, -69.22916666530107932, 2.574251347313722516 ) ) ;
#24817=CARTESIAN_POINT ( 'NONE',  ( 1.975475456537005874E-15, -61.74999999999999289, 5.000000000000000000 ) ) ;
#24818=CARTESIAN_POINT ( 'NONE',  ( -3.535250795749689387E-16, -1.124999997268814056, -5.773502691896257311 ) ) ;
#24819=CARTESIAN_POINT ( 'NONE',  ( 4.458734124999998549, -34.72916666530107221, -2.574251347313721627 ) ) ;
#24820=VERTEX_POINT ( 'NONE', #40882 ) ;
#24821=DIRECTION ( 'NONE',  ( -0.000000000000000000, 1.000000000000000000, -0.000000000000000000 ) ) ;
#24822=DIRECTION ( 'NONE',  ( 0.000000000000000000, 0.000000000000000000, 1.000000000000000000 ) ) ;
#24825=CARTESIAN_POINT ( 'NONE',  ( -4.999999999999999112, -51.91666666666667140, 2.886751345948131764 ) ) ;
#24826=CARTESIAN_POINT ( 'NONE',  ( 2.499999999999998668, -17.20833333060214443, -4.330127018922193649 ) ) ;
#24828=CARTESIAN_POINT ( 'NONE',  ( 2.499999999999998668, -32.20833333060215153, -4.330127018922193649 ) ) ;
#24829=CARTESIAN_POINT ( 'NONE',  ( -2.229367062500000163, -72.47916666530107932, -3.861377020970580443 ) ) ;
#24830=CARTESIAN_POINT ( 'NONE',  ( -3.152801135295367096, -144.3125000013655779, -3.152801135295367541 ) ) ;
#24831=CARTESIAN_POINT ( 'NONE',  ( 4.458734124999999437, -80.81249999863440792, -5.460374474430324690E-16 ) ) ;
#24833=CARTESIAN_POINT ( 'NONE',  ( -4.458734124999998549, -30.47916666530107221, 2.574251347313722516 ) ) ;
#24834=CARTESIAN_POINT ( 'NONE',  ( -5.000000000000000000, -73.95833333060214443, -2.886751345948128211 ) ) ;
#24836=VERTEX_POINT ( 'NONE', #30599 ) ;
#24838=CARTESIAN_POINT ( 'NONE',  ( 1.339745962155612702, -51.29465819873851729, -5.000000000000000000 ) ) ;
#24841=CARTESIAN_POINT ( 'NONE',  ( -2.499999999999996447, 8.291666669397852019, 4.330127018922195425 ) ) ;
#24844=CARTESIAN_POINT ( 'NONE',  ( 1.975475456537005874E-15, 17.25000000000000000, 5.000000000000000000 ) ) ;
#24845=CARTESIAN_POINT ( 'NONE',  ( 2.229367062499998831, -59.89583333196774362, -3.861377020970580887 ) ) ;
#24846=EDGE_CURVE ( 'NONE', #14700, #43870, #43354, .T. ) ;
#24849=EDGE_CURVE ( 'NONE', #2012, #1843, #3564, .T. ) ;
#24850=LINE ( 'NONE', #53791, #27502 ) ;
#24851=CARTESIAN_POINT ( 'NONE',  ( 0.000000000000000000, -170.0000000000000000, 0.000000000000000000 ) ) ;
#24852=ADVANCED_FACE ( 'NONE', ( #62427 ), #37645, .T. ) ;
#24853=CARTESIAN_POINT ( 'NONE',  ( -4.458734124999999437, 12.60416666803225993, -2.574251347313719407 ) ) ;
#24856=CARTESIAN_POINT ( 'NONE',  ( 4.458734124999999437, -165.4375000013655779, 0.000000000000000000 ) ) ;
#24865=CARTESIAN_POINT ( 'NONE',  ( 5.000000000000000000, -40.29166666393548013, -2.886751345948130876 ) ) ;
#24868=LINE ( 'NONE', #45436, #19334 ) ;
#24874=CARTESIAN_POINT ( 'NONE',  ( -4.458734124999999437, 6.437500001365593860, 0.000000000000000000 ) ) ;
#24875=CARTESIAN_POINT ( 'NONE',  ( 5.000000000000000888, -150.9375000000000000, -2.071067811865475505 ) ) ;
#24877=CARTESIAN_POINT ( 'NONE',  ( -3.535533905932738641, -148.5000000027311842, 3.535533905932737309 ) ) ;
#24882=FACE_OUTER_BOUND ( 'NONE', #15018, .T. ) ;
#24885=CARTESIAN_POINT ( 'NONE',  ( -1.846868145590737420, -164.0000000013656063, 4.458734124999997661 ) ) ;
#24886=CARTESIAN_POINT ( 'NONE',  ( -2.229367062499996610, -38.14583333196773651, 3.861377020970582219 ) ) ;
#24890=CARTESIAN_POINT ( 'NONE',  ( -4.458734124999999437, -141.9375000013656063, -5.460374474430324690E-16 ) ) ;
#24891=ORIENTED_EDGE ( 'NONE', *, *, #27618, .T. ) ;
#24892=CARTESIAN_POINT ( 'NONE',  ( 4.458734124999999437, 27.93750000136559208, -5.460374474430324690E-16 ) ) ;
#24894=CARTESIAN_POINT ( 'NONE',  ( -2.229367062499996610, -63.39583333196774362, 3.861377020970582219 ) ) ;
#24897=CARTESIAN_POINT ( 'NONE',  ( -5.000000000000000000, 11.00000000000000000, 0.000000000000000000 ) ) ;
#24898=CARTESIAN_POINT ( 'NONE',  ( -2.229367062499996610, -49.14583333196772941, 3.861377020970582219 ) ) ;
#24899=CARTESIAN_POINT ( 'NONE',  ( -4.458734124999998549, -7.229166665301073103, 2.574251347313722516 ) ) ;
#24900=CARTESIAN_POINT ( 'NONE',  ( -1.339745962155613812, -9.205341801261479162, -5.000000000000000000 ) ) ;
#24903=CARTESIAN_POINT ( 'NONE',  ( -5.000000000000000000, -10.08333333333333393, -2.886751345948128211 ) ) ;
#24907=CARTESIAN_POINT ( 'NONE',  ( -3.152548672688508926E-16, -56.56249999863439371, -5.148502694627439702 ) ) ;
#24908=CARTESIAN_POINT ( 'NONE',  ( 1.846868145590736310, -155.8750000013655779, 4.458734124999999437 ) ) ;
#24909=CARTESIAN_POINT ( 'NONE',  ( 2.499999999999998668, -58.20833333060214443, -4.330127018922193649 ) ) ;
#24911=CARTESIAN_POINT ( 'NONE',  ( -6.972266317189433020E-16, -86.25000000000001421, -5.000000000000000000 ) ) ;
#24912=CARTESIAN_POINT ( 'NONE',  ( -2.229367062500000163, 3.270833334698929118, -3.861377020970580443 ) ) ;
#24914=CARTESIAN_POINT ( 'NONE',  ( 5.000000000000000000, -56.41666666666667140, -2.886751345948130876 ) ) ;
#24916=CARTESIAN_POINT ( 'NONE',  ( -4.458734124999999437, -156.9375000013655779, -5.460374474430324690E-16 ) ) ;
#24918=CARTESIAN_POINT ( 'NONE',  ( 1.339745962155612702, -83.29465819873851729, -5.000000000000000000 ) ) ;
#24920=CARTESIAN_POINT ( 'NONE',  ( 5.000000000000000000, -161.1875000027312126, 2.071067811865478614 ) ) ;
#24921=CARTESIAN_POINT ( 'NONE',  ( -2.229367062500000163, -45.72916666530106511, -3.861377020970580443 ) ) ;
#24922=EDGE_LOOP ( 'NONE', ( #12724, #10456, #48736, #32764 ) ) ;
#24927=CARTESIAN_POINT ( 'NONE',  ( 2.229367062499998831, 28.35416666803225993, -3.861377020970580887 ) ) ;
#24935=( BOUNDED_CURVE ( )  B_SPLINE_CURVE ( 2, ( #30047, #24918, #484, #25234, #44845, #808, #20415, #13989, #23962 ),
 .UNSPECIFIED., .F., .F. ) 
 B_SPLINE_CURVE_WITH_KNOTS ( ( 3, 2, 2, 2, 3 ),
 ( 0.9437499999999999778, 0.9444444444444444198, 0.9458333333333333037, 0.9472222222222221877, 0.9479166666666666297 ),
 .UNSPECIFIED. ) 
 CURVE ( )  GEOMETRIC_REPRESENTATION_ITEM ( )  RATIONAL_B_SPLINE_CURVE ( ( 0.9330127018922194093, 0.9330127018922194093, 1.000000000000000000, 0.8660254037844387076, 1.000000000000000000, 0.8660254037844387076, 1.000000000000000000, 0.9330127018922194093, 0.9330127018922194093 ) ) 
 REPRESENTATION_ITEM ( '' )  );
#24936=CARTESIAN_POINT ( 'NONE',  ( 2.499999999999998668, -33.33333333333332860, -4.330127018922193649 ) ) ;
#24937=EDGE_CURVE ( 'NONE', #4579, #18873, #62729, .T. ) ;
#24942=CARTESIAN_POINT ( 'NONE',  ( 0.000000000000000000, -170.0000000000000000, 0.000000000000000000 ) ) ;
#24945=ORIENTED_EDGE ( 'NONE', *, *, #37160, .T. ) ;
#24946=CARTESIAN_POINT ( 'NONE',  ( 2.499999999999998668, -31.33333333333333215, -4.330127018922193649 ) ) ;
#24948=CARTESIAN_POINT ( 'NONE',  ( -3.535533905932738641, -160.5000000027312126, 3.535533905932737309 ) ) ;
#24952=CARTESIAN_POINT ( 'NONE',  ( -2.499999999999996447, -66.83333333333332860, 4.330127018922195425 ) ) ;
#24954=( BOUNDED_CURVE ( )  B_SPLINE_CURVE ( 2, ( #9744, #20369, #59284, #435, #29682, #20041, #39646, #15215, #54465 ),
 .UNSPECIFIED., .F., .F. ) 
 B_SPLINE_CURVE_WITH_KNOTS ( ( 3, 2, 2, 2, 3 ),
 ( 0.3229166666666666852, 0.3236111111111111271, 0.3250000000000000111, 0.3263888888888888951, 0.3270833333333333370 ),
 .UNSPECIFIED. ) 
 CURVE ( )  GEOMETRIC_REPRESENTATION_ITEM ( )  RATIONAL_B_SPLINE_CURVE ( ( 0.9330127018922194093, 0.9330127018922194093, 1.000000000000000000, 0.8660254037844387076, 1.000000000000000000, 0.8660254037844387076, 1.000000000000000000, 0.9330127018922194093, 0.9330127018922194093 ) ) 
 REPRESENTATION_ITEM ( '' )  );
#24959=CARTESIAN_POINT ( 'NONE',  ( 3.061616997868383141E-16, -141.8750000027312126, -5.000000000000000000 ) ) ;
#24960=CARTESIAN_POINT ( 'NONE',  ( 9.457646018065525792E-16, -20.06249999863440081, 5.148502694627439702 ) ) ;
#24961=CARTESIAN_POINT ( 'NONE',  ( -2.499999999999996447, -79.70833333060213022, 4.330127018922195425 ) ) ;
#24962=CARTESIAN_POINT ( 'NONE',  ( 2.071067811865475505, -155.8125000000000284, -5.000000000000000888 ) ) ;
#24965=CARTESIAN_POINT ( 'NONE',  ( -3.152548672688508926E-16, -47.81249999863440792, -5.148502694627439702 ) ) ;
#24966=CARTESIAN_POINT ( 'NONE',  ( -6.972266317189433020E-16, -50.24999999999999289, -5.000000000000000000 ) ) ;
#24967=CARTESIAN_POINT ( 'NONE',  ( 1.975475456537005874E-15, -11.74999999999999645, 5.000000000000000000 ) ) ;
#24968=CARTESIAN_POINT ( 'NONE',  ( 2.500000000000002220, 28.33333333333333215, 4.330127018922192761 ) ) ;
#24971=CARTESIAN_POINT ( 'NONE',  ( -3.152548672688508926E-16, 7.437500001365594748, -5.148502694627439702 ) ) ;
#24973=CARTESIAN_POINT ( 'NONE',  ( 1.975475456537005874E-15, 12.24999999999999822, 5.000000000000000000 ) ) ;
#24975=CARTESIAN_POINT ( 'NONE',  ( -3.152548672688508926E-16, 19.18750000136559208, -5.148502694627439702 ) ) ;
#24977=CARTESIAN_POINT ( 'NONE',  ( 5.000000000000000000, 7.708333336064517205, -2.886751345948129988 ) ) ;
#24978=VERTEX_POINT ( 'NONE', #32826 ) ;
#24982=CARTESIAN_POINT ( 'NONE',  ( -2.229367062500000163, -37.47916666530107221, -3.861377020970580443 ) ) ;
#24983=CARTESIAN_POINT ( 'NONE',  ( 1.060575238724906964E-15, -40.62499999726880162, 5.773502691896257311 ) ) ;
#24986=CARTESIAN_POINT ( 'NONE',  ( 4.458734124999998549, -11.72916666530107044, -2.574251347313721627 ) ) ;
#24987=CARTESIAN_POINT ( 'NONE',  ( 2.229367062499998831, -11.89583333196774007, -3.861377020970580887 ) ) ;
#24989=CARTESIAN_POINT ( 'NONE',  ( 5.000000000000000000, -82.41666666666665719, -2.886751345948129988 ) ) ;
#24990=CARTESIAN_POINT ( 'NONE',  ( -1.846868145590734756, -168.1250000013656063, -4.458734125000000326 ) ) ;
#24992=CARTESIAN_POINT ( 'NONE',  ( 2.500000000000002220, -80.54166666393547303, 4.330127018922192761 ) ) ;
#24995=CARTESIAN_POINT ( 'NONE',  ( 4.458734124999999437, -26.06249999863440792, -5.460374474430324690E-16 ) ) ;
#24997=ORIENTED_EDGE ( 'NONE', *, *, #27165, .T. ) ;
#24998=CARTESIAN_POINT ( 'NONE',  ( 4.458734124999999437, -164.7500000013656063, 1.846868145590737864 ) ) ;
#25000=VERTEX_POINT ( 'NONE', #52455 ) ;
#25002=CARTESIAN_POINT ( 'NONE',  ( 4.458734124999999437, -74.06249999863440792, -5.460374474430324690E-16 ) ) ;
#25005=CARTESIAN_POINT ( 'NONE',  ( -4.458734125000000326, -146.1250000013655779, 1.846868145590734089 ) ) ;
#25006=( BOUNDED_CURVE ( )  B_SPLINE_CURVE ( 2, ( #48199, #57868, #13789, #62067, #4153, #52718, #37605, #8968, #12846 ),
 .UNSPECIFIED., .F., .F. ) 
 B_SPLINE_CURVE_WITH_KNOTS ( ( 3, 2, 2, 2, 3 ),
 ( 0.3604166666666666630, 0.3611111111111111049, 0.3624999999999999889, 0.3638888888888888729, 0.3645833333333333148 ),
 .UNSPECIFIED. ) 
 CURVE ( )  GEOMETRIC_REPRESENTATION_ITEM ( )  RATIONAL_B_SPLINE_CURVE ( ( 0.9330127018922194093, 0.9330127018922194093, 1.000000000000000000, 0.8660254037844387076, 1.000000000000000000, 0.8660254037844387076, 1.000000000000000000, 0.9330127018922194093, 0.9330127018922194093 ) ) 
 REPRESENTATION_ITEM ( '' )  );
#25009=CARTESIAN_POINT ( 'NONE',  ( -4.999999999999998224, 28.08333333333332860, 2.886751345948131764 ) ) ;
#25012=CARTESIAN_POINT ( 'NONE',  ( -1.846868145590734756, -140.3750000013656063, -4.458734125000000326 ) ) ;
#25017=CARTESIAN_POINT ( 'NONE',  ( -2.229367062500000163, -74.72916666530106511, -3.861377020970580443 ) ) ;
#25018=CARTESIAN_POINT ( 'NONE',  ( -2.071067811865391128, -144.8125000027312410, -5.000000000000086153 ) ) ;
#25022=VERTEX_POINT ( 'NONE', #2615 ) ;
#25023=CARTESIAN_POINT ( 'NONE',  ( 5.000000000000000888, -15.58333333333332860, 2.886751345948126879 ) ) ;
#25028=CARTESIAN_POINT ( 'NONE',  ( -2.229367062500000163, 16.27083333469892779, -3.861377020970580443 ) ) ;
#25030=AXIS2_PLACEMENT_3D ( 'NONE', #48882, #4827, #21860 ) ;
#25035=CARTESIAN_POINT ( 'NONE',  ( -2.229367062499996610, -3.145833331967738733, 3.861377020970582219 ) ) ;
#25036=CARTESIAN_POINT ( 'NONE',  ( -2.229367062499996610, -28.39583333196774007, 3.861377020970582219 ) ) ;
#25037=SHAPE_REPRESENTATION ( 'pulling arm', ( #43054 ), #38957 ) ;
#25040=EDGE_CURVE ( 'NONE', #20951, #24591, #25722, .T. ) ;
#25041=CARTESIAN_POINT ( 'NONE',  ( -4.458734124999998549, 27.77083333469892423, 2.574251347313722516 ) ) ;
#25042=CARTESIAN_POINT ( 'NONE',  ( -6.972266317189433020E-16, 26.87500000273118417, -5.000000000000000000 ) ) ;
#25044=CARTESIAN_POINT ( 'NONE',  ( 2.229367062499998831, -70.89583333196773651, -3.861377020970580887 ) ) ;
#25047=CARTESIAN_POINT ( 'NONE',  ( 1.060575238724906964E-15, 23.37500000273118062, 5.773502691896257311 ) ) ;
#25050=CARTESIAN_POINT ( 'NONE',  ( 3.061616997868383141E-16, -162.8750000027311842, -5.000000000000000000 ) ) ;
#25051=( BOUNDED_CURVE ( )  B_SPLINE_CURVE ( 2, ( #49299, #44782, #53799, #9733, #29337, #19065, #63470, #39316, #13933 ),
 .UNSPECIFIED., .F., .F. ) 
 B_SPLINE_CURVE_WITH_KNOTS ( ( 3, 2, 2, 2, 3 ),
 ( 0.6729166666666667185, 0.6736111111111111605, 0.6750000000000000444, 0.6763888888888889284, 0.6770833333333333703 ),
 .UNSPECIFIED. ) 
 CURVE ( )  GEOMETRIC_REPRESENTATION_ITEM ( )  RATIONAL_B_SPLINE_CURVE ( ( 0.9330127018922194093, 0.9330127018922194093, 1.000000000000000000, 0.8660254037844387076, 1.000000000000000000, 0.8660254037844387076, 1.000000000000000000, 0.9330127018922194093, 0.9330127018922194093 ) ) 
 REPRESENTATION_ITEM ( '' )  );
#25052=CARTESIAN_POINT ( 'NONE',  ( -5.000000000000000000, -16.08333333333333215, -2.886751345948128211 ) ) ;
#25053=CARTESIAN_POINT ( 'NONE',  ( -3.152548672688508926E-16, -23.56249999863440436, -5.148502694627439702 ) ) ;
#25055=CARTESIAN_POINT ( 'NONE',  ( -4.458734124999999437, -82.31249999863440792, 0.000000000000000000 ) ) ;
#25056=CARTESIAN_POINT ( 'NONE',  ( -2.499999999999996447, -23.70833333060214443, 4.330127018922195425 ) ) ;
#25057=CARTESIAN_POINT ( 'NONE',  ( -4.458734124999999437, -51.39583333196772941, -2.574251347313719407 ) ) ;
#25061=CARTESIAN_POINT ( 'NONE',  ( 2.229367062500001939, -0.2291666653010705768, 3.861377020970579999 ) ) ;
#25064=CARTESIAN_POINT ( 'NONE',  ( 2.499999999999998668, -68.33333333333332860, -4.330127018922193649 ) ) ;
#25065=CARTESIAN_POINT ( 'NONE',  ( 1.846868145590736310, -150.8750000013655779, 4.458734124999999437 ) ) ;
#25067=CARTESIAN_POINT ( 'NONE',  ( -2.499999999999996447, -80.70833333060213022, 4.330127018922195425 ) ) ;
#25068=CARTESIAN_POINT ( 'NONE',  ( 5.000000000000000888, -163.9375000000000000, -2.071067811865475505 ) ) ;
#25069=CARTESIAN_POINT ( 'NONE',  ( -5.000000000000000000, 7.125000002731185944, 0.000000000000000000 ) ) ;
#25071=CARTESIAN_POINT ( 'NONE',  ( -4.458734124999998549, -10.47916666530107044, 2.574251347313722516 ) ) ;
#25072=CARTESIAN_POINT ( 'NONE',  ( 4.458734125000001214, -44.14583333196773651, 2.574251347313718519 ) ) ;
#25073=CARTESIAN_POINT ( 'NONE',  ( 5.000000000000000888, -151.0625000027311842, -2.071067811865475505 ) ) ;
#25074=CARTESIAN_POINT ( 'NONE',  ( -1.846868145590737420, -145.7500000013655779, 4.458734124999999437 ) ) ;
#25077=ORIENTED_EDGE ( 'NONE', *, *, #59398, .F. ) ;
#25078=CARTESIAN_POINT ( 'NONE',  ( 6.123233995736766282E-16, -170.0000000000000000, -5.000000000000000000 ) ) ;
#25079=CARTESIAN_POINT ( 'NONE',  ( -2.500000000000000444, -6.041666663935481019, -4.330127018922193649 ) ) ;
#25083=ORIENTED_EDGE ( 'NONE', *, *, #826, .F. ) ;
#25088=CARTESIAN_POINT ( 'NONE',  ( -2.229367062499996610, -5.145833331967740065, 3.861377020970582219 ) ) ;
#25089=CARTESIAN_POINT ( 'NONE',  ( 3.061616997868383141E-16, -145.8750000027312126, -5.000000000000000000 ) ) ;
#25090=CARTESIAN_POINT ( 'NONE',  ( -4.458734125000000326, -147.8750000013655779, 1.846868145590734089 ) ) ;
#25097=CARTESIAN_POINT ( 'NONE',  ( -6.972266317189433020E-16, -25.12499999726881228, -5.000000000000000000 ) ) ;
#25103=CARTESIAN_POINT ( 'NONE',  ( -1.339745962155610925, -89.66965819600733312, 5.000000000000000000 ) ) ;
#25105=CARTESIAN_POINT ( 'NONE',  ( 4.458734125000000326, 20.10416666803225638, 2.574251347313718519 ) ) ;
#25107=ORIENTED_EDGE ( 'NONE', *, *, #36970, .T. ) ;
#25108=CARTESIAN_POINT ( 'NONE',  ( 4.458734124999999437, -11.06249999863440792, -5.460374474430324690E-16 ) ) ;
#25110=CARTESIAN_POINT ( 'NONE',  ( -1.846868145590734756, -164.1250000013656063, -4.458734125000000326 ) ) ;
#25113=EDGE_CURVE ( 'NONE', #18601, #12246, #42987, .T. ) ;
#25117=CARTESIAN_POINT ( 'NONE',  ( -1.339745962155610925, -88.66965819600733312, 5.000000000000000000 ) ) ;
#25118=CARTESIAN_POINT ( 'NONE',  ( 1.846868145590736310, -152.8750000013655779, 4.458734124999997661 ) ) ;
#25125=CARTESIAN_POINT ( 'NONE',  ( 2.500000000000002220, -4.666666666666666075, 4.330127018922192761 ) ) ;
#25126=EDGE_CURVE ( 'NONE', #27450, #23493, #19501, .T. ) ;
#25127=CARTESIAN_POINT ( 'NONE',  ( -4.458734124999997661, -67.22916666530106511, 2.574251347313722516 ) ) ;
#25128=( BOUNDED_CURVE ( )  B_SPLINE_CURVE ( 2, ( #20612, #39885, #49229, #40217, #59853, #15777, #35394, #55016, #10308 ),
 .UNSPECIFIED., .F., .F. ) 
 B_SPLINE_CURVE_WITH_KNOTS ( ( 3, 2, 2, 2, 3 ),
 ( 0.8687500000000000222, 0.8694444444444444642, 0.8708333333333333481, 0.8722222222222222321, 0.8729166666666666741 ),
 .UNSPECIFIED. ) 
 CURVE ( )  GEOMETRIC_REPRESENTATION_ITEM ( )  RATIONAL_B_SPLINE_CURVE ( ( 0.9330127018922194093, 0.9330127018922194093, 1.000000000000000000, 0.8660254037844387076, 1.000000000000000000, 0.8660254037844387076, 1.000000000000000000, 0.9330127018922194093, 0.9330127018922194093 ) ) 
 REPRESENTATION_ITEM ( '' )  );
#25130=CARTESIAN_POINT ( 'NONE',  ( 2.499999999999998668, -4.208333330602147981, -4.330127018922193649 ) ) ;
#25131=CARTESIAN_POINT ( 'NONE',  ( -2.229367062500000163, -36.47916666530107221, -3.861377020970580443 ) ) ;
#25133=CARTESIAN_POINT ( 'NONE',  ( -1.339745962155613812, -78.20534180126146850, -5.000000000000000000 ) ) ;
#25134=CARTESIAN_POINT ( 'NONE',  ( 3.535533905932738197, -156.8750000000000284, -3.535533905932738197 ) ) ;
#25138=CARTESIAN_POINT ( 'NONE',  ( -3.535250795749689387E-16, -49.25000000000000000, -5.773502691896257311 ) ) ;
#25139=CARTESIAN_POINT ( 'NONE',  ( 2.500000000000002220, -17.54166666393547658, 4.330127018922192761 ) ) ;
#25141=CARTESIAN_POINT ( 'NONE',  ( 5.000000000000000000, -32.29166666393548724, -2.886751345948130876 ) ) ;
#25142=CARTESIAN_POINT ( 'NONE',  ( -2.229367062499996610, -73.14583333196773651, 3.861377020970582219 ) ) ;
#25143=CARTESIAN_POINT ( 'NONE',  ( 3.152801135295367541, -144.5625000013655779, -3.152801135295367541 ) ) ;
#25144=CARTESIAN_POINT ( 'NONE',  ( -4.458734124999999437, -81.31249999863440792, 0.000000000000000000 ) ) ;
#25146=CARTESIAN_POINT ( 'NONE',  ( 4.458734124999999437, -29.06249999863440436, -5.460374474430324690E-16 ) ) ;
#25147=CARTESIAN_POINT ( 'NONE',  ( 5.000000000000000000, -73.37499999726880162, -6.123233995736766282E-16 ) ) ;
#25150=EDGE_LOOP ( 'NONE', ( #37320, #47336, #20797, #57902 ) ) ;
#25154=CARTESIAN_POINT ( 'NONE',  ( -1.339745962155610925, 17.20534180126147916, 5.000000000000000000 ) ) ;
#25156=CARTESIAN_POINT ( 'NONE',  ( 4.458734125000001214, -58.14583333196773651, 2.574251347313718519 ) ) ;
#25160=CARTESIAN_POINT ( 'NONE',  ( 0.000000000000000000, -170.0000000000000000, 0.000000000000000000 ) ) ;
#25161=CARTESIAN_POINT ( 'NONE',  ( 2.229367062499998831, 11.35416666803225993, -3.861377020970580887 ) ) ;
#25163=CARTESIAN_POINT ( 'NONE',  ( -5.000000000000000000, -1.083333333333331927, -2.886751345948128211 ) ) ;
#25164=CARTESIAN_POINT ( 'NONE',  ( -8.190561711645485556E-16, -160.6875000013655779, 4.458734124999999437 ) ) ;
#25165=DIRECTION ( 'NONE',  ( 0.000000000000000000, 0.000000000000000000, 1.000000000000000000 ) ) ;
#25166=ORIENTED_EDGE ( 'NONE', *, *, #36910, .T. ) ;
#25168=CARTESIAN_POINT ( 'NONE',  ( 6.123233995736766282E-16, -170.0000000000000000, -5.000000000000000000 ) ) ;
#25170=DIRECTION ( 'NONE',  ( 0.000000000000000000, 0.000000000000000000, 1.000000000000000000 ) ) ;
#25172=CARTESIAN_POINT ( 'NONE',  ( 1.339745962155612702, -36.29465819873852439, -5.000000000000000000 ) ) ;
#25175=CARTESIAN_POINT ( 'NONE',  ( -2.500000000000000444, -21.16666666666666785, -4.330127018922193649 ) ) ;
#25178=( BOUNDED_CURVE ( )  B_SPLINE_CURVE ( 2, ( #9568, #53003, #4129, #43346, #47549, #62990, #18902, #3499, #13463 ),
 .UNSPECIFIED., .F., .F. ) 
 B_SPLINE_CURVE_WITH_KNOTS ( ( 3, 2, 2, 2, 3 ),
 ( 0.09791666666666666574, 0.09861111111111110772, 0.1000000000000000056, 0.1013888888888888895, 0.1020833333333333315 ),
 .UNSPECIFIED. ) 
 CURVE ( )  GEOMETRIC_REPRESENTATION_ITEM ( )  RATIONAL_B_SPLINE_CURVE ( ( 0.9330127018922194093, 0.9330127018922194093, 1.000000000000000000, 0.8660254037844387076, 1.000000000000000000, 0.8660254037844387076, 1.000000000000000000, 0.9330127018922194093, 0.9330127018922194093 ) ) 
 REPRESENTATION_ITEM ( '' )  );
#25182=CARTESIAN_POINT ( 'NONE',  ( 4.458734125000000326, 5.854166668032262599, 2.574251347313718519 ) ) ;
#25183=CARTESIAN_POINT ( 'NONE',  ( 2.071067811865349828, -151.1875000000000000, 5.000000000000126121 ) ) ;
#25185=CARTESIAN_POINT ( 'NONE',  ( 3.061616997868383141E-16, -150.8750000027312126, -5.000000000000000000 ) ) ;
#25186=LINE ( 'NONE', #39332, #23334 ) ;
#25190=CARTESIAN_POINT ( 'NONE',  ( -3.535533905932737309, -140.6250000000000000, -3.535533905932738197 ) ) ;
#25193=EDGE_CURVE ( 'NONE', #5493, #11807, #52404, .T. ) ;
#25195=CARTESIAN_POINT ( 'NONE',  ( -1.846868145590734756, -167.3750000013656347, -4.458734124999999437 ) ) ;
#25197=LINE ( 'NONE', #30659, #38885 ) ;
#25200=CARTESIAN_POINT ( 'NONE',  ( 4.458734124999999437, -142.5000000013656347, 1.846868145590737864 ) ) ;
#25202=CARTESIAN_POINT ( 'NONE',  ( -4.458734124999999437, 27.35416666803225993, -2.574251347313719407 ) ) ;
#25204=CARTESIAN_POINT ( 'NONE',  ( -4.458734124999997661, -63.47916666530106511, 2.574251347313722516 ) ) ;
#25207=CARTESIAN_POINT ( 'NONE',  ( -2.500000000000000444, 11.83333333333333037, -4.330127018922193649 ) ) ;
#25209=CARTESIAN_POINT ( 'NONE',  ( -2.229367062499996610, -51.14583333196772941, 3.861377020970582219 ) ) ;
#25211=CARTESIAN_POINT ( 'NONE',  ( 2.229367062500001939, -9.979166665301068662, 3.861377020970579999 ) ) ;
#25212=DIRECTION ( 'NONE',  ( -0.000000000000000000, 1.000000000000000000, -0.000000000000000000 ) ) ;
#25213=CARTESIAN_POINT ( 'NONE',  ( -1.339745962155613812, -64.08034179853029855, -5.000000000000000000 ) ) ;
#25217=CARTESIAN_POINT ( 'NONE',  ( 1.339745962155612702, -66.16965819600733312, -5.000000000000000000 ) ) ;
#25221=CARTESIAN_POINT ( 'NONE',  ( 9.457646018065525792E-16, -53.06249999863441502, 5.148502694627439702 ) ) ;
#25222=CARTESIAN_POINT ( 'NONE',  ( -1.846868145590734756, -157.3750000013656347, -4.458734125000000326 ) ) ;
#25224=CARTESIAN_POINT ( 'NONE',  ( -2.500000000000000444, -55.04166666393548013, -4.330127018922193649 ) ) ;
#25227=CARTESIAN_POINT ( 'NONE',  ( -4.458734124999999437, 2.354166668032262599, -2.574251347313719407 ) ) ;
#25230=DIRECTION ( 'NONE',  ( 0.000000000000000000, 0.000000000000000000, -1.000000000000000000 ) ) ;
#25231=CARTESIAN_POINT ( 'NONE',  ( -1.846868145590737420, -156.7500000013656063, 4.458734124999999437 ) ) ;
#25232=ORIENTED_EDGE ( 'NONE', *, *, #56679, .F. ) ;
#25234=CARTESIAN_POINT ( 'NONE',  ( 5.000000000000000000, -83.41666666666667140, -2.886751345948130876 ) ) ;
#25236=CARTESIAN_POINT ( 'NONE',  ( 4.458734124999999437, -42.06249999863440081, -5.460374474430324690E-16 ) ) ;
#25240=CARTESIAN_POINT ( 'NONE',  ( -2.229367062500000163, -89.72916666530106511, -3.861377020970580443 ) ) ;
#25242=CARTESIAN_POINT ( 'NONE',  ( -2.071067811865517250, -165.6875000000000000, -4.999999999999958256 ) ) ;
#25248=AXIS2_PLACEMENT_3D ( 'NONE', #36104, #25490, #11012 ) ;
#25249=CARTESIAN_POINT ( 'NONE',  ( -2.500000000000000444, -79.04166666393547303, -4.330127018922193649 ) ) ;
#25252=CARTESIAN_POINT ( 'NONE',  ( -1.339745962155610925, 5.205341801261479162, 5.000000000000000000 ) ) ;
#25253=DIRECTION ( 'NONE',  ( 0.000000000000000000, 0.000000000000000000, 1.000000000000000000 ) ) ;
#25254=CARTESIAN_POINT ( 'NONE',  ( -2.229367062499996610, -88.39583333196773651, 3.861377020970582219 ) ) ;
#25257=ORIENTED_EDGE ( 'NONE', *, *, #12317, .F. ) ;
#25260=CARTESIAN_POINT ( 'NONE',  ( 2.071067811865476394, -162.3125000027312694, 5.000000000000000000 ) ) ;
#25263=CARTESIAN_POINT ( 'NONE',  ( 5.000000000000000888, -49.45833333060213732, 2.886751345948126879 ) ) ;
#25265=CARTESIAN_POINT ( 'NONE',  ( -2.499999999999996447, -71.70833333060214443, 4.330127018922195425 ) ) ;
#25268=EDGE_CURVE ( 'NONE', #31680, #7616, #45815, .T. ) ;
#25273=CARTESIAN_POINT ( 'NONE',  ( -4.458734124999999437, -18.31249999863440792, 0.000000000000000000 ) ) ;
#25275=CARTESIAN_POINT ( 'NONE',  ( 5.000000000000000888, -155.9375000000000000, -2.071067811865475505 ) ) ;
#25277=CARTESIAN_POINT ( 'NONE',  ( -4.458734125000000326, -155.0000000013656063, -1.846868145590735644 ) ) ;
#25279=CARTESIAN_POINT ( 'NONE',  ( 4.458734124999998549, -47.97916666530106511, -2.574251347313721627 ) ) ;
#25280=CARTESIAN_POINT ( 'NONE',  ( 1.975475456537005874E-15, -44.62499999726880162, 5.000000000000000000 ) ) ;
#25282=CARTESIAN_POINT ( 'NONE',  ( -2.499999999999996447, 27.16666666666666430, 4.330127018922195425 ) ) ;
#25283=CARTESIAN_POINT ( 'NONE',  ( 2.229367062499998831, 12.35416666803226171, -3.861377020970580887 ) ) ;
#25287=CARTESIAN_POINT ( 'NONE',  ( 9.457646018065525792E-16, 19.68750000136559208, 5.148502694627439702 ) ) ;
#25289=CARTESIAN_POINT ( 'NONE',  ( 1.060575238724906964E-15, 8.375000002731187720, 5.773502691896257311 ) ) ;
#25290=ADVANCED_FACE ( 'NONE', ( #44927 ), #15657, .T. ) ;
#25291=VERTEX_POINT ( 'NONE', #59731 ) ;
#25295=CARTESIAN_POINT ( 'NONE',  ( 2.229367062500001939, -39.97916666530107221, 3.861377020970579999 ) ) ;
#25297=VECTOR ( 'NONE', #58572, 1000.000000000000000 ) ;
#25298=AXIS2_PLACEMENT_3D ( 'NONE', #45270, #5718, #30143 ) ;
#25299=ADVANCED_FACE ( 'NONE', ( #40409 ), #32287, .T. ) ;
#25300=CARTESIAN_POINT ( 'NONE',  ( -2.500000000000000444, -41.04166666393548013, -4.330127018922193649 ) ) ;
#25301=ORIENTED_EDGE ( 'NONE', *, *, #13438, .T. ) ;
#25302=CARTESIAN_POINT ( 'NONE',  ( -4.458734124999999437, -12.39583333196774184, -2.574251347313719407 ) ) ;
#25303=CARTESIAN_POINT ( 'NONE',  ( 4.458734124999998549, -18.97916666530107221, -2.574251347313721627 ) ) ;
#25305=CARTESIAN_POINT ( 'NONE',  ( -5.000000000000000000, -80.00000000000000000, 0.000000000000000000 ) ) ;
#25306=CARTESIAN_POINT ( 'NONE',  ( -8.190561711645485556E-16, -166.6875000013655779, 4.458734124999999437 ) ) ;
#25308=CARTESIAN_POINT ( 'NONE',  ( -4.999999999999999112, -88.79166666393547303, 2.886751345948131764 ) ) ;
#25310=VERTEX_POINT ( 'NONE', #25969 ) ;
#25312=CARTESIAN_POINT ( 'NONE',  ( -3.152548672688508926E-16, -27.81249999863440436, -5.148502694627439702 ) ) ;
#25316=CARTESIAN_POINT ( 'NONE',  ( 2.730187237215162345E-16, -162.4375000013655779, -4.458734124999999437 ) ) ;
#25318=CARTESIAN_POINT ( 'NONE',  ( -2.499999999999996447, -38.70833333060213732, 4.330127018922195425 ) ) ;
#25321=CARTESIAN_POINT ( 'NONE',  ( -3.152548672688508926E-16, -75.81249999863440792, -5.148502694627439702 ) ) ;
#25324=CARTESIAN_POINT ( 'NONE',  ( -4.458734124999999437, -144.1875000013656063, -5.460374474430324690E-16 ) ) ;
#25325=CARTESIAN_POINT ( 'NONE',  ( -1.127183054612291972E-14, 23.25000000000000000, 4.999999999999999112 ) ) ;
#25330=CARTESIAN_POINT ( 'NONE',  ( -1.846868145590737420, -140.0000000013655779, 4.458734124999999437 ) ) ;
#25335=CARTESIAN_POINT ( 'NONE',  ( 9.457646018065525792E-16, -76.31249999863439371, 5.148502694627439702 ) ) ;
#25336=DIRECTION ( 'NONE',  ( -0.000000000000000000, 1.000000000000000000, -0.000000000000000000 ) ) ;
#25337=CARTESIAN_POINT ( 'NONE',  ( 0.000000000000000000, -170.0000000000000000, 5.000000000000000000 ) ) ;
#25339=VERTEX_POINT ( 'NONE', #20517 ) ;
#25340=DIRECTION ( 'NONE',  ( -0.000000000000000000, 1.000000000000000000, -0.000000000000000000 ) ) ;
#25341=CARTESIAN_POINT ( 'NONE',  ( 5.000000000000000888, 23.54166666939785202, 2.886751345948126879 ) ) ;
#25347=CARTESIAN_POINT ( 'NONE',  ( 2.229367062499998831, 19.10416666803225993, -3.861377020970580887 ) ) ;
#25351=EDGE_CURVE ( 'NONE', #25405, #18740, #58948, .T. ) ;
#25357=CARTESIAN_POINT ( 'NONE',  ( 4.458734125000000326, -1.895833331967737623, 2.574251347313718519 ) ) ;
#25359=CARTESIAN_POINT ( 'NONE',  ( -3.152548672688508926E-16, -30.81249999863440436, -5.148502694627439702 ) ) ;
#25363=CARTESIAN_POINT ( 'NONE',  ( -2.229367062499996610, 26.85416666803225993, 3.861377020970582219 ) ) ;
#25364=CARTESIAN_POINT ( 'NONE',  ( 1.339745962155612258, 26.41965820146970501, 5.000000000000000888 ) ) ;
#25366=CARTESIAN_POINT ( 'NONE',  ( -4.458734124999997661, -78.47916666530106511, 2.574251347313722516 ) ) ;
#25369=CARTESIAN_POINT ( 'NONE',  ( 1.060575238724906964E-15, 25.37500000273118417, 5.773502691896257311 ) ) ;
#25370=ORIENTED_EDGE ( 'NONE', *, *, #9075, .F. ) ;
#25373=CARTESIAN_POINT ( 'NONE',  ( 5.000000000000000000, -20.49999999999999645, -6.123233995736766282E-16 ) ) ;
#25374=CARTESIAN_POINT ( 'NONE',  ( -3.152548672688508926E-16, -21.56249999863440081, -5.148502694627439702 ) ) ;
#25375=CARTESIAN_POINT ( 'NONE',  ( 2.229367062499998831, -82.64583333196773651, -3.861377020970580887 ) ) ;
#25376=CARTESIAN_POINT ( 'NONE',  ( -2.499999999999996447, -22.70833333060214443, 4.330127018922195425 ) ) ;
#25377=CARTESIAN_POINT ( 'NONE',  ( 4.458734124999999437, -49.81249999863440792, -5.460374474430324690E-16 ) ) ;
#25379=CARTESIAN_POINT ( 'NONE',  ( -6.972266317189433020E-16, -70.12499999726880162, -5.000000000000000000 ) ) ;
#25381=CARTESIAN_POINT ( 'NONE',  ( -4.458734124999999437, -2.562499998634407028, 0.000000000000000000 ) ) ;
#25384=CARTESIAN_POINT ( 'NONE',  ( -5.000000000000000000, -67.00000000000000000, 0.000000000000000000 ) ) ;
#25385=CARTESIAN_POINT ( 'NONE',  ( -4.458734125000000326, -151.2500000013656063, -1.846868145590735644 ) ) ;
#25387=( BOUNDED_CURVE ( )  B_SPLINE_CURVE ( 2, ( #53611, #33363, #48466, #58749, #52978, #10181, #14678, #9846, #39122 ),
 .UNSPECIFIED., .F., .F. ) 
 B_SPLINE_CURVE_WITH_KNOTS ( ( 3, 2, 2, 2, 3 ),
 ( 0.2979166666666666630, 0.2986111111111111049, 0.2999999999999999889, 0.3013888888888888729, 0.3020833333333333148 ),
 .UNSPECIFIED. ) 
 CURVE ( )  GEOMETRIC_REPRESENTATION_ITEM ( )  RATIONAL_B_SPLINE_CURVE ( ( 0.9330127018922194093, 0.9330127018922194093, 1.000000000000000000, 0.8660254037844387076, 1.000000000000000000, 0.8660254037844387076, 1.000000000000000000, 0.9330127018922194093, 0.9330127018922194093 ) ) 
 REPRESENTATION_ITEM ( '' )  );
#25388=CARTESIAN_POINT ( 'NONE',  ( -5.000000000000000888, -158.5625000000000000, -2.071067811865475949 ) ) ;
#25389=CARTESIAN_POINT ( 'NONE',  ( -1.339745962155610925, 11.20534180126147739, 5.000000000000000000 ) ) ;
#25391=AXIS2_PLACEMENT_3D ( 'NONE', #2577, #6205, #56614 ) ;
#25392=CARTESIAN_POINT ( 'NONE',  ( 4.458734124999998549, -10.97916666530107044, -2.574251347313721627 ) ) ;
#25394=CARTESIAN_POINT ( 'NONE',  ( 9.457646018065525792E-16, -47.31249999863440792, 5.148502694627439702 ) ) ;
#25396=CARTESIAN_POINT ( 'NONE',  ( 2.730187237215162345E-16, -146.1875000013656063, -4.458734124999999437 ) ) ;
#25400=VERTEX_POINT ( 'NONE', #50421 ) ;
#25403=CARTESIAN_POINT ( 'NONE',  ( -6.972266317189433020E-16, -62.24999999999999289, -5.000000000000000000 ) ) ;
#25405=VERTEX_POINT ( 'NONE', #25654 ) ;
#25409=CARTESIAN_POINT ( 'NONE',  ( 4.458734124999999437, -6.812499998634404363, -5.460374474430324690E-16 ) ) ;
#25411=CARTESIAN_POINT ( 'NONE',  ( 4.458734124999999437, -147.4375000013656063, 0.000000000000000000 ) ) ;
#25414=ORIENTED_EDGE ( 'NONE', *, *, #53478, .F. ) ;
#25415=FACE_OUTER_BOUND ( 'NONE', #31906, .T. ) ;
#25419=CARTESIAN_POINT ( 'NONE',  ( 0.000000000000000000, -170.0000000000000000, 5.000000000000000000 ) ) ;
#25426=CARTESIAN_POINT ( 'NONE',  ( 4.458734124999999437, 11.18750000136559386, -5.460374474430324690E-16 ) ) ;
#25429=CARTESIAN_POINT ( 'NONE',  ( -4.458734124999997661, -16.47916666530107577, 2.574251347313722516 ) ) ;
#25432=CARTESIAN_POINT ( 'NONE',  ( -4.458734125000000326, -165.0000000013655779, -1.846868145590735644 ) ) ;
#25438=CARTESIAN_POINT ( 'NONE',  ( 5.000000000000000000, -69.49999999999998579, -6.123233995736766282E-16 ) ) ;
#25440=CARTESIAN_POINT ( 'NONE',  ( -1.846868145590737420, -150.0000000013656063, 4.458734124999997661 ) ) ;
#25447=DIRECTION ( 'NONE',  ( 0.000000000000000000, 0.000000000000000000, 1.000000000000000000 ) ) ;
#25448=CARTESIAN_POINT ( 'NONE',  ( -4.999999999999999112, -1.916666666666663854, 2.886751345948131764 ) ) ;
#25449=CARTESIAN_POINT ( 'NONE',  ( -4.458734124999999437, -64.31249999863440792, 0.000000000000000000 ) ) ;
#25451=CARTESIAN_POINT ( 'NONE',  ( -2.500000000000000444, -6.041666663935481019, -4.330127018922193649 ) ) ;
#25452=CARTESIAN_POINT ( 'NONE',  ( 4.458734125000001214, -33.89583333196773651, 2.574251347313718519 ) ) ;
#25454=CARTESIAN_POINT ( 'NONE',  ( -1.339745962155610925, -77.79465819873853150, 5.000000000000000000 ) ) ;
#25458=CARTESIAN_POINT ( 'NONE',  ( 5.000000000000000888, -49.58333333333332860, 2.886751345948126879 ) ) ;
#25460=CARTESIAN_POINT ( 'NONE',  ( -2.499999999999996447, -41.70833333060214443, 4.330127018922195425 ) ) ;
#25461=CARTESIAN_POINT ( 'NONE',  ( 4.458734125000001214, -75.89583333196775072, 2.574251347313718519 ) ) ;
#25462=CARTESIAN_POINT ( 'NONE',  ( 5.000000000000000000, -169.0625000000000000, 2.071067811865478614 ) ) ;
#25463=CARTESIAN_POINT ( 'NONE',  ( 2.229367062500001939, -80.97916666530106511, 3.861377020970579999 ) ) ;
#25465=CARTESIAN_POINT ( 'NONE',  ( 4.458734124999998549, -30.97916666530107577, -2.574251347313721627 ) ) ;
#25467=CARTESIAN_POINT ( 'NONE',  ( 1.339745962155615144, -51.70534180126148271, 4.999999999999999112 ) ) ;
#25470=CARTESIAN_POINT ( 'NONE',  ( -2.500000000000000444, 21.95833333606451987, -4.330127018922193649 ) ) ;
#25472=AXIS2_PLACEMENT_3D ( 'NONE', #30393, #40681, #21397 ) ;
#25473=DIRECTION ( 'NONE',  ( 0.000000000000000000, 0.000000000000000000, 1.000000000000000000 ) ) ;
#25474=CARTESIAN_POINT ( 'NONE',  ( -2.229367062500000163, -63.72916666530106511, -3.861377020970580443 ) ) ;
#25475=EDGE_CURVE ( 'NONE', #61933, #30240, #18748, .T. ) ;
#25480=CARTESIAN_POINT ( 'NONE',  ( -6.972266317189433020E-16, -21.12499999726881228, -5.000000000000000000 ) ) ;
#25481=CARTESIAN_POINT ( 'NONE',  ( 9.457646018065525792E-16, 14.93750000136559564, 5.148502694627439702 ) ) ;
#25483=CARTESIAN_POINT ( 'NONE',  ( 1.975475456537005874E-15, -24.74999999999999645, 5.000000000000000000 ) ) ;
#25484=CARTESIAN_POINT ( 'NONE',  ( -4.458734125000000326, -161.8750000013656063, 1.846868145590734089 ) ) ;
#25490=DIRECTION ( 'NONE',  ( -0.000000000000000000, 1.000000000000000000, -0.000000000000000000 ) ) ;
#25491=VECTOR ( 'NONE', #50013, 1000.000000000000000 ) ;
#25492=EDGE_CURVE ( 'NONE', #46232, #28871, #37213, .T. ) ;
#25493=CARTESIAN_POINT ( 'NONE',  ( 5.000000000000000000, 4.708333336064518093, -2.886751345948130876 ) ) ;
#25496=EDGE_CURVE ( 'NONE', #11953, #3491, #20451, .T. ) ;
#25499=CARTESIAN_POINT ( 'NONE',  ( 2.229367062500001939, 29.02083333469892779, 3.861377020970579999 ) ) ;
#25502=CARTESIAN_POINT ( 'NONE',  ( -2.229367062499996610, 1.604166668032262155, 3.861377020970582219 ) ) ;
#25503=CARTESIAN_POINT ( 'NONE',  ( 3.535533905932736864, -146.2500000027311842, 3.535533905932738641 ) ) ;
#25505=CARTESIAN_POINT ( 'NONE',  ( -5.000000000000000888, -145.5625000027311842, 2.071067811865474617 ) ) ;
#25509=EDGE_CURVE ( 'NONE', #11915, #41425, #13864, .T. ) ;
#25512=DIRECTION ( 'NONE',  ( -0.000000000000000000, 1.000000000000000000, -0.000000000000000000 ) ) ;
#25515=CARTESIAN_POINT ( 'NONE',  ( -3.152801135295367985, -166.0625000013656063, 3.152801135295367096 ) ) ;
#25519=CARTESIAN_POINT ( 'NONE',  ( 4.458734124999999437, -141.5000000013655779, 1.846868145590737864 ) ) ;
#25520=VERTEX_POINT ( 'NONE', #2488 ) ;
#25521=CARTESIAN_POINT ( 'NONE',  ( -4.458734124999999437, 22.43750000136559564, 0.000000000000000000 ) ) ;
#25522=VERTEX_POINT ( 'NONE', #21790 ) ;
#25523=CARTESIAN_POINT ( 'NONE',  ( 4.458734124999999437, -64.06249999863440792, -5.460374474430324690E-16 ) ) ;
#25524=AXIS2_PLACEMENT_3D ( 'NONE', #49924, #36413, #6837 ) ;
#25526=CARTESIAN_POINT ( 'NONE',  ( 5.000000000000000000, 2.583333333333333481, -2.886751345948130876 ) ) ;
#25527=CARTESIAN_POINT ( 'NONE',  ( -5.000000000000000000, 14.91666666666666607, -2.886751345948128211 ) ) ;
#25529=CARTESIAN_POINT ( 'NONE',  ( -4.458734124999999437, -48.39583333196772941, -2.574251347313719407 ) ) ;
#25530=CARTESIAN_POINT ( 'NONE',  ( 4.458734124999999437, -10.81249999863440792, -5.460374474430324690E-16 ) ) ;
#25532=EDGE_CURVE ( 'NONE', #54505, #39380, #27031, .T. ) ;
#25533=CARTESIAN_POINT ( 'NONE',  ( -5.000000000000000000, 0.1250000027311869155, 0.000000000000000000 ) ) ;
#25535=CYLINDRICAL_SURFACE ( 'NONE', #38685, 5.000000000000000000 ) ;
#25536=CARTESIAN_POINT ( 'NONE',  ( -6.972266317189433020E-16, -5.249999999999998224, -5.000000000000000000 ) ) ;
#25538=CARTESIAN_POINT ( 'NONE',  ( 1.975475456537005874E-15, -12.62499999726881050, 5.000000000000000000 ) ) ;
#25539=CARTESIAN_POINT ( 'NONE',  ( 2.229367062499998831, -59.64583333196774362, -3.861377020970580887 ) ) ;
#25540=CARTESIAN_POINT ( 'NONE',  ( -8.190561711645485556E-16, -156.9375000013655779, 4.458734124999999437 ) ) ;
#25541=CARTESIAN_POINT ( 'NONE',  ( 5.000000000000000000, -56.29166666393548013, -2.886751345948129988 ) ) ;
#25543=CYLINDRICAL_SURFACE ( 'NONE', #37386, 5.000000000000000000 ) ;
#25544=CARTESIAN_POINT ( 'NONE',  ( -4.458734124999999437, 0.3541666680322609340, -2.574251347313719407 ) ) ;
#25546=CARTESIAN_POINT ( 'NONE',  ( -2.071067811865351604, -157.4375000027312126, 5.000000000000126121 ) ) ;
#25548=CARTESIAN_POINT ( 'NONE',  ( -1.846868145590734756, -158.1250000013656063, -4.458734125000000326 ) ) ;
#25553=CARTESIAN_POINT ( 'NONE',  ( -4.458734124999999437, -47.64583333196775072, -2.574251347313719407 ) ) ;
#25556=EDGE_CURVE ( 'NONE', #17081, #8963, #17897, .T. ) ;
#25557=ADVANCED_FACE ( 'NONE', ( #16636 ), #11491, .T. ) ;
#25558=CARTESIAN_POINT ( 'NONE',  ( 1.339745962155637349, 10.83034180399266333, -4.999999999999985789 ) ) ;
#25560=( BOUNDED_CURVE ( )  B_SPLINE_CURVE ( 2, ( #13842, #53710, #48875, #14465, #18357, #9643, #23186, #23817, #58849 ),
 .UNSPECIFIED., .F., .F. ) 
 B_SPLINE_CURVE_WITH_KNOTS ( ( 3, 2, 2, 2, 3 ),
 ( 0.1770833333333333426, 0.1777777777777777846, 0.1791666666666666685, 0.1805555555555555525, 0.1812499999999999944 ),
 .UNSPECIFIED. ) 
 CURVE ( )  GEOMETRIC_REPRESENTATION_ITEM ( )  RATIONAL_B_SPLINE_CURVE ( ( 0.9330127018922194093, 0.9330127018922194093, 1.000000000000000000, 0.8660254037844387076, 1.000000000000000000, 0.8660254037844387076, 1.000000000000000000, 0.9330127018922194093, 0.9330127018922194093 ) ) 
 REPRESENTATION_ITEM ( '' )  );
#25561=CARTESIAN_POINT ( 'NONE',  ( 4.458734125000001214, 27.10416666803225993, 2.574251347313718519 ) ) ;
#25571=CARTESIAN_POINT ( 'NONE',  ( -2.500000000000000444, 6.833333333333333925, -4.330127018922193649 ) ) ;
#25576=ADVANCED_FACE ( 'NONE', ( #61033 ), #26929, .T. ) ;
#25578=CARTESIAN_POINT ( 'NONE',  ( -2.229367062500000163, -88.72916666530106511, -3.861377020970580443 ) ) ;
#25579=CARTESIAN_POINT ( 'NONE',  ( -5.000000000000000000, 11.12500000273118594, 0.000000000000000000 ) ) ;
#25582=CARTESIAN_POINT ( 'NONE',  ( -9.184850993605147944E-16, -163.3750000027311842, 5.000000000000000000 ) ) ;
#25584=CARTESIAN_POINT ( 'NONE',  ( -2.071067811865475061, -158.8125000027312126, -5.000000000000000888 ) ) ;
#25585=ORIENTED_EDGE ( 'NONE', *, *, #52292, .F. ) ;
#25589=CARTESIAN_POINT ( 'NONE',  ( -5.000000000000000000, -67.08333333333332860, -2.886751345948128211 ) ) ;
#25594=( BOUNDED_CURVE ( )  B_SPLINE_CURVE ( 2, ( #32338, #62255, #33599, #51964, #3712, #52282, #58042, #28139, #3399 ),
 .UNSPECIFIED., .F., .F. ) 
 B_SPLINE_CURVE_WITH_KNOTS ( ( 3, 2, 2, 2, 3 ),
 ( 0.6520833333333333481, 0.6527777777777777901, 0.6541666666666666741, 0.6555555555555555580, 0.6562500000000000000 ),
 .UNSPECIFIED. ) 
 CURVE ( )  GEOMETRIC_REPRESENTATION_ITEM ( )  RATIONAL_B_SPLINE_CURVE ( ( 0.9330127018922194093, 0.9330127018922194093, 1.000000000000000000, 0.8660254037844387076, 1.000000000000000000, 0.8660254037844387076, 1.000000000000000000, 0.9330127018922194093, 0.9330127018922194093 ) ) 
 REPRESENTATION_ITEM ( '' )  );
#25596=CARTESIAN_POINT ( 'NONE',  ( 1.339745962155612702, -48.16965819600734022, -5.000000000000000000 ) ) ;
#25597=CARTESIAN_POINT ( 'NONE',  ( 2.229367062500001939, -17.97916666530106866, 3.861377020970579999 ) ) ;
#25598=CARTESIAN_POINT ( 'NONE',  ( 2.499999999999998668, -75.33333333333332860, -4.330127018922193649 ) ) ;
#25599=CARTESIAN_POINT ( 'NONE',  ( 5.000000000000000888, -151.9375000000000000, -2.071067811865475505 ) ) ;
#25601=CARTESIAN_POINT ( 'NONE',  ( -3.152801135295367985, -155.8125000013656063, 3.152801135295367096 ) ) ;
#25602=EDGE_LOOP ( 'NONE', ( #56757, #24658, #33131, #2936 ) ) ;
#25603=CARTESIAN_POINT ( 'NONE',  ( -4.458734124999999437, -46.56249999863440792, 0.000000000000000000 ) ) ;
#25604=CARTESIAN_POINT ( 'NONE',  ( -1.339745962155613812, 25.79465819873851729, -5.000000000000000000 ) ) ;
#25605=CARTESIAN_POINT ( 'NONE',  ( 0.000000000000000000, -170.0000000000000000, 0.000000000000000000 ) ) ;
#25606=CARTESIAN_POINT ( 'NONE',  ( 2.500000000000002220, 29.33333333333333215, 4.330127018922192761 ) ) ;
#25607=CARTESIAN_POINT ( 'NONE',  ( 4.458734125000001214, 3.104166668032260379, 2.574251347313718519 ) ) ;
#25609=LINE ( 'NONE', #26566, #43012 ) ;
#25611=CARTESIAN_POINT ( 'NONE',  ( 4.458734124999999437, 20.93750000136559208, -5.460374474430324690E-16 ) ) ;
#25613=CARTESIAN_POINT ( 'NONE',  ( 5.000000000000000000, 9.708333336064519870, -2.886751345948129988 ) ) ;
#25617=AXIS2_PLACEMENT_3D ( 'NONE', #47083, #42247, #28085 ) ;
#25619=CYLINDRICAL_SURFACE ( 'NONE', #15240, 5.000000000000000000 ) ;
#25620=CARTESIAN_POINT ( 'NONE',  ( -3.152548672688508926E-16, -41.56249999863439371, -5.148502694627439702 ) ) ;
#25622=CARTESIAN_POINT ( 'NONE',  ( 2.500000000000002220, -39.54166666393548013, 4.330127018922192761 ) ) ;
#25624=CARTESIAN_POINT ( 'NONE',  ( 4.458734124999998549, -16.72916666530107577, -2.574251347313721627 ) ) ;
#25625=VERTEX_POINT ( 'NONE', #21469 ) ;
#25626=CARTESIAN_POINT ( 'NONE',  ( 5.000000000000000888, -83.58333333333332860, 2.886751345948126879 ) ) ;
#25627=CARTESIAN_POINT ( 'NONE',  ( 3.152801135295367541, -169.3125000013656063, -3.152801135295367541 ) ) ;
#25628=CARTESIAN_POINT ( 'NONE',  ( 5.000000000000000000, -85.37499999726880162, -6.123233995736766282E-16 ) ) ;
#25629=CARTESIAN_POINT ( 'NONE',  ( -2.500000000000000444, -35.04166666393547303, -4.330127018922193649 ) ) ;
#25632=CARTESIAN_POINT ( 'NONE',  ( 4.458734124999999437, -28.06249999863440081, -5.460374474430324690E-16 ) ) ;
#25633=VERTEX_POINT ( 'NONE', #36259 ) ;
#25636=CARTESIAN_POINT ( 'NONE',  ( -3.152801135295367096, -164.3125000013656063, -3.152801135295367541 ) ) ;
#25638=CARTESIAN_POINT ( 'NONE',  ( -2.500000000000000444, -39.04166666393548013, -4.330127018922193649 ) ) ;
#25640=CARTESIAN_POINT ( 'NONE',  ( -2.499999999999996447, -25.83333333333333215, 4.330127018922195425 ) ) ;
#25642=CARTESIAN_POINT ( 'NONE',  ( 9.457646018065525792E-16, -76.31249999863439371, 5.148502694627439702 ) ) ;
#25645=CARTESIAN_POINT ( 'NONE',  ( -4.458734125000000326, -142.1250000013656063, 1.846868145590734089 ) ) ;
#25649=DIRECTION ( 'NONE',  ( -0.000000000000000000, 1.000000000000000000, -0.000000000000000000 ) ) ;
#25654=CARTESIAN_POINT ( 'NONE',  ( 3.061616997868383141E-16, -167.7500000000000000, -5.000000000000000000 ) ) ;
#25657=CARTESIAN_POINT ( 'NONE',  ( -6.972266317189433020E-16, -53.24999999999999289, -5.000000000000000000 ) ) ;
#25659=CARTESIAN_POINT ( 'NONE',  ( 2.229367062500001939, -75.22916666530106511, 3.861377020970579999 ) ) ;
#25661=CARTESIAN_POINT ( 'NONE',  ( -2.071067811865435981, -166.3124999999999716, 5.000000000000041744 ) ) ;
#25662=DIRECTION ( 'NONE',  ( -0.8660254037844313801, 0.5000000000000125455, -0.000000000000000000 ) ) ;
#25667=EDGE_CURVE ( 'NONE', #7439, #12840, #58079, .T. ) ;
#25668=CARTESIAN_POINT ( 'NONE',  ( 2.499999999999998668, 23.79166666939785202, -4.330127018922193649 ) ) ;
#25674=CARTESIAN_POINT ( 'NONE',  ( 9.457646018065525792E-16, 19.68750000136559208, 5.148502694627439702 ) ) ;
#25677=EDGE_CURVE ( 'NONE', #40725, #25930, #27862, .T. ) ;
#25682=CARTESIAN_POINT ( 'NONE',  ( -4.458734124999998549, -85.22916666530107932, 2.574251347313722516 ) ) ;
#25683=CARTESIAN_POINT ( 'NONE',  ( 4.458734125000000326, -4.895833331967740065, 2.574251347313718519 ) ) ;
#25685=CARTESIAN_POINT ( 'NONE',  ( -3.152548672688508926E-16, -27.81249999863440436, -5.148502694627439702 ) ) ;
#25689=CARTESIAN_POINT ( 'NONE',  ( -2.229367062499996610, 20.85416666803226349, 3.861377020970582219 ) ) ;
#25690=CARTESIAN_POINT ( 'NONE',  ( -6.972266317189433020E-16, -28.25000000000000000, -5.000000000000000000 ) ) ;
#25691=CARTESIAN_POINT ( 'NONE',  ( 2.229367062500001939, -76.22916666530106511, 3.861377020970579999 ) ) ;
#25694=CARTESIAN_POINT ( 'NONE',  ( -2.500000000000000444, 25.95833333606451632, -4.330127018922193649 ) ) ;
#25695=ORIENTED_EDGE ( 'NONE', *, *, #13801, .F. ) ;
#25696=LINE ( 'NONE', #16038, #8861 ) ;
#25698=CARTESIAN_POINT ( 'NONE',  ( -9.184850993605147944E-16, -149.2500000000000284, 5.000000000000000000 ) ) ;
#25699=CARTESIAN_POINT ( 'NONE',  ( -5.000000000000000000, -18.08333333333333570, -2.886751345948128211 ) ) ;
#25700=CARTESIAN_POINT ( 'NONE',  ( 4.458734124999998549, -23.72916666530107221, -2.574251347313721627 ) ) ;
#25701=CARTESIAN_POINT ( 'NONE',  ( 4.458734124999998549, -85.72916666530107932, -2.574251347313721627 ) ) ;
#25703=CARTESIAN_POINT ( 'NONE',  ( -2.500000000000000444, -21.04166666393548013, -4.330127018922193649 ) ) ;
#25704=CARTESIAN_POINT ( 'NONE',  ( -2.229367062499996610, -53.14583333196773651, 3.861377020970582219 ) ) ;
#25706=CARTESIAN_POINT ( 'NONE',  ( 5.000000000000000000, -65.41666666666667140, -2.886751345948130876 ) ) ;
#25707=DIRECTION ( 'NONE',  ( -0.000000000000000000, 1.000000000000000000, -0.000000000000000000 ) ) ;
#25708=CARTESIAN_POINT ( 'NONE',  ( 4.458734125000001214, -2.145833331967737845, 2.574251347313718519 ) ) ;
#25711=CARTESIAN_POINT ( 'NONE',  ( 5.000000000000000000, -67.50000000000000000, -6.123233995736766282E-16 ) ) ;
#25712=CARTESIAN_POINT ( 'NONE',  ( -1.846868145590734756, -151.3750000013656063, -4.458734125000000326 ) ) ;
#25713=AXIS2_PLACEMENT_3D ( 'NONE', #58335, #38089, #13640 ) ;
#25715=CARTESIAN_POINT ( 'NONE',  ( -2.499999999999996447, -76.70833333060214443, 4.330127018922195425 ) ) ;
#25716=CARTESIAN_POINT ( 'NONE',  ( -2.071067811865478170, -158.3125000000000284, 5.000000000000000000 ) ) ;
#25720=CARTESIAN_POINT ( 'NONE',  ( -2.229367062499996610, -13.39583333196774007, 3.861377020970582219 ) ) ;
#25721=CARTESIAN_POINT ( 'NONE',  ( 4.458734124999999437, -52.06249999863440792, -5.460374474430324690E-16 ) ) ;
#25722=( BOUNDED_CURVE ( )  B_SPLINE_CURVE ( 2, ( #2940, #56339, #22233, #61477, #8076, #17411, #46992, #3258, #37026 ),
 .UNSPECIFIED., .F., .F. ) 
 B_SPLINE_CURVE_WITH_KNOTS ( ( 3, 2, 2, 2, 3 ),
 ( 0.6083333333333329485, 0.6124999999999997113, 0.6166666666666663632, 0.6208333333333330151, 0.6249999999999996669 ),
 .UNSPECIFIED. ) 
 CURVE ( )  GEOMETRIC_REPRESENTATION_ITEM ( )  RATIONAL_B_SPLINE_CURVE ( ( 1.000000000000005995, 0.9238795325112806323, 1.000000000000000000, 0.9238795325112867385, 1.000000000000000000, 0.9238795325112867385, 1.000000000000000000, 0.9238795325112928447, 0.9999999999999938938 ) ) 
 REPRESENTATION_ITEM ( '' )  );
#25723=CARTESIAN_POINT ( 'NONE',  ( 4.458734124999999437, -144.5000000013656063, 1.846868145590737864 ) ) ;
#25725=CARTESIAN_POINT ( 'NONE',  ( -1.339745962155601378, 20.91965820146970501, -5.000000000000007105 ) ) ;
#25728=CARTESIAN_POINT ( 'NONE',  ( 4.458734124999998549, 26.02083333469892779, -2.574251347313721627 ) ) ;
#25730=CYLINDRICAL_SURFACE ( 'NONE', #25030, 5.000000000000000000 ) ;
#25736=CARTESIAN_POINT ( 'NONE',  ( 4.458734124999999437, -5.812499998634403475, -5.460374474430324690E-16 ) ) ;
#25738=CARTESIAN_POINT ( 'NONE',  ( -1.846868145590734756, -149.1250000013656063, -4.458734124999999437 ) ) ;
#25740=VERTEX_POINT ( 'NONE', #9191 ) ;
#25741=CARTESIAN_POINT ( 'NONE',  ( -2.500000000000000444, -27.04166666393548013, -4.330127018922193649 ) ) ;
#25744=CARTESIAN_POINT ( 'NONE',  ( 1.339745962155612702, 1.830341803992665772, -5.000000000000000000 ) ) ;
#25746=EDGE_CURVE ( 'NONE', #18873, #12181, #3189, .T. ) ;
#25748=CYLINDRICAL_SURFACE ( 'NONE', #50780, 5.000000000000000000 ) ;
#25751=CARTESIAN_POINT ( 'NONE',  ( 5.000000000000000888, 9.416666666666666075, 2.886751345948126879 ) ) ;
#25752=CARTESIAN_POINT ( 'NONE',  ( 2.229367062500001939, 10.02083333469892779, 3.861377020970579999 ) ) ;
#25755=VECTOR ( 'NONE', #63251, 1000.000000000000000 ) ;
#25756=CARTESIAN_POINT ( 'NONE',  ( 9.457646018065525792E-16, -14.31249999863440614, 5.148502694627439702 ) ) ;
#25758=CARTESIAN_POINT ( 'NONE',  ( 1.846868145590735200, -165.2500000013655779, -4.458734125000000326 ) ) ;
#25765=DIRECTION ( 'NONE',  ( 0.8660254037844385966, 0.5000000000000001110, 0.000000000000000000 ) ) ;
#25766=CARTESIAN_POINT ( 'NONE',  ( 6.123233995736766282E-16, -170.0000000000000000, -5.000000000000000000 ) ) ;
#25768=CARTESIAN_POINT ( 'NONE',  ( 1.846868145590736310, -149.8750000013655779, 4.458734124999997661 ) ) ;
#25770=CARTESIAN_POINT ( 'NONE',  ( -2.500000000000000444, -14.16666666666666785, -4.330127018922193649 ) ) ;
#25771=CARTESIAN_POINT ( 'NONE',  ( -9.184850993605147944E-16, -156.3750000027311842, 5.000000000000000000 ) ) ;
#25777=CARTESIAN_POINT ( 'NONE',  ( -2.499999999999996447, -3.833333333333334370, 4.330127018922195425 ) ) ;
#25778=CARTESIAN_POINT ( 'NONE',  ( 9.457646018065525792E-16, -67.06249999863440792, 5.148502694627439702 ) ) ;
#25779=CARTESIAN_POINT ( 'NONE',  ( 5.000000000000000000, -22.29166666393548013, -2.886751345948130876 ) ) ;
#25780=CARTESIAN_POINT ( 'NONE',  ( 2.500000000000002220, -9.541666663935483683, 4.330127018922192761 ) ) ;
#25781=CARTESIAN_POINT ( 'NONE',  ( -2.229367062500000163, -33.47916666530107221, -3.861377020970580443 ) ) ;
#25782=ORIENTED_EDGE ( 'NONE', *, *, #33982, .T. ) ;
#25783=CARTESIAN_POINT ( 'NONE',  ( -4.999999999999998224, -77.91666666666665719, 2.886751345948131764 ) ) ;
#25784=CYLINDRICAL_SURFACE ( 'NONE', #54922, 5.000000000000000000 ) ;
#25785=CARTESIAN_POINT ( 'NONE',  ( -2.229367062499996610, 11.60416666803225993, 3.861377020970582219 ) ) ;
#25786=VERTEX_POINT ( 'NONE', #57779 ) ;
#25788=CARTESIAN_POINT ( 'NONE',  ( 1.060575238724906964E-15, -52.75000000000000000, 5.773502691896257311 ) ) ;
#25791=CARTESIAN_POINT ( 'NONE',  ( -4.458734124999999437, -73.31249999863439371, 0.000000000000000000 ) ) ;
#25792=CARTESIAN_POINT ( 'NONE',  ( 4.458734124999999437, -139.7500000013655779, 1.846868145590737864 ) ) ;
#25793=CARTESIAN_POINT ( 'NONE',  ( 2.229367062500001939, -83.97916666530106511, 3.861377020970579999 ) ) ;
#25795=CARTESIAN_POINT ( 'NONE',  ( -2.229367062499996610, -37.39583333196773651, 3.861377020970582219 ) ) ;
#25796=ORIENTED_EDGE ( 'NONE', *, *, #62983, .T. ) ;
#25798=EDGE_LOOP ( 'NONE', ( #17774, #46669, #26954, #40837 ) ) ;
#25800=EDGE_LOOP ( 'NONE', ( #29951, #37130, #18876, #56641 ) ) ;
#25804=CARTESIAN_POINT ( 'NONE',  ( -4.458734124999999437, -62.64583333196774362, -2.574251347313719407 ) ) ;
#25807=CARTESIAN_POINT ( 'NONE',  ( -6.972266317189433020E-16, 4.875000002731184168, -5.000000000000000000 ) ) ;
#25808=CARTESIAN_POINT ( 'NONE',  ( -2.498395430326213474E-14, 16.24999999999999645, 5.000000000000000000 ) ) ;
#25809=CARTESIAN_POINT ( 'NONE',  ( 4.458734124999998549, 8.270833334698926009, -2.574251347313721627 ) ) ;
#25811=CARTESIAN_POINT ( 'NONE',  ( -6.972266317189433020E-16, -1.250000000000000000, -5.000000000000000000 ) ) ;
#25812=CARTESIAN_POINT ( 'NONE',  ( 1.846868145590736310, -159.6250000013655779, 4.458734124999997661 ) ) ;
#25813=CARTESIAN_POINT ( 'NONE',  ( 6.123233995736766282E-16, -170.0000000000000000, -5.000000000000000000 ) ) ;
#25818=CARTESIAN_POINT ( 'NONE',  ( 5.000000000000000888, -71.45833333060214443, 2.886751345948126879 ) ) ;
#25822=CARTESIAN_POINT ( 'NONE',  ( -5.000000000000000000, -20.99999999999999645, 0.000000000000000000 ) ) ;
#25823=CARTESIAN_POINT ( 'NONE',  ( 5.000000000000000000, -78.29166666393547303, -2.886751345948130876 ) ) ;
#25824=CARTESIAN_POINT ( 'NONE',  ( -2.229367062499996610, 26.85416666803225993, 3.861377020970582219 ) ) ;
#25827=CARTESIAN_POINT ( 'NONE',  ( 2.229367062500001939, 3.770833334698926009, 3.861377020970579999 ) ) ;
#25829=CARTESIAN_POINT ( 'NONE',  ( -3.535533905932738641, -144.5000000027311842, 3.535533905932737309 ) ) ;
#25834=FACE_OUTER_BOUND ( 'NONE', #15499, .T. ) ;
#25835=CARTESIAN_POINT ( 'NONE',  ( 5.000000000000000000, 3.499999999999999556, -6.123233995736766282E-16 ) ) ;
#25837=CARTESIAN_POINT ( 'NONE',  ( 3.152801135295366208, -161.8125000013656063, 3.152801135295367985 ) ) ;
#25838=CARTESIAN_POINT ( 'NONE',  ( 2.500000000000002220, 7.333333333333333925, 4.330127018922192761 ) ) ;
#25841=VERTEX_POINT ( 'NONE', #57474 ) ;
#25842=CARTESIAN_POINT ( 'NONE',  ( 4.458734124999998549, 24.02083333469892423, -2.574251347313721627 ) ) ;
#25843=ORIENTED_EDGE ( 'NONE', *, *, #24937, .F. ) ;
#25844=CARTESIAN_POINT ( 'NONE',  ( 2.229367062499998831, -64.89583333196773651, -3.861377020970580887 ) ) ;
#25846=CARTESIAN_POINT ( 'NONE',  ( 2.500000000000002220, 2.333333333333333037, 4.330127018922192761 ) ) ;
#25847=CARTESIAN_POINT ( 'NONE',  ( 5.000000000000000888, 14.41666666666666785, 2.886751345948126879 ) ) ;
#25849=CARTESIAN_POINT ( 'NONE',  ( 4.458734124999999437, -51.81249999863440792, -5.460374474430324690E-16 ) ) ;
#25850=CARTESIAN_POINT ( 'NONE',  ( 4.458734125000001214, -9.895833331967736513, 2.574251347313718519 ) ) ;
#25852=DIRECTION ( 'NONE',  ( 0.000000000000000000, 0.000000000000000000, 1.000000000000000000 ) ) ;
#25853=CARTESIAN_POINT ( 'NONE',  ( -1.339745962155610925, -63.79465819873851729, 5.000000000000000000 ) ) ;
#25854=CARTESIAN_POINT ( 'NONE',  ( 0.000000000000000000, -170.0000000000000000, 5.000000000000000000 ) ) ;
#25855=CARTESIAN_POINT ( 'NONE',  ( -2.500000000000000444, -32.16666666666666430, -4.330127018922193649 ) ) ;
#25856=CARTESIAN_POINT ( 'NONE',  ( 1.339745962155615144, -66.58034179853028434, 4.999999999999999112 ) ) ;
#25857=CARTESIAN_POINT ( 'NONE',  ( -6.972266317189433020E-16, 21.87500000273118417, -5.000000000000000000 ) ) ;
#25860=CARTESIAN_POINT ( 'NONE',  ( 9.457646018065525792E-16, -58.06249999863440081, 5.148502694627439702 ) ) ;
#25861=CARTESIAN_POINT ( 'NONE',  ( -3.152801135295367985, -150.0625000013655779, 3.152801135295367096 ) ) ;
#25862=CARTESIAN_POINT ( 'NONE',  ( -2.229367062500000163, -64.47916666530106511, -3.861377020970580443 ) ) ;
#25864=CARTESIAN_POINT ( 'NONE',  ( -2.499999999999996447, -54.70833333060213732, 4.330127018922195425 ) ) ;
#25865=ORIENTED_EDGE ( 'NONE', *, *, #49593, .F. ) ;
#25867=CARTESIAN_POINT ( 'NONE',  ( -3.152548672688508926E-16, -1.812499998634406362, -5.148502694627439702 ) ) ;
#25868=VERTEX_POINT ( 'NONE', #32695 ) ;
#25870=DIRECTION ( 'NONE',  ( -0.000000000000000000, 1.000000000000000000, -0.000000000000000000 ) ) ;
#25871=CARTESIAN_POINT ( 'NONE',  ( 4.458734125000000326, -158.3750000013655779, -1.846868145590734978 ) ) ;
#25872=ORIENTED_EDGE ( 'NONE', *, *, #55147, .T. ) ;
#25873=FACE_OUTER_BOUND ( 'NONE', #61043, .T. ) ;
#25876=CARTESIAN_POINT ( 'NONE',  ( 4.458734125000001214, -46.14583333196773651, 2.574251347313718519 ) ) ;
#25877=ORIENTED_EDGE ( 'NONE', *, *, #22246, .F. ) ;
#25878=CARTESIAN_POINT ( 'NONE',  ( -2.500000000000000444, 16.95833333606451987, -4.330127018922193649 ) ) ;
#25880=CARTESIAN_POINT ( 'NONE',  ( 2.229367062499998831, 25.35416666803225993, -3.861377020970580887 ) ) ;
#25882=DIRECTION ( 'NONE',  ( -0.000000000000000000, 1.000000000000000000, -0.000000000000000000 ) ) ;
#25883=CARTESIAN_POINT ( 'NONE',  ( -1.339745962155613812, -36.08034179853029144, -5.000000000000000000 ) ) ;
#25886=CARTESIAN_POINT ( 'NONE',  ( 5.000000000000000000, -28.37499999726881228, -6.123233995736766282E-16 ) ) ;
#25892=CYLINDRICAL_SURFACE ( 'NONE', #28371, 5.000000000000000000 ) ;
#25893=DIRECTION ( 'NONE',  ( -0.000000000000000000, 1.000000000000000000, -0.000000000000000000 ) ) ;
#25897=VERTEX_POINT ( 'NONE', #37519 ) ;
#25900=CARTESIAN_POINT ( 'NONE',  ( 5.000000000000000000, -156.1250000027311842, 0.000000000000000000 ) ) ;
#25910=CARTESIAN_POINT ( 'NONE',  ( 4.458734125000000326, -19.89583333196774007, 2.574251347313718519 ) ) ;
#25911=CARTESIAN_POINT ( 'NONE',  ( 1.975475456537005874E-15, -79.62499999726881583, 5.000000000000000000 ) ) ;
#25912=CARTESIAN_POINT ( 'NONE',  ( 2.071067811865475505, -152.8125000000000284, -5.000000000000000888 ) ) ;
#25914=CARTESIAN_POINT ( 'NONE',  ( 2.730187237215162345E-16, -150.1875000013656063, -4.458734124999999437 ) ) ;
#25915=ORIENTED_EDGE ( 'NONE', *, *, #25532, .F. ) ;
#25916=CARTESIAN_POINT ( 'NONE',  ( -4.458734124999999437, -48.64583333196773651, -2.574251347313719407 ) ) ;
#25917=DIRECTION ( 'NONE',  ( -0.000000000000000000, 1.000000000000000000, -0.000000000000000000 ) ) ;
#25919=CARTESIAN_POINT ( 'NONE',  ( 5.000000000000000000, 27.58333333333332860, -2.886751345948129988 ) ) ;
#25920=EDGE_CURVE ( 'NONE', #51356, #53696, #62294, .T. ) ;
#25921=CARTESIAN_POINT ( 'NONE',  ( 4.458734125000001214, 2.104166668032262599, 2.574251347313718519 ) ) ;
#25922=CARTESIAN_POINT ( 'NONE',  ( -5.000000000000000000, -73.87499999726880162, 0.000000000000000000 ) ) ;
#25923=CARTESIAN_POINT ( 'NONE',  ( 5.000000000000000000, -41.37499999726880162, -6.123233995736766282E-16 ) ) ;
#25925=CARTESIAN_POINT ( 'NONE',  ( -4.458734124999999437, 13.43750000136559386, 0.000000000000000000 ) ) ;
#25927=CARTESIAN_POINT ( 'NONE',  ( 1.060575238724906964E-15, 10.37500000273118594, 5.773502691896257311 ) ) ;
#25929=CARTESIAN_POINT ( 'NONE',  ( -5.000000000000000000, 8.000000000000000000, 0.000000000000000000 ) ) ;
#25930=VERTEX_POINT ( 'NONE', #23370 ) ;
#25932=CARTESIAN_POINT ( 'NONE',  ( 4.458734125000001214, -43.89583333196775072, 2.574251347313718519 ) ) ;
#25933=CARTESIAN_POINT ( 'NONE',  ( -8.190561711645485556E-16, -165.9375000013655779, 4.458734124999999437 ) ) ;
#25935=CARTESIAN_POINT ( 'NONE',  ( -5.000000000000000000, -41.87499999726880873, 0.000000000000000000 ) ) ;
#25937=CARTESIAN_POINT ( 'NONE',  ( 4.458734124999998549, -17.72916666530106866, -2.574251347313721627 ) ) ;
#25938=EDGE_CURVE ( 'NONE', #22889, #61790, #17999, .T. ) ;
#25940=( BOUNDED_CURVE ( )  B_SPLINE_CURVE ( 2, ( #18742, #14541, #24841, #28395, #43183, #38366, #28706, #33545, #48638 ),
 .UNSPECIFIED., .F., .F. ) 
 B_SPLINE_CURVE_WITH_KNOTS ( ( 3, 2, 2, 2, 3 ),
 ( 0.1729166666666666630, 0.1736111111111111049, 0.1749999999999999889, 0.1763888888888889006, 0.1770833333333333426 ),
 .UNSPECIFIED. ) 
 CURVE ( )  GEOMETRIC_REPRESENTATION_ITEM ( )  RATIONAL_B_SPLINE_CURVE ( ( 0.9330127018922194093, 0.9330127018922194093, 1.000000000000000000, 0.8660254037844387076, 1.000000000000000000, 0.8660254037844387076, 1.000000000000000000, 0.9330127018922194093, 0.9330127018922194093 ) ) 
 REPRESENTATION_ITEM ( '' )  );
#25942=CARTESIAN_POINT ( 'NONE',  ( -3.152801135295367096, -168.0625000013656063, -3.152801135295367541 ) ) ;
#25943=EDGE_CURVE ( 'NONE', #39802, #13190, #24578, .T. ) ;
#25945=CARTESIAN_POINT ( 'NONE',  ( -5.000000000000000000, -86.87499999726880162, 0.000000000000000000 ) ) ;
#25946=CARTESIAN_POINT ( 'NONE',  ( -1.339745962155610925, -18.79465819873852084, 5.000000000000000000 ) ) ;
#25949=CARTESIAN_POINT ( 'NONE',  ( -2.229367062500000163, -34.72916666530107221, -3.861377020970580443 ) ) ;
#25950=CARTESIAN_POINT ( 'NONE',  ( 2.499999999999998668, -29.33333333333332860, -4.330127018922193649 ) ) ;
#25951=VERTEX_POINT ( 'NONE', #58709 ) ;
#25956=ORIENTED_EDGE ( 'NONE', *, *, #46056, .F. ) ;
#25958=CARTESIAN_POINT ( 'NONE',  ( -2.229367062500000163, -75.72916666530106511, -3.861377020970580443 ) ) ;
#25961=CARTESIAN_POINT ( 'NONE',  ( 2.730187237215162345E-16, -140.4375000013656063, -4.458734124999999437 ) ) ;
#25962=CARTESIAN_POINT ( 'NONE',  ( 5.000000000000000000, -84.37499999726880162, -6.123233995736766282E-16 ) ) ;
#25964=CARTESIAN_POINT ( 'NONE',  ( 4.458734125000000326, -42.89583333196773651, 2.574251347313718519 ) ) ;
#25969=CARTESIAN_POINT ( 'NONE',  ( 1.975475456537005874E-15, -66.62499999726881583, 5.000000000000000000 ) ) ;
#25975=CARTESIAN_POINT ( 'NONE',  ( -3.152548672688508926E-16, -72.81249999863439371, -5.148502694627439702 ) ) ;
#25977=CARTESIAN_POINT ( 'NONE',  ( 5.000000000000000000, -68.49999999999998579, -6.123233995736766282E-16 ) ) ;
#25981=CARTESIAN_POINT ( 'NONE',  ( 5.000000000000000000, -15.41666666666666963, -2.886751345948130876 ) ) ;
#25984=FACE_OUTER_BOUND ( 'NONE', #4741, .T. ) ;
#25986=CARTESIAN_POINT ( 'NONE',  ( -4.458734124999999437, 15.43750000136559386, 0.000000000000000000 ) ) ;
#25993=CARTESIAN_POINT ( 'NONE',  ( 2.229367062499998831, -84.64583333196773651, -3.861377020970580887 ) ) ;
#25994=CARTESIAN_POINT ( 'NONE',  ( 2.229367062500001939, -4.979166665301071326, 3.861377020970579999 ) ) ;
#25995=CARTESIAN_POINT ( 'NONE',  ( -4.999999999999998224, -30.91666666666667140, 2.886751345948131764 ) ) ;
#25997=CARTESIAN_POINT ( 'NONE',  ( 9.457646018065525792E-16, -31.31249999863440436, 5.148502694627439702 ) ) ;
#25998=( BOUNDED_CURVE ( )  B_SPLINE_CURVE ( 2, ( #27038, #26723, #56949, #8061, #31537, #36689, #13189, #41817, #2296 ),
 .UNSPECIFIED., .F., .F. ) 
 B_SPLINE_CURVE_WITH_KNOTS ( ( 3, 2, 2, 2, 3 ),
 ( 0.5437499999999999556, 0.5444444444444443976, 0.5458333333333332815, 0.5472222222222222765, 0.5479166666666667185 ),
 .UNSPECIFIED. ) 
 CURVE ( )  GEOMETRIC_REPRESENTATION_ITEM ( )  RATIONAL_B_SPLINE_CURVE ( ( 0.9330127018922194093, 0.9330127018922194093, 1.000000000000000000, 0.8660254037844387076, 1.000000000000000000, 0.8660254037844387076, 1.000000000000000000, 0.9330127018922194093, 0.9330127018922194093 ) ) 
 REPRESENTATION_ITEM ( '' )  );
#26002=CARTESIAN_POINT ( 'NONE',  ( 4.458734124999998549, 21.27083333469892779, -2.574251347313721627 ) ) ;
#26005=CARTESIAN_POINT ( 'NONE',  ( 1.975475456537005874E-15, -43.62499999726880873, 5.000000000000000000 ) ) ;
#26007=CARTESIAN_POINT ( 'NONE',  ( 2.229367062500001939, -78.22916666530106511, 3.861377020970579999 ) ) ;
#26011=CARTESIAN_POINT ( 'NONE',  ( -2.500000000000000444, 22.95833333606451632, -4.330127018922193649 ) ) ;
#26015=CARTESIAN_POINT ( 'NONE',  ( 3.061616997868383141E-16, -149.7500000000000284, -5.000000000000000000 ) ) ;
#26016=CARTESIAN_POINT ( 'NONE',  ( -4.999999999999999112, -24.91666666666666075, 2.886751345948131764 ) ) ;
#26017=CARTESIAN_POINT ( 'NONE',  ( 2.229367062500001939, -24.97916666530106866, 3.861377020970579999 ) ) ;
#26018=CARTESIAN_POINT ( 'NONE',  ( -2.229367062499996610, -87.14583333196773651, 3.861377020970582219 ) ) ;
#26019=ADVANCED_FACE ( 'NONE', ( #24614 ), #20751, .T. ) ;
#26020=CARTESIAN_POINT ( 'NONE',  ( -5.000000000000000000, -24.87499999726881583, 0.000000000000000000 ) ) ;
#26021=CARTESIAN_POINT ( 'NONE',  ( 4.458734125000001214, -53.89583333196773651, 2.574251347313718519 ) ) ;
#26023=CARTESIAN_POINT ( 'NONE',  ( 1.975475456537005874E-15, -65.74999999999998579, 5.000000000000000000 ) ) ;
#26024=EDGE_CURVE ( 'NONE', #51028, #5037, #37734, .T. ) ;
#26025=CARTESIAN_POINT ( 'NONE',  ( -2.229367062499996610, -1.395833331967737179, 3.861377020970582219 ) ) ;
#26027=CARTESIAN_POINT ( 'NONE',  ( -4.999999999999999112, -71.91666666666667140, 2.886751345948131764 ) ) ;
#26028=ADVANCED_FACE ( 'NONE', ( #49691 ), #30063, .T. ) ;
#26029=CARTESIAN_POINT ( 'NONE',  ( 3.152801135295367541, -152.5625000013655779, -3.152801135295367541 ) ) ;
#26031=CARTESIAN_POINT ( 'NONE',  ( 1.975475456537005874E-15, -13.75000000000000000, 5.000000000000000000 ) ) ;
#26032=CARTESIAN_POINT ( 'NONE',  ( 2.071067811865475505, -159.8125000000000284, -5.000000000000000888 ) ) ;
#26033=EDGE_CURVE ( 'NONE', #21872, #28553, #7696, .T. ) ;
#26036=CARTESIAN_POINT ( 'NONE',  ( 4.458734124999999437, -19.06249999863440792, -5.460374474430324690E-16 ) ) ;
#26037=CARTESIAN_POINT ( 'NONE',  ( 9.457646018065525792E-16, -50.31249999863440792, 5.148502694627439702 ) ) ;
#26039=CARTESIAN_POINT ( 'NONE',  ( 4.458734124999999437, -146.4375000013656063, 0.000000000000000000 ) ) ;
#26044=CARTESIAN_POINT ( 'NONE',  ( -4.458734124999999437, 26.43750000136559564, 0.000000000000000000 ) ) ;
#26046=CYLINDRICAL_SURFACE ( 'NONE', #39381, 5.000000000000000000 ) ;
#26049=AXIS2_PLACEMENT_3D ( 'NONE', #54437, #6506, #25473 ) ;
#26052=CARTESIAN_POINT ( 'NONE',  ( 5.000000000000000000, 11.70833333606451809, -2.886751345948130876 ) ) ;
#26053=CARTESIAN_POINT ( 'NONE',  ( -4.458734124999999437, -8.395833331967736513, -2.574251347313719407 ) ) ;
#26055=CARTESIAN_POINT ( 'NONE',  ( 4.458734124999999437, -149.4375000013656063, 0.000000000000000000 ) ) ;
#26057=ORIENTED_EDGE ( 'NONE', *, *, #35360, .T. ) ;
#26058=CARTESIAN_POINT ( 'NONE',  ( -1.339745962155610925, -62.66965819600734022, 5.000000000000000000 ) ) ;
#26062=CARTESIAN_POINT ( 'NONE',  ( 5.000000000000000000, -88.29166666393548724, -2.886751345948130876 ) ) ;
#26067=CYLINDRICAL_SURFACE ( 'NONE', #23238, 5.000000000000000000 ) ;
#26069=CARTESIAN_POINT ( 'NONE',  ( 4.458734124999998549, 13.27083333469892779, -2.574251347313721627 ) ) ;
#26071=CARTESIAN_POINT ( 'NONE',  ( -2.229367062499996610, -16.39583333196773651, 3.861377020970582219 ) ) ;
#26073=CARTESIAN_POINT ( 'NONE',  ( -1.846868145590734756, -163.1250000013656063, -4.458734125000000326 ) ) ;
#26074=CARTESIAN_POINT ( 'NONE',  ( -4.999999999999998224, -37.91666666666667851, 2.886751345948131764 ) ) ;
#26078=CARTESIAN_POINT ( 'NONE',  ( -5.000000000000000000, -77.08333333333334281, -2.886751345948128211 ) ) ;
#26080=CARTESIAN_POINT ( 'NONE',  ( 2.229367062500001939, -36.97916666530107221, 3.861377020970579999 ) ) ;
#26081=CARTESIAN_POINT ( 'NONE',  ( -6.972266317189433020E-16, -71.25000000000000000, -5.000000000000000000 ) ) ;
#26085=VERTEX_POINT ( 'NONE', #40995 ) ;
#26089=CARTESIAN_POINT ( 'NONE',  ( 2.500000000000002220, -5.666666666666666963, 4.330127018922192761 ) ) ;
#26090=CARTESIAN_POINT ( 'NONE',  ( 2.229367062500001939, -72.97916666530107932, 3.861377020970579999 ) ) ;
#26092=( BOUNDED_CURVE ( )  B_SPLINE_CURVE ( 2, ( #4875, #62493, #19028, #34444, #44100, #9689, #18412, #23563, #57970 ),
 .UNSPECIFIED., .F., .F. ) 
 B_SPLINE_CURVE_WITH_KNOTS ( ( 3, 2, 2, 2, 3 ),
 ( 0.9729166666666666519, 0.9736111111111110938, 0.9749999999999999778, 0.9763888888888888618, 0.9770833333333333037 ),
 .UNSPECIFIED. ) 
 CURVE ( )  GEOMETRIC_REPRESENTATION_ITEM ( )  RATIONAL_B_SPLINE_CURVE ( ( 0.9330127018922194093, 0.9330127018922194093, 1.000000000000000000, 0.8660254037844387076, 1.000000000000000000, 0.8660254037844387076, 1.000000000000000000, 0.9330127018922194093, 0.9330127018922194093 ) ) 
 REPRESENTATION_ITEM ( '' )  );
#26093=CARTESIAN_POINT ( 'NONE',  ( -1.339745962155610925, -16.79465819873852084, 5.000000000000000000 ) ) ;
#26094=CARTESIAN_POINT ( 'NONE',  ( 5.000000000000000000, -7.374999997268813168, -6.123233995736766282E-16 ) ) ;
#26095=CARTESIAN_POINT ( 'NONE',  ( 9.457646018065525792E-16, -37.06249999863440792, 5.148502694627439702 ) ) ;
#26098=CARTESIAN_POINT ( 'NONE',  ( 4.458734124999999437, 10.93750000136559386, -5.460374474430324690E-16 ) ) ;
#26099=ORIENTED_EDGE ( 'NONE', *, *, #27896, .F. ) ;
#26101=CARTESIAN_POINT ( 'NONE',  ( 2.500000000000002220, -48.66666666666666430, 4.330127018922192761 ) ) ;
#26104=CARTESIAN_POINT ( 'NONE',  ( 2.499999999999998668, -4.333333333333334814, -4.330127018922193649 ) ) ;
#26105=CARTESIAN_POINT ( 'NONE',  ( 4.458734124999998549, -76.72916666530106511, -2.574251347313721627 ) ) ;
#26106=CARTESIAN_POINT ( 'NONE',  ( 5.000000000000000888, -169.9375000000000000, -2.071067811865475505 ) ) ;
#26108=CARTESIAN_POINT ( 'NONE',  ( -3.152548672688508926E-16, -85.56249999863439371, -5.148502694627439702 ) ) ;
#26110=CARTESIAN_POINT ( 'NONE',  ( -2.229367062500000163, -34.72916666530107221, -3.861377020970580443 ) ) ;
#26114=ORIENTED_EDGE ( 'NONE', *, *, #7436, .T. ) ;
#26118=CARTESIAN_POINT ( 'NONE',  ( -5.000000000000000000, -75.95833333060214443, -2.886751345948128211 ) ) ;
#26119=CARTESIAN_POINT ( 'NONE',  ( 4.458734125000001214, -64.14583333196773651, 2.574251347313718519 ) ) ;
#26124=ORIENTED_EDGE ( 'NONE', *, *, #49381, .T. ) ;
#26126=CARTESIAN_POINT ( 'NONE',  ( -4.458734124999999437, 8.687500001365595637, 0.000000000000000000 ) ) ;
#26127=CYLINDRICAL_SURFACE ( 'NONE', #12073, 5.000000000000000000 ) ;
#26128=CARTESIAN_POINT ( 'NONE',  ( -4.458734124999999437, -161.9375000013655779, -5.460374474430324690E-16 ) ) ;
#26132=CARTESIAN_POINT ( 'NONE',  ( -9.184850993605147944E-16, -140.3750000027312126, 5.000000000000000000 ) ) ;
#26134=CARTESIAN_POINT ( 'NONE',  ( 6.123233995736766282E-16, -170.0000000000000000, -5.000000000000000000 ) ) ;
#26135=CARTESIAN_POINT ( 'NONE',  ( -1.339745962155613812, -68.20534180126148271, -5.000000000000000000 ) ) ;
#26137=CARTESIAN_POINT ( 'NONE',  ( -1.339745962155613812, -21.20534180126147561, -5.000000000000000000 ) ) ;
#26140=CARTESIAN_POINT ( 'NONE',  ( -4.458734124999997661, 26.77083333469892779, 2.574251347313722516 ) ) ;
#26143=CARTESIAN_POINT ( 'NONE',  ( 4.458734124999998549, 3.020833334698928674, -2.574251347313721627 ) ) ;
#26144=CARTESIAN_POINT ( 'NONE',  ( 3.535533905932738197, -160.0000000027312126, -3.535533905932738197 ) ) ;
#26146=CARTESIAN_POINT ( 'NONE',  ( -9.184850993605147944E-16, -147.3750000027312126, 5.000000000000000000 ) ) ;
#26151=CARTESIAN_POINT ( 'NONE',  ( 3.535533905932738197, -140.8750000000000000, -3.535533905932738197 ) ) ;
#26152=CARTESIAN_POINT ( 'NONE',  ( -5.147856630858197489E-14, 3.249999999999997335, 5.000000000000000000 ) ) ;
#26154=CARTESIAN_POINT ( 'NONE',  ( 1.846868145590736310, -160.8750000013656063, 4.458734124999997661 ) ) ;
#26157=CARTESIAN_POINT ( 'NONE',  ( 4.458734124999999437, -141.4375000013656063, 0.000000000000000000 ) ) ;
#26158=ORIENTED_EDGE ( 'NONE', *, *, #10253, .T. ) ;
#26159=CARTESIAN_POINT ( 'NONE',  ( -4.458734124999999437, 25.43750000136559208, 0.000000000000000000 ) ) ;
#26164=LINE ( 'NONE', #34864, #39092 ) ;
#26165=CARTESIAN_POINT ( 'NONE',  ( 2.500000000000002220, 13.33333333333333215, 4.330127018922192761 ) ) ;
#26166=CARTESIAN_POINT ( 'NONE',  ( 4.458734125000000326, -53.89583333196773651, 2.574251347313718519 ) ) ;
#26167=CARTESIAN_POINT ( 'NONE',  ( -2.229367062500000163, -9.479166665301068662, -3.861377020970580443 ) ) ;
#26171=DIRECTION ( 'NONE',  ( -0.000000000000000000, 1.000000000000000000, -0.000000000000000000 ) ) ;
#26172=CARTESIAN_POINT ( 'NONE',  ( -5.000000000000000000, -32.08333333333333570, -2.886751345948128211 ) ) ;
#26173=DIRECTION ( 'NONE',  ( -0.000000000000000000, 1.000000000000000000, -0.000000000000000000 ) ) ;
#26175=CARTESIAN_POINT ( 'NONE',  ( 2.499999999999998668, 21.79166666939785202, -4.330127018922193649 ) ) ;
#26178=CARTESIAN_POINT ( 'NONE',  ( -4.458734124999999437, -59.39583333196773651, -2.574251347313719407 ) ) ;
#26179=CARTESIAN_POINT ( 'NONE',  ( 2.730187237215162345E-16, -153.4375000013655779, -4.458734124999999437 ) ) ;
#26180=CARTESIAN_POINT ( 'NONE',  ( 4.458734125000001214, -63.89583333196772941, 2.574251347313718519 ) ) ;
#26183=CARTESIAN_POINT ( 'NONE',  ( 5.000000000000000000, -63.29166666393547303, -2.886751345948129988 ) ) ;
#26185=CARTESIAN_POINT ( 'NONE',  ( 2.499999999999998668, -31.20833333060214443, -4.330127018922193649 ) ) ;
#26187=FACE_OUTER_BOUND ( 'NONE', #41335, .T. ) ;
#26189=CARTESIAN_POINT ( 'NONE',  ( 4.458734124999999437, -152.5000000013656347, 1.846868145590737864 ) ) ;
#26193=CARTESIAN_POINT ( 'NONE',  ( 2.500000000000002220, -80.54166666393547303, 4.330127018922192761 ) ) ;
#26194=CARTESIAN_POINT ( 'NONE',  ( 2.229367062499998831, -49.89583333196772941, -3.861377020970580887 ) ) ;
#26198=CARTESIAN_POINT ( 'NONE',  ( -2.229367062499996610, 24.85416666803225993, 3.861377020970582219 ) ) ;
#26200=CARTESIAN_POINT ( 'NONE',  ( 5.000000000000000888, -13.45833333060214976, 2.886751345948126879 ) ) ;
#26202=VERTEX_POINT ( 'NONE', #6918 ) ;
#26207=CARTESIAN_POINT ( 'NONE',  ( 2.500000000000002220, -63.66666666666666430, 4.330127018922192761 ) ) ;
#26208=CARTESIAN_POINT ( 'NONE',  ( 3.535533905932736864, -157.2500000027312126, 3.535533905932738641 ) ) ;
#26211=CARTESIAN_POINT ( 'NONE',  ( 5.000000000000000000, -23.29166666393548368, -2.886751345948130876 ) ) ;
#26212=CARTESIAN_POINT ( 'NONE',  ( 0.000000000000000000, -170.0000000000000000, 0.000000000000000000 ) ) ;
#26215=VERTEX_POINT ( 'NONE', #41305 ) ;
#26218=CARTESIAN_POINT ( 'NONE',  ( -5.000000000000000000, -157.6250000027311842, -6.123233995736766282E-16 ) ) ;
#26219=ORIENTED_EDGE ( 'NONE', *, *, #12505, .T. ) ;
#26228=CARTESIAN_POINT ( 'NONE',  ( -2.229367062500000163, -17.47916666530106866, -3.861377020970580443 ) ) ;
#26229=CARTESIAN_POINT ( 'NONE',  ( 5.000000000000000888, -75.58333333333334281, 2.886751345948126879 ) ) ;
#26230=CARTESIAN_POINT ( 'NONE',  ( -5.000000000000000888, -149.4375000000000000, 2.071067811865474617 ) ) ;
#26232=CARTESIAN_POINT ( 'NONE',  ( -1.846868145590737420, -150.7500000013655779, 4.458734124999999437 ) ) ;
#26233=ORIENTED_EDGE ( 'NONE', *, *, #35453, .F. ) ;
#26234=CARTESIAN_POINT ( 'NONE',  ( 4.458734124999999437, -47.06249999863440792, -5.460374474430324690E-16 ) ) ;
#26237=CARTESIAN_POINT ( 'NONE',  ( -2.229367062499996610, -88.14583333196773651, 3.861377020970582219 ) ) ;
#26238=CARTESIAN_POINT ( 'NONE',  ( -3.152548672688508926E-16, 6.437500001365592972, -5.148502694627439702 ) ) ;
#26239=CARTESIAN_POINT ( 'NONE',  ( 0.000000000000000000, -170.0000000000000000, 5.000000000000000000 ) ) ;
#26241=CARTESIAN_POINT ( 'NONE',  ( -4.458734124999998549, 13.52083333469892779, 2.574251347313722516 ) ) ;
#26242=CARTESIAN_POINT ( 'NONE',  ( -2.500000000000000444, 1.958333336064519647, -4.330127018922193649 ) ) ;
#26243=ORIENTED_EDGE ( 'NONE', *, *, #42116, .T. ) ;
#26244=CARTESIAN_POINT ( 'NONE',  ( 2.071067811865401787, -161.9375000027311842, -5.000000000000074607 ) ) ;
#26245=VERTEX_POINT ( 'NONE', #8421 ) ;
#26247=CARTESIAN_POINT ( 'NONE',  ( 4.458734125000001214, -45.89583333196774362, 2.574251347313718519 ) ) ;
#26248=CARTESIAN_POINT ( 'NONE',  ( -1.846868145590734756, -163.3750000013656347, -4.458734125000000326 ) ) ;
#26249=CARTESIAN_POINT ( 'NONE',  ( 5.000000000000000000, -37.37499999726881583, -6.123233995736766282E-16 ) ) ;
#26251=CARTESIAN_POINT ( 'NONE',  ( 9.457646018065525792E-16, -18.06249999863440436, 5.148502694627439702 ) ) ;
#26253=CARTESIAN_POINT ( 'NONE',  ( -2.500000000000000444, -89.16666666666665719, -4.330127018922193649 ) ) ;
#26254=CARTESIAN_POINT ( 'NONE',  ( -4.458734125000000326, -166.0000000013656063, -1.846868145590735644 ) ) ;
#26255=CARTESIAN_POINT ( 'NONE',  ( -4.999999999999999112, -85.79166666393547303, 2.886751345948131764 ) ) ;
#26256=CARTESIAN_POINT ( 'NONE',  ( -1.339745962155613812, -61.08034179853027723, -5.000000000000000000 ) ) ;
#26259=CARTESIAN_POINT ( 'NONE',  ( -2.229367062499996610, -31.39583333196773651, 3.861377020970582219 ) ) ;
#26260=CARTESIAN_POINT ( 'NONE',  ( 1.975475456537005874E-15, -29.74999999999999645, 5.000000000000000000 ) ) ;
#26262=VECTOR ( 'NONE', #53015, 1000.000000000000114 ) ;
#26263=( BOUNDED_CURVE ( )  B_SPLINE_CURVE ( 2, ( #39345, #15227, #5580, #59295, #20707, #40312, #49643, #58975, #59950 ),
 .UNSPECIFIED., .F., .F. ) 
 B_SPLINE_CURVE_WITH_KNOTS ( ( 3, 2, 2, 2, 3 ),
 ( 0.3083333333333336257, 0.3125000000000002776, 0.3166666666666669294, 0.3208333333333336368, 0.3250000000000002887 ),
 .UNSPECIFIED. ) 
 CURVE ( )  GEOMETRIC_REPRESENTATION_ITEM ( )  RATIONAL_B_SPLINE_CURVE ( ( 0.9999999999999948930, 0.9238795325112918455, 1.000000000000000000, 0.9238795325112867385, 1.000000000000000000, 0.9238795325112867385, 1.000000000000000000, 0.9238795325112816315, 1.000000000000005107 ) ) 
 REPRESENTATION_ITEM ( '' )  );
#26268=CARTESIAN_POINT ( 'NONE',  ( -2.071067811865394237, -161.3125000000000284, 5.000000000000084377 ) ) ;
#26270=CARTESIAN_POINT ( 'NONE',  ( 4.458734124999999437, -83.06249999863440792, -5.460374474430324690E-16 ) ) ;
#26273=CARTESIAN_POINT ( 'NONE',  ( -4.458734124999999437, -142.2500000013656063, -1.846868145590735644 ) ) ;
#26274=DIRECTION ( 'NONE',  ( -0.000000000000000000, 1.000000000000000000, -0.000000000000000000 ) ) ;
#26276=CARTESIAN_POINT ( 'NONE',  ( -4.458734124999999437, -43.39583333196773651, -2.574251347313719407 ) ) ;
#26280=CARTESIAN_POINT ( 'NONE',  ( 3.535533905932738197, -159.0000000027312126, -3.535533905932738197 ) ) ;
#26285=CARTESIAN_POINT ( 'NONE',  ( -4.458734124999998549, -81.47916666530106511, 2.574251347313722516 ) ) ;
#26286=CARTESIAN_POINT ( 'NONE',  ( 5.000000000000000000, -34.50000000000000000, -6.123233995736766282E-16 ) ) ;
#26288=CARTESIAN_POINT ( 'NONE',  ( 2.499999999999998668, -76.33333333333334281, -4.330127018922193649 ) ) ;
#26291=CARTESIAN_POINT ( 'NONE',  ( 3.535533905932736864, -146.1250000000000000, 3.535533905932738641 ) ) ;
#26293=CARTESIAN_POINT ( 'NONE',  ( 1.975475456537005874E-15, -62.62499999726880873, 5.000000000000000000 ) ) ;
#26295=CARTESIAN_POINT ( 'NONE',  ( 4.458734125000000326, 9.854166668032261711, 2.574251347313718519 ) ) ;
#26303=CARTESIAN_POINT ( 'NONE',  ( -5.000000000000000000, -13.87499999726881228, 0.000000000000000000 ) ) ;
#26304=CARTESIAN_POINT ( 'NONE',  ( -4.458734124999999437, -87.31249999863439371, 0.000000000000000000 ) ) ;
#26305=CARTESIAN_POINT ( 'NONE',  ( 4.458734124999998549, -1.729166665301068440, -2.574251347313721627 ) ) ;
#26308=CARTESIAN_POINT ( 'NONE',  ( 4.458734124999999437, -30.06249999863440436, -5.460374474430324690E-16 ) ) ;
#26313=EDGE_CURVE ( 'NONE', #41008, #12871, #40545, .T. ) ;
#26314=AXIS2_PLACEMENT_3D ( 'NONE', #33107, #2580, #8353 ) ;
#26315=CARTESIAN_POINT ( 'NONE',  ( -2.229367062499996610, 19.85416666803225993, 3.861377020970582219 ) ) ;
#26316=CARTESIAN_POINT ( 'NONE',  ( 1.339745962155612702, -53.29465819873850307, -5.000000000000000000 ) ) ;
#26317=CARTESIAN_POINT ( 'NONE',  ( 5.000000000000000000, 1.500000000000001332, -6.123233995736766282E-16 ) ) ;
#26318=CARTESIAN_POINT ( 'NONE',  ( 9.457646018065525792E-16, -80.31249999863440792, 5.148502694627439702 ) ) ;
#26320=( BOUNDED_CURVE ( )  B_SPLINE_CURVE ( 2, ( #39372, #38428, #5296, #24914, #34227, #53854, #9783, #59003, #10430 ),
 .UNSPECIFIED., .F., .F. ) 
 B_SPLINE_CURVE_WITH_KNOTS ( ( 3, 2, 2, 2, 3 ),
 ( 0.7187500000000000000, 0.7194444444444444420, 0.7208333333333333259, 0.7222222222222222099, 0.7229166666666666519 ),
 .UNSPECIFIED. ) 
 CURVE ( )  GEOMETRIC_REPRESENTATION_ITEM ( )  RATIONAL_B_SPLINE_CURVE ( ( 0.9330127018922194093, 0.9330127018922194093, 1.000000000000000000, 0.8660254037844387076, 1.000000000000000000, 0.8660254037844387076, 1.000000000000000000, 0.9330127018922194093, 0.9330127018922194093 ) ) 
 REPRESENTATION_ITEM ( '' )  );
#26321=CARTESIAN_POINT ( 'NONE',  ( -6.972266317189433020E-16, -11.25000000000000178, -5.000000000000000000 ) ) ;
#26322=CARTESIAN_POINT ( 'NONE',  ( 2.499999999999998668, 24.79166666939785202, -4.330127018922193649 ) ) ;
#26326=CARTESIAN_POINT ( 'NONE',  ( 3.061616997868383141E-16, -168.8750000027312126, -5.000000000000000000 ) ) ;
#26327=CARTESIAN_POINT ( 'NONE',  ( -4.999999999999999112, -25.91666666666666430, 2.886751345948131764 ) ) ;
#26328=CARTESIAN_POINT ( 'NONE',  ( -2.229367062499996610, -28.14583333196774007, 3.861377020970582219 ) ) ;
#26329=CARTESIAN_POINT ( 'NONE',  ( -2.229367062500000163, -89.47916666530106511, -3.861377020970580443 ) ) ;
#26330=CARTESIAN_POINT ( 'NONE',  ( 2.500000000000002220, -22.54166666393548013, 4.330127018922192761 ) ) ;
#26331=ADVANCED_FACE ( 'NONE', ( #14482 ), #15128, .T. ) ;
#26332=CARTESIAN_POINT ( 'NONE',  ( 2.229367062500001939, -57.97916666530107932, 3.861377020970579999 ) ) ;
#26334=CARTESIAN_POINT ( 'NONE',  ( 5.000000000000000000, -27.41666666666666430, -2.886751345948130876 ) ) ;
#26335=LINE ( 'NONE', #16691, #11797 ) ;
#26336=CARTESIAN_POINT ( 'NONE',  ( 4.458734124999998549, -3.979166665301070438, -2.574251347313721627 ) ) ;
#26337=ORIENTED_EDGE ( 'NONE', *, *, #61736, .F. ) ;
#26338=CARTESIAN_POINT ( 'NONE',  ( -2.500000000000000444, -73.16666666666665719, -4.330127018922193649 ) ) ;
#26339=CARTESIAN_POINT ( 'NONE',  ( -8.190561711645485556E-16, -152.9375000013655779, 4.458734124999999437 ) ) ;
#26341=CARTESIAN_POINT ( 'NONE',  ( 5.000000000000000000, -160.0000000000000000, 0.000000000000000000 ) ) ;
#26342=CARTESIAN_POINT ( 'NONE',  ( -4.999999999999999112, -72.79166666393547303, 2.886751345948131764 ) ) ;
#26343=CARTESIAN_POINT ( 'NONE',  ( -5.000000000000000000, -86.00000000000000000, 0.000000000000000000 ) ) ;
#26345=CARTESIAN_POINT ( 'NONE',  ( 9.457646018065525792E-16, -17.31249999863440436, 5.148502694627439702 ) ) ;
#26346=CARTESIAN_POINT ( 'NONE',  ( -4.458734124999999437, -52.56249999863440792, 0.000000000000000000 ) ) ;
#26348=CARTESIAN_POINT ( 'NONE',  ( -3.152801135295367985, -142.8125000013655779, 3.152801135295367096 ) ) ;
#26352=CARTESIAN_POINT ( 'NONE',  ( -3.535533905932737309, -155.6250000000000000, -3.535533905932738197 ) ) ;
#26353=CARTESIAN_POINT ( 'NONE',  ( -4.458734124999999437, 25.35416666803225993, -2.574251347313719407 ) ) ;
#26355=VECTOR ( 'NONE', #58512, 1000.000000000000000 ) ;
#26356=DIRECTION ( 'NONE',  ( -0.000000000000000000, 1.000000000000000000, -0.000000000000000000 ) ) ;
#26363=CARTESIAN_POINT ( 'NONE',  ( -2.229367062500000163, -62.72916666530106511, -3.861377020970580443 ) ) ;
#26364=CARTESIAN_POINT ( 'NONE',  ( 1.975475456537005874E-15, -2.624999997268813168, 5.000000000000000000 ) ) ;
#26365=CARTESIAN_POINT ( 'NONE',  ( 9.457646018065525792E-16, -6.062499998634403475, 5.148502694627439702 ) ) ;
#26367=CARTESIAN_POINT ( 'NONE',  ( -3.152801135295367096, -147.0625000013655779, -3.152801135295367541 ) ) ;
#26377=CARTESIAN_POINT ( 'NONE',  ( 5.000000000000000000, 1.708333336064519425, -2.886751345948130876 ) ) ;
#26382=CARTESIAN_POINT ( 'NONE',  ( -2.500000000000000444, -90.04166666393547303, -4.330127018922193649 ) ) ;
#26383=EDGE_CURVE ( 'NONE', #25740, #1775, #16325, .T. ) ;
#26384=CARTESIAN_POINT ( 'NONE',  ( -4.999999999999998224, -14.91666666666666785, 2.886751345948131764 ) ) ;
#26385=CARTESIAN_POINT ( 'NONE',  ( -2.229367062500000163, 14.52083333469892779, -3.861377020970580443 ) ) ;
#26387=CARTESIAN_POINT ( 'NONE',  ( -2.229367062499996610, -14.39583333196774184, 3.861377020970582219 ) ) ;
#26389=CARTESIAN_POINT ( 'NONE',  ( -1.846868145590734756, -162.1250000013655779, -4.458734125000000326 ) ) ;
#26390=CARTESIAN_POINT ( 'NONE',  ( 1.975475456537005874E-15, -37.74999999999999289, 5.000000000000000000 ) ) ;
#26393=CARTESIAN_POINT ( 'NONE',  ( -2.500000000000000444, 9.833333333333332149, -4.330127018922193649 ) ) ;
#26394=CARTESIAN_POINT ( 'NONE',  ( -6.972266317189433020E-16, -36.25000000000000000, -5.000000000000000000 ) ) ;
#26395=CARTESIAN_POINT ( 'NONE',  ( -4.458734124999999437, -37.31249999863440792, 0.000000000000000000 ) ) ;
#26399=CARTESIAN_POINT ( 'NONE',  ( 0.000000000000000000, -170.0000000000000000, 0.000000000000000000 ) ) ;
#26405=CARTESIAN_POINT ( 'NONE',  ( -5.000000000000000000, -8.083333333333330373, -2.886751345948128211 ) ) ;
#26406=CARTESIAN_POINT ( 'NONE',  ( -4.458734124999997661, -70.22916666530107932, 2.574251347313722516 ) ) ;
#26407=AXIS2_PLACEMENT_3D ( 'NONE', #48040, #28730, #21800 ) ;
#26409=CARTESIAN_POINT ( 'NONE',  ( 5.000000000000000000, -7.291666663935481907, -2.886751345948129988 ) ) ;
#26410=CARTESIAN_POINT ( 'NONE',  ( 4.458734124999999437, -39.81249999863440081, -5.460374474430324690E-16 ) ) ;
#26414=CARTESIAN_POINT ( 'NONE',  ( -3.152548672688508926E-16, 14.18750000136559386, -5.148502694627439702 ) ) ;
#26417=CARTESIAN_POINT ( 'NONE',  ( 5.000000000000000000, -55.41666666666667140, -2.886751345948129988 ) ) ;
#26420=CARTESIAN_POINT ( 'NONE',  ( -4.458734124999998549, -75.22916666530106511, 2.574251347313722516 ) ) ;
#26421=CARTESIAN_POINT ( 'NONE',  ( 3.061616997868383141E-16, -168.7500000000000000, -5.000000000000000000 ) ) ;
#26422=CARTESIAN_POINT ( 'NONE',  ( -4.458734124999998549, -86.22916666530106511, 2.574251347313722516 ) ) ;
#26424=CARTESIAN_POINT ( 'NONE',  ( 4.458734125000001214, -35.14583333196772941, 2.574251347313718519 ) ) ;
#26425=CARTESIAN_POINT ( 'NONE',  ( -9.184850993605147944E-16, -150.3750000027312126, 5.000000000000000000 ) ) ;
#26426=ORIENTED_EDGE ( 'NONE', *, *, #8291, .F. ) ;
#26430=DIRECTION ( 'NONE',  ( -0.000000000000000000, 1.000000000000000000, -0.000000000000000000 ) ) ;
#26431=CARTESIAN_POINT ( 'NONE',  ( -6.972266317189433020E-16, -19.12499999726880873, -5.000000000000000000 ) ) ;
#26432=CARTESIAN_POINT ( 'NONE',  ( -3.152548672688508926E-16, -64.81249999863440792, -5.148502694627439702 ) ) ;
#26435=CARTESIAN_POINT ( 'NONE',  ( -2.071067811865351604, -156.4375000027311842, 5.000000000000126121 ) ) ;
#26438=VERTEX_POINT ( 'NONE', #30550 ) ;
#26440=CARTESIAN_POINT ( 'NONE',  ( 4.458734124999999437, 10.18750000136559386, -5.460374474430324690E-16 ) ) ;
#26441=CARTESIAN_POINT ( 'NONE',  ( 2.071067811865264563, -153.8125000000000000, -5.000000000000211386 ) ) ;
#26442=CARTESIAN_POINT ( 'NONE',  ( -4.458734125000000326, -157.8750000013655779, 1.846868145590734089 ) ) ;
#26444=VECTOR ( 'NONE', #48649, 1000.000000000000000 ) ;
#26448=CARTESIAN_POINT ( 'NONE',  ( 0.000000000000000000, -170.0000000000000000, 0.000000000000000000 ) ) ;
#26453=( BOUNDED_CURVE ( )  B_SPLINE_CURVE ( 2, ( #36252, #50412, #60068, #61341, #17263, #31409, #56517, #55244, #12438 ),
 .UNSPECIFIED., .F., .F. ) 
 B_SPLINE_CURVE_WITH_KNOTS ( ( 3, 2, 2, 2, 3 ),
 ( 0.04375000000000000416, 0.04444444444444444614, 0.04583333333333333010, 0.04722222222222222099, 0.04791666666666666990 ),
 .UNSPECIFIED. ) 
 CURVE ( )  GEOMETRIC_REPRESENTATION_ITEM ( )  RATIONAL_B_SPLINE_CURVE ( ( 0.9330127018922192983, 0.9330127018922196314, 1.000000000000000000, 0.8660254037844387076, 1.000000000000000000, 0.8660254037844387076, 1.000000000000000000, 0.9330127018922189652, 0.9330127018922192983 ) ) 
 REPRESENTATION_ITEM ( '' )  );
#26459=CARTESIAN_POINT ( 'NONE',  ( 1.339745962155615144, -58.70534180126147561, 4.999999999999999112 ) ) ;
#26463=CARTESIAN_POINT ( 'NONE',  ( 4.458734124999999437, 1.937500001365593416, -5.460374474430324690E-16 ) ) ;
#26464=CARTESIAN_POINT ( 'NONE',  ( -9.184850993605147944E-16, -160.3750000027311842, 5.000000000000000000 ) ) ;
#26467=CARTESIAN_POINT ( 'NONE',  ( 5.000000000000000888, -147.0625000027311842, -2.071067811865475505 ) ) ;
#26472=CARTESIAN_POINT ( 'NONE',  ( -6.972266317189433020E-16, -87.25000000000001421, -5.000000000000000000 ) ) ;
#26474=CARTESIAN_POINT ( 'NONE',  ( -1.339745962155610925, -87.79465819873851729, 5.000000000000000000 ) ) ;
#26476=CARTESIAN_POINT ( 'NONE',  ( -4.458734124999999437, -161.1875000013655779, -5.460374474430324690E-16 ) ) ;
#26479=CARTESIAN_POINT ( 'NONE',  ( -3.152801135295367985, -140.8125000013655779, 3.152801135295367096 ) ) ;
#26481=CARTESIAN_POINT ( 'NONE',  ( 4.458734125000001214, 22.85416666803225993, 2.574251347313718519 ) ) ;
#26486=LINE ( 'NONE', #1107, #19588 ) ;
#26487=CARTESIAN_POINT ( 'NONE',  ( -3.535250795749689387E-16, 9.749999999999998224, -5.773502691896257311 ) ) ;
#26488=CARTESIAN_POINT ( 'NONE',  ( 2.229367062500001939, -55.97916666530107221, 3.861377020970579999 ) ) ;
#26489=CARTESIAN_POINT ( 'NONE',  ( -2.229367062499996610, -14.14583333196774184, 3.861377020970582219 ) ) ;
#26493=DIRECTION ( 'NONE',  ( -0.000000000000000000, 1.000000000000000000, -0.000000000000000000 ) ) ;
#26494=CARTESIAN_POINT ( 'NONE',  ( -3.535250795749689387E-16, -37.25000000000001421, -5.773502691896257311 ) ) ;
#26495=CARTESIAN_POINT ( 'NONE',  ( 6.123233995736766282E-16, -170.0000000000000000, -5.000000000000000000 ) ) ;
#26500=CARTESIAN_POINT ( 'NONE',  ( 2.229367062500001939, -58.97916666530106511, 3.861377020970579999 ) ) ;
#26501=CARTESIAN_POINT ( 'NONE',  ( 4.458734124999999437, -153.7500000013656063, 1.846868145590737864 ) ) ;
#26502=CARTESIAN_POINT ( 'NONE',  ( -2.229367062499996610, -70.14583333196773651, 3.861377020970582219 ) ) ;
#26503=AXIS2_PLACEMENT_3D ( 'NONE', #7552, #32616, #42580 ) ;
#26505=CARTESIAN_POINT ( 'NONE',  ( -2.229367062500000163, -18.72916666530106866, -3.861377020970580443 ) ) ;
#26506=CARTESIAN_POINT ( 'NONE',  ( -4.999999999999999112, -60.79166666393547303, 2.886751345948131764 ) ) ;
#26508=ORIENTED_EDGE ( 'NONE', *, *, #9075, .T. ) ;
#26510=DIRECTION ( 'NONE',  ( 0.000000000000000000, 0.000000000000000000, 1.000000000000000000 ) ) ;
#26511=CARTESIAN_POINT ( 'NONE',  ( -4.458734125000001214, -150.8750000013655779, 1.846868145590734089 ) ) ;
#26515=CARTESIAN_POINT ( 'NONE',  ( 1.975475456537005874E-15, -64.62499999726880162, 5.000000000000000000 ) ) ;
#26516=CARTESIAN_POINT ( 'NONE',  ( -2.229367062500000163, -48.72916666530106511, -3.861377020970580443 ) ) ;
#26517=ORIENTED_EDGE ( 'NONE', *, *, #31885, .F. ) ;
#26520=CARTESIAN_POINT ( 'NONE',  ( 4.458734125000001214, 26.10416666803225993, 2.574251347313718519 ) ) ;
#26524=( BOUNDED_CURVE ( )  B_SPLINE_CURVE ( 2, ( #62213, #18129, #61581, #12364, #31978, #36487, #61900, #2719, #57074, #27781, #56756, #12679, #28096, #31663, #37756, #22342, #7860, #51613, #32932, #47405, #41612, #42573, #47714, #51299, #41940, #42884, #57388, #7546, #26849, #17516, #52555, #3669, #37136, #56114, #23282, #12038, #46462, #2405, #43196, #9730, #19386, #49296, #62530, #53486, #39002, #8797, #9110, #28717, #58004, #54112, #9415, #48341, #58634, #5236, #48963, #24535, #108, #23599, #62838, #3979, #29025, #48650, #18449, #43821, #24856, #14244, #38072, #63467, #19704, #57700, #58319, #52864, #13626, #34173, #33867, #4592, #33244, #29333, #39313, #43506, #28409, #4915, #18753, #38377, #24215, #44138, #4287, #14554, #48029, #10052, #53796, #58941, #23905, #14871, #13930, #34480, #29665, #33555, #53176, #63151, #19062, #38680, #21305, #30627, #20349, #35462, #740, #36097, #55724, #55406, #50893, #1071, #59267, #15199, #39948, #60555, #45105, #35784, #44460, #419, #26128, #25484, #44778, #59596, #20023, #6197, #10693, #45425, #1390, #20677, #40283, #11638, #34824, #45748, #30303, #59921, #15529, #40910, #15843, #49613, #25164, #31259, #54447, #54765, #6835, #11322, #35149, #10375, #49923, #50249, #1702, #5876, #39629, #55083, #11005, #20990, #16477, #25812, #30947, #40594, #60239, #29983, #16157, #50573, #5552, #6516, #36734, #21939, #18050, #17438, #56366, #22585, #13231, #12909, #52160, #27707, #51219, #26766, #31585, #37055, #22900, #46064, #7784, #52482, #41861, #26442, #27387, #47334, #2024, #22262, #16794, #32854, #61822, #61508, #56683, #21629, #37364, #3284, #7470, #41221, #27079, #7156, #46386, #12599, #8103, #12288, #42183, #36412, #37672, #17747, #41537, #31904, #56994, #60868, #56042, #2332, #62132, #47019, #11958, #61189, #32212, #17111, #32531, #51533, #46695, #51841, #42495, #2643, #2969, #57313, #8416, #13854, #19308, #38922, #29263, #23198, #48260, #47638, #18989, #28019, #53408, #38604, #9654, #9340, #33477, #53099, #14795, #58557, #34407, #39237, #4836, #47948, #26, #34098, #53723, #42811, #58863, #58237, #14477, #13554, #52788, #3902, #63390, #3593, #4517, #63079, #14164, #48891, #4218, #62451, #28645, #48577, #24143, #33792, #9033, #43746, #8720, #24455, #44061, #18373, #23831, #28954, #19627, #37994, #57626, #33173, #23521, #28334, #43122, #62762, #18682, #38308, #57935, #43434, #5157, #24777, #29906, #6446, #54687, #45352, #54036, #59194, #19941, #44698, #5794, #10298, #40835, #21229, #34743, #60480, #16083, #59842, #35707, #55334, #50170, #20272, #50503, #998, #29585, #59518, #26055, #15123, #54371, #15767, #6124, #25738, #9974, #20602, #44380, #49217, #30223, #11251, #20914, #16405, #45669, #341, #55003, #49534, #39553, #1628, #5475, #15453, #1319, #40518, #30875, #25090, #49848, #663, #40206, #39871, #35383, #35070, #25411, #10610, #10931, #45030, #30546, #60162, #26367, #22827, #7715, #11880, #27634, #61748, #17675, #50818, #3207, #2570, #22507, #41149, #16722, #31829, #37290, #21869, #32136, #45986, #47262, #27319, #51144, #46309, #46948, #12524, #51771, #46624, #61116, #2895, #36338, #12837, #32457, #1952, #51460, #31189, #42102, #42417, #22186, #36023, #55969, #8027, #56919, #31499, #7078, #52089, #62060, #56285, #6755, #21553, #26692, #55655, #36656, #11569, #60796, #2266, #41465, #17040, #12211, #7398, #27005, #41787, #61431, #17355, #36979, #56607, #13783, #9587, #32778, #63311, #47870, #33405, #57554, #14409, #53020, #23127, #62376, #23764, #33718, #53337, #37597, #28571, #8343, #17973, #57861, #4145, #38849, #8645, #57241, #48192, #8961, #18918, #58483, #18299, #28886, #38532, #58160, #42731, #48507, #43363, #37922, #9270, #13157, #27942, #63009, #14092, #3830, #4445, #24074, #23449, #34031, #43670, #52412, #43053, #53652, #3516, #24385, #19233, #29193, #47565, #28258, #43986, #48819, #52711, #13480 ),
 .UNSPECIFIED., .F., .F. ) 
 B_SPLINE_CURVE_WITH_KNOTS ( ( 3, 2, 2, 2, 2, 2, 2, 2, 2, 2, 2, 2, 2, 2, 2, 2, 2, 2, 2, 2, 2, 2, 2, 2, 2, 2, 2, 2, 2, 2, 2, 2, 2, 2, 2, 2, 2, 2, 2, 2, 2, 2, 2, 2, 2, 2, 2, 2, 2, 2, 2, 2, 2, 2, 2, 2, 2, 2, 2, 2, 2, 2, 2, 2, 2, 2, 2, 2, 2, 2, 2, 2, 2, 2, 2, 2, 2, 2, 2, 2, 2, 2, 2, 2, 2, 2, 2, 2, 2, 2, 2, 2, 2, 2, 2, 2, 2, 2, 2, 2, 2, 2, 2, 2, 2, 2, 2, 2, 2, 2, 2, 2, 2, 2, 2, 2, 2, 2, 2, 2, 2, 2, 2, 2, 2, 2, 2, 2, 2, 2, 2, 2, 2, 2, 2, 2, 2, 2, 2, 2, 2, 2, 2, 2, 2, 2, 2, 2, 2, 2, 2, 2, 2, 2, 2, 2, 2, 2, 2, 2, 2, 2, 2, 2, 2, 2, 2, 2, 2, 2, 2, 2, 2, 2, 2, 2, 2, 2, 2, 2, 2, 2, 2, 2, 2, 2, 2, 2, 2, 2, 2, 2, 2, 2, 2, 2, 2, 2, 2, 2, 2, 2, 2, 2, 2, 2, 2, 2, 2, 2, 2, 2, 2, 2, 2, 2, 2, 2, 2, 2, 2, 2, 2, 2, 2, 2, 2, 2, 2, 2, 2, 2, 2, 2, 2, 2, 2, 2, 2, 2, 3 ),
 ( 0.000000000000000000, 0.004166666666666666609, 0.008333333333333333218, 0.01250000000000000069, 0.01666666666666666644, 0.02083333333333333218, 0.02500000000000000139, 0.02916666666666666713, 0.03333333333333333287, 0.03749999999999999861, 0.04166666666666666435, 0.04583333333333333010, 0.05000000000000000278, 0.05416666666666666852, 0.05833333333333333426, 0.06250000000000000000, 0.06666666666666666574, 0.07083333333333333148, 0.07499999999999999722, 0.07916666666666666297, 0.08333333333333332871, 0.08749999999999999445, 0.09166666666666666019, 0.09583333333333333981, 0.1000000000000000056, 0.1041666666666666713, 0.1083333333333333370, 0.1125000000000000028, 0.1166666666666666685, 0.1208333333333333343, 0.1250000000000000000, 0.1291666666666666796, 0.1333333333333333315, 0.1375000000000000111, 0.1416666666666666630, 0.1458333333333333426, 0.1499999999999999944, 0.1541666666666666741, 0.1583333333333333259, 0.1625000000000000056, 0.1666666666666666574, 0.1708333333333333370, 0.1749999999999999889, 0.1791666666666666685, 0.1833333333333333204, 0.1875000000000000000, 0.1916666666666666796, 0.1958333333333333315, 0.2000000000000000111, 0.2041666666666666630, 0.2083333333333333426, 0.2124999999999999944, 0.2166666666666666741, 0.2208333333333333259, 0.2250000000000000056, 0.2291666666666666574, 0.2333333333333333370, 0.2374999999999999889, 0.2416666666666666685, 0.2458333333333333204, 0.2500000000000000000, 0.2541666666666666519, 0.2583333333333333592, 0.2625000000000000111, 0.2666666666666666630, 0.2708333333333333148, 0.2750000000000000222, 0.2791666666666666741, 0.2833333333333333259, 0.2874999999999999778, 0.2916666666666666852, 0.2958333333333333370, 0.2999999999999999889, 0.3041666666666666408, 0.3083333333333333481, 0.3125000000000000000, 0.3166666666666666519, 0.3208333333333333592, 0.3250000000000000111, 0.3291666666666666630, 0.3333333333333333148, 0.3375000000000000222, 0.3416666666666666741, 0.3458333333333333259, 0.3499999999999999778, 0.3541666666666666852, 0.3583333333333333370, 0.3624999999999999889, 0.3666666666666666408, 0.3708333333333333481, 0.3750000000000000000, 0.3791666666666666519, 0.3833333333333333592, 0.3875000000000000111, 0.3916666666666666630, 0.3958333333333333148, 0.4000000000000000222, 0.4041666666666666741, 0.4083333333333333259, 0.4124999999999999778, 0.4166666666666666852, 0.4208333333333333370, 0.4249999999999999889, 0.4291666666666666408, 0.4333333333333333481, 0.4375000000000000000, 0.4416666666666666519, 0.4458333333333333592, 0.4500000000000000111, 0.4541666666666666630, 0.4583333333333333148, 0.4625000000000000222, 0.4666666666666666741, 0.4708333333333333259, 0.4749999999999999778, 0.4791666666666666852, 0.4833333333333333370, 0.4874999999999999889, 0.4916666666666666408, 0.4958333333333333481, 0.5000000000000000000, 0.5041666666666666519, 0.5083333333333333037, 0.5124999999999999556, 0.5166666666666667185, 0.5208333333333333703, 0.5250000000000000222, 0.5291666666666666741, 0.5333333333333333259, 0.5374999999999999778, 0.5416666666666666297, 0.5458333333333332815, 0.5500000000000000444, 0.5541666666666666963, 0.5583333333333333481, 0.5625000000000000000, 0.5666666666666666519, 0.5708333333333333037, 0.5749999999999999556, 0.5791666666666667185, 0.5833333333333333703, 0.5875000000000000222, 0.5916666666666666741, 0.5958333333333333259, 0.5999999999999999778, 0.6041666666666666297, 0.6083333333333332815, 0.6125000000000000444, 0.6166666666666666963, 0.6208333333333333481, 0.6250000000000000000, 0.6291666666666666519, 0.6333333333333333037, 0.6374999999999999556, 0.6416666666666667185, 0.6458333333333333703, 0.6500000000000000222, 0.6541666666666666741, 0.6583333333333333259, 0.6624999999999999778, 0.6666666666666666297, 0.6708333333333332815, 0.6750000000000000444, 0.6791666666666666963, 0.6833333333333333481, 0.6875000000000000000, 0.6916666666666666519, 0.6958333333333333037, 0.6999999999999999556, 0.7041666666666667185, 0.7083333333333333703, 0.7125000000000000222, 0.7166666666666666741, 0.7208333333333333259, 0.7249999999999999778, 0.7291666666666666297, 0.7333333333333332815, 0.7375000000000000444, 0.7416666666666666963, 0.7458333333333333481, 0.7500000000000000000, 0.7541666666666666519, 0.7583333333333333037, 0.7624999999999999556, 0.7666666666666667185, 0.7708333333333333703, 0.7750000000000000222, 0.7791666666666666741, 0.7833333333333333259, 0.7874999999999999778, 0.7916666666666666297, 0.7958333333333332815, 0.8000000000000000444, 0.8041666666666666963, 0.8083333333333333481, 0.8125000000000000000, 0.8166666666666666519, 0.8208333333333333037, 0.8249999999999999556, 0.8291666666666667185, 0.8333333333333333703, 0.8375000000000000222, 0.8416666666666666741, 0.8458333333333333259, 0.8499999999999999778, 0.8541666666666666297, 0.8583333333333332815, 0.8625000000000000444, 0.8666666666666666963, 0.8708333333333333481, 0.8750000000000000000, 0.8791666666666666519, 0.8833333333333333037, 0.8874999999999999556, 0.8916666666666667185, 0.8958333333333333703, 0.9000000000000000222, 0.9041666666666666741, 0.9083333333333333259, 0.9124999999999999778, 0.9166666666666666297, 0.9208333333333332815, 0.9250000000000000444, 0.9291666666666666963, 0.9333333333333333481, 0.9375000000000000000, 0.9416666666666666519, 0.9458333333333333037, 0.9499999999999999556, 0.9541666666666667185, 0.9583333333333333703, 0.9625000000000000222, 0.9666666666666666741, 0.9708333333333333259, 0.9749999999999999778, 0.9791666666666666297, 0.9833333333333332815, 0.9875000000000000444, 0.9916666666666666963, 0.9958333333333333481, 1.000000000000000000 ),
 .UNSPECIFIED. ) 
 CURVE ( )  GEOMETRIC_REPRESENTATION_ITEM ( )  RATIONAL_B_SPLINE_CURVE ( ( 1.000000000000000000, 0.9238795325112867385, 1.000000000000000000, 0.9238795325112867385, 1.000000000000000000, 0.9238795325112867385, 1.000000000000000000, 0.9238795325112867385, 1.000000000000000000, 0.9238795325112867385, 1.000000000000000000, 0.9238795325112867385, 1.000000000000000000, 0.9238795325112867385, 1.000000000000000000, 0.9238795325112867385, 1.000000000000000000, 0.9238795325112867385, 1.000000000000000000, 0.9238795325112867385, 1.000000000000000000, 0.9238795325112867385, 1.000000000000000000, 0.9238795325112867385, 1.000000000000000000, 0.9238795325112867385, 1.000000000000000000, 0.9238795325112867385, 1.000000000000000000, 0.9238795325112867385, 1.000000000000000000, 0.9238795325112867385, 1.000000000000000000, 0.9238795325112867385, 1.000000000000000000, 0.9238795325112867385, 1.000000000000000000, 0.9238795325112867385, 1.000000000000000000, 0.9238795325112867385, 1.000000000000000000, 0.9238795325112867385, 1.000000000000000000, 0.9238795325112867385, 1.000000000000000000, 0.9238795325112867385, 1.000000000000000000, 0.9238795325112867385, 1.000000000000000000, 0.9238795325112867385, 1.000000000000000000, 0.9238795325112867385, 1.000000000000000000, 0.9238795325112867385, 1.000000000000000000, 0.9238795325112867385, 1.000000000000000000, 0.9238795325112867385, 1.000000000000000000, 0.9238795325112867385, 1.000000000000000000, 0.9238795325112867385, 1.000000000000000000, 0.9238795325112867385, 1.000000000000000000, 0.9238795325112867385, 1.000000000000000000, 0.9238795325112867385, 1.000000000000000000, 0.9238795325112867385, 1.000000000000000000, 0.9238795325112867385, 1.000000000000000000, 0.9238795325112867385, 1.000000000000000000, 0.9238795325112867385, 1.000000000000000000, 0.9238795325112867385, 1.000000000000000000, 0.9238795325112867385, 1.000000000000000000, 0.9238795325112867385, 1.000000000000000000, 0.9238795325112867385, 1.000000000000000000, 0.9238795325112867385, 1.000000000000000000, 0.9238795325112867385, 1.000000000000000000, 0.9238795325112867385, 1.000000000000000000, 0.9238795325112867385, 1.000000000000000000, 0.9238795325112867385, 1.000000000000000000, 0.9238795325112867385, 1.000000000000000000, 0.9238795325112867385, 1.000000000000000000, 0.9238795325112867385, 1.000000000000000000, 0.9238795325112867385, 1.000000000000000000, 0.9238795325112867385, 1.000000000000000000, 0.9238795325112867385, 1.000000000000000000, 0.9238795325112867385, 1.000000000000000000, 0.9238795325112867385, 1.000000000000000000, 0.9238795325112867385, 1.000000000000000000, 0.9238795325112867385, 1.000000000000000000, 0.9238795325112867385, 1.000000000000000000, 0.9238795325112867385, 1.000000000000000000, 0.9238795325112867385, 1.000000000000000000, 0.9238795325112867385, 1.000000000000000000, 0.9238795325112867385, 1.000000000000000000, 0.9238795325112867385, 1.000000000000000000, 0.9238795325112867385, 1.000000000000000000, 0.9238795325112867385, 1.000000000000000000, 0.9238795325112867385, 1.000000000000000000, 0.9238795325112867385, 1.000000000000000000, 0.9238795325112867385, 1.000000000000000000, 0.9238795325112867385, 1.000000000000000000, 0.9238795325112867385, 1.000000000000000000, 0.9238795325112867385, 1.000000000000000000, 0.9238795325112867385, 1.000000000000000000, 0.9238795325112867385, 1.000000000000000000, 0.9238795325112867385, 1.000000000000000000, 0.9238795325112867385, 1.000000000000000000, 0.9238795325112867385, 1.000000000000000000, 0.9238795325112867385, 1.000000000000000000, 0.9238795325112867385, 1.000000000000000000, 0.9238795325112867385, 1.000000000000000000, 0.9238795325112867385, 1.000000000000000000, 0.9238795325112867385, 1.000000000000000000, 0.9238795325112867385, 1.000000000000000000, 0.9238795325112867385, 1.000000000000000000, 0.9238795325112867385, 1.000000000000000000, 0.9238795325112867385, 1.000000000000000000, 0.9238795325112867385, 1.000000000000000000, 0.9238795325112867385, 1.000000000000000000, 0.9238795325112867385, 1.000000000000000000, 0.9238795325112867385, 1.000000000000000000, 0.9238795325112867385, 1.000000000000000000, 0.9238795325112867385, 1.000000000000000000, 0.9238795325112867385, 1.000000000000000000, 0.9238795325112867385, 1.000000000000000000, 0.9238795325112867385, 1.000000000000000000, 0.9238795325112867385, 1.000000000000000000, 0.9238795325112867385, 1.000000000000000000, 0.9238795325112867385, 1.000000000000000000, 0.9238795325112867385, 1.000000000000000000, 0.9238795325112867385, 1.000000000000000000, 0.9238795325112867385, 1.000000000000000000, 0.9238795325112867385, 1.000000000000000000, 0.9238795325112867385, 1.000000000000000000, 0.9238795325112867385, 1.000000000000000000, 0.9238795325112867385, 1.000000000000000000, 0.9238795325112867385, 1.000000000000000000, 0.9238795325112867385, 1.000000000000000000, 0.9238795325112867385, 1.000000000000000000, 0.9238795325112867385, 1.000000000000000000, 0.9238795325112867385, 1.000000000000000000, 0.9238795325112867385, 1.000000000000000000, 0.9238795325112867385, 1.000000000000000000, 0.9238795325112867385, 1.000000000000000000, 0.9238795325112867385, 1.000000000000000000, 0.9238795325112867385, 1.000000000000000000, 0.9238795325112867385, 1.000000000000000000, 0.9238795325112867385, 1.000000000000000000, 0.9238795325112867385, 1.000000000000000000, 0.9238795325112867385, 1.000000000000000000, 0.9238795325112867385, 1.000000000000000000, 0.9238795325112867385, 1.000000000000000000, 0.9238795325112867385, 1.000000000000000000, 0.9238795325112867385, 1.000000000000000000, 0.9238795325112867385, 1.000000000000000000, 0.9238795325112867385, 1.000000000000000000, 0.9238795325112867385, 1.000000000000000000, 0.9238795325112867385, 1.000000000000000000, 0.9238795325112867385, 1.000000000000000000, 0.9238795325112867385, 1.000000000000000000, 0.9238795325112867385, 1.000000000000000000, 0.9238795325112867385, 1.000000000000000000, 0.9238795325112867385, 1.000000000000000000, 0.9238795325112867385, 1.000000000000000000, 0.9238795325112867385, 1.000000000000000000, 0.9238795325112867385, 1.000000000000000000, 0.9238795325112867385, 1.000000000000000000, 0.9238795325112867385, 1.000000000000000000, 0.9238795325112867385, 1.000000000000000000, 0.9238795325112867385, 1.000000000000000000, 0.9238795325112867385, 1.000000000000000000, 0.9238795325112867385, 1.000000000000000000, 0.9238795325112867385, 1.000000000000000000, 0.9238795325112867385, 1.000000000000000000, 0.9238795325112867385, 1.000000000000000000, 0.9238795325112867385, 1.000000000000000000, 0.9238795325112867385, 1.000000000000000000, 0.9238795325112867385, 1.000000000000000000, 0.9238795325112867385, 1.000000000000000000, 0.9238795325112867385, 1.000000000000000000, 0.9238795325112867385, 1.000000000000000000, 0.9238795325112867385, 1.000000000000000000, 0.9238795325112867385, 1.000000000000000000, 0.9238795325112867385, 1.000000000000000000, 0.9238795325112867385, 1.000000000000000000, 0.9238795325112867385, 1.000000000000000000, 0.9238795325112867385, 1.000000000000000000, 0.9238795325112867385, 1.000000000000000000, 0.9238795325112867385, 1.000000000000000000, 0.9238795325112867385, 1.000000000000000000, 0.9238795325112867385, 1.000000000000000000, 0.9238795325112867385, 1.000000000000000000, 0.9238795325112867385, 1.000000000000000000, 0.9238795325112867385, 1.000000000000000000, 0.9238795325112867385, 1.000000000000000000, 0.9238795325112867385, 1.000000000000000000, 0.9238795325112867385, 1.000000000000000000, 0.9238795325112867385, 1.000000000000000000, 0.9238795325112867385, 1.000000000000000000, 0.9238795325112867385, 1.000000000000000000, 0.9238795325112867385, 1.000000000000000000, 0.9238795325112867385, 1.000000000000000000, 0.9238795325112867385, 1.000000000000000000, 0.9238795325112867385, 1.000000000000000000, 0.9238795325112867385, 1.000000000000000000, 0.9238795325112867385, 1.000000000000000000, 0.9238795325112867385, 1.000000000000000000, 0.9238795325112867385, 1.000000000000000000, 0.9238795325112867385, 1.000000000000000000, 0.9238795325112867385, 1.000000000000000000, 0.9238795325112867385, 1.000000000000000000, 0.9238795325112867385, 1.000000000000000000, 0.9238795325112867385, 1.000000000000000000, 0.9238795325112867385, 1.000000000000000000, 0.9238795325112867385, 1.000000000000000000, 0.9238795325112867385, 1.000000000000000000, 0.9238795325112867385, 1.000000000000000000, 0.9238795325112867385, 1.000000000000000000, 0.9238795325112867385, 1.000000000000000000, 0.9238795325112867385, 1.000000000000000000, 0.9238795325112867385, 1.000000000000000000, 0.9238795325112867385, 1.000000000000000000, 0.9238795325112867385, 1.000000000000000000, 0.9238795325112867385, 1.000000000000000000, 0.9238795325112867385, 1.000000000000000000, 0.9238795325112867385, 1.000000000000000000, 0.9238795325112867385, 1.000000000000000000, 0.9238795325112867385, 1.000000000000000000, 0.9238795325112867385, 1.000000000000000000, 0.9238795325112867385, 1.000000000000000000, 0.9238795325112867385, 1.000000000000000000, 0.9238795325112867385, 1.000000000000000000, 0.9238795325112867385, 1.000000000000000000, 0.9238795325112867385, 1.000000000000000000, 0.9238795325112867385, 1.000000000000000000, 0.9238795325112867385, 1.000000000000000000, 0.9238795325112867385, 1.000000000000000000, 0.9238795325112867385, 1.000000000000000000, 0.9238795325112867385, 1.000000000000000000, 0.9238795325112867385, 1.000000000000000000, 0.9238795325112867385, 1.000000000000000000, 0.9238795325112867385, 1.000000000000000000, 0.9238795325112867385, 1.000000000000000000, 0.9238795325112867385, 1.000000000000000000, 0.9238795325112867385, 1.000000000000000000, 0.9238795325112867385, 1.000000000000000000, 0.9238795325112867385, 1.000000000000000000, 0.9238795325112867385, 1.000000000000000000, 0.9238795325112867385, 1.000000000000000000, 0.9238795325112867385, 1.000000000000000000, 0.9238795325112867385, 1.000000000000000000, 0.9238795325112867385, 1.000000000000000000, 0.9238795325112867385, 1.000000000000000000, 0.9238795325112867385, 1.000000000000000000, 0.9238795325112867385, 1.000000000000000000, 0.9238795325112867385, 1.000000000000000000, 0.9238795325112867385, 1.000000000000000000, 0.9238795325112867385, 1.000000000000000000, 0.9238795325112867385, 1.000000000000000000, 0.9238795325112867385, 1.000000000000000000, 0.9238795325112867385, 1.000000000000000000, 0.9238795325112867385, 1.000000000000000000, 0.9238795325112867385, 1.000000000000000000, 0.9238795325112867385, 1.000000000000000000, 0.9238795325112867385, 1.000000000000000000, 0.9238795325112867385, 1.000000000000000000, 0.9238795325112867385, 1.000000000000000000, 0.9238795325112867385, 1.000000000000000000, 0.9238795325112867385, 1.000000000000000000, 0.9238795325112867385, 1.000000000000000000, 0.9238795325112867385, 1.000000000000000000, 0.9238795325112867385, 1.000000000000000000 ) ) 
 REPRESENTATION_ITEM ( '' )  );
#26530=CARTESIAN_POINT ( 'NONE',  ( 5.000000000000000000, -169.1250000027312126, 0.000000000000000000 ) ) ;
#26537=CARTESIAN_POINT ( 'NONE',  ( -2.499999999999996447, -4.708333330602147981, 4.330127018922195425 ) ) ;
#26540=CARTESIAN_POINT ( 'NONE',  ( -3.535533905932738641, -157.5000000027312126, 3.535533905932737309 ) ) ;
#26541=VERTEX_POINT ( 'NONE', #36027 ) ;
#26551=CARTESIAN_POINT ( 'NONE',  ( -4.458734124999999437, -27.31249999863440081, 0.000000000000000000 ) ) ;
#26552=CARTESIAN_POINT ( 'NONE',  ( -9.184850993605147944E-16, -147.2500000000000284, 5.000000000000000000 ) ) ;
#26553=CARTESIAN_POINT ( 'NONE',  ( -5.000000000000000888, -151.4375000000000000, 2.071067811865474617 ) ) ;
#26555=CARTESIAN_POINT ( 'NONE',  ( 3.152801135295366208, -152.5625000013655779, 3.152801135295367985 ) ) ;
#26556=VERTEX_POINT ( 'NONE', #21233 ) ;
#26557=CARTESIAN_POINT ( 'NONE',  ( 2.229367062499998831, -52.89583333196773651, -3.861377020970580887 ) ) ;
#26561=CARTESIAN_POINT ( 'NONE',  ( -5.000000000000000000, 21.91666666666666785, -2.886751345948128211 ) ) ;
#26564=CARTESIAN_POINT ( 'NONE',  ( 4.458734124999998549, 6.270833334698928674, -2.574251347313721627 ) ) ;
#26565=DIRECTION ( 'NONE',  ( -1.000000000000000000, 0.000000000000000000, 0.000000000000000000 ) ) ;
#26566=CARTESIAN_POINT ( 'NONE',  ( -5.000000000000000000, 29.56250000136559208, 0.000000000000000000 ) ) ;
#26567=CARTESIAN_POINT ( 'NONE',  ( 5.000000000000000888, -7.583333333333330373, 2.886751345948126879 ) ) ;
#26568=CARTESIAN_POINT ( 'NONE',  ( 4.458734125000001214, 16.85416666803225638, 2.574251347313718519 ) ) ;
#26569=AXIS2_PLACEMENT_3D ( 'NONE', #60155, #35702, #658 ) ;
#26570=CARTESIAN_POINT ( 'NONE',  ( 5.000000000000000000, 3.708333336064517205, -2.886751345948129988 ) ) ;
#26571=ORIENTED_EDGE ( 'NONE', *, *, #51583, .F. ) ;
#26572=CARTESIAN_POINT ( 'NONE',  ( -6.972266317189433020E-16, -42.24999999999998579, -5.000000000000000000 ) ) ;
#26575=CARTESIAN_POINT ( 'NONE',  ( -2.229367062500000163, -43.47916666530106511, -3.861377020970580443 ) ) ;
#26576=CARTESIAN_POINT ( 'NONE',  ( -4.458734125000000326, -165.2500000013655779, -1.846868145590735644 ) ) ;
#26577=CARTESIAN_POINT ( 'NONE',  ( -2.499999999999996447, -42.70833333060214443, 4.330127018922195425 ) ) ;
#26578=ORIENTED_EDGE ( 'NONE', *, *, #38048, .F. ) ;
#26579=CARTESIAN_POINT ( 'NONE',  ( 4.458734124999998549, -18.72916666530106866, -2.574251347313721627 ) ) ;
#26581=CARTESIAN_POINT ( 'NONE',  ( 5.000000000000000000, -89.50000000000000000, -6.123233995736766282E-16 ) ) ;
#26582=CARTESIAN_POINT ( 'NONE',  ( 3.152801135295366208, -163.5625000013656063, 3.152801135295367985 ) ) ;
#26587=VECTOR ( 'NONE', #39215, 1000.000000000000000 ) ;
#26588=CARTESIAN_POINT ( 'NONE',  ( 4.458734125000001214, -30.14583333196773296, 2.574251347313718519 ) ) ;
#26589=CARTESIAN_POINT ( 'NONE',  ( -2.499999999999996447, -38.83333333333332860, 4.330127018922195425 ) ) ;
#26598=CARTESIAN_POINT ( 'NONE',  ( 9.457646018065525792E-16, -79.31249999863439371, 5.148502694627439702 ) ) ;
#26601=CARTESIAN_POINT ( 'NONE',  ( 4.458734124999999437, -140.6875000013656063, 0.000000000000000000 ) ) ;
#26604=CARTESIAN_POINT ( 'NONE',  ( -2.229367062499996610, -46.14583333196774362, 3.861377020970582219 ) ) ;
#26611=CARTESIAN_POINT ( 'NONE',  ( -4.458734124999999437, -77.56249999863440792, 0.000000000000000000 ) ) ;
#26617=DIRECTION ( 'NONE',  ( -0.000000000000000000, 1.000000000000000000, -0.000000000000000000 ) ) ;
#26620=CARTESIAN_POINT ( 'NONE',  ( 4.458734124999998549, 12.02083333469892601, -2.574251347313721627 ) ) ;
#26626=CARTESIAN_POINT ( 'NONE',  ( -2.500000000000000444, -16.04166666393548368, -4.330127018922193649 ) ) ;
#26627=CARTESIAN_POINT ( 'NONE',  ( -4.458734124999999437, -86.39583333196772230, -2.574251347313719407 ) ) ;
#26628=CARTESIAN_POINT ( 'NONE',  ( 2.229367062499998831, -8.645833331967736513, -3.861377020970580887 ) ) ;
#26630=ORIENTED_EDGE ( 'NONE', *, *, #26912, .T. ) ;
#26631=CARTESIAN_POINT ( 'NONE',  ( 4.458734124999998549, -37.97916666530107221, -2.574251347313721627 ) ) ;
#26632=VECTOR ( 'NONE', #61568, 1000.000000000000000 ) ;
#26636=VECTOR ( 'NONE', #8247, 1000.000000000000000 ) ;
#26638=CARTESIAN_POINT ( 'NONE',  ( 4.458734125000001214, 18.10416666803225638, 2.574251347313718519 ) ) ;
#26639=CARTESIAN_POINT ( 'NONE',  ( -2.500000000000000444, -44.04166666393546592, -4.330127018922193649 ) ) ;
#26640=CARTESIAN_POINT ( 'NONE',  ( -2.071067811865562991, -145.4375000027312126, 4.999999999999913847 ) ) ;
#26641=CARTESIAN_POINT ( 'NONE',  ( 4.458734125000000326, -79.14583333196773651, 2.574251347313718519 ) ) ;
#26643=CARTESIAN_POINT ( 'NONE',  ( 1.975475456537005874E-15, -72.62499999726878741, 5.000000000000000000 ) ) ;
#26644=CARTESIAN_POINT ( 'NONE',  ( -3.535250795749689387E-16, 17.87500000273118417, -5.773502691896257311 ) ) ;
#26646=DIRECTION ( 'NONE',  ( -0.000000000000000000, 1.000000000000000000, -0.000000000000000000 ) ) ;
#26648=CARTESIAN_POINT ( 'NONE',  ( 0.000000000000000000, -170.0000000000000000, 5.000000000000000000 ) ) ;
#26649=CARTESIAN_POINT ( 'NONE',  ( -5.000000000000000000, -22.08333333333333215, -2.886751345948128211 ) ) ;
#26650=CARTESIAN_POINT ( 'NONE',  ( 4.458734125000001214, -27.89583333196774007, 2.574251347313718519 ) ) ;
#26652=CARTESIAN_POINT ( 'NONE',  ( -3.152548672688508926E-16, -85.56249999863439371, -5.148502694627439702 ) ) ;
#26653=( BOUNDED_CURVE ( )  B_SPLINE_CURVE ( 2, ( #52329, #8264, #16960, #3439, #36572, #62921, #48732, #190, #48114 ),
 .UNSPECIFIED., .F., .F. ) 
 B_SPLINE_CURVE_WITH_KNOTS ( ( 3, 2, 2, 2, 3 ),
 ( 0.6229166666666666741, 0.6236111111111111160, 0.6250000000000000000, 0.6263888888888888840, 0.6270833333333333259 ),
 .UNSPECIFIED. ) 
 CURVE ( )  GEOMETRIC_REPRESENTATION_ITEM ( )  RATIONAL_B_SPLINE_CURVE ( ( 0.9330127018922194093, 0.9330127018922194093, 1.000000000000000000, 0.8660254037844387076, 1.000000000000000000, 0.8660254037844387076, 1.000000000000000000, 0.9330127018922194093, 0.9330127018922194093 ) ) 
 REPRESENTATION_ITEM ( '' )  );
#26654=CARTESIAN_POINT ( 'NONE',  ( -2.500000000000000444, -28.04166666393548013, -4.330127018922193649 ) ) ;
#26655=CARTESIAN_POINT ( 'NONE',  ( -4.458734124999998549, -55.22916666530107932, 2.574251347313722516 ) ) ;
#26656=ORIENTED_EDGE ( 'NONE', *, *, #41340, .T. ) ;
#26659=CARTESIAN_POINT ( 'NONE',  ( -4.458734124999999437, -5.562499998634402587, 0.000000000000000000 ) ) ;
#26661=CARTESIAN_POINT ( 'NONE',  ( -5.000000000000000000, -69.99999999999998579, 0.000000000000000000 ) ) ;
#26664=DIRECTION ( 'NONE',  ( -0.000000000000000000, 1.000000000000000000, -0.000000000000000000 ) ) ;
#26665=CARTESIAN_POINT ( 'NONE',  ( -5.000000000000000000, -68.95833333060214443, -2.886751345948128211 ) ) ;
#26666=CARTESIAN_POINT ( 'NONE',  ( 1.975475456537005874E-15, -10.62499999726881228, 5.000000000000000000 ) ) ;
#26668=CARTESIAN_POINT ( 'NONE',  ( 4.458734124999998549, -13.97916666530107221, -2.574251347313721627 ) ) ;
#26669=CARTESIAN_POINT ( 'NONE',  ( 2.229367062500001939, -54.22916666530107221, 3.861377020970579999 ) ) ;
#26672=CARTESIAN_POINT ( 'NONE',  ( 3.152801135295366208, -140.5625000013655779, 3.152801135295367985 ) ) ;
#26675=DIRECTION ( 'NONE',  ( -0.000000000000000000, 1.000000000000000000, -0.000000000000000000 ) ) ;
#26677=CARTESIAN_POINT ( 'NONE',  ( -5.000000000000000888, -155.4375000000000000, 2.071067811865474617 ) ) ;
#26678=CARTESIAN_POINT ( 'NONE',  ( 2.229367062500001939, 23.77083333469892779, 3.861377020970579999 ) ) ;
#26681=DIRECTION ( 'NONE',  ( -0.000000000000000000, 1.000000000000000000, -0.000000000000000000 ) ) ;
#26683=ADVANCED_FACE ( 'NONE', ( #61752 ), #51148, .T. ) ;
#26686=CARTESIAN_POINT ( 'NONE',  ( 1.846868145590736310, -149.8750000013655779, 4.458734124999999437 ) ) ;
#26688=LINE ( 'NONE', #8338, #39610 ) ;
#26689=CARTESIAN_POINT ( 'NONE',  ( 4.458734124999999437, -65.06249999863440792, -5.460374474430324690E-16 ) ) ;
#26692=CARTESIAN_POINT ( 'NONE',  ( -3.152801135295367096, -144.0625000013655779, -3.152801135295367541 ) ) ;
#26694=ORIENTED_EDGE ( 'NONE', *, *, #9347, .T. ) ;
#26699=CARTESIAN_POINT ( 'NONE',  ( 4.458734124999999437, 28.93750000136559208, -5.460374474430324690E-16 ) ) ;
#26700=CARTESIAN_POINT ( 'NONE',  ( 2.500000000000002220, -88.54166666393548724, 4.330127018922192761 ) ) ;
#26708=CARTESIAN_POINT ( 'NONE',  ( -4.458734124999999437, 14.68750000136559386, 0.000000000000000000 ) ) ;
#26710=CARTESIAN_POINT ( 'NONE',  ( -2.229367062499996610, -18.39583333196774007, 3.861377020970582219 ) ) ;
#26711=( BOUNDED_CURVE ( )  B_SPLINE_CURVE ( 2, ( #9684, #34130, #4870, #54400, #59, #39905, #39268, #373, #29292 ),
 .UNSPECIFIED., .F., .F. ) 
 B_SPLINE_CURVE_WITH_KNOTS ( ( 3, 2, 2, 2, 3 ),
 ( 0.6354166666666666297, 0.6361111111111110716, 0.6374999999999999556, 0.6388888888888888395, 0.6395833333333332815 ),
 .UNSPECIFIED. ) 
 CURVE ( )  GEOMETRIC_REPRESENTATION_ITEM ( )  RATIONAL_B_SPLINE_CURVE ( ( 0.9330127018922194093, 0.9330127018922194093, 1.000000000000000000, 0.8660254037844387076, 1.000000000000000000, 0.8660254037844387076, 1.000000000000000000, 0.9330127018922194093, 0.9330127018922194093 ) ) 
 REPRESENTATION_ITEM ( '' )  );
#26713=CARTESIAN_POINT ( 'NONE',  ( 2.730187237215162345E-16, -161.1875000013655779, -4.458734124999999437 ) ) ;
#26717=CARTESIAN_POINT ( 'NONE',  ( 3.061616997868383141E-16, -161.8750000027311842, -5.000000000000000000 ) ) ;
#26719=CARTESIAN_POINT ( 'NONE',  ( 2.229367062499998831, -36.64583333196773651, -3.861377020970580887 ) ) ;
#26723=CARTESIAN_POINT ( 'NONE',  ( 1.339745962155612702, -36.16965819600732601, -5.000000000000000000 ) ) ;
#26724=VERTEX_POINT ( 'NONE', #57245 ) ;
#26727=CARTESIAN_POINT ( 'NONE',  ( 1.975475456537005874E-15, -67.62499999726881583, 5.000000000000000000 ) ) ;
#26728=CARTESIAN_POINT ( 'NONE',  ( 1.060575238724906964E-15, -8.750000000000000000, 5.773502691896257311 ) ) ;
#26730=EDGE_CURVE ( 'NONE', #61537, #14751, #49181, .T. ) ;
#26731=CARTESIAN_POINT ( 'NONE',  ( 2.229367062499998831, -74.64583333196773651, -3.861377020970580887 ) ) ;
#26732=CARTESIAN_POINT ( 'NONE',  ( 5.000000000000000000, -22.37499999726881228, -6.123233995736766282E-16 ) ) ;
#26733=CARTESIAN_POINT ( 'NONE',  ( 5.000000000000000888, -6.458333330602148870, 2.886751345948126879 ) ) ;
#26734=CARTESIAN_POINT ( 'NONE',  ( 4.458734125000001214, -37.89583333196772941, 2.574251347313718519 ) ) ;
#26735=EDGE_LOOP ( 'NONE', ( #11148, #34541, #41281, #32747 ) ) ;
#26737=CARTESIAN_POINT ( 'NONE',  ( 9.457646018065525792E-16, 12.68750000136559208, 5.148502694627439702 ) ) ;
#26738=ORIENTED_EDGE ( 'NONE', *, *, #37339, .F. ) ;
#26739=DIRECTION ( 'NONE',  ( -0.000000000000000000, 1.000000000000000000, -0.000000000000000000 ) ) ;
#26740=CARTESIAN_POINT ( 'NONE',  ( -5.000000000000000000, -56.08333333333332860, -2.886751345948128211 ) ) ;
#26741=CARTESIAN_POINT ( 'NONE',  ( 4.458734124999999437, -159.7500000013656063, 1.846868145590737864 ) ) ;
#26743=CARTESIAN_POINT ( 'NONE',  ( -2.500000000000000444, -35.16666666666666430, -4.330127018922193649 ) ) ;
#26744=CARTESIAN_POINT ( 'NONE',  ( 4.458734124999998549, -82.72916666530106511, -2.574251347313721627 ) ) ;
#26745=CARTESIAN_POINT ( 'NONE',  ( 2.071067811865475505, -169.8125000000000000, -5.000000000000000888 ) ) ;
#26746=CARTESIAN_POINT ( 'NONE',  ( 2.229367062499998831, -85.64583333196773651, -3.861377020970580887 ) ) ;
#26748=CARTESIAN_POINT ( 'NONE',  ( -2.229367062499996610, -33.39583333196772941, 3.861377020970582219 ) ) ;
#26750=VERTEX_POINT ( 'NONE', #31503 ) ;
#26751=EDGE_CURVE ( 'NONE', #1132, #55402, #51653, .T. ) ;
#26758=CARTESIAN_POINT ( 'NONE',  ( 2.229367062500001939, -63.22916666530106511, 3.861377020970579999 ) ) ;
#26764=CARTESIAN_POINT ( 'NONE',  ( 2.229367062499998831, 9.354166668032261711, -3.861377020970580887 ) ) ;
#26766=CARTESIAN_POINT ( 'NONE',  ( 4.458734124999999437, -158.3750000013655779, -1.846868145590734978 ) ) ;
#26767=CARTESIAN_POINT ( 'NONE',  ( -1.339745962155613812, 18.91965820146970501, -5.000000000000000000 ) ) ;
#26768=ORIENTED_EDGE ( 'NONE', *, *, #26730, .F. ) ;
#26772=ADVANCED_FACE ( 'NONE', ( #36983 ), #8348, .T. ) ;
#26775=CARTESIAN_POINT ( 'NONE',  ( 5.000000000000000000, -78.50000000000000000, -6.123233995736766282E-16 ) ) ;
#26778=CARTESIAN_POINT ( 'NONE',  ( -4.458734124999997661, 28.77083333469892779, 2.574251347313722516 ) ) ;
#26781=CARTESIAN_POINT ( 'NONE',  ( -4.458734124999999437, -0.6458333319677399542, -2.574251347313719407 ) ) ;
#26783=CARTESIAN_POINT ( 'NONE',  ( -3.535533905932737309, -144.7500000027311842, -3.535533905932738197 ) ) ;
#26792=CARTESIAN_POINT ( 'NONE',  ( -8.190561711645485556E-16, -161.9375000013655779, 4.458734124999999437 ) ) ;
#26795=CARTESIAN_POINT ( 'NONE',  ( -5.000000000000000000, -90.87499999726880162, 0.000000000000000000 ) ) ;
#26796=ORIENTED_EDGE ( 'NONE', *, *, #37716, .F. ) ;
#26797=CARTESIAN_POINT ( 'NONE',  ( -4.458734124999999437, 21.35416666803225993, -2.574251347313719407 ) ) ;
#26802=CARTESIAN_POINT ( 'NONE',  ( 5.000000000000000000, 9.499999999999998224, -6.123233995736766282E-16 ) ) ;
#26803=CARTESIAN_POINT ( 'NONE',  ( 9.457646018065525792E-16, -54.06249999863440081, 5.148502694627439702 ) ) ;
#26812=CARTESIAN_POINT ( 'NONE',  ( -3.535250795749689387E-16, -42.24999999999999289, -5.773502691896257311 ) ) ;
#26813=CARTESIAN_POINT ( 'NONE',  ( -5.000000000000000000, 13.04166666939785379, -2.886751345948128211 ) ) ;
#26817=CARTESIAN_POINT ( 'NONE',  ( -2.071067811865562991, -143.3124999999999716, 4.999999999999913847 ) ) ;
#26818=CARTESIAN_POINT ( 'NONE',  ( -4.458734124999999437, -61.39583333196774362, -2.574251347313719407 ) ) ;
#26819=CARTESIAN_POINT ( 'NONE',  ( -4.458734125000000326, -150.2500000013656063, -1.846868145590735644 ) ) ;
#26821=CARTESIAN_POINT ( 'NONE',  ( 2.229367062500001939, -72.97916666530107932, 3.861377020970579999 ) ) ;
#26825=CARTESIAN_POINT ( 'NONE',  ( -3.152548672688508926E-16, -18.81249999863440792, -5.148502694627439702 ) ) ;
#26826=CARTESIAN_POINT ( 'NONE',  ( 5.000000000000000000, -59.29166666393547303, -2.886751345948129988 ) ) ;
#26827=ORIENTED_EDGE ( 'NONE', *, *, #25920, .F. ) ;
#26828=CARTESIAN_POINT ( 'NONE',  ( 1.339745962155615144, -31.58034179853029499, 4.999999999999999112 ) ) ;
#26833=CARTESIAN_POINT ( 'NONE',  ( 4.458734125000000326, -152.3750000013655779, -1.846868145590734978 ) ) ;
#26836=ADVANCED_FACE ( 'NONE', ( #3835 ), #23453, .T. ) ;
#26837=EDGE_CURVE ( 'NONE', #35151, #29442, #58200, .T. ) ;
#26838=CARTESIAN_POINT ( 'NONE',  ( 5.000000000000000000, -54.41666666666667140, -2.886751345948130876 ) ) ;
#26840=CARTESIAN_POINT ( 'NONE',  ( -5.000000000000000000, -55.87499999726880162, 0.000000000000000000 ) ) ;
#26841=CARTESIAN_POINT ( 'NONE',  ( 4.458734125000001214, -50.14583333196773651, 2.574251347313718519 ) ) ;
#26843=( BOUNDED_CURVE ( )  B_SPLINE_CURVE ( 2, ( #43426, #62443, #38594, #9647, #57927, #37985, #62122, #13544, #28322 ),
 .UNSPECIFIED., .F., .F. ) 
 B_SPLINE_CURVE_WITH_KNOTS ( ( 3, 2, 2, 2, 3 ),
 ( 0.2604166666666666852, 0.2611111111111111271, 0.2625000000000000111, 0.2638888888888888951, 0.2645833333333333370 ),
 .UNSPECIFIED. ) 
 CURVE ( )  GEOMETRIC_REPRESENTATION_ITEM ( )  RATIONAL_B_SPLINE_CURVE ( ( 0.9330127018922194093, 0.9330127018922194093, 1.000000000000000000, 0.8660254037844387076, 1.000000000000000000, 0.8660254037844387076, 1.000000000000000000, 0.9330127018922194093, 0.9330127018922194093 ) ) 
 REPRESENTATION_ITEM ( '' )  );
#26846=CARTESIAN_POINT ( 'NONE',  ( 2.229367062500001939, 22.02083333469892779, 3.861377020970579999 ) ) ;
#26849=CARTESIAN_POINT ( 'NONE',  ( -8.190561711645485556E-16, -167.6875000013655779, 4.458734124999999437 ) ) ;
#26858=CARTESIAN_POINT ( 'NONE',  ( -5.147856630858197489E-14, 4.249999999999996447, 5.000000000000000000 ) ) ;
#26859=CARTESIAN_POINT ( 'NONE',  ( -6.972266317189433020E-16, -45.24999999999999289, -5.000000000000000000 ) ) ;
#26863=CARTESIAN_POINT ( 'NONE',  ( -4.999999999999998224, -4.791666663935479242, 2.886751345948131764 ) ) ;
#26865=CARTESIAN_POINT ( 'NONE',  ( -5.000000000000000888, -158.5625000027312126, 2.071067811865474617 ) ) ;
#26868=VECTOR ( 'NONE', #26171, 1000.000000000000000 ) ;
#26872=CARTESIAN_POINT ( 'NONE',  ( -5.000000000000000888, -147.5625000000000284, -2.071067811865475949 ) ) ;
#26876=CARTESIAN_POINT ( 'NONE',  ( 4.458734124999998549, -23.72916666530107577, -2.574251347313721627 ) ) ;
#26877=CARTESIAN_POINT ( 'NONE',  ( 2.071067811865476394, -150.1874999999999716, 5.000000000000000000 ) ) ;
#26879=CARTESIAN_POINT ( 'NONE',  ( 2.730187237215162345E-16, -152.1875000013656063, -4.458734124999999437 ) ) ;
#26880=ORIENTED_EDGE ( 'NONE', *, *, #27013, .T. ) ;
#26881=CYLINDRICAL_SURFACE ( 'NONE', #4042, 5.000000000000000000 ) ;
#26882=CARTESIAN_POINT ( 'NONE',  ( 4.458734124999998549, -49.97916666530106511, -2.574251347313721627 ) ) ;
#26883=CARTESIAN_POINT ( 'NONE',  ( 2.499999999999998668, -58.20833333060214443, -4.330127018922193649 ) ) ;
#26885=CARTESIAN_POINT ( 'NONE',  ( -2.499999999999996447, 24.16666666666666785, 4.330127018922195425 ) ) ;
#26887=CARTESIAN_POINT ( 'NONE',  ( 2.229367062499998831, 6.354166668032262599, -3.861377020970580887 ) ) ;
#26889=CARTESIAN_POINT ( 'NONE',  ( 5.000000000000000000, -11.37499999726881583, -6.123233995736766282E-16 ) ) ;
#26890=DIRECTION ( 'NONE',  ( -0.000000000000000000, 1.000000000000000000, -0.000000000000000000 ) ) ;
#26891=CARTESIAN_POINT ( 'NONE',  ( -2.229367062499996610, 16.60416666803225638, 3.861377020970582219 ) ) ;
#26892=CARTESIAN_POINT ( 'NONE',  ( -5.000000000000000000, 2.041666669397854239, -2.886751345948128211 ) ) ;
#26894=CARTESIAN_POINT ( 'NONE',  ( 2.499999999999998668, 26.66666666666666430, -4.330127018922193649 ) ) ;
#26895=VERTEX_POINT ( 'NONE', #58165 ) ;
#26896=CARTESIAN_POINT ( 'NONE',  ( -1.339745962155610925, -23.66965819600732956, 5.000000000000000000 ) ) ;
#26897=CARTESIAN_POINT ( 'NONE',  ( -2.229367062500000163, -44.47916666530106511, -3.861377020970580443 ) ) ;
#26898=CARTESIAN_POINT ( 'NONE',  ( -1.846868145590737420, -164.0000000013656063, 4.458734124999999437 ) ) ;
#26899=CARTESIAN_POINT ( 'NONE',  ( 2.500000000000002220, -42.54166666393548013, 4.330127018922192761 ) ) ;
#26901=CARTESIAN_POINT ( 'NONE',  ( 2.229367062499998831, -19.64583333196774007, -3.861377020970580887 ) ) ;
#26902=ORIENTED_EDGE ( 'NONE', *, *, #31803, .F. ) ;
#26903=CARTESIAN_POINT ( 'NONE',  ( 5.000000000000000000, -87.41666666666667140, -2.886751345948129988 ) ) ;
#26904=CARTESIAN_POINT ( 'NONE',  ( -4.458734124999999437, -165.9375000013655779, -5.460374474430324690E-16 ) ) ;
#26906=CARTESIAN_POINT ( 'NONE',  ( -4.999999999999998224, -60.79166666393547303, 2.886751345948131764 ) ) ;
#26909=CARTESIAN_POINT ( 'NONE',  ( 4.458734125000001214, -31.14583333196773651, 2.574251347313718519 ) ) ;
#26911=ORIENTED_EDGE ( 'NONE', *, *, #60368, .T. ) ;
#26912=EDGE_CURVE ( 'NONE', #9066, #13678, #55779, .T. ) ;
#26916=CARTESIAN_POINT ( 'NONE',  ( 2.499999999999998668, 24.79166666939785202, -4.330127018922193649 ) ) ;
#26921=CARTESIAN_POINT ( 'NONE',  ( -4.458734124999999437, -82.56249999863440792, 0.000000000000000000 ) ) ;
#26924=CARTESIAN_POINT ( 'NONE',  ( -1.339745962155613812, 5.919658201469705894, -5.000000000000000000 ) ) ;
#26926=CARTESIAN_POINT ( 'NONE',  ( 2.229367062500001939, -44.97916666530106511, 3.861377020970579999 ) ) ;
#26929=CYLINDRICAL_SURFACE ( 'NONE', #22738, 5.000000000000000000 ) ;
#26933=CARTESIAN_POINT ( 'NONE',  ( 0.000000000000000000, -170.0000000000000000, 0.000000000000000000 ) ) ;
#26934=CARTESIAN_POINT ( 'NONE',  ( 9.457646018065525792E-16, -79.31249999863439371, 5.148502694627439702 ) ) ;
#26943=CARTESIAN_POINT ( 'NONE',  ( -5.000000000000000888, -167.5625000027312126, 2.071067811865474617 ) ) ;
#26945=CARTESIAN_POINT ( 'NONE',  ( -4.458734124999997661, 13.52083333469892779, 2.574251347313722516 ) ) ;
#26951=CARTESIAN_POINT ( 'NONE',  ( 2.500000000000002220, -38.54166666393548013, 4.330127018922192761 ) ) ;
#26952=CARTESIAN_POINT ( 'NONE',  ( -4.458734124999999437, -85.39583333196773651, -2.574251347313719407 ) ) ;
#26953=CARTESIAN_POINT ( 'NONE',  ( -3.152548672688508926E-16, -7.562499998634404363, -5.148502694627439702 ) ) ;
#26954=ORIENTED_EDGE ( 'NONE', *, *, #8682, .T. ) ;
#26955=CARTESIAN_POINT ( 'NONE',  ( -3.152548672688508926E-16, -33.81249999863440792, -5.148502694627439702 ) ) ;
#26959=CARTESIAN_POINT ( 'NONE',  ( 1.846868145590735200, -150.5000000013656347, -4.458734124999999437 ) ) ;
#26960=CARTESIAN_POINT ( 'NONE',  ( -2.229367062499996610, 22.85416666803225993, 3.861377020970582219 ) ) ;
#26963=CARTESIAN_POINT ( 'NONE',  ( -4.458734124999997661, -83.47916666530106511, 2.574251347313722516 ) ) ;
#26966=CARTESIAN_POINT ( 'NONE',  ( 5.000000000000000888, 17.54166666939785557, 2.886751345948126879 ) ) ;
#26970=CARTESIAN_POINT ( 'NONE',  ( 5.000000000000000888, -22.58333333333333215, 2.886751345948126879 ) ) ;
#26971=CARTESIAN_POINT ( 'NONE',  ( 4.458734124999999437, -27.81249999863440081, -5.460374474430324690E-16 ) ) ;
#26972=CARTESIAN_POINT ( 'NONE',  ( -4.458734124999999437, -88.31249999863439371, 0.000000000000000000 ) ) ;
#26973=CARTESIAN_POINT ( 'NONE',  ( -5.000000000000000000, -27.95833333060214798, -2.886751345948128211 ) ) ;
#26974=CARTESIAN_POINT ( 'NONE',  ( 9.457646018065525792E-16, -56.06249999863440792, 5.148502694627439702 ) ) ;
#26977=CARTESIAN_POINT ( 'NONE',  ( -4.458734124999999437, -9.645833331967738289, -2.574251347313719407 ) ) ;
#26978=ORIENTED_EDGE ( 'NONE', *, *, #8824, .T. ) ;
#26979=CARTESIAN_POINT ( 'NONE',  ( 2.499999999999998668, -71.33333333333332860, -4.330127018922193649 ) ) ;
#26983=CARTESIAN_POINT ( 'NONE',  ( -3.535250795749689387E-16, -78.12499999726880162, -5.773502691896257311 ) ) ;
#26984=CARTESIAN_POINT ( 'NONE',  ( -2.500000000000000444, -86.16666666666667140, -4.330127018922193649 ) ) ;
#26986=CARTESIAN_POINT ( 'NONE',  ( 4.458734124999998549, -16.97916666530107221, -2.574251347313721627 ) ) ;
#26987=CARTESIAN_POINT ( 'NONE',  ( -3.152548672688508926E-16, -50.81249999863440792, -5.148502694627439702 ) ) ;
#26988=CARTESIAN_POINT ( 'NONE',  ( -1.339745962155610925, -29.66965819600733312, 5.000000000000000000 ) ) ;
#26989=CARTESIAN_POINT ( 'NONE',  ( 4.458734124999999437, -140.4375000013656063, 0.000000000000000000 ) ) ;
#26992=ORIENTED_EDGE ( 'NONE', *, *, #44872, .T. ) ;
#26993=FACE_OUTER_BOUND ( 'NONE', #25800, .T. ) ;
#26995=CARTESIAN_POINT ( 'NONE',  ( 1.339745962155612702, 18.70534180126147916, -5.000000000000000000 ) ) ;
#26998=CARTESIAN_POINT ( 'NONE',  ( -3.152801135295367096, -149.3125000013655779, -3.152801135295367541 ) ) ;
#27002=CARTESIAN_POINT ( 'NONE',  ( 9.457646018065525792E-16, -62.31249999863440792, 5.148502694627439702 ) ) ;
#27003=CYLINDRICAL_SURFACE ( 'NONE', #43511, 5.000000000000000000 ) ;
#27005=CARTESIAN_POINT ( 'NONE',  ( 4.458734124999999437, -143.4375000013656063, 0.000000000000000000 ) ) ;
#27013=EDGE_CURVE ( 'NONE', #5864, #7305, #55400, .T. ) ;
#27021=LINE ( 'NONE', #7411, #45825 ) ;
#27023=CARTESIAN_POINT ( 'NONE',  ( -2.229367062500000163, 5.520833334698927786, -3.861377020970580443 ) ) ;
#27025=CARTESIAN_POINT ( 'NONE',  ( 2.229367062499998831, -18.89583333196774007, -3.861377020970580887 ) ) ;
#27027=CARTESIAN_POINT ( 'NONE',  ( 4.458734125000000326, -159.3750000013656347, -1.846868145590734978 ) ) ;
#27028=CARTESIAN_POINT ( 'NONE',  ( -2.071067811865580754, -158.6875000000000000, -4.999999999999894307 ) ) ;
#27031=( BOUNDED_CURVE ( )  B_SPLINE_CURVE ( 2, ( #52003, #36568, #31746, #42023, #42339, #41384, #12443, #51377, #32055 ),
 .UNSPECIFIED., .F., .F. ) 
 B_SPLINE_CURVE_WITH_KNOTS ( ( 3, 2, 2, 2, 3 ),
 ( 0.4916666666666670849, 0.4958333333333337922, 0.5000000000000004441, 0.5041666666666670960, 0.5083333333333337478 ),
 .UNSPECIFIED. ) 
 CURVE ( )  GEOMETRIC_REPRESENTATION_ITEM ( )  RATIONAL_B_SPLINE_CURVE ( ( 0.9999999999999918954, 0.9238795325112948431, 1.000000000000000000, 0.9238795325112867385, 1.000000000000000000, 0.9238795325112867385, 1.000000000000000000, 0.9238795325112786339, 1.000000000000008216 ) ) 
 REPRESENTATION_ITEM ( '' )  );
#27033=CARTESIAN_POINT ( 'NONE',  ( -4.458734124999999437, -40.39583333196773651, -2.574251347313719407 ) ) ;
#27034=CARTESIAN_POINT ( 'NONE',  ( 5.000000000000000000, 19.62500000273118772, -6.123233995736766282E-16 ) ) ;
#27035=CARTESIAN_POINT ( 'NONE',  ( 4.458734124999998549, -65.97916666530106511, -2.574251347313721627 ) ) ;
#27037=CARTESIAN_POINT ( 'NONE',  ( 0.000000000000000000, -170.0000000000000000, 5.000000000000000000 ) ) ;
#27038=CARTESIAN_POINT ( 'NONE',  ( -6.972266317189433020E-16, -36.12499999726880162, -5.000000000000000000 ) ) ;
#27042=CARTESIAN_POINT ( 'NONE',  ( -2.499999999999996447, -67.70833333060214443, 4.330127018922195425 ) ) ;
#27043=CARTESIAN_POINT ( 'NONE',  ( 2.499999999999998668, -10.33333333333333393, -4.330127018922193649 ) ) ;
#27044=CARTESIAN_POINT ( 'NONE',  ( 4.458734124999998549, -70.72916666530107932, -2.574251347313721627 ) ) ;
#27046=CARTESIAN_POINT ( 'NONE',  ( -5.000000000000000000, -13.87499999726881228, 0.000000000000000000 ) ) ;
#27047=CARTESIAN_POINT ( 'NONE',  ( -3.152548672688508926E-16, -40.56249999863440081, -5.148502694627439702 ) ) ;
#27048=ORIENTED_EDGE ( 'NONE', *, *, #1576, .F. ) ;
#27050=CARTESIAN_POINT ( 'NONE',  ( 2.229367062499998831, 10.10416666803225993, -3.861377020970580887 ) ) ;
#27051=EDGE_LOOP ( 'NONE', ( #49091, #57147, #51667, #50376 ) ) ;
#27052=CARTESIAN_POINT ( 'NONE',  ( 1.975475456537005874E-15, -81.74999999999998579, 5.000000000000000000 ) ) ;
#27053=CARTESIAN_POINT ( 'NONE',  ( 5.000000000000000000, -54.49999999999999289, -6.123233995736766282E-16 ) ) ;
#27054=CARTESIAN_POINT ( 'NONE',  ( 3.152801135295367541, -160.5625000013656063, -3.152801135295367541 ) ) ;
#27057=CARTESIAN_POINT ( 'NONE',  ( -4.458734124999998549, -79.22916666530107932, 2.574251347313722516 ) ) ;
#27058=CARTESIAN_POINT ( 'NONE',  ( 5.000000000000000888, -164.9375000000000284, -2.071067811865475505 ) ) ;
#27059=CARTESIAN_POINT ( 'NONE',  ( 4.458734124999998549, -87.72916666530107932, -2.574251347313721627 ) ) ;
#27061=CARTESIAN_POINT ( 'NONE',  ( -3.152548672688508926E-16, -0.8124999986344055847, -5.148502694627439702 ) ) ;
#27062=CARTESIAN_POINT ( 'NONE',  ( 2.229367062499998831, -36.89583333196773651, -3.861377020970580887 ) ) ;
#27064=CARTESIAN_POINT ( 'NONE',  ( 5.000000000000000000, -72.41666666666665719, -2.886751345948130876 ) ) ;
#27066=FACE_OUTER_BOUND ( 'NONE', #43217, .T. ) ;
#27067=ORIENTED_EDGE ( 'NONE', *, *, #52004, .F. ) ;
#27068=CARTESIAN_POINT ( 'NONE',  ( -3.535533905932737309, -141.6250000000000000, -3.535533905932738197 ) ) ;
#27069=CARTESIAN_POINT ( 'NONE',  ( -2.500000000000000444, -19.04166666393547658, -4.330127018922193649 ) ) ;
#27070=CARTESIAN_POINT ( 'NONE',  ( 2.229367062499998831, -71.89583333196773651, -3.861377020970580887 ) ) ;
#27072=VERTEX_POINT ( 'NONE', #50741 ) ;
#27073=CARTESIAN_POINT ( 'NONE',  ( -3.535533905932737309, -150.7500000027312126, -3.535533905932738197 ) ) ;
#27074=CARTESIAN_POINT ( 'NONE',  ( -3.535533905932737309, -146.7500000027311842, -3.535533905932738197 ) ) ;
#27077=CARTESIAN_POINT ( 'NONE',  ( 9.457646018065525792E-16, 6.937500001365594748, 5.148502694627439702 ) ) ;
#27078=LINE ( 'NONE', #40593, #61405 ) ;
#27079=CARTESIAN_POINT ( 'NONE',  ( -4.458734124999999437, -156.9375000013655779, -5.460374474430324690E-16 ) ) ;
#27080=( BOUNDED_CURVE ( )  B_SPLINE_CURVE ( 2, ( #30480, #929, #35960, #21160, #51704, #32067, #45599, #16970, #36581 ),
 .UNSPECIFIED., .F., .F. ) 
 B_SPLINE_CURVE_WITH_KNOTS ( ( 3, 2, 2, 2, 3 ),
 ( 0.2895833333333333592, 0.2902777777777778012, 0.2916666666666666852, 0.2930555555555555691, 0.2937500000000000111 ),
 .UNSPECIFIED. ) 
 CURVE ( )  GEOMETRIC_REPRESENTATION_ITEM ( )  RATIONAL_B_SPLINE_CURVE ( ( 0.9330127018922194093, 0.9330127018922220739, 1.000000000000000000, 0.8660254037844387076, 1.000000000000000000, 0.8660254037844387076, 1.000000000000000000, 0.9330127018922194093, 0.9330127018922194093 ) ) 
 REPRESENTATION_ITEM ( '' )  );
#27088=CYLINDRICAL_SURFACE ( 'NONE', #11973, 5.000000000000000000 ) ;
#27093=CARTESIAN_POINT ( 'NONE',  ( -4.458734124999999437, 24.68750000136559208, 0.000000000000000000 ) ) ;
#27096=CARTESIAN_POINT ( 'NONE',  ( 4.458734125000000326, -5.145833331967740065, 2.574251347313718519 ) ) ;
#27097=CARTESIAN_POINT ( 'NONE',  ( -5.000000000000000000, -149.6250000027312126, -6.123233995736766282E-16 ) ) ;
#27099=CARTESIAN_POINT ( 'NONE',  ( -2.071067811865475061, -140.8125000027312126, -5.000000000000000888 ) ) ;
#27100=CARTESIAN_POINT ( 'NONE',  ( 2.500000000000002220, -33.54166666393547303, 4.330127018922192761 ) ) ;
#27106=DIRECTION ( 'NONE',  ( -0.000000000000000000, 1.000000000000000000, -0.000000000000000000 ) ) ;
#27110=CARTESIAN_POINT ( 'NONE',  ( 3.152801135295367541, -162.5625000013656063, -3.152801135295367541 ) ) ;
#27112=FACE_OUTER_BOUND ( 'NONE', #61637, .T. ) ;
#27113=ORIENTED_EDGE ( 'NONE', *, *, #29470, .T. ) ;
#27114=CARTESIAN_POINT ( 'NONE',  ( -4.458734124999998549, 18.52083333469892779, 2.574251347313722516 ) ) ;
#27115=VERTEX_POINT ( 'NONE', #15695 ) ;
#27120=CARTESIAN_POINT ( 'NONE',  ( -2.500000000000000444, 10.83333333333333393, -4.330127018922193649 ) ) ;
#27121=CARTESIAN_POINT ( 'NONE',  ( -3.152548672688508926E-16, -57.56249999863440792, -5.148502694627439702 ) ) ;
#27122=DIRECTION ( 'NONE',  ( 0.8660254037844505870, 0.4999999999999792388, -0.000000000000000000 ) ) ;
#27127=CARTESIAN_POINT ( 'NONE',  ( 1.060575238724906964E-15, -40.74999999999999289, 5.773502691896257311 ) ) ;
#27131=CARTESIAN_POINT ( 'NONE',  ( -2.071067811865432873, -143.6875000000000000, -5.000000000000041744 ) ) ;
#27132=CARTESIAN_POINT ( 'NONE',  ( -4.458734124999999437, -63.39583333196772941, -2.574251347313719407 ) ) ;
#27133=( BOUNDED_CURVE ( )  B_SPLINE_CURVE ( 2, ( #10464, #5652, #25265, #3118, #27858, #12753, #17593, #53252, #3432 ),
 .UNSPECIFIED., .F., .F. ) 
 B_SPLINE_CURVE_WITH_KNOTS ( ( 3, 2, 2, 2, 3 ),
 ( 0.8395833333333333481, 0.8402777777777777901, 0.8416666666666666741, 0.8430555555555555580, 0.8437500000000000000 ),
 .UNSPECIFIED. ) 
 CURVE ( )  GEOMETRIC_REPRESENTATION_ITEM ( )  RATIONAL_B_SPLINE_CURVE ( ( 0.9330127018922194093, 0.9330127018922194093, 1.000000000000000000, 0.8660254037844387076, 1.000000000000000000, 0.8660254037844387076, 1.000000000000000000, 0.9330127018922194093, 0.9330127018922194093 ) ) 
 REPRESENTATION_ITEM ( '' )  );
#27134=CARTESIAN_POINT ( 'NONE',  ( -1.846868145590737420, -153.0000000013656063, 4.458734124999999437 ) ) ;
#27135=CARTESIAN_POINT ( 'NONE',  ( 4.458734124999999437, -69.81249999863439371, -5.460374474430324690E-16 ) ) ;
#27137=CARTESIAN_POINT ( 'NONE',  ( -2.229367062500000163, -19.72916666530107221, -3.861377020970580443 ) ) ;
#27138=CARTESIAN_POINT ( 'NONE',  ( 5.000000000000000000, -62.29166666393547303, -2.886751345948129988 ) ) ;
#27139=ORIENTED_EDGE ( 'NONE', *, *, #41984, .T. ) ;
#27140=EDGE_CURVE ( 'NONE', #16274, #56674, #53688, .T. ) ;
#27141=CARTESIAN_POINT ( 'NONE',  ( -6.972266317189433020E-16, -49.24999999999999289, -5.000000000000000000 ) ) ;
#27144=CARTESIAN_POINT ( 'NONE',  ( 5.000000000000000888, -149.0625000027311842, -2.071067811865475505 ) ) ;
#27145=CARTESIAN_POINT ( 'NONE',  ( -3.152801135295367985, -152.8125000013656063, 3.152801135295367096 ) ) ;
#27146=ORIENTED_EDGE ( 'NONE', *, *, #30734, .T. ) ;
#27147=CARTESIAN_POINT ( 'NONE',  ( -1.339745962155613812, 2.919658201469706782, -5.000000000000000000 ) ) ;
#27149=CARTESIAN_POINT ( 'NONE',  ( 1.975475456537005874E-15, -55.62499999726880873, 5.000000000000000000 ) ) ;
#27150=CARTESIAN_POINT ( 'NONE',  ( 4.458734125000001214, -56.14583333196774362, 2.574251347313718519 ) ) ;
#27153=FACE_OUTER_BOUND ( 'NONE', #49204, .T. ) ;
#27155=CARTESIAN_POINT ( 'NONE',  ( 4.458734124999998549, 25.27083333469892779, -2.574251347313721627 ) ) ;
#27157=CARTESIAN_POINT ( 'NONE',  ( 1.062108568985190270E-13, -13.12499999726881583, -4.999999999999999112 ) ) ;
#27161=CARTESIAN_POINT ( 'NONE',  ( -6.972266317189433020E-16, -86.12499999726880162, -5.000000000000000000 ) ) ;
#27164=CARTESIAN_POINT ( 'NONE',  ( 0.000000000000000000, -170.0000000000000000, 0.000000000000000000 ) ) ;
#27165=EDGE_CURVE ( 'NONE', #53696, #48010, #60291, .T. ) ;
#27172=ORIENTED_EDGE ( 'NONE', *, *, #39359, .T. ) ;
#27173=CARTESIAN_POINT ( 'NONE',  ( 1.975475456537005874E-15, -27.62499999726880873, 5.000000000000000000 ) ) ;
#27175=CARTESIAN_POINT ( 'NONE',  ( 3.535533905932738197, -154.0000000027312126, -3.535533905932738197 ) ) ;
#27176=ORIENTED_EDGE ( 'NONE', *, *, #22478, .T. ) ;
#27180=EDGE_CURVE ( 'NONE', #21022, #37557, #27246, .T. ) ;
#27182=CARTESIAN_POINT ( 'NONE',  ( -3.535533905932738641, -147.3750000000000000, 3.535533905932737309 ) ) ;
#27184=EDGE_CURVE ( 'NONE', #34622, #35553, #9723, .T. ) ;
#27186=CARTESIAN_POINT ( 'NONE',  ( -2.229367062499996610, -25.14583333196773651, 3.861377020970582219 ) ) ;
#27188=CARTESIAN_POINT ( 'NONE',  ( -2.500000000000000444, 8.958333336064518093, -4.330127018922193649 ) ) ;
#27190=CARTESIAN_POINT ( 'NONE',  ( -1.846868145590737420, -151.7500000013655779, 4.458734124999999437 ) ) ;
#27193=CARTESIAN_POINT ( 'NONE',  ( -4.458734124999999437, -53.64583333196773651, -2.574251347313719407 ) ) ;
#27194=CARTESIAN_POINT ( 'NONE',  ( 1.339745962155612702, -58.16965819600732601, -5.000000000000000000 ) ) ;
#27196=CARTESIAN_POINT ( 'NONE',  ( 1.060575238724906964E-15, 26.25000000000000000, 5.773502691896257311 ) ) ;
#27198=CARTESIAN_POINT ( 'NONE',  ( -4.458734124999999437, 0.6041666680322611560, -2.574251347313719407 ) ) ;
#27199=CARTESIAN_POINT ( 'NONE',  ( -2.071067811865394237, -160.4375000027312410, 5.000000000000084377 ) ) ;
#27200=CARTESIAN_POINT ( 'NONE',  ( -9.184850993605147944E-16, -164.2500000000000000, 5.000000000000000000 ) ) ;
#27202=CARTESIAN_POINT ( 'NONE',  ( 2.229367062499998831, 16.10416666803225993, -3.861377020970580887 ) ) ;
#27203=CARTESIAN_POINT ( 'NONE',  ( -2.500000000000000444, 2.958333336064520314, -4.330127018922193649 ) ) ;
#27206=VERTEX_POINT ( 'NONE', #32065 ) ;
#27207=CARTESIAN_POINT ( 'NONE',  ( 5.000000000000000000, -7.291666663935481907, -2.886751345948130876 ) ) ;
#27208=CARTESIAN_POINT ( 'NONE',  ( -4.458734124999998549, -47.22916666530106511, 2.574251347313722516 ) ) ;
#27209=CARTESIAN_POINT ( 'NONE',  ( -4.458734125000001214, -164.1250000013656063, 1.846868145590734089 ) ) ;
#27210=( BOUNDED_CURVE ( )  B_SPLINE_CURVE ( 2, ( #15035, #40428, #2181, #51047, #16950, #51372, #6667, #26924, #36888 ),
 .UNSPECIFIED., .F., .F. ) 
 B_SPLINE_CURVE_WITH_KNOTS ( ( 3, 2, 2, 2, 3 ),
 ( 0.1895833333333333259, 0.1902777777777777679, 0.1916666666666666796, 0.1930555555555555636, 0.1937500000000000056 ),
 .UNSPECIFIED. ) 
 CURVE ( )  GEOMETRIC_REPRESENTATION_ITEM ( )  RATIONAL_B_SPLINE_CURVE ( ( 0.9330127018922194093, 0.9330127018922194093, 1.000000000000000000, 0.8660254037844387076, 1.000000000000000000, 0.8660254037844387076, 1.000000000000000000, 0.9330127018922194093, 0.9330127018922194093 ) ) 
 REPRESENTATION_ITEM ( '' )  );
#27211=CARTESIAN_POINT ( 'NONE',  ( 5.000000000000000000, -44.29166666393546592, -2.886751345948129988 ) ) ;
#27213=CARTESIAN_POINT ( 'NONE',  ( 4.458734125000001214, -24.89583333196773651, 2.574251347313718519 ) ) ;
#27214=ORIENTED_EDGE ( 'NONE', *, *, #7927, .T. ) ;
#27215=CARTESIAN_POINT ( 'NONE',  ( 2.499999999999998668, -87.33333333333332860, -4.330127018922193649 ) ) ;
#27216=CARTESIAN_POINT ( 'NONE',  ( -4.458734125000000326, -163.0000000013655779, -1.846868145590735644 ) ) ;
#27217=CARTESIAN_POINT ( 'NONE',  ( 5.000000000000000000, -39.37499999726880162, -6.123233995736766282E-16 ) ) ;
#27219=CARTESIAN_POINT ( 'NONE',  ( -2.229367062499996610, -30.39583333196773651, 3.861377020970582219 ) ) ;
#27227=CARTESIAN_POINT ( 'NONE',  ( 4.458734124999998549, -79.97916666530107932, -2.574251347313721627 ) ) ;
#27230=CARTESIAN_POINT ( 'NONE',  ( -1.846868145590737420, -140.0000000013655779, 4.458734124999997661 ) ) ;
#27231=CARTESIAN_POINT ( 'NONE',  ( 5.000000000000000000, -84.29166666393547303, -2.886751345948130876 ) ) ;
#27233=CARTESIAN_POINT ( 'NONE',  ( 2.229367062499998831, -47.64583333196774362, -3.861377020970580887 ) ) ;
#27234=CARTESIAN_POINT ( 'NONE',  ( -6.972266317189433020E-16, 27.74999999999999645, -5.000000000000000000 ) ) ;
#27242=CARTESIAN_POINT ( 'NONE',  ( 4.458734124999999437, -80.06249999863440792, -5.460374474430324690E-16 ) ) ;
#27246=LINE ( 'NONE', #2815, #50364 ) ;
#27248=CARTESIAN_POINT ( 'NONE',  ( 2.071067811865475505, -167.9375000027312126, -5.000000000000000888 ) ) ;
#27250=CARTESIAN_POINT ( 'NONE',  ( -4.458734124999999437, 13.35416666803225993, -2.574251347313719407 ) ) ;
#27251=CYLINDRICAL_SURFACE ( 'NONE', #32557, 5.000000000000000000 ) ;
#27257=CARTESIAN_POINT ( 'NONE',  ( -4.999999999999998224, -13.79166666393548191, 2.886751345948131764 ) ) ;
#27258=CARTESIAN_POINT ( 'NONE',  ( 2.499999999999998668, 17.66666666666666430, -4.330127018922193649 ) ) ;
#27259=CARTESIAN_POINT ( 'NONE',  ( -4.458734124999999437, -6.395833331967741842, -2.574251347313719407 ) ) ;
#27261=ADVANCED_FACE ( 'NONE', ( #57169 ), #36903, .T. ) ;
#27263=CARTESIAN_POINT ( 'NONE',  ( 2.229367062500001939, -34.22916666530107221, 3.861377020970579999 ) ) ;
#27269=CARTESIAN_POINT ( 'NONE',  ( -4.458734124999999437, -151.2500000013656063, -1.846868145590735644 ) ) ;
#27270=CARTESIAN_POINT ( 'NONE',  ( -2.229367062500000163, 14.52083333469892779, -3.861377020970580443 ) ) ;
#27271=EDGE_CURVE ( 'NONE', #26215, #11760, #52013, .T. ) ;
#27273=CARTESIAN_POINT ( 'NONE',  ( 5.000000000000000888, -55.58333333333332860, 2.886751345948126879 ) ) ;
#27274=CARTESIAN_POINT ( 'NONE',  ( 4.458734124999999437, -83.06249999863440792, -5.460374474430324690E-16 ) ) ;
#27277=CARTESIAN_POINT ( 'NONE',  ( -5.000000000000000000, 17.12500000273118417, 0.000000000000000000 ) ) ;
#27278=ORIENTED_EDGE ( 'NONE', *, *, #13645, .F. ) ;
#27279=CARTESIAN_POINT ( 'NONE',  ( 5.000000000000000000, -25.41666666666666430, -2.886751345948130876 ) ) ;
#27280=CARTESIAN_POINT ( 'NONE',  ( -9.184850993605147944E-16, -168.3750000027312126, 5.000000000000000000 ) ) ;
#27282=CARTESIAN_POINT ( 'NONE',  ( 5.000000000000000000, -25.50000000000000355, -6.123233995736766282E-16 ) ) ;
#27283=CARTESIAN_POINT ( 'NONE',  ( -4.458734124999999437, -25.39583333196773651, -2.574251347313719407 ) ) ;
#27285=VECTOR ( 'NONE', #33618, 1000.000000000000000 ) ;
#27286=CARTESIAN_POINT ( 'NONE',  ( 2.500000000000002220, -27.54166666393548013, 4.330127018922192761 ) ) ;
#27287=CARTESIAN_POINT ( 'NONE',  ( -4.458734124999999437, -58.31249999863440081, 0.000000000000000000 ) ) ;
#27290=CARTESIAN_POINT ( 'NONE',  ( -4.458734124999999437, -10.56249999863440792, 0.000000000000000000 ) ) ;
#27291=ORIENTED_EDGE ( 'NONE', *, *, #16503, .T. ) ;
#27292=CARTESIAN_POINT ( 'NONE',  ( -3.535250795749689387E-16, -74.25000000000000000, -5.773502691896257311 ) ) ;
#27295=CARTESIAN_POINT ( 'NONE',  ( 5.000000000000000000, -74.37499999726880162, -6.123233995736766282E-16 ) ) ;
#27296=CARTESIAN_POINT ( 'NONE',  ( -5.000000000000000000, -86.08333333333332860, -2.886751345948128211 ) ) ;
#27297=ORIENTED_EDGE ( 'NONE', *, *, #45520, .T. ) ;
#27299=CARTESIAN_POINT ( 'NONE',  ( -2.229367062500000163, -16.72916666530107577, -3.861377020970580443 ) ) ;
#27300=CARTESIAN_POINT ( 'NONE',  ( -2.229367062500000163, -54.72916666530107221, -3.861377020970580443 ) ) ;
#27302=CARTESIAN_POINT ( 'NONE',  ( -4.458734124999999437, -169.1875000013656063, -5.460374474430324690E-16 ) ) ;
#27309=CARTESIAN_POINT ( 'NONE',  ( -5.000000000000000000, -12.95833333060214798, -2.886751345948128211 ) ) ;
#27312=CARTESIAN_POINT ( 'NONE',  ( 4.458734124999999437, -146.6875000013656063, 0.000000000000000000 ) ) ;
#27316=CARTESIAN_POINT ( 'NONE',  ( -4.458734124999998549, -63.47916666530106511, 2.574251347313722516 ) ) ;
#27319=CARTESIAN_POINT ( 'NONE',  ( -4.458734125000000326, -145.8750000013656063, 1.846868145590734089 ) ) ;
#27321=ORIENTED_EDGE ( 'NONE', *, *, #5165, .T. ) ;
#27322=DIRECTION ( 'NONE',  ( 0.000000000000000000, 0.000000000000000000, 1.000000000000000000 ) ) ;
#27325=CARTESIAN_POINT ( 'NONE',  ( 5.000000000000000000, 4.625000002731187720, -6.123233995736766282E-16 ) ) ;
#27327=CARTESIAN_POINT ( 'NONE',  ( -3.152548672688508926E-16, 28.18750000136558853, -5.148502694627439702 ) ) ;
#27328=CARTESIAN_POINT ( 'NONE',  ( 1.975475456537005874E-15, -38.62499999726880873, 5.000000000000000000 ) ) ;
#27334=CARTESIAN_POINT ( 'NONE',  ( 2.229367062499998831, 8.354166668032261711, -3.861377020970580887 ) ) ;
#27336=CARTESIAN_POINT ( 'NONE',  ( 2.229367062500001939, -20.22916666530107221, 3.861377020970579999 ) ) ;
#27338=CARTESIAN_POINT ( 'NONE',  ( -4.458734125000000326, -161.0000000013656063, -1.846868145590735644 ) ) ;
#27342=CARTESIAN_POINT ( 'NONE',  ( 4.458734125000000326, -38.89583333196773651, 2.574251347313718519 ) ) ;
#27344=CARTESIAN_POINT ( 'NONE',  ( -2.229367062500000163, -67.72916666530106511, -3.861377020970580443 ) ) ;
#27347=ORIENTED_EDGE ( 'NONE', *, *, #3493, .T. ) ;
#27348=CYLINDRICAL_SURFACE ( 'NONE', #7315, 5.000000000000000000 ) ;
#27349=CARTESIAN_POINT ( 'NONE',  ( -5.000000000000000000, -7.083333333333330373, -2.886751345948128211 ) ) ;
#27350=CARTESIAN_POINT ( 'NONE',  ( -4.458734124999997661, -71.22916666530107932, 2.574251347313722516 ) ) ;
#27352=CARTESIAN_POINT ( 'NONE',  ( 2.500000000000002220, -14.54166666393548191, 4.330127018922192761 ) ) ;
#27353=CARTESIAN_POINT ( 'NONE',  ( -4.458734124999999437, -38.39583333196773651, -2.574251347313719407 ) ) ;
#27355=DIRECTION ( 'NONE',  ( 0.000000000000000000, 0.000000000000000000, 1.000000000000000000 ) ) ;
#27356=CARTESIAN_POINT ( 'NONE',  ( -4.458734124999999437, 6.437500001365593860, 0.000000000000000000 ) ) ;
#27358=CARTESIAN_POINT ( 'NONE',  ( 5.000000000000000000, -34.37499999726881583, -6.123233995736766282E-16 ) ) ;
#27359=CARTESIAN_POINT ( 'NONE',  ( 1.060575238724906964E-15, -56.74999999999999289, 5.773502691896257311 ) ) ;
#27360=CARTESIAN_POINT ( 'NONE',  ( 4.458734125000000326, -159.6250000013656063, -1.846868145590734978 ) ) ;
#27362=CARTESIAN_POINT ( 'NONE',  ( 5.000000000000000000, -145.0000000000000284, 0.000000000000000000 ) ) ;
#27363=CARTESIAN_POINT ( 'NONE',  ( 2.229367062500001939, -78.97916666530106511, 3.861377020970579999 ) ) ;
#27364=CARTESIAN_POINT ( 'NONE',  ( -3.535533905932737309, -167.6250000000000284, -3.535533905932738197 ) ) ;
#27365=CARTESIAN_POINT ( 'NONE',  ( -2.229367062500000163, -89.47916666530106511, -3.861377020970580443 ) ) ;
#27367=CARTESIAN_POINT ( 'NONE',  ( 2.229367062499998831, 2.104166668032262599, -3.861377020970580887 ) ) ;
#27368=VECTOR ( 'NONE', #48269, 1000.000000000000000 ) ;
#27369=CARTESIAN_POINT ( 'NONE',  ( -4.458734124999999437, -39.64583333196774362, -2.574251347313719407 ) ) ;
#27375=CARTESIAN_POINT ( 'NONE',  ( 5.000000000000000000, -152.0000000000000284, 0.000000000000000000 ) ) ;
#27376=CARTESIAN_POINT ( 'NONE',  ( -3.152548672688508926E-16, -71.81249999863439371, -5.148502694627439702 ) ) ;
#27381=CARTESIAN_POINT ( 'NONE',  ( 5.000000000000000888, -163.9375000000000000, -2.071067811865475505 ) ) ;
#27384=CARTESIAN_POINT ( 'NONE',  ( -5.000000000000000000, 2.916666666666668739, -2.886751345948128211 ) ) ;
#27385=CARTESIAN_POINT ( 'NONE',  ( 4.458734124999998549, 1.270833334698927342, -2.574251347313721627 ) ) ;
#27386=CARTESIAN_POINT ( 'NONE',  ( 5.000000000000000000, -154.0625000000000284, 2.071067811865478614 ) ) ;
#27387=CARTESIAN_POINT ( 'NONE',  ( -3.152801135295367985, -157.8125000013656063, 3.152801135295367096 ) ) ;
#27389=VERTEX_POINT ( 'NONE', #22436 ) ;
#27391=CARTESIAN_POINT ( 'NONE',  ( 1.975475456537005874E-15, -46.74999999999999289, 5.000000000000000000 ) ) ;
#27401=CARTESIAN_POINT ( 'NONE',  ( -4.458734124999999437, 23.68750000136559564, 0.000000000000000000 ) ) ;
#27403=CARTESIAN_POINT ( 'NONE',  ( 4.458734124999998549, -3.979166665301070438, -2.574251347313721627 ) ) ;
#27404=CARTESIAN_POINT ( 'NONE',  ( 2.071067811865370256, -159.9375000027312410, -5.000000000000105693 ) ) ;
#27406=CARTESIAN_POINT ( 'NONE',  ( -9.184850993605147944E-16, -140.3750000027312126, 5.000000000000000000 ) ) ;
#27413=CARTESIAN_POINT ( 'NONE',  ( -6.972266317189433020E-16, -22.24999999999999645, -5.000000000000000000 ) ) ;
#27415=CARTESIAN_POINT ( 'NONE',  ( -3.152801135295367096, -158.3125000013656063, -3.152801135295367541 ) ) ;
#27419=CARTESIAN_POINT ( 'NONE',  ( -4.458734124999999437, 19.43750000136559208, 0.000000000000000000 ) ) ;
#27425=CARTESIAN_POINT ( 'NONE',  ( -4.999999999999999112, 9.083333333333333925, 2.886751345948131764 ) ) ;
#27426=CARTESIAN_POINT ( 'NONE',  ( 2.229367062500001939, -53.97916666530107221, 3.861377020970579999 ) ) ;
#27427=CARTESIAN_POINT ( 'NONE',  ( -4.999999999999998224, -52.79166666393548013, 2.886751345948131764 ) ) ;
#27432=CARTESIAN_POINT ( 'NONE',  ( 5.000000000000000888, -38.58333333333332860, 2.886751345948126879 ) ) ;
#27433=CARTESIAN_POINT ( 'NONE',  ( 2.071067811865349828, -149.1875000000000284, 5.000000000000126121 ) ) ;
#27437=CARTESIAN_POINT ( 'NONE',  ( -3.152548672688508926E-16, -66.56249999863440792, -5.148502694627439702 ) ) ;
#27438=CARTESIAN_POINT ( 'NONE',  ( 1.846868145590735200, -147.5000000013656063, -4.458734125000000326 ) ) ;
#27439=CARTESIAN_POINT ( 'NONE',  ( 9.457646018065525792E-16, -69.06249999863439371, 5.148502694627439702 ) ) ;
#27442=CARTESIAN_POINT ( 'NONE',  ( -4.458734124999999437, -18.56249999863440792, 0.000000000000000000 ) ) ;
#27443=CARTESIAN_POINT ( 'NONE',  ( 2.499999999999998668, -61.20833333060214443, -4.330127018922193649 ) ) ;
#27445=CARTESIAN_POINT ( 'NONE',  ( -3.535533905932737309, -150.6250000000000000, -3.535533905932738197 ) ) ;
#27450=VERTEX_POINT ( 'NONE', #42349 ) ;
#27452=CARTESIAN_POINT ( 'NONE',  ( -5.000000000000000000, 3.125000002731185944, 0.000000000000000000 ) ) ;
#27454=CARTESIAN_POINT ( 'NONE',  ( -4.999999999999998224, -55.79166666393548013, 2.886751345948131764 ) ) ;
#27455=CARTESIAN_POINT ( 'NONE',  ( -2.229367062499996610, -56.39583333196773651, 3.861377020970582219 ) ) ;
#27456=AXIS2_PLACEMENT_3D ( 'NONE', #43061, #33725, #9277 ) ;
#27457=ORIENTED_EDGE ( 'NONE', *, *, #28268, .F. ) ;
#27461=EDGE_CURVE ( 'NONE', #31328, #30756, #38468, .T. ) ;
#27463=CARTESIAN_POINT ( 'NONE',  ( 2.229367062500001939, 20.02083333469892779, 3.861377020970579999 ) ) ;
#27471=EDGE_CURVE ( 'NONE', #53941, #27799, #1125, .T. ) ;
#27472=DIRECTION ( 'NONE',  ( 0.000000000000000000, 0.000000000000000000, 1.000000000000000000 ) ) ;
#27477=CARTESIAN_POINT ( 'NONE',  ( 1.975475456537005874E-15, 19.25000000000000000, 5.000000000000000000 ) ) ;
#27480=ORIENTED_EDGE ( 'NONE', *, *, #31853, .T. ) ;
#27483=CARTESIAN_POINT ( 'NONE',  ( -3.535533905932738641, -153.5000000027312126, 3.535533905932737309 ) ) ;
#27484=EDGE_LOOP ( 'NONE', ( #16903, #59683, #27673, #21371 ) ) ;
#27489=CARTESIAN_POINT ( 'NONE',  ( -5.000000000000000000, -145.5000000000000284, -6.123233995736766282E-16 ) ) ;
#27490=EDGE_CURVE ( 'NONE', #8617, #4579, #4845, .T. ) ;
#27493=CARTESIAN_POINT ( 'NONE',  ( 5.000000000000000000, 22.62500000273118772, -6.123233995736766282E-16 ) ) ;
#27494=CARTESIAN_POINT ( 'NONE',  ( 2.229367062500001939, -24.97916666530106866, 3.861377020970579999 ) ) ;
#27495=CARTESIAN_POINT ( 'NONE',  ( 5.000000000000000000, 14.49999999999999822, -6.123233995736766282E-16 ) ) ;
#27498=CARTESIAN_POINT ( 'NONE',  ( -1.846868145590737420, -147.7500000013655779, 4.458734124999999437 ) ) ;
#27501=CARTESIAN_POINT ( 'NONE',  ( 4.458734124999999437, -50.06249999863440792, -5.460374474430324690E-16 ) ) ;
#27502=VECTOR ( 'NONE', #5231, 1000.000000000000000 ) ;
#27504=CARTESIAN_POINT ( 'NONE',  ( 2.499999999999998668, 24.66666666666666785, -4.330127018922193649 ) ) ;
#27507=CARTESIAN_POINT ( 'NONE',  ( -2.229367062499996610, -3.145833331967738733, 3.861377020970582219 ) ) ;
#27508=CARTESIAN_POINT ( 'NONE',  ( -5.000000000000000888, -154.5625000000000000, -2.071067811865475949 ) ) ;
#27511=CARTESIAN_POINT ( 'NONE',  ( -4.458734124999999437, 10.43750000136559386, 0.000000000000000000 ) ) ;
#27514=ORIENTED_EDGE ( 'NONE', *, *, #61394, .F. ) ;
#27516=CARTESIAN_POINT ( 'NONE',  ( -4.458734124999999437, -46.39583333196774362, -2.574251347313719407 ) ) ;
#27517=CARTESIAN_POINT ( 'NONE',  ( 4.458734125000000326, -161.6250000013656063, -1.846868145590734978 ) ) ;
#27518=EDGE_CURVE ( 'NONE', #33686, #49037, #7318, .T. ) ;
#27519=EDGE_CURVE ( 'NONE', #21524, #53932, #29432, .T. ) ;
#27520=CARTESIAN_POINT ( 'NONE',  ( -2.500000000000000444, -43.04166666393548013, -4.330127018922193649 ) ) ;
#27522=ORIENTED_EDGE ( 'NONE', *, *, #33933, .T. ) ;
#27523=CARTESIAN_POINT ( 'NONE',  ( 4.458734124999999437, -22.81249999863440436, -5.460374474430324690E-16 ) ) ;
#27524=EDGE_LOOP ( 'NONE', ( #54177, #17852, #34100, #4130 ) ) ;
#27526=CARTESIAN_POINT ( 'NONE',  ( -4.458734125000001214, -164.8750000013655779, 1.846868145590734089 ) ) ;
#27527=CYLINDRICAL_SURFACE ( 'NONE', #44708, 5.000000000000000000 ) ;
#27529=CARTESIAN_POINT ( 'NONE',  ( 4.458734124999998549, -37.97916666530107932, -2.574251347313721627 ) ) ;
#27535=ORIENTED_EDGE ( 'NONE', *, *, #18493, .F. ) ;
#27536=CARTESIAN_POINT ( 'NONE',  ( 0.000000000000000000, -170.0000000000000000, 0.000000000000000000 ) ) ;
#27538=CARTESIAN_POINT ( 'NONE',  ( 2.229367062500001939, -86.22916666530107932, 3.861377020970579999 ) ) ;
#27542=CARTESIAN_POINT ( 'NONE',  ( 2.499999999999998668, -57.33333333333333570, -4.330127018922193649 ) ) ;
#27547=CARTESIAN_POINT ( 'NONE',  ( -4.999999999999998224, 4.083333333333334814, 2.886751345948131764 ) ) ;
#27551=CARTESIAN_POINT ( 'NONE',  ( 1.975475456537005874E-15, -82.62499999726878741, 5.000000000000000000 ) ) ;
#27552=CARTESIAN_POINT ( 'NONE',  ( -2.229367062499996610, -81.39583333196773651, 3.861377020970582219 ) ) ;
#27556=DIRECTION ( 'NONE',  ( 0.000000000000000000, 0.000000000000000000, 1.000000000000000000 ) ) ;
#27558=CARTESIAN_POINT ( 'NONE',  ( -3.535533905932738641, -165.5000000027312126, 3.535533905932737309 ) ) ;
#27560=CARTESIAN_POINT ( 'NONE',  ( 4.458734124999999437, 10.93750000136559386, -5.460374474430324690E-16 ) ) ;
#27566=CARTESIAN_POINT ( 'NONE',  ( -6.972266317189433020E-16, -16.12499999726881228, -5.000000000000000000 ) ) ;
#27567=CYLINDRICAL_SURFACE ( 'NONE', #33650, 5.000000000000000000 ) ;
#27568=CARTESIAN_POINT ( 'NONE',  ( 4.458734124999998549, -6.729166665301073103, -2.574251347313721627 ) ) ;
#27570=EDGE_LOOP ( 'NONE', ( #5444, #34344, #13380, #28097 ) ) ;
#27571=CARTESIAN_POINT ( 'NONE',  ( 2.229367062500001939, -37.22916666530107221, 3.861377020970579999 ) ) ;
#27573=CARTESIAN_POINT ( 'NONE',  ( 1.975475456537005874E-15, -11.74999999999999645, 5.000000000000000000 ) ) ;
#27577=CARTESIAN_POINT ( 'NONE',  ( 4.458734124999998549, 14.27083333469892779, -2.574251347313721627 ) ) ;
#27580=CARTESIAN_POINT ( 'NONE',  ( 4.458734125000000326, -86.14583333196775072, 2.574251347313718519 ) ) ;
#27583=CARTESIAN_POINT ( 'NONE',  ( -3.535250795749689387E-16, 20.87500000273118417, -5.773502691896257311 ) ) ;
#27584=ORIENTED_EDGE ( 'NONE', *, *, #43803, .T. ) ;
#27585=CARTESIAN_POINT ( 'NONE',  ( 5.000000000000000888, -35.58333333333332860, 2.886751345948126879 ) ) ;
#27588=CARTESIAN_POINT ( 'NONE',  ( -5.000000000000000000, -31.08333333333332860, -2.886751345948128211 ) ) ;
#27589=CARTESIAN_POINT ( 'NONE',  ( 2.229367062499998831, -31.64583333196773651, -3.861377020970580887 ) ) ;
#27591=CARTESIAN_POINT ( 'NONE',  ( 1.975475456537005874E-15, 0.2500000000000001665, 5.000000000000000000 ) ) ;
#27592=EDGE_CURVE ( 'NONE', #35368, #45099, #44665, .T. ) ;
#27593=CARTESIAN_POINT ( 'NONE',  ( 5.000000000000000000, -28.37499999726881228, -6.123233995736766282E-16 ) ) ;
#27594=EDGE_CURVE ( 'NONE', #48474, #42868, #14238, .T. ) ;
#27595=CARTESIAN_POINT ( 'NONE',  ( -4.458734124999998549, -61.22916666530106511, 2.574251347313722516 ) ) ;
#27597=DIRECTION ( 'NONE',  ( 0.000000000000000000, 0.000000000000000000, 1.000000000000000000 ) ) ;
#27598=CARTESIAN_POINT ( 'NONE',  ( -4.458734124999998549, -6.479166665301073103, 2.574251347313722516 ) ) ;
#27599=ORIENTED_EDGE ( 'NONE', *, *, #18015, .T. ) ;
#27601=CARTESIAN_POINT ( 'NONE',  ( 1.060575238724906964E-15, -77.75000000000000000, 5.773502691896257311 ) ) ;
#27605=CARTESIAN_POINT ( 'NONE',  ( -2.500000000000000444, -78.04166666393547303, -4.330127018922193649 ) ) ;
#27606=FACE_OUTER_BOUND ( 'NONE', #40683, .T. ) ;
#27609=EDGE_CURVE ( 'NONE', #48046, #14245, #20833, .T. ) ;
#27610=CARTESIAN_POINT ( 'NONE',  ( -2.229367062499996610, -20.39583333196774007, 3.861377020970582219 ) ) ;
#27612=CARTESIAN_POINT ( 'NONE',  ( 4.458734124999999437, -59.06249999863440081, -5.460374474430324690E-16 ) ) ;
#27613=FILL_AREA_STYLE_COLOUR ( '', #11242 ) ;
#27614=CARTESIAN_POINT ( 'NONE',  ( 4.458734124999999437, -141.4375000013656063, 0.000000000000000000 ) ) ;
#27616=DIRECTION ( 'NONE',  ( -0.000000000000000000, 1.000000000000000000, -0.000000000000000000 ) ) ;
#27618=EDGE_CURVE ( 'NONE', #2786, #26202, #62356, .T. ) ;
#27626=CARTESIAN_POINT ( 'NONE',  ( -1.846868145590734756, -149.3750000013656347, -4.458734125000000326 ) ) ;
#27630=( BOUNDED_CURVE ( )  B_SPLINE_CURVE ( 2, ( #47166, #56186, #3110, #12106, #31733, #51363, #7619, #22410, #45888 ),
 .UNSPECIFIED., .F., .F. ) 
 B_SPLINE_CURVE_WITH_KNOTS ( ( 3, 2, 2, 2, 3 ),
 ( 0.4812500000000000111, 0.4819444444444444531, 0.4833333333333333370, 0.4847222222222222210, 0.4854166666666666630 ),
 .UNSPECIFIED. ) 
 CURVE ( )  GEOMETRIC_REPRESENTATION_ITEM ( )  RATIONAL_B_SPLINE_CURVE ( ( 0.9330127018922194093, 0.9330127018922194093, 1.000000000000000000, 0.8660254037844387076, 1.000000000000000000, 0.8660254037844387076, 1.000000000000000000, 0.9330127018922194093, 0.9330127018922194093 ) ) 
 REPRESENTATION_ITEM ( '' )  );
#27631=CARTESIAN_POINT ( 'NONE',  ( 4.458734124999998549, -64.97916666530106511, -2.574251347313721627 ) ) ;
#27634=CARTESIAN_POINT ( 'NONE',  ( -3.152801135295367985, -146.8125000013655779, 3.152801135295367096 ) ) ;
#27644=CYLINDRICAL_SURFACE ( 'NONE', #56120, 5.000000000000000000 ) ;
#27647=CYLINDRICAL_SURFACE ( 'NONE', #12993, 5.000000000000000000 ) ;
#27649=CARTESIAN_POINT ( 'NONE',  ( -3.152548672688508926E-16, 5.437500001365592084, -5.148502694627439702 ) ) ;
#27651=CARTESIAN_POINT ( 'NONE',  ( -4.458734124999997661, -21.47916666530107221, 2.574251347313722516 ) ) ;
#27653=CARTESIAN_POINT ( 'NONE',  ( 4.458734124999999437, -160.5000000013656347, 1.846868145590737864 ) ) ;
#27654=CARTESIAN_POINT ( 'NONE',  ( -5.000000000000000000, -158.5000000000000000, -6.123233995736766282E-16 ) ) ;
#27658=CARTESIAN_POINT ( 'NONE',  ( 9.457646018065525792E-16, -40.06249999863440081, 5.148502694627439702 ) ) ;
#27660=CARTESIAN_POINT ( 'NONE',  ( 4.458734124999998549, -64.97916666530106511, -2.574251347313721627 ) ) ;
#27664=ORIENTED_EDGE ( 'NONE', *, *, #49692, .T. ) ;
#27666=CYLINDRICAL_SURFACE ( 'NONE', #32971, 5.000000000000000000 ) ;
#27667=CARTESIAN_POINT ( 'NONE',  ( 2.500000000000002220, -15.66666666666666963, 4.330127018922192761 ) ) ;
#27668=CARTESIAN_POINT ( 'NONE',  ( 4.458734124999998549, -17.72916666530106866, -2.574251347313721627 ) ) ;
#27669=CARTESIAN_POINT ( 'NONE',  ( -4.458734124999999437, -77.31249999863440792, 0.000000000000000000 ) ) ;
#27670=DIRECTION ( 'NONE',  ( -0.000000000000000000, 1.000000000000000000, -0.000000000000000000 ) ) ;
#27671=CARTESIAN_POINT ( 'NONE',  ( 5.000000000000000000, -11.29166666393547835, -2.886751345948129988 ) ) ;
#27672=CARTESIAN_POINT ( 'NONE',  ( -4.458734124999999437, -44.31249999863440081, 0.000000000000000000 ) ) ;
#27673=ORIENTED_EDGE ( 'NONE', *, *, #51539, .T. ) ;
#27675=CARTESIAN_POINT ( 'NONE',  ( -4.458734124999999437, 9.354166668032261711, -2.574251347313719407 ) ) ;
#27678=CARTESIAN_POINT ( 'NONE',  ( -5.000000000000000000, -57.08333333333333570, -2.886751345948128211 ) ) ;
#27679=CARTESIAN_POINT ( 'NONE',  ( 2.730187237215162345E-16, -158.4375000013655779, -4.458734124999999437 ) ) ;
#27683=CARTESIAN_POINT ( 'NONE',  ( 2.229367062499998831, -79.64583333196773651, -3.861377020970580887 ) ) ;
#27685=CARTESIAN_POINT ( 'NONE',  ( 2.071067811865475505, -165.8125000000000000, -5.000000000000000888 ) ) ;
#27687=VECTOR ( 'NONE', #63180, 1000.000000000000000 ) ;
#27689=CARTESIAN_POINT ( 'NONE',  ( -3.152548672688508926E-16, -2.812499998634407028, -5.148502694627439702 ) ) ;
#27690=CARTESIAN_POINT ( 'NONE',  ( 4.458734124999998549, -38.97916666530107221, -2.574251347313721627 ) ) ;
#27691=CARTESIAN_POINT ( 'NONE',  ( 1.975475456537005874E-15, -54.74999999999999289, 5.000000000000000000 ) ) ;
#27693=DIRECTION ( 'NONE',  ( 0.000000000000000000, 0.000000000000000000, 1.000000000000000000 ) ) ;
#27694=VERTEX_POINT ( 'NONE', #12694 ) ;
#27695=CARTESIAN_POINT ( 'NONE',  ( 0.000000000000000000, -170.0000000000000000, 5.000000000000000000 ) ) ;
#27696=CARTESIAN_POINT ( 'NONE',  ( -1.339745962155610925, -11.66965819600733667, 5.000000000000000000 ) ) ;
#27697=CARTESIAN_POINT ( 'NONE',  ( -4.458734124999998549, -68.47916666530106511, 2.574251347313722516 ) ) ;
#27699=VERTEX_POINT ( 'NONE', #7561 ) ;
#27700=CARTESIAN_POINT ( 'NONE',  ( 1.339745962155615144, -5.705341801261479162, 4.999999999999999112 ) ) ;
#27701=ADVANCED_FACE ( 'NONE', ( #31345 ), #51936, .T. ) ;
#27705=CARTESIAN_POINT ( 'NONE',  ( 4.458734125000001214, 0.1041666680322607674, 2.574251347313718519 ) ) ;
#27707=CARTESIAN_POINT ( 'NONE',  ( 4.458734124999997661, -158.5000000013656347, 1.846868145590737864 ) ) ;
#27711=CARTESIAN_POINT ( 'NONE',  ( -4.999999999999998224, -46.91666666666666430, 2.886751345948131764 ) ) ;
#27713=CARTESIAN_POINT ( 'NONE',  ( 3.535533905932736864, -140.1250000000000000, 3.535533905932738641 ) ) ;
#27714=LINE ( 'NONE', #38316, #3732 ) ;
#27717=CARTESIAN_POINT ( 'NONE',  ( 2.499999999999998668, -78.33333333333332860, -4.330127018922193649 ) ) ;
#27719=CARTESIAN_POINT ( 'NONE',  ( 2.499999999999998668, -10.33333333333333393, -4.330127018922193649 ) ) ;
#27720=CARTESIAN_POINT ( 'NONE',  ( -2.229367062500000163, 23.52083333469892779, -3.861377020970580443 ) ) ;
#27722=CARTESIAN_POINT ( 'NONE',  ( 2.229367062500001939, -2.229166665301068662, 3.861377020970579999 ) ) ;
#27725=CARTESIAN_POINT ( 'NONE',  ( -2.071067811865478170, -143.4375000027312410, 5.000000000000000000 ) ) ;
#27730=LINE ( 'NONE', #7810, #6203 ) ;
#27733=CARTESIAN_POINT ( 'NONE',  ( 3.152801135295367541, -159.5625000013656063, -3.152801135295367541 ) ) ;
#27736=ORIENTED_EDGE ( 'NONE', *, *, #22246, .T. ) ;
#27737=CARTESIAN_POINT ( 'NONE',  ( 2.229367062500001939, 15.77083333469892601, 3.861377020970579999 ) ) ;
#27743=CARTESIAN_POINT ( 'NONE',  ( 5.000000000000000000, 8.500000000000000000, -6.123233995736766282E-16 ) ) ;
#27744=CARTESIAN_POINT ( 'NONE',  ( 4.458734125000000326, -60.89583333196774362, 2.574251347313718519 ) ) ;
#27747=CARTESIAN_POINT ( 'NONE',  ( 9.457646018065525792E-16, -31.06249999863440436, 5.148502694627439702 ) ) ;
#27748=DIRECTION ( 'NONE',  ( -0.000000000000000000, 1.000000000000000000, -0.000000000000000000 ) ) ;
#27749=CARTESIAN_POINT ( 'NONE',  ( 6.123233995736766282E-16, -170.0000000000000000, -5.000000000000000000 ) ) ;
#27751=CARTESIAN_POINT ( 'NONE',  ( -5.000000000000000000, -42.08333333333333570, -2.886751345948128211 ) ) ;
#27753=CARTESIAN_POINT ( 'NONE',  ( -2.500000000000000444, -48.16666666666666430, -4.330127018922193649 ) ) ;
#27756=CARTESIAN_POINT ( 'NONE',  ( -3.152548672688508926E-16, -67.56249999863440792, -5.148502694627439702 ) ) ;
#27757=CARTESIAN_POINT ( 'NONE',  ( 1.846868145590736310, -147.8750000013656063, 4.458734124999999437 ) ) ;
#27758=CARTESIAN_POINT ( 'NONE',  ( 4.458734125000001214, -73.89583333196773651, 2.574251347313718519 ) ) ;
#27760=( BOUNDED_CURVE ( )  B_SPLINE_CURVE ( 2, ( #8545, #42950, #17879, #17574, #27217, #52920, #32035, #47157, #8858 ),
 .UNSPECIFIED., .F., .F. ) 
 B_SPLINE_CURVE_WITH_KNOTS ( ( 3, 2, 2, 2, 3 ),
 ( 0.5687499999999999778, 0.5694444444444444198, 0.5708333333333333037, 0.5722222222222221877, 0.5729166666666666297 ),
 .UNSPECIFIED. ) 
 CURVE ( )  GEOMETRIC_REPRESENTATION_ITEM ( )  RATIONAL_B_SPLINE_CURVE ( ( 0.9330127018922194093, 0.9330127018922194093, 1.000000000000000000, 0.8660254037844387076, 1.000000000000000000, 0.8660254037844387076, 1.000000000000000000, 0.9330127018922194093, 0.9330127018922194093 ) ) 
 REPRESENTATION_ITEM ( '' )  );
#27761=CARTESIAN_POINT ( 'NONE',  ( 4.458734124999998549, -23.97916666530107221, -2.574251347313721627 ) ) ;
#27762=CARTESIAN_POINT ( 'NONE',  ( 1.060575238724906964E-15, -65.62499999726881583, 5.773502691896257311 ) ) ;
#27763=ORIENTED_EDGE ( 'NONE', *, *, #21284, .F. ) ;
#27765=VERTEX_POINT ( 'NONE', #27173 ) ;
#27773=CARTESIAN_POINT ( 'NONE',  ( 9.457646018065525792E-16, -52.31249999863440792, 5.148502694627439702 ) ) ;
#27774=VERTEX_POINT ( 'NONE', #51627 ) ;
#27778=CARTESIAN_POINT ( 'NONE',  ( -3.152548672688508926E-16, 20.43750000136559208, -5.148502694627439702 ) ) ;
#27781=CARTESIAN_POINT ( 'NONE',  ( -4.458734125000000326, -168.8750000013656063, 1.846868145590734089 ) ) ;
#27782=ORIENTED_EDGE ( 'NONE', *, *, #45086, .F. ) ;
#27784=CYLINDRICAL_SURFACE ( 'NONE', #23289, 5.000000000000000000 ) ;
#27786=CARTESIAN_POINT ( 'NONE',  ( -9.184850993605147944E-16, -140.3750000027312126, 5.000000000000000000 ) ) ;
#27790=CARTESIAN_POINT ( 'NONE',  ( 3.535533905932738197, -160.8750000000000284, -3.535533905932738197 ) ) ;
#27791=CARTESIAN_POINT ( 'NONE',  ( 1.339745962155615144, -76.70534180126148271, 4.999999999999999112 ) ) ;
#27792=FACE_OUTER_BOUND ( 'NONE', #9104, .T. ) ;
#27795=EDGE_LOOP ( 'NONE', ( #28225, #2396, #54264, #40821 ) ) ;
#27798=CARTESIAN_POINT ( 'NONE',  ( 5.000000000000000000, -155.1875000027312126, 2.071067811865478614 ) ) ;
#27799=VERTEX_POINT ( 'NONE', #12380 ) ;
#27801=EDGE_CURVE ( 'NONE', #13440, #44449, #42617, .T. ) ;
#27805=CARTESIAN_POINT ( 'NONE',  ( 3.535533905932736864, -145.1250000000000000, 3.535533905932738641 ) ) ;
#27808=CARTESIAN_POINT ( 'NONE',  ( 4.458734124999999437, -168.6250000013656063, -1.846868145590734978 ) ) ;
#27809=CARTESIAN_POINT ( 'NONE',  ( -2.229367062499996610, -26.14583333196773651, 3.861377020970582219 ) ) ;
#27811=CARTESIAN_POINT ( 'NONE',  ( -6.972266317189433020E-16, 8.875000002731184168, -5.000000000000000000 ) ) ;
#27813=CARTESIAN_POINT ( 'NONE',  ( 1.846868145590736310, -146.6250000013655779, 4.458734124999999437 ) ) ;
#27815=CARTESIAN_POINT ( 'NONE',  ( 6.123233995736766282E-16, -170.0000000000000000, -5.000000000000000000 ) ) ;
#27816=CARTESIAN_POINT ( 'NONE',  ( 2.229367062500001939, -56.22916666530107221, 3.861377020970579999 ) ) ;
#27819=CARTESIAN_POINT ( 'NONE',  ( -2.500000000000000444, 26.83333333333333570, -4.330127018922193649 ) ) ;
#27820=AXIS2_PLACEMENT_3D ( 'NONE', #5196, #38641, #58901 ) ;
#27821=CARTESIAN_POINT ( 'NONE',  ( 1.975475456537005874E-15, -17.62499999726881938, 5.000000000000000000 ) ) ;
#27822=CARTESIAN_POINT ( 'NONE',  ( 2.229367062499998831, -2.645833331967738289, -3.861377020970580887 ) ) ;
#27823=EDGE_CURVE ( 'NONE', #47490, #10933, #16570, .T. ) ;
#27825=CARTESIAN_POINT ( 'NONE',  ( 2.071067811865517694, -140.8124999999999716, -4.999999999999958256 ) ) ;
#27826=CARTESIAN_POINT ( 'NONE',  ( -2.229367062499996610, 12.60416666803226171, 3.861377020970582219 ) ) ;
#27829=ORIENTED_EDGE ( 'NONE', *, *, #50727, .F. ) ;
#27830=( BOUNDED_CURVE ( )  B_SPLINE_CURVE ( 2, ( #32735, #62016, #46905, #56244, #7358, #12483, #17934, #52362, #57198 ),
 .UNSPECIFIED., .F., .F. ) 
 B_SPLINE_CURVE_WITH_KNOTS ( ( 3, 2, 2, 2, 3 ),
 ( 0.7249999999999996447, 0.7291666666666662966, 0.7333333333333329485, 0.7374999999999998224, 0.7416666666666664742 ),
 .UNSPECIFIED. ) 
 CURVE ( )  GEOMETRIC_REPRESENTATION_ITEM ( )  RATIONAL_B_SPLINE_CURVE ( ( 1.000000000000005995, 0.9238795325112806323, 1.000000000000000000, 0.9238795325112867385, 1.000000000000000000, 0.9238795325112867385, 1.000000000000000000, 0.9238795325112908463, 0.9999999999999958922 ) ) 
 REPRESENTATION_ITEM ( '' )  );
#27832=CARTESIAN_POINT ( 'NONE',  ( 4.458734124999999437, -49.81249999863440792, -5.460374474430324690E-16 ) ) ;
#27833=CARTESIAN_POINT ( 'NONE',  ( -4.458734125000001214, -160.1250000013655779, 1.846868145590734089 ) ) ;
#27834=CARTESIAN_POINT ( 'NONE',  ( -2.499999999999996447, -44.70833333060214443, 4.330127018922195425 ) ) ;
#27835=VERTEX_POINT ( 'NONE', #61915 ) ;
#27836=CARTESIAN_POINT ( 'NONE',  ( 9.457646018065525792E-16, -23.06249999863440792, 5.148502694627439702 ) ) ;
#27839=CARTESIAN_POINT ( 'NONE',  ( -1.846868145590734756, -160.1250000013655779, -4.458734125000000326 ) ) ;
#27840=CARTESIAN_POINT ( 'NONE',  ( 0.000000000000000000, -170.0000000000000000, 0.000000000000000000 ) ) ;
#27842=CARTESIAN_POINT ( 'NONE',  ( 9.457646018065525792E-16, -40.31249999863440081, 5.148502694627439702 ) ) ;
#27843=CARTESIAN_POINT ( 'NONE',  ( -6.972266317189433020E-16, 19.87500000273118417, -5.000000000000000000 ) ) ;
#27844=VERTEX_POINT ( 'NONE', #22356 ) ;
#27851=CARTESIAN_POINT ( 'NONE',  ( -2.229367062499996610, -83.39583333196773651, 3.861377020970582219 ) ) ;
#27854=CARTESIAN_POINT ( 'NONE',  ( -9.184850993605147944E-16, -158.3750000027311842, 5.000000000000000000 ) ) ;
#27856=CARTESIAN_POINT ( 'NONE',  ( -1.339745962155610925, -46.66965819600733312, 5.000000000000000000 ) ) ;
#27858=CARTESIAN_POINT ( 'NONE',  ( -5.000000000000000000, -71.87499999726880162, 0.000000000000000000 ) ) ;
#27862=LINE ( 'NONE', #43586, #61769 ) ;
#27867=CARTESIAN_POINT ( 'NONE',  ( -2.229367062500000163, -85.72916666530107932, -3.861377020970580443 ) ) ;
#27870=VERTEX_POINT ( 'NONE', #11729 ) ;
#27871=CARTESIAN_POINT ( 'NONE',  ( -2.500000000000000444, -15.04166666393548191, -4.330127018922193649 ) ) ;
#27873=CARTESIAN_POINT ( 'NONE',  ( 2.071067811865475505, -163.9375000027311842, -5.000000000000000888 ) ) ;
#27876=CARTESIAN_POINT ( 'NONE',  ( 2.229367062500001939, 6.770833334698928674, 3.861377020970579999 ) ) ;
#27877=CYLINDRICAL_SURFACE ( 'NONE', #57189, 5.000000000000000000 ) ;
#27882=CARTESIAN_POINT ( 'NONE',  ( -1.339745962155660663, -19.79465819873851729, 4.999999999999972466 ) ) ;
#27884=CARTESIAN_POINT ( 'NONE',  ( 4.458734124999999437, -9.812499998634406140, -5.460374474430324690E-16 ) ) ;
#27887=CARTESIAN_POINT ( 'NONE',  ( -2.229367062499996610, -35.39583333196772941, 3.861377020970582219 ) ) ;
#27891=CARTESIAN_POINT ( 'NONE',  ( -1.339745962155613812, 9.794658198738519062, -5.000000000000000000 ) ) ;
#27894=CARTESIAN_POINT ( 'NONE',  ( 4.458734125000001214, 16.10416666803225993, 2.574251347313718519 ) ) ;
#27896=EDGE_CURVE ( 'NONE', #13678, #39270, #17200, .T. ) ;
#27897=CYLINDRICAL_SURFACE ( 'NONE', #35861, 5.000000000000000000 ) ;
#27898=CARTESIAN_POINT ( 'NONE',  ( 4.458734124999998549, -82.97916666530106511, -2.574251347313721627 ) ) ;
#27900=CARTESIAN_POINT ( 'NONE',  ( 2.499999999999998668, 20.79166666939784847, -4.330127018922193649 ) ) ;
#27903=CARTESIAN_POINT ( 'NONE',  ( 2.071067811865508812, -167.1875000000000284, 4.999999999999968026 ) ) ;
#27904=CARTESIAN_POINT ( 'NONE',  ( -6.972266317189433020E-16, -52.25000000000000711, -5.000000000000000000 ) ) ;
#27905=CARTESIAN_POINT ( 'NONE',  ( -4.999999999999999112, -30.91666666666666785, 2.886751345948131764 ) ) ;
#27906=CARTESIAN_POINT ( 'NONE',  ( -4.458734124999999437, -35.39583333196773651, -2.574251347313719407 ) ) ;
#27907=CARTESIAN_POINT ( 'NONE',  ( 5.000000000000000000, 0.5833333333333314830, -2.886751345948130876 ) ) ;
#27908=CARTESIAN_POINT ( 'NONE',  ( -2.499999999999996447, -28.70833333060214798, 4.330127018922195425 ) ) ;
#27909=CARTESIAN_POINT ( 'NONE',  ( 2.229367062500001939, -58.97916666530106511, 3.861377020970579999 ) ) ;
#27910=ORIENTED_EDGE ( 'NONE', *, *, #37339, .T. ) ;
#27912=CARTESIAN_POINT ( 'NONE',  ( 2.229367062500001939, -7.229166665301073103, 3.861377020970579999 ) ) ;
#27914=CARTESIAN_POINT ( 'NONE',  ( 5.000000000000000888, -77.58333333333334281, 2.886751345948126879 ) ) ;
#27915=CARTESIAN_POINT ( 'NONE',  ( -1.339745962155610925, 1.330341803992665106, 5.000000000000000000 ) ) ;
#27917=CARTESIAN_POINT ( 'NONE',  ( 1.060575238724906964E-15, -78.62499999726880162, 5.773502691896257311 ) ) ;
#27918=CARTESIAN_POINT ( 'NONE',  ( 5.000000000000000000, -65.29166666393547303, -2.886751345948130876 ) ) ;
#27919=ORIENTED_EDGE ( 'NONE', *, *, #25475, .T. ) ;
#27922=CARTESIAN_POINT ( 'NONE',  ( -3.152548672688508926E-16, -22.81249999863440436, -5.148502694627439702 ) ) ;
#27923=CARTESIAN_POINT ( 'NONE',  ( 2.229367062500001939, -59.22916666530106511, 3.861377020970579999 ) ) ;
#27924=ORIENTED_EDGE ( 'NONE', *, *, #35458, .T. ) ;
#27926=CARTESIAN_POINT ( 'NONE',  ( -8.190561711645485556E-16, -141.6875000013656063, 4.458734124999999437 ) ) ;
#27928=CARTESIAN_POINT ( 'NONE',  ( 5.000000000000000000, -50.29166666393548013, -2.886751345948130876 ) ) ;
#27935=CARTESIAN_POINT ( 'NONE',  ( -4.458734125000000326, -146.2500000013656063, -1.846868145590735644 ) ) ;
#27939=CARTESIAN_POINT ( 'NONE',  ( 4.458734125000001214, -70.14583333196773651, 2.574251347313718519 ) ) ;
#27942=CARTESIAN_POINT ( 'NONE',  ( -1.846868145590737420, -140.7500000013655779, 4.458734124999997661 ) ) ;
#27946=CARTESIAN_POINT ( 'NONE',  ( -2.071067811865391128, -144.6875000000000568, -5.000000000000086153 ) ) ;
#27951=CARTESIAN_POINT ( 'NONE',  ( -4.458734124999999437, 27.35416666803225993, -2.574251347313719407 ) ) ;
#27952=CARTESIAN_POINT ( 'NONE',  ( 2.499999999999998668, -76.20833333060214443, -4.330127018922193649 ) ) ;
#27959=CARTESIAN_POINT ( 'NONE',  ( 4.458734125000000326, 8.104166668032261711, 2.574251347313718519 ) ) ;
#27961=CARTESIAN_POINT ( 'NONE',  ( -2.229367062499996610, -20.39583333196774007, 3.861377020970582219 ) ) ;
#27963=CARTESIAN_POINT ( 'NONE',  ( -3.152801135295367985, -158.8125000013656063, 3.152801135295367096 ) ) ;
#27964=CARTESIAN_POINT ( 'NONE',  ( 3.061616997868383141E-16, -158.7500000000000000, -5.000000000000000000 ) ) ;
#27967=EDGE_CURVE ( 'NONE', #2367, #27870, #32627, .T. ) ;
#27968=CARTESIAN_POINT ( 'NONE',  ( 0.000000000000000000, -170.0000000000000000, 0.000000000000000000 ) ) ;
#27969=CARTESIAN_POINT ( 'NONE',  ( -4.458734124999997661, -39.22916666530107221, 2.574251347313722516 ) ) ;
#27971=EDGE_CURVE ( 'NONE', #3560, #11132, #11798, .T. ) ;
#27973=CARTESIAN_POINT ( 'NONE',  ( -2.229367062500000163, -65.72916666530106511, -3.861377020970580443 ) ) ;
#27975=CARTESIAN_POINT ( 'NONE',  ( 1.339745962155612702, -57.16965819600733312, -5.000000000000000000 ) ) ;
#27976=CARTESIAN_POINT ( 'NONE',  ( 3.535533905932738197, -152.0000000027312126, -3.535533905932738197 ) ) ;
#27979=CARTESIAN_POINT ( 'NONE',  ( 1.975475456537005874E-15, -89.62499999726880162, 5.000000000000000000 ) ) ;
#27980=CARTESIAN_POINT ( 'NONE',  ( 1.060575238724906964E-15, -12.74999999999999822, 5.773502691896257311 ) ) ;
#27981=CARTESIAN_POINT ( 'NONE',  ( -4.458734124999998549, -18.22916666530107221, 2.574251347313722516 ) ) ;
#27983=CARTESIAN_POINT ( 'NONE',  ( 4.458734124999999437, -75.81249999863440792, -5.460374474430324690E-16 ) ) ;
#27985=CARTESIAN_POINT ( 'NONE',  ( -2.499999999999996447, -12.70833333060214798, 4.330127018922195425 ) ) ;
#27986=CARTESIAN_POINT ( 'NONE',  ( 4.458734124999998549, -45.72916666530106511, -2.574251347313721627 ) ) ;
#27988=CYLINDRICAL_SURFACE ( 'NONE', #53849, 5.000000000000000000 ) ;
#27989=CARTESIAN_POINT ( 'NONE',  ( -3.152548672688508926E-16, 8.187500001365595637, -5.148502694627439702 ) ) ;
#27991=CARTESIAN_POINT ( 'NONE',  ( 1.339745962155612702, -81.16965819600734733, -5.000000000000000000 ) ) ;
#27992=CARTESIAN_POINT ( 'NONE',  ( -5.000000000000000000, -60.08333333333333570, -2.886751345948128211 ) ) ;
#27993=CARTESIAN_POINT ( 'NONE',  ( 1.846868145590735200, -159.5000000013655779, -4.458734125000000326 ) ) ;
#27995=CARTESIAN_POINT ( 'NONE',  ( 1.339745962155615144, -14.70534180126147916, 4.999999999999999112 ) ) ;
#27996=CARTESIAN_POINT ( 'NONE',  ( -4.458734124999999437, -81.31249999863440792, 0.000000000000000000 ) ) ;
#27997=CARTESIAN_POINT ( 'NONE',  ( 5.000000000000000000, -168.0000000000000000, 0.000000000000000000 ) ) ;
#27998=CARTESIAN_POINT ( 'NONE',  ( 9.457646018065525792E-16, -90.06249999863440792, 5.148502694627439702 ) ) ;
#28000=CARTESIAN_POINT ( 'NONE',  ( 4.458734124999999437, -4.062499998634408804, -5.460374474430324690E-16 ) ) ;
#28001=CARTESIAN_POINT ( 'NONE',  ( -2.229367062499996610, -43.39583333196773651, 3.861377020970582219 ) ) ;
#28002=CARTESIAN_POINT ( 'NONE',  ( 1.339745962155612702, -67.16965819600733312, -5.000000000000000000 ) ) ;
#28006=ORIENTED_EDGE ( 'NONE', *, *, #33138, .F. ) ;
#28010=CARTESIAN_POINT ( 'NONE',  ( -2.229367062500000163, -68.72916666530107932, -3.861377020970580443 ) ) ;
#28011=CARTESIAN_POINT ( 'NONE',  ( -8.190561711645485556E-16, -147.9375000013656063, 4.458734124999999437 ) ) ;
#28013=CARTESIAN_POINT ( 'NONE',  ( 3.535533905932738197, -163.8750000000000284, -3.535533905932738197 ) ) ;
#28014=LINE ( 'NONE', #12594, #22467 ) ;
#28017=CARTESIAN_POINT ( 'NONE',  ( 4.458734124999998549, 4.270833334698926897, -2.574251347313721627 ) ) ;
#28018=FACE_OUTER_BOUND ( 'NONE', #61161, .T. ) ;
#28019=CARTESIAN_POINT ( 'NONE',  ( 4.458734124999997661, -154.5000000013656347, 1.846868145590737864 ) ) ;
#28029=ADVANCED_FACE ( 'NONE', ( #38698 ), #4607, .T. ) ;
#28031=CYLINDRICAL_SURFACE ( 'NONE', #12359, 5.000000000000000000 ) ;
#28034=( BOUNDED_CURVE ( )  B_SPLINE_CURVE ( 2, ( #31298, #40640, #17152, #46426, #6875, #46106, #50935, #36776, #6241 ),
 .UNSPECIFIED., .F., .F. ) 
 B_SPLINE_CURVE_WITH_KNOTS ( ( 3, 2, 2, 2, 3 ),
 ( 0.3020833333333333148, 0.3027777777777777568, 0.3041666666666666408, 0.3055555555555555802, 0.3062500000000000222 ),
 .UNSPECIFIED. ) 
 CURVE ( )  GEOMETRIC_REPRESENTATION_ITEM ( )  RATIONAL_B_SPLINE_CURVE ( ( 0.9330127018922194093, 0.9330127018922194093, 1.000000000000000000, 0.8660254037844387076, 1.000000000000000000, 0.8660254037844387076, 1.000000000000000000, 0.9330127018922194093, 0.9330127018922194093 ) ) 
 REPRESENTATION_ITEM ( '' )  );
#28035=CARTESIAN_POINT ( 'NONE',  ( 4.458734125000000326, 25.10416666803225993, 2.574251347313718519 ) ) ;
#28037=CARTESIAN_POINT ( 'NONE',  ( -4.458734124999997661, -2.479166665301069106, 2.574251347313722516 ) ) ;
#28040=CARTESIAN_POINT ( 'NONE',  ( 3.535533905932738197, -142.0000000027311842, -3.535533905932738197 ) ) ;
#28041=FACE_OUTER_BOUND ( 'NONE', #17961, .T. ) ;
#28048=CARTESIAN_POINT ( 'NONE',  ( -1.846868145590734756, -156.3750000013655779, -4.458734124999999437 ) ) ;
#28050=ORIENTED_EDGE ( 'NONE', *, *, #45176, .T. ) ;
#28052=CARTESIAN_POINT ( 'NONE',  ( -2.229367062499996610, 18.60416666803225993, 3.861377020970582219 ) ) ;
#28053=EDGE_CURVE ( 'NONE', #60982, #42868, #33261, .T. ) ;
#28060=ADVANCED_FACE ( 'NONE', ( #28733 ), #4303, .T. ) ;
#28061=CARTESIAN_POINT ( 'NONE',  ( 2.499999999999998668, 1.666666666666666963, -4.330127018922193649 ) ) ;
#28062=CARTESIAN_POINT ( 'NONE',  ( -4.458734124999999437, -63.31249999863440792, 0.000000000000000000 ) ) ;
#28063=CARTESIAN_POINT ( 'NONE',  ( 1.975475456537005874E-15, 6.375000002731185944, 5.000000000000000000 ) ) ;
#28065=CARTESIAN_POINT ( 'NONE',  ( -3.152548672688508926E-16, -29.56249999863440436, -5.148502694627439702 ) ) ;
#28066=CARTESIAN_POINT ( 'NONE',  ( -2.500000000000000444, -38.04166666393548013, -4.330127018922193649 ) ) ;
#28067=DIRECTION ( 'NONE',  ( -0.000000000000000000, 1.000000000000000000, -0.000000000000000000 ) ) ;
#28069=CARTESIAN_POINT ( 'NONE',  ( 5.000000000000000000, -46.41666666666666430, -2.886751345948129988 ) ) ;
#28071=CARTESIAN_POINT ( 'NONE',  ( 2.499999999999998668, -26.20833333060214798, -4.330127018922193649 ) ) ;
#28074=CARTESIAN_POINT ( 'NONE',  ( -4.458734124999999437, -64.31249999863440792, 0.000000000000000000 ) ) ;
#28075=CARTESIAN_POINT ( 'NONE',  ( 4.458734125000000326, -148.6250000013655779, -1.846868145590734978 ) ) ;
#28076=CARTESIAN_POINT ( 'NONE',  ( -4.458734124999999437, -77.31249999863440792, 0.000000000000000000 ) ) ;
#28078=CARTESIAN_POINT ( 'NONE',  ( 4.458734124999998549, -26.97916666530107221, -2.574251347313721627 ) ) ;
#28079=CARTESIAN_POINT ( 'NONE',  ( 5.000000000000000000, -68.37499999726881583, -6.123233995736766282E-16 ) ) ;
#28081=CARTESIAN_POINT ( 'NONE',  ( 6.123233995736766282E-16, -170.0000000000000000, -5.000000000000000000 ) ) ;
#28082=ORIENTED_EDGE ( 'NONE', *, *, #2095, .F. ) ;
#28084=DIRECTION ( 'NONE',  ( -0.000000000000000000, 1.000000000000000000, -0.000000000000000000 ) ) ;
#28085=DIRECTION ( 'NONE',  ( 0.000000000000000000, 0.000000000000000000, 1.000000000000000000 ) ) ;
#28086=ORIENTED_EDGE ( 'NONE', *, *, #24496, .F. ) ;
#28087=DIRECTION ( 'NONE',  ( -0.000000000000000000, 1.000000000000000000, -0.000000000000000000 ) ) ;
#28088=CARTESIAN_POINT ( 'NONE',  ( -4.458734124999998549, -53.47916666530106511, 2.574251347313722516 ) ) ;
#28093=CARTESIAN_POINT ( 'NONE',  ( -2.229367062499996610, 20.85416666803226349, 3.861377020970582219 ) ) ;
#28096=CARTESIAN_POINT ( 'NONE',  ( -8.190561711645485556E-16, -168.6875000013656063, 4.458734124999999437 ) ) ;
#28097=ORIENTED_EDGE ( 'NONE', *, *, #52242, .F. ) ;
#28103=CYLINDRICAL_SURFACE ( 'NONE', #58312, 5.000000000000000000 ) ;
#28106=CARTESIAN_POINT ( 'NONE',  ( 5.000000000000000000, -20.49999999999999645, -6.123233995736766282E-16 ) ) ;
#28108=DIRECTION ( 'NONE',  ( -0.000000000000000000, 1.000000000000000000, -0.000000000000000000 ) ) ;
#28109=CARTESIAN_POINT ( 'NONE',  ( 2.500000000000002220, -18.54166666393547658, 4.330127018922192761 ) ) ;
#28115=CARTESIAN_POINT ( 'NONE',  ( -9.184850993605147944E-16, -154.3750000027311842, 5.000000000000000000 ) ) ;
#28121=CARTESIAN_POINT ( 'NONE',  ( 2.071067811865476394, -148.1875000000000000, 5.000000000000000000 ) ) ;
#28124=CARTESIAN_POINT ( 'NONE',  ( -8.190561711645485556E-16, -167.9375000013655779, 4.458734124999999437 ) ) ;
#28125=CARTESIAN_POINT ( 'NONE',  ( 4.458734125000000326, -28.89583333196774007, 2.574251347313718519 ) ) ;
#28129=CARTESIAN_POINT ( 'NONE',  ( -4.458734125000001214, -147.8750000013656063, 1.846868145590734089 ) ) ;
#28132=CARTESIAN_POINT ( 'NONE',  ( -2.229367062500000163, -55.72916666530107221, -3.861377020970580443 ) ) ;
#28135=CARTESIAN_POINT ( 'NONE',  ( 5.000000000000000888, 19.41666666666666075, 2.886751345948126879 ) ) ;
#28137=CARTESIAN_POINT ( 'NONE',  ( 6.123233995736766282E-16, -170.0000000000000000, -5.000000000000000000 ) ) ;
#28138=CARTESIAN_POINT ( 'NONE',  ( 4.458734125000001214, 1.104166668032261711, 2.574251347313718519 ) ) ;
#28139=CARTESIAN_POINT ( 'NONE',  ( 1.339745962155615144, -48.70534180126148271, 4.999999999999999112 ) ) ;
#28140=CARTESIAN_POINT ( 'NONE',  ( 0.000000000000000000, -170.0000000000000000, 0.000000000000000000 ) ) ;
#28141=CARTESIAN_POINT ( 'NONE',  ( 2.229367062499998831, 10.10416666803225993, -3.861377020970580887 ) ) ;
#28146=CARTESIAN_POINT ( 'NONE',  ( -2.229367062500000163, -49.47916666530107221, -3.861377020970580443 ) ) ;
#28147=CARTESIAN_POINT ( 'NONE',  ( -3.152801135295367096, -159.3125000013656063, -3.152801135295367541 ) ) ;
#28149=( BOUNDED_CURVE ( )  B_SPLINE_CURVE ( 2, ( #47599, #28605, #38270, #23482, #57894, #43703, #33437, #43085, #13818 ),
 .UNSPECIFIED., .F., .F. ) 
 B_SPLINE_CURVE_WITH_KNOTS ( ( 3, 2, 2, 2, 3 ),
 ( 0.1395833333333333370, 0.1402777777777777790, 0.1416666666666666630, 0.1430555555555555469, 0.1437499999999999889 ),
 .UNSPECIFIED. ) 
 CURVE ( )  GEOMETRIC_REPRESENTATION_ITEM ( )  RATIONAL_B_SPLINE_CURVE ( ( 0.9330127018922194093, 0.9330127018922194093, 1.000000000000000000, 0.8660254037844387076, 1.000000000000000000, 0.8660254037844387076, 1.000000000000000000, 0.9330127018922194093, 0.9330127018922194093 ) ) 
 REPRESENTATION_ITEM ( '' )  );
#28150=CARTESIAN_POINT ( 'NONE',  ( -5.000000000000000000, -47.87499999726880873, 0.000000000000000000 ) ) ;
#28151=EDGE_LOOP ( 'NONE', ( #21231, #57660, #30225, #63141 ) ) ;
#28152=CARTESIAN_POINT ( 'NONE',  ( -2.229367062500000163, -22.47916666530107221, -3.861377020970580443 ) ) ;
#28155=CARTESIAN_POINT ( 'NONE',  ( -2.071067811865562991, -142.4375000027312126, 4.999999999999913847 ) ) ;
#28156=CARTESIAN_POINT ( 'NONE',  ( -4.458734124999999437, -160.9375000013655779, -5.460374474430324690E-16 ) ) ;
#28159=EDGE_CURVE ( 'NONE', #859, #57124, #18383, .T. ) ;
#28160=CARTESIAN_POINT ( 'NONE',  ( 9.457646018065525792E-16, -38.31249999863441502, 5.148502694627439702 ) ) ;
#28167=CARTESIAN_POINT ( 'NONE',  ( -2.229367062499996610, -86.39583333196773651, 3.861377020970582219 ) ) ;
#28170=CARTESIAN_POINT ( 'NONE',  ( 5.000000000000000000, -57.41666666666667140, -2.886751345948130876 ) ) ;
#28174=CARTESIAN_POINT ( 'NONE',  ( 0.000000000000000000, -170.0000000000000000, 0.000000000000000000 ) ) ;
#28180=CARTESIAN_POINT ( 'NONE',  ( 4.458734125000001214, -87.14583333196772230, 2.574251347313718519 ) ) ;
#28183=EDGE_LOOP ( 'NONE', ( #2008, #63517, #13344, #51970 ) ) ;
#28184=CARTESIAN_POINT ( 'NONE',  ( -3.535533905932738641, -155.5000000027312126, 3.535533905932737309 ) ) ;
#28186=CARTESIAN_POINT ( 'NONE',  ( 5.000000000000000888, -166.0625000027312410, -2.071067811865475505 ) ) ;
#28190=AXIS2_PLACEMENT_3D ( 'NONE', #31960, #36471, #57059 ) ;
#28196=CARTESIAN_POINT ( 'NONE',  ( 0.000000000000000000, -170.0000000000000000, 5.000000000000000000 ) ) ;
#28197=CARTESIAN_POINT ( 'NONE',  ( -3.152548672688508926E-16, -14.56249999863440259, -5.148502694627439702 ) ) ;
#28200=CARTESIAN_POINT ( 'NONE',  ( -2.229367062500000163, -39.72916666530107221, -3.861377020970580443 ) ) ;
#28201=( BOUNDED_CURVE ( )  B_SPLINE_CURVE ( 2, ( #6404, #40476, #46265, #1585, #21185, #2224, #13118, #37558, #42377 ),
 .UNSPECIFIED., .F., .F. ) 
 B_SPLINE_CURVE_WITH_KNOTS ( ( 3, 2, 2, 2, 3 ),
 ( 0.7979166666666667185, 0.7986111111111111605, 0.8000000000000000444, 0.8013888888888889284, 0.8020833333333333703 ),
 .UNSPECIFIED. ) 
 CURVE ( )  GEOMETRIC_REPRESENTATION_ITEM ( )  RATIONAL_B_SPLINE_CURVE ( ( 0.9330127018922194093, 0.9330127018922194093, 1.000000000000000000, 0.8660254037844387076, 1.000000000000000000, 0.8660254037844387076, 1.000000000000000000, 0.9330127018922194093, 0.9330127018922194093 ) ) 
 REPRESENTATION_ITEM ( '' )  );
#28204=DIRECTION ( 'NONE',  ( -0.000000000000000000, 1.000000000000000000, -0.000000000000000000 ) ) ;
#28207=CARTESIAN_POINT ( 'NONE',  ( 9.457646018065525792E-16, 15.93750000136559564, 5.148502694627439702 ) ) ;
#28209=CARTESIAN_POINT ( 'NONE',  ( -5.000000000000000000, -64.87499999726881583, 0.000000000000000000 ) ) ;
#28210=CARTESIAN_POINT ( 'NONE',  ( 4.458734124999998549, -84.97916666530107932, -2.574251347313721627 ) ) ;
#28212=CARTESIAN_POINT ( 'NONE',  ( 2.500000000000002220, 12.45833333606451809, 4.330127018922192761 ) ) ;
#28215=CARTESIAN_POINT ( 'NONE',  ( -5.000000000000000000, 16.00000000000000000, 0.000000000000000000 ) ) ;
#28217=CARTESIAN_POINT ( 'NONE',  ( 1.060575238724906964E-15, -27.74999999999999645, 5.773502691896257311 ) ) ;
#28218=CARTESIAN_POINT ( 'NONE',  ( -2.229367062499996610, -32.14583333196773651, 3.861377020970582219 ) ) ;
#28220=CARTESIAN_POINT ( 'NONE',  ( 5.000000000000000000, -35.29166666393547303, -2.886751345948129988 ) ) ;
#28221=CARTESIAN_POINT ( 'NONE',  ( -2.229367062500000163, -61.47916666530106511, -3.861377020970580443 ) ) ;
#28222=ORIENTED_EDGE ( 'NONE', *, *, #814, .F. ) ;
#28224=CARTESIAN_POINT ( 'NONE',  ( -2.229367062500000163, -7.729166665301073991, -3.861377020970580443 ) ) ;
#28225=ORIENTED_EDGE ( 'NONE', *, *, #12141, .F. ) ;
#28226=CARTESIAN_POINT ( 'NONE',  ( -3.535250795749689387E-16, -77.25000000000000000, -5.773502691896257311 ) ) ;
#28229=( BOUNDED_CURVE ( )  B_SPLINE_CURVE ( 2, ( #40471, #61383, #45624, #61069, #16990, #1267, #1579, #35661, #22138 ),
 .UNSPECIFIED., .F., .F. ) 
 B_SPLINE_CURVE_WITH_KNOTS ( ( 3, 2, 2, 2, 3 ),
 ( 0.8020833333333333703, 0.8027777777777778123, 0.8041666666666666963, 0.8055555555555555802, 0.8062500000000000222 ),
 .UNSPECIFIED. ) 
 CURVE ( )  GEOMETRIC_REPRESENTATION_ITEM ( )  RATIONAL_B_SPLINE_CURVE ( ( 0.9330127018922194093, 0.9330127018922194093, 1.000000000000000000, 0.8660254037844387076, 1.000000000000000000, 0.8660254037844387076, 1.000000000000000000, 0.9330127018922194093, 0.9330127018922194093 ) ) 
 REPRESENTATION_ITEM ( '' )  );
#28230=CARTESIAN_POINT ( 'NONE',  ( 5.000000000000000888, -75.45833333060214443, 2.886751345948126879 ) ) ;
#28231=CARTESIAN_POINT ( 'NONE',  ( 1.339745962155612702, -13.29465819873852084, -5.000000000000000000 ) ) ;
#28232=VERTEX_POINT ( 'NONE', #24552 ) ;
#28234=ADVANCED_FACE ( 'NONE', ( #20695 ), #30646, .T. ) ;
#28235=CARTESIAN_POINT ( 'NONE',  ( 4.458734125000001214, -23.14583333196773651, 2.574251347313718519 ) ) ;
#28236=CARTESIAN_POINT ( 'NONE',  ( -2.229367062499996610, -54.39583333196773651, 3.861377020970582219 ) ) ;
#28237=ORIENTED_EDGE ( 'NONE', *, *, #31900, .T. ) ;
#28240=CARTESIAN_POINT ( 'NONE',  ( -8.190561711645485556E-16, -166.9375000013655779, 4.458734124999999437 ) ) ;
#28243=ORIENTED_EDGE ( 'NONE', *, *, #13736, .F. ) ;
#28250=CARTESIAN_POINT ( 'NONE',  ( 4.458734124999999437, -144.7500000013656063, 1.846868145590737864 ) ) ;
#28252=EDGE_CURVE ( 'NONE', #24591, #53169, #734, .T. ) ;
#28255=CARTESIAN_POINT ( 'NONE',  ( -3.152548672688508926E-16, -70.81249999863440792, -5.148502694627439702 ) ) ;
#28257=DIRECTION ( 'NONE',  ( 0.000000000000000000, 0.000000000000000000, 1.000000000000000000 ) ) ;
#28258=CARTESIAN_POINT ( 'NONE',  ( -8.190561711645485556E-16, -139.6875000013656063, 4.458734124999999437 ) ) ;
#28260=EDGE_LOOP ( 'NONE', ( #56490, #5778, #11098, #14617 ) ) ;
#28267=CARTESIAN_POINT ( 'NONE',  ( 4.458734125000000326, 22.85416666803225993, 2.574251347313718519 ) ) ;
#28268=EDGE_CURVE ( 'NONE', #62891, #3107, #45443, .T. ) ;
#28274=CARTESIAN_POINT ( 'NONE',  ( -3.152548672688508926E-16, 4.437500001365595637, -5.148502694627439702 ) ) ;
#28275=AXIS2_PLACEMENT_3D ( 'NONE', #31326, #2098, #21700 ) ;
#28277=CARTESIAN_POINT ( 'NONE',  ( 9.457646018065525792E-16, -22.31249999863440792, 5.148502694627439702 ) ) ;
#28278=CARTESIAN_POINT ( 'NONE',  ( 2.730187237215162345E-16, -156.1875000013655779, -4.458734124999999437 ) ) ;
#28282=CARTESIAN_POINT ( 'NONE',  ( -4.458734124999999437, 28.68750000136559208, 0.000000000000000000 ) ) ;
#28283=CARTESIAN_POINT ( 'NONE',  ( -2.229367062500000163, -41.47916666530107932, -3.861377020970580443 ) ) ;
#28284=CARTESIAN_POINT ( 'NONE',  ( -4.999999999999998224, -83.91666666666667140, 2.886751345948131764 ) ) ;
#28287=CARTESIAN_POINT ( 'NONE',  ( -4.458734124999997661, -69.47916666530107932, 2.574251347313722516 ) ) ;
#28290=DIRECTION ( 'NONE',  ( -0.000000000000000000, 1.000000000000000000, -0.000000000000000000 ) ) ;
#28291=ORIENTED_EDGE ( 'NONE', *, *, #40167, .F. ) ;
#28292=CARTESIAN_POINT ( 'NONE',  ( -2.500000000000000444, 14.95833333606451809, -4.330127018922193649 ) ) ;
#28293=CARTESIAN_POINT ( 'NONE',  ( 5.000000000000000000, 2.625000002731185500, -6.123233995736766282E-16 ) ) ;
#28294=CARTESIAN_POINT ( 'NONE',  ( 1.060575238724906964E-15, -10.75000000000000178, 5.773502691896257311 ) ) ;
#28295=CARTESIAN_POINT ( 'NONE',  ( 9.457646018065525792E-16, -19.06249999863440792, 5.148502694627439702 ) ) ;
#28296=CARTESIAN_POINT ( 'NONE',  ( 9.457646018065525792E-16, -79.06249999863440792, 5.148502694627439702 ) ) ;
#28297=CARTESIAN_POINT ( 'NONE',  ( 5.000000000000000000, -59.29166666393547303, -2.886751345948130876 ) ) ;
#28298=CARTESIAN_POINT ( 'NONE',  ( 2.499999999999998668, -15.20833333060214443, -4.330127018922193649 ) ) ;
#28299=CARTESIAN_POINT ( 'NONE',  ( -4.458734124999999437, -42.31249999863440081, 0.000000000000000000 ) ) ;
#28300=ORIENTED_EDGE ( 'NONE', *, *, #31974, .F. ) ;
#28302=CARTESIAN_POINT ( 'NONE',  ( -2.229367062500000163, 6.270833334698928674, -3.861377020970580443 ) ) ;
#28304=CARTESIAN_POINT ( 'NONE',  ( -2.499999999999996447, -59.83333333333333570, 4.330127018922195425 ) ) ;
#28305=CARTESIAN_POINT ( 'NONE',  ( -4.458734125000000326, -158.2500000013656063, -1.846868145590735644 ) ) ;
#28308=CARTESIAN_POINT ( 'NONE',  ( 5.000000000000000888, -166.9375000000000284, -2.071067811865475505 ) ) ;
#28309=CARTESIAN_POINT ( 'NONE',  ( 3.061616997868383141E-16, -167.7500000000000000, -5.000000000000000000 ) ) ;
#28312=CARTESIAN_POINT ( 'NONE',  ( -2.229367062500000163, -3.729166665301070438, -3.861377020970580443 ) ) ;
#28313=CARTESIAN_POINT ( 'NONE',  ( -4.458734124999999437, -38.56249999863440081, 0.000000000000000000 ) ) ;
#28314=EDGE_CURVE ( 'NONE', #30756, #52679, #24954, .T. ) ;
#28315=EDGE_CURVE ( 'NONE', #11358, #8866, #40168, .T. ) ;
#28317=CARTESIAN_POINT ( 'NONE',  ( -8.190561711645485556E-16, -153.6875000013656063, 4.458734124999999437 ) ) ;
#28319=CARTESIAN_POINT ( 'NONE',  ( 5.000000000000000000, -167.1250000027312126, 0.000000000000000000 ) ) ;
#28321=CARTESIAN_POINT ( 'NONE',  ( -2.071067811865604735, -148.4375000027312410, 4.999999999999872990 ) ) ;
#28322=CARTESIAN_POINT ( 'NONE',  ( 1.975475456537005874E-15, -2.624999997268813168, 5.000000000000000000 ) ) ;
#28323=CARTESIAN_POINT ( 'NONE',  ( 2.229367062500001939, -69.22916666530107932, 3.861377020970579999 ) ) ;
#28324=CARTESIAN_POINT ( 'NONE',  ( -8.190561711645485556E-16, -144.9375000013656063, 4.458734124999999437 ) ) ;
#28325=ORIENTED_EDGE ( 'NONE', *, *, #60075, .T. ) ;
#28332=CARTESIAN_POINT ( 'NONE',  ( 9.457646018065525792E-16, 4.937500001365596525, 5.148502694627439702 ) ) ;
#28333=CARTESIAN_POINT ( 'NONE',  ( -1.339745962155610925, -79.79465819873850307, 5.000000000000000000 ) ) ;
#28334=CARTESIAN_POINT ( 'NONE',  ( 4.458734124999997661, -151.5000000013655779, 1.846868145590737864 ) ) ;
#28338=CARTESIAN_POINT ( 'NONE',  ( -1.339745962155564296, -25.20534180126148271, -5.000000000000028422 ) ) ;
#28343=DIRECTION ( 'NONE',  ( -0.000000000000000000, 1.000000000000000000, -0.000000000000000000 ) ) ;
#28345=CARTESIAN_POINT ( 'NONE',  ( -4.999999999999998224, -71.91666666666667140, 2.886751345948131764 ) ) ;
#28346=CARTESIAN_POINT ( 'NONE',  ( -4.458734124999997661, 22.77083333469892068, 2.574251347313722516 ) ) ;
#28348=CARTESIAN_POINT ( 'NONE',  ( -2.229367062499996610, -4.395833331967740065, 3.861377020970582219 ) ) ;
#28349=CARTESIAN_POINT ( 'NONE',  ( -2.499999999999996447, -62.83333333333333570, 4.330127018922195425 ) ) ;
#28351=CARTESIAN_POINT ( 'NONE',  ( -5.000000000000000888, -140.6875000027311842, -2.071067811865475949 ) ) ;
#28358=CARTESIAN_POINT ( 'NONE',  ( 3.152801135295367541, -157.5625000013656063, -3.152801135295367541 ) ) ;
#28360=CARTESIAN_POINT ( 'NONE',  ( 3.061616997868383141E-16, -147.7500000000000284, -5.000000000000000000 ) ) ;
#28361=VERTEX_POINT ( 'NONE', #36115 ) ;
#28362=CARTESIAN_POINT ( 'NONE',  ( -2.229367062500000163, 18.27083333469892779, -3.861377020970580443 ) ) ;
#28367=CARTESIAN_POINT ( 'NONE',  ( 1.339745962155612702, 12.70534180126147916, -5.000000000000000000 ) ) ;
#28368=CARTESIAN_POINT ( 'NONE',  ( -2.500000000000000444, 3.833333333333334370, -4.330127018922193649 ) ) ;
#28369=AXIS2_PLACEMENT_3D ( 'NONE', #24340, #28843, #19509 ) ;
#28370=CARTESIAN_POINT ( 'NONE',  ( -2.229367062500000163, -60.47916666530106511, -3.861377020970580443 ) ) ;
#28371=AXIS2_PLACEMENT_3D ( 'NONE', #44546, #16249, #24617 ) ;
#28373=CARTESIAN_POINT ( 'NONE',  ( -3.535250795749689387E-16, 1.875000002731185056, -5.773502691896257311 ) ) ;
#28374=CARTESIAN_POINT ( 'NONE',  ( 2.229367062499998831, -27.64583333196774007, -3.861377020970580887 ) ) ;
#28376=DIRECTION ( 'NONE',  ( -0.000000000000000000, 1.000000000000000000, -0.000000000000000000 ) ) ;
#28377=( BOUNDED_CURVE ( )  B_SPLINE_CURVE ( 2, ( #33453, #53070, #28622, #4195, #23808, #43410, #38581, #33766, #59819 ),
 .UNSPECIFIED., .F., .F. ) 
 B_SPLINE_CURVE_WITH_KNOTS ( ( 3, 2, 2, 2, 3 ),
 ( 0.9062500000000000000, 0.9069444444444444420, 0.9083333333333333259, 0.9097222222222222099, 0.9104166666666666519 ),
 .UNSPECIFIED. ) 
 CURVE ( )  GEOMETRIC_REPRESENTATION_ITEM ( )  RATIONAL_B_SPLINE_CURVE ( ( 0.9330127018922194093, 0.9330127018922194093, 1.000000000000000000, 0.8660254037844387076, 1.000000000000000000, 0.8660254037844387076, 1.000000000000000000, 0.9330127018922194093, 0.9330127018922194093 ) ) 
 REPRESENTATION_ITEM ( '' )  );
#28379=CARTESIAN_POINT ( 'NONE',  ( -5.000000000000000000, -44.00000000000000000, 0.000000000000000000 ) ) ;
#28380=DIRECTION ( 'NONE',  ( -0.000000000000000000, 1.000000000000000000, -0.000000000000000000 ) ) ;
#28381=( BOUNDED_CURVE ( )  B_SPLINE_CURVE ( 2, ( #38494, #4405, #39752, #24342, #5362, #9233, #28846, #63271, #63590 ),
 .UNSPECIFIED., .F., .F. ) 
 B_SPLINE_CURVE_WITH_KNOTS ( ( 3, 2, 2, 2, 3 ),
 ( 0.9604166666666666963, 0.9611111111111111382, 0.9625000000000000222, 0.9638888888888889062, 0.9645833333333333481 ),
 .UNSPECIFIED. ) 
 CURVE ( )  GEOMETRIC_REPRESENTATION_ITEM ( )  RATIONAL_B_SPLINE_CURVE ( ( 0.9330127018922194093, 0.9330127018922194093, 1.000000000000000000, 0.8660254037844387076, 1.000000000000000000, 0.8660254037844387076, 1.000000000000000000, 0.9330127018922194093, 0.9330127018922194093 ) ) 
 REPRESENTATION_ITEM ( '' )  );
#28383=CARTESIAN_POINT ( 'NONE',  ( 1.975475456537005874E-15, -4.624999997268815832, 5.000000000000000000 ) ) ;
#28384=CARTESIAN_POINT ( 'NONE',  ( 4.458734124999999437, -66.81249999863440792, -5.460374474430324690E-16 ) ) ;
#28385=CARTESIAN_POINT ( 'NONE',  ( -4.458734125000001214, -146.1250000013655779, 1.846868145590734089 ) ) ;
#28386=CARTESIAN_POINT ( 'NONE',  ( -4.458734124999998549, -77.22916666530106511, 2.574251347313722516 ) ) ;
#28388=CARTESIAN_POINT ( 'NONE',  ( -4.458734124999999437, -26.56249999863440792, 0.000000000000000000 ) ) ;
#28389=CARTESIAN_POINT ( 'NONE',  ( -2.499999999999996447, -65.70833333060213022, 4.330127018922195425 ) ) ;
#28391=EDGE_LOOP ( 'NONE', ( #50363, #47761, #53997, #9656 ) ) ;
#28392=CARTESIAN_POINT ( 'NONE',  ( 1.339745962155615144, -1.705341801261478274, 4.999999999999999112 ) ) ;
#28393=ORIENTED_EDGE ( 'NONE', *, *, #9167, .T. ) ;
#28395=CARTESIAN_POINT ( 'NONE',  ( -4.999999999999998224, 8.208333336064518093, 2.886751345948131764 ) ) ;
#28397=ORIENTED_EDGE ( 'NONE', *, *, #19163, .T. ) ;
#28399=CARTESIAN_POINT ( 'NONE',  ( 0.000000000000000000, -170.0000000000000000, 5.000000000000000000 ) ) ;
#28400=CARTESIAN_POINT ( 'NONE',  ( -4.458734124999998549, -54.47916666530107932, 2.574251347313722516 ) ) ;
#28401=EDGE_CURVE ( 'NONE', #10944, #37366, #35285, .T. ) ;
#28405=EDGE_CURVE ( 'NONE', #3107, #56488, #33226, .T. ) ;
#28406=CARTESIAN_POINT ( 'NONE',  ( 4.458734124999999437, 16.18750000136559564, -5.460374474430324690E-16 ) ) ;
#28408=LINE ( 'NONE', #58003, #19217 ) ;
#28409=CARTESIAN_POINT ( 'NONE',  ( 4.458734124999999437, -164.4375000013655779, 0.000000000000000000 ) ) ;
#28410=ORIENTED_EDGE ( 'NONE', *, *, #4006, .T. ) ;
#28411=EDGE_CURVE ( 'NONE', #18181, #50566, #60571, .T. ) ;
#28413=FACE_OUTER_BOUND ( 'NONE', #25602, .T. ) ;
#28417=EDGE_CURVE ( 'NONE', #57628, #23954, #6935, .T. ) ;
#28420=AXIS2_PLACEMENT_3D ( 'NONE', #18313, #37938, #43380 ) ;
#28422=CARTESIAN_POINT ( 'NONE',  ( -4.999999999999998224, 6.083333333333333037, 2.886751345948131764 ) ) ;
#28429=( BOUNDED_CURVE ( )  B_SPLINE_CURVE ( 2, ( #10025, #19995, #24826, #39603, #54419, #29957, #25139, #22702, #27821 ),
 .UNSPECIFIED., .F., .F. ) 
 B_SPLINE_CURVE_WITH_KNOTS ( ( 3, 2, 2, 2, 3 ),
 ( 0.3854166666666666852, 0.3861111111111111271, 0.3875000000000000111, 0.3888888888888888951, 0.3895833333333333370 ),
 .UNSPECIFIED. ) 
 CURVE ( )  GEOMETRIC_REPRESENTATION_ITEM ( )  RATIONAL_B_SPLINE_CURVE ( ( 0.9330127018922194093, 0.9330127018922194093, 1.000000000000000000, 0.8660254037844387076, 1.000000000000000000, 0.8660254037844387076, 1.000000000000000000, 0.9330127018922194093, 0.9330127018922194093 ) ) 
 REPRESENTATION_ITEM ( '' )  );
#28432=CARTESIAN_POINT ( 'NONE',  ( -3.535533905932737309, -151.7500000027312126, -3.535533905932738197 ) ) ;
#28433=ORIENTED_EDGE ( 'NONE', *, *, #48778, .F. ) ;
#28438=CARTESIAN_POINT ( 'NONE',  ( -2.071067811865475061, -144.6875000000000853, -5.000000000000000888 ) ) ;
#28441=CARTESIAN_POINT ( 'NONE',  ( -4.458734124999999437, -28.31249999863440081, 0.000000000000000000 ) ) ;
#28443=CARTESIAN_POINT ( 'NONE',  ( -6.972266317189433020E-16, 18.87500000273119127, -5.000000000000000000 ) ) ;
#28445=CARTESIAN_POINT ( 'NONE',  ( -4.458734125000000326, -146.0000000013655779, -1.846868145590735644 ) ) ;
#28447=DIRECTION ( 'NONE',  ( 0.000000000000000000, 0.000000000000000000, 1.000000000000000000 ) ) ;
#28448=CARTESIAN_POINT ( 'NONE',  ( -2.229367062499996610, -59.39583333196773651, 3.861377020970582219 ) ) ;
#28450=CARTESIAN_POINT ( 'NONE',  ( 0.000000000000000000, -170.0000000000000000, 5.000000000000000000 ) ) ;
#28451=CARTESIAN_POINT ( 'NONE',  ( 2.499999999999998668, 18.66666666666666430, -4.330127018922193649 ) ) ;
#28452=CARTESIAN_POINT ( 'NONE',  ( -5.000000000000000000, -36.87499999726881583, 0.000000000000000000 ) ) ;
#28453=CARTESIAN_POINT ( 'NONE',  ( 4.458734124999999437, 1.187500001365596081, -5.460374474430324690E-16 ) ) ;
#28456=CARTESIAN_POINT ( 'NONE',  ( 9.457646018065525792E-16, 11.68750000136559564, 5.148502694627439702 ) ) ;
#28457=DIRECTION ( 'NONE',  ( -0.000000000000000000, 1.000000000000000000, -0.000000000000000000 ) ) ;
#28458=VERTEX_POINT ( 'NONE', #33190 ) ;
#28461=CARTESIAN_POINT ( 'NONE',  ( -3.152548672688508926E-16, -51.56249999863441502, -5.148502694627439702 ) ) ;
#28462=CARTESIAN_POINT ( 'NONE',  ( -1.846868145590734756, -161.3750000013656063, -4.458734125000000326 ) ) ;
#28464=VECTOR ( 'NONE', #25340, 1000.000000000000000 ) ;
#28465=CARTESIAN_POINT ( 'NONE',  ( 2.500000000000002220, -50.54166666393547303, 4.330127018922192761 ) ) ;
#28466=ORIENTED_EDGE ( 'NONE', *, *, #10634, .T. ) ;
#28468=CARTESIAN_POINT ( 'NONE',  ( -2.229367062500000163, -23.47916666530107221, -3.861377020970580443 ) ) ;
#28471=CARTESIAN_POINT ( 'NONE',  ( -3.535533905932737309, -142.7500000027311842, -3.535533905932738197 ) ) ;
#28472=CARTESIAN_POINT ( 'NONE',  ( 4.458734124999999437, -159.4375000013655779, 0.000000000000000000 ) ) ;
#28476=CARTESIAN_POINT ( 'NONE',  ( -2.229367062499996610, -35.39583333196772941, 3.861377020970582219 ) ) ;
#28477=ORIENTED_EDGE ( 'NONE', *, *, #52830, .F. ) ;
#28481=VERTEX_POINT ( 'NONE', #38622 ) ;
#28483=CARTESIAN_POINT ( 'NONE',  ( -3.152548672688508926E-16, -83.81249999863439371, -5.148502694627439702 ) ) ;
#28485=CARTESIAN_POINT ( 'NONE',  ( -6.972266317189433020E-16, -4.124999997268814056, -5.000000000000000000 ) ) ;
#28495=DIRECTION ( 'NONE',  ( -0.000000000000000000, 1.000000000000000000, -0.000000000000000000 ) ) ;
#28496=CARTESIAN_POINT ( 'NONE',  ( 4.458734124999999437, -82.06249999863440792, -5.460374474430324690E-16 ) ) ;
#28499=ORIENTED_EDGE ( 'NONE', *, *, #16940, .F. ) ;
#28500=CARTESIAN_POINT ( 'NONE',  ( 2.500000000000002220, -9.541666663935483683, 4.330127018922192761 ) ) ;
#28502=CARTESIAN_POINT ( 'NONE',  ( -9.184850993605147944E-16, -164.3750000027311842, 5.000000000000000000 ) ) ;
#28507=( BOUNDED_CURVE ( )  B_SPLINE_CURVE ( 2, ( #11229, #32112, #16700, #7690, #50483, #50798, #6734, #6422, #26666 ),
 .UNSPECIFIED., .F., .F. ) 
 B_SPLINE_CURVE_WITH_KNOTS ( ( 3, 2, 2, 2, 3 ),
 ( 0.3270833333333333370, 0.3277777777777777790, 0.3291666666666666630, 0.3305555555555555469, 0.3312499999999999889 ),
 .UNSPECIFIED. ) 
 CURVE ( )  GEOMETRIC_REPRESENTATION_ITEM ( )  RATIONAL_B_SPLINE_CURVE ( ( 0.9330127018922194093, 0.9330127018922194093, 1.000000000000000000, 0.8660254037844387076, 1.000000000000000000, 0.8660254037844387076, 1.000000000000000000, 0.9330127018922194093, 0.9330127018922194093 ) ) 
 REPRESENTATION_ITEM ( '' )  );
#28515=CARTESIAN_POINT ( 'NONE',  ( 2.229367062500001939, -16.97916666530106866, 3.861377020970579999 ) ) ;
#28516=CARTESIAN_POINT ( 'NONE',  ( 2.500000000000002220, -71.66666666666667140, 4.330127018922192761 ) ) ;
#28517=ORIENTED_EDGE ( 'NONE', *, *, #21575, .F. ) ;
#28518=CARTESIAN_POINT ( 'NONE',  ( 4.458734125000000326, -43.14583333196773651, 2.574251347313718519 ) ) ;
#28520=CARTESIAN_POINT ( 'NONE',  ( 5.000000000000000888, -83.45833333060213022, 2.886751345948126879 ) ) ;
#28525=CARTESIAN_POINT ( 'NONE',  ( 2.229367062499998831, 13.35416666803226171, -3.861377020970580887 ) ) ;
#28526=( BOUNDED_CURVE ( )  B_SPLINE_CURVE ( 2, ( #8684, #18014, #13197, #28297, #32819, #47910, #11136, #18652, #55217 ),
 .UNSPECIFIED., .F., .F. ) 
 B_SPLINE_CURVE_WITH_KNOTS ( ( 3, 2, 2, 2, 3 ),
 ( 0.7354166666666667185, 0.7361111111111111605, 0.7375000000000000444, 0.7388888888888889284, 0.7395833333333333703 ),
 .UNSPECIFIED. ) 
 CURVE ( )  GEOMETRIC_REPRESENTATION_ITEM ( )  RATIONAL_B_SPLINE_CURVE ( ( 0.9330127018922194093, 0.9330127018922194093, 1.000000000000000000, 0.8660254037844387076, 1.000000000000000000, 0.8660254037844387076, 1.000000000000000000, 0.9330127018922194093, 0.9330127018922194093 ) ) 
 REPRESENTATION_ITEM ( '' )  );
#28528=CARTESIAN_POINT ( 'NONE',  ( 4.458734124999998549, -88.97916666530106511, -2.574251347313721627 ) ) ;
#28530=CARTESIAN_POINT ( 'NONE',  ( -2.499999999999996447, 16.29166666939785202, 4.330127018922195425 ) ) ;
#28531=ORIENTED_EDGE ( 'NONE', *, *, #3320, .T. ) ;
#28533=CARTESIAN_POINT ( 'NONE',  ( -9.184850993605147944E-16, -167.2500000000000000, 5.000000000000000000 ) ) ;
#28534=DIRECTION ( 'NONE',  ( -0.000000000000000000, 1.000000000000000000, -0.000000000000000000 ) ) ;
#28535=CARTESIAN_POINT ( 'NONE',  ( -2.499999999999996447, -29.83333333333332860, 4.330127018922195425 ) ) ;
#28536=CARTESIAN_POINT ( 'NONE',  ( 9.457646018065525792E-16, -33.06249999863440792, 5.148502694627439702 ) ) ;
#28537=CARTESIAN_POINT ( 'NONE',  ( -5.000000000000000000, -35.95833333060213732, -2.886751345948128211 ) ) ;
#28538=CARTESIAN_POINT ( 'NONE',  ( 4.458734124999999437, -60.81249999863440081, -5.460374474430324690E-16 ) ) ;
#28541=CARTESIAN_POINT ( 'NONE',  ( 2.229367062499998831, -12.89583333196774007, -3.861377020970580887 ) ) ;
#28543=CARTESIAN_POINT ( 'NONE',  ( -5.000000000000000000, -75.08333333333332860, -2.886751345948128211 ) ) ;
#28547=CARTESIAN_POINT ( 'NONE',  ( -5.000000000000000000, -82.87499999726881583, 0.000000000000000000 ) ) ;
#28548=CARTESIAN_POINT ( 'NONE',  ( 0.000000000000000000, -170.0000000000000000, 0.000000000000000000 ) ) ;
#28551=CARTESIAN_POINT ( 'NONE',  ( -2.229367062499996610, -21.39583333196774007, 3.861377020970582219 ) ) ;
#28552=CARTESIAN_POINT ( 'NONE',  ( -4.458734124999998549, -57.47916666530108643, 2.574251347313722516 ) ) ;
#28553=VERTEX_POINT ( 'NONE', #47656 ) ;
#28554=CARTESIAN_POINT ( 'NONE',  ( -1.846868145590734756, -168.3750000013655779, -4.458734125000000326 ) ) ;
#28564=CARTESIAN_POINT ( 'NONE',  ( 1.846868145590736310, -142.8750000013656063, 4.458734124999999437 ) ) ;
#28568=CARTESIAN_POINT ( 'NONE',  ( -3.152548672688508926E-16, -67.81249999863440792, -5.148502694627439702 ) ) ;
#28571=CARTESIAN_POINT ( 'NONE',  ( -1.846868145590734756, -142.1250000013656063, -4.458734124999999437 ) ) ;
#28573=( BOUNDED_CURVE ( )  B_SPLINE_CURVE ( 2, ( #24225, #63477, #36110, #40921, #45117, #6210, #35477, #1401, #31269 ),
 .UNSPECIFIED., .F., .F. ) 
 B_SPLINE_CURVE_WITH_KNOTS ( ( 3, 2, 2, 2, 3 ),
 ( 0.9312500000000000222, 0.9319444444444444642, 0.9333333333333333481, 0.9347222222222222321, 0.9354166666666666741 ),
 .UNSPECIFIED. ) 
 CURVE ( )  GEOMETRIC_REPRESENTATION_ITEM ( )  RATIONAL_B_SPLINE_CURVE ( ( 0.9330127018922194093, 0.9330127018922194093, 1.000000000000000000, 0.8660254037844387076, 1.000000000000000000, 0.8660254037844387076, 1.000000000000000000, 0.9330127018922194093, 0.9330127018922194093 ) ) 
 REPRESENTATION_ITEM ( '' )  );
#28575=CARTESIAN_POINT ( 'NONE',  ( 1.975475456537005874E-15, -70.62499999726880162, 5.000000000000000000 ) ) ;
#28579=FACE_OUTER_BOUND ( 'NONE', #8386, .T. ) ;
#28581=CARTESIAN_POINT ( 'NONE',  ( -4.458734124999999437, 23.35416666803226349, -2.574251347313719407 ) ) ;
#28582=CARTESIAN_POINT ( 'NONE',  ( 5.000000000000000000, -18.50000000000000355, -6.123233995736766282E-16 ) ) ;
#28588=CARTESIAN_POINT ( 'NONE',  ( 2.229367062500001939, 1.020833334698927120, 3.861377020970579999 ) ) ;
#28589=CARTESIAN_POINT ( 'NONE',  ( -4.458734124999997661, -23.47916666530107221, 2.574251347313722516 ) ) ;
#28591=CARTESIAN_POINT ( 'NONE',  ( 4.458734124999999437, -155.5000000013655779, 1.846868145590737864 ) ) ;
#28596=CARTESIAN_POINT ( 'NONE',  ( -2.229367062500000163, 28.52083333469892779, -3.861377020970580443 ) ) ;
#28599=CARTESIAN_POINT ( 'NONE',  ( 9.457646018065525792E-16, -73.31249999863439371, 5.148502694627439702 ) ) ;
#28602=CARTESIAN_POINT ( 'NONE',  ( 0.000000000000000000, -170.0000000000000000, 5.000000000000000000 ) ) ;
#28603=ORIENTED_EDGE ( 'NONE', *, *, #20789, .F. ) ;
#28604=( BOUNDED_CURVE ( )  B_SPLINE_CURVE ( 2, ( #24530, #44455, #735, #415, #58629, #20018, #19381, #4587, #59262 ),
 .UNSPECIFIED., .F., .F. ) 
 B_SPLINE_CURVE_WITH_KNOTS ( ( 3, 2, 2, 2, 3 ),
 ( 0.7749999999999998002, 0.7791666666666664520, 0.7833333333333331039, 0.7874999999999997558, 0.7916666666666664076 ),
 .UNSPECIFIED. ) 
 CURVE ( )  GEOMETRIC_REPRESENTATION_ITEM ( )  RATIONAL_B_SPLINE_CURVE ( ( 1.000000000000003997, 0.9238795325112826307, 1.000000000000000000, 0.9238795325112867385, 1.000000000000000000, 0.9238795325112867385, 1.000000000000000000, 0.9238795325112908463, 0.9999999999999958922 ) ) 
 REPRESENTATION_ITEM ( '' )  );
#28605=CARTESIAN_POINT ( 'NONE',  ( -1.339745962155610925, 12.33034180399266333, 5.000000000000000000 ) ) ;
#28606=CARTESIAN_POINT ( 'NONE',  ( 2.500000000000002220, -11.66666666666666607, 4.330127018922192761 ) ) ;
#28607=CARTESIAN_POINT ( 'NONE',  ( 4.458734124999999437, -14.81249999863440436, -5.460374474430324690E-16 ) ) ;
#28608=CARTESIAN_POINT ( 'NONE',  ( 4.458734125000000326, -75.89583333196775072, 2.574251347313718519 ) ) ;
#28609=CARTESIAN_POINT ( 'NONE',  ( -3.152801135295367096, -168.3125000013656063, -3.152801135295367541 ) ) ;
#28611=CARTESIAN_POINT ( 'NONE',  ( -2.499999999999996447, -17.70833333060214443, 4.330127018922195425 ) ) ;
#28612=CARTESIAN_POINT ( 'NONE',  ( 9.457646018065525792E-16, -47.06249999863440792, 5.148502694627439702 ) ) ;
#28616=CARTESIAN_POINT ( 'NONE',  ( -2.229367062499996610, 5.604166668032261711, 3.861377020970582219 ) ) ;
#28618=CARTESIAN_POINT ( 'NONE',  ( -5.000000000000000000, -86.87499999726880162, 0.000000000000000000 ) ) ;
#28619=CARTESIAN_POINT ( 'NONE',  ( -5.000000000000000000, -63.00000000000000000, 0.000000000000000000 ) ) ;
#28620=CARTESIAN_POINT ( 'NONE',  ( -3.152801135295367985, -158.0625000013656063, 3.152801135295367096 ) ) ;
#28622=CARTESIAN_POINT ( 'NONE',  ( -2.499999999999996447, -78.83333333333332860, 4.330127018922195425 ) ) ;
#28623=CARTESIAN_POINT ( 'NONE',  ( -3.535533905932738641, -163.3750000000000284, 3.535533905932737309 ) ) ;
#28626=CARTESIAN_POINT ( 'NONE',  ( -4.458734124999999437, -7.562499998634404363, 0.000000000000000000 ) ) ;
#28627=CARTESIAN_POINT ( 'NONE',  ( 2.229367062499998831, -40.89583333196773651, -3.861377020970580887 ) ) ;
#28629=CARTESIAN_POINT ( 'NONE',  ( 4.458734125000000326, -148.3750000013655779, -1.846868145590734978 ) ) ;
#28635=AXIS2_PLACEMENT_3D ( 'NONE', #20963, #44745, #5520 ) ;
#28636=CARTESIAN_POINT ( 'NONE',  ( -4.458734124999999437, -77.56249999863440792, 0.000000000000000000 ) ) ;
#28639=DIRECTION ( 'NONE',  ( -0.000000000000000000, 1.000000000000000000, -0.000000000000000000 ) ) ;
#28640=EDGE_CURVE ( 'NONE', #43748, #18601, #349, .T. ) ;
#28643=CARTESIAN_POINT ( 'NONE',  ( -2.229367062499996610, -1.145833331967736957, 3.861377020970582219 ) ) ;
#28645=CARTESIAN_POINT ( 'NONE',  ( 3.152801135295366208, -152.5625000013655779, 3.152801135295367985 ) ) ;
#28647=ORIENTED_EDGE ( 'NONE', *, *, #57893, .T. ) ;
#28650=CARTESIAN_POINT ( 'NONE',  ( 5.000000000000000000, -12.37499999726881050, -6.123233995736766282E-16 ) ) ;
#28659=CARTESIAN_POINT ( 'NONE',  ( -3.152548672688508926E-16, 19.43750000136559208, -5.148502694627439702 ) ) ;
#28661=CARTESIAN_POINT ( 'NONE',  ( 9.457646018065525792E-16, -10.31249999863440969, 5.148502694627439702 ) ) ;
#28662=CARTESIAN_POINT ( 'NONE',  ( -2.500000000000000444, -63.16666666666666430, -4.330127018922193649 ) ) ;
#28664=CARTESIAN_POINT ( 'NONE',  ( -4.458734125000001214, -167.8750000013656063, 1.846868145590734089 ) ) ;
#28667=EDGE_CURVE ( 'NONE', #176, #21872, #39392, .T. ) ;
#28670=DIRECTION ( 'NONE',  ( -0.000000000000000000, 1.000000000000000000, -0.000000000000000000 ) ) ;
#28672=CARTESIAN_POINT ( 'NONE',  ( 4.458734124999997661, -158.7500000013656063, 1.846868145590737864 ) ) ;
#28676=ORIENTED_EDGE ( 'NONE', *, *, #54891, .T. ) ;
#28680=LINE ( 'NONE', #38032, #49388 ) ;
#28681=CARTESIAN_POINT ( 'NONE',  ( -2.499999999999996447, 1.166666666666666519, 4.330127018922195425 ) ) ;
#28683=CARTESIAN_POINT ( 'NONE',  ( 4.458734124999998549, -59.72916666530106511, -2.574251347313721627 ) ) ;
#28685=CARTESIAN_POINT ( 'NONE',  ( -2.499999999999996447, -1.708333330602145761, 4.330127018922195425 ) ) ;
#28686=CARTESIAN_POINT ( 'NONE',  ( 4.458734125000001214, -30.89583333196773296, 2.574251347313718519 ) ) ;
#28687=CARTESIAN_POINT ( 'NONE',  ( 5.000000000000000000, 17.70833333606451632, -2.886751345948130876 ) ) ;
#28690=CARTESIAN_POINT ( 'NONE',  ( -4.999999999999999112, -46.91666666666665719, 2.886751345948131764 ) ) ;
#28691=ADVANCED_FACE ( 'NONE', ( #62472 ), #3610, .T. ) ;
#28694=CARTESIAN_POINT ( 'NONE',  ( 5.000000000000000888, -64.58333333333332860, 2.886751345948126879 ) ) ;
#28695=CARTESIAN_POINT ( 'NONE',  ( 4.458734124999998549, -69.72916666530107932, -2.574251347313721627 ) ) ;
#28696=CARTESIAN_POINT ( 'NONE',  ( 2.730187237215162345E-16, -147.4375000013656063, -4.458734124999999437 ) ) ;
#28697=CARTESIAN_POINT ( 'NONE',  ( -2.229367062500000163, -78.47916666530106511, -3.861377020970580443 ) ) ;
#28699=CARTESIAN_POINT ( 'NONE',  ( 2.229367062500001939, -24.22916666530107577, 3.861377020970579999 ) ) ;
#28700=( BOUNDED_CURVE ( )  B_SPLINE_CURVE ( 2, ( #49305, #55417, #49626, #59608, #25822, #754, #25175, #26137, #10061 ),
 .UNSPECIFIED., .F., .F. ) 
 B_SPLINE_CURVE_WITH_KNOTS ( ( 3, 2, 2, 2, 3 ),
 ( 0.4229166666666666630, 0.4236111111111111049, 0.4249999999999999889, 0.4263888888888888729, 0.4270833333333333148 ),
 .UNSPECIFIED. ) 
 CURVE ( )  GEOMETRIC_REPRESENTATION_ITEM ( )  RATIONAL_B_SPLINE_CURVE ( ( 0.9330127018922194093, 0.9330127018922194093, 1.000000000000000000, 0.8660254037844387076, 1.000000000000000000, 0.8660254037844387076, 1.000000000000000000, 0.9330127018922194093, 0.9330127018922194093 ) ) 
 REPRESENTATION_ITEM ( '' )  );
#28701=CARTESIAN_POINT ( 'NONE',  ( -2.500000000000000444, -64.04166666393547303, -4.330127018922193649 ) ) ;
#28702=ORIENTED_EDGE ( 'NONE', *, *, #4006, .F. ) ;
#28706=CARTESIAN_POINT ( 'NONE',  ( -2.500000000000000444, 7.958333336064518093, -4.330127018922193649 ) ) ;
#28708=CARTESIAN_POINT ( 'NONE',  ( -2.500000000000000444, -78.04166666393547303, -4.330127018922193649 ) ) ;
#28709=EDGE_CURVE ( 'NONE', #61790, #29720, #13874, .T. ) ;
#28710=CARTESIAN_POINT ( 'NONE',  ( -2.229367062499996610, -60.39583333196774362, 3.861377020970582219 ) ) ;
#28713=CARTESIAN_POINT ( 'NONE',  ( -9.184850993605147944E-16, -142.2500000000000284, 5.000000000000000000 ) ) ;
#28714=CARTESIAN_POINT ( 'NONE',  ( 9.457646018065525792E-16, 16.93750000136559564, 5.148502694627439702 ) ) ;
#28717=CARTESIAN_POINT ( 'NONE',  ( 4.458734124999997661, -166.5000000013655779, 1.846868145590737864 ) ) ;
#28719=ORIENTED_EDGE ( 'NONE', *, *, #12995, .F. ) ;
#28721=LINE ( 'NONE', #20354, #22333 ) ;
#28723=CARTESIAN_POINT ( 'NONE',  ( 5.000000000000000000, -40.37499999726880162, -6.123233995736766282E-16 ) ) ;
#28726=CARTESIAN_POINT ( 'NONE',  ( 5.000000000000000888, -20.58333333333333215, 2.886751345948126879 ) ) ;
#28729=CARTESIAN_POINT ( 'NONE',  ( -3.535533905932738641, -156.3750000000000000, 3.535533905932737309 ) ) ;
#28730=DIRECTION ( 'NONE',  ( -0.000000000000000000, 1.000000000000000000, -0.000000000000000000 ) ) ;
#28733=FACE_OUTER_BOUND ( 'NONE', #18194, .T. ) ;
#28735=CARTESIAN_POINT ( 'NONE',  ( -2.071067811865475061, -147.8125000027311842, -5.000000000000000888 ) ) ;
#28740=CARTESIAN_POINT ( 'NONE',  ( -9.184850993605147944E-16, -142.2500000000000284, 5.000000000000000000 ) ) ;
#28742=EDGE_CURVE ( 'NONE', #47984, #39890, #8120, .T. ) ;
#28744=CARTESIAN_POINT ( 'NONE',  ( -1.846868145590737420, -168.0000000013656347, 4.458734124999997661 ) ) ;
#28745=CARTESIAN_POINT ( 'NONE',  ( 2.229367062500001939, -29.97916666530107221, 3.861377020970579999 ) ) ;
#28747=FACE_OUTER_BOUND ( 'NONE', #24779, .T. ) ;
#28748=CARTESIAN_POINT ( 'NONE',  ( 5.000000000000000000, -45.37499999726880873, -6.123233995736766282E-16 ) ) ;
#28750=CARTESIAN_POINT ( 'NONE',  ( -1.846868145590734756, -148.1250000013655779, -4.458734125000000326 ) ) ;
#28752=CARTESIAN_POINT ( 'NONE',  ( 5.000000000000000888, -89.45833333060215864, 2.886751345948126879 ) ) ;
#28754=CARTESIAN_POINT ( 'NONE',  ( -4.458734124999999437, -58.64583333196773651, -2.574251347313719407 ) ) ;
#28756=EDGE_CURVE ( 'NONE', #4948, #2786, #57473, .T. ) ;
#28759=CARTESIAN_POINT ( 'NONE',  ( -2.499999999999996447, 18.16666666666666430, 4.330127018922195425 ) ) ;
#28762=CARTESIAN_POINT ( 'NONE',  ( 9.457646018065525792E-16, -5.062499998634401699, 5.148502694627439702 ) ) ;
#28763=CARTESIAN_POINT ( 'NONE',  ( -9.184850993605147944E-16, -154.2500000000000000, 5.000000000000000000 ) ) ;
#28765=CARTESIAN_POINT ( 'NONE',  ( -2.229367062500000163, 8.270833334698926009, -3.861377020970580443 ) ) ;
#28767=EDGE_CURVE ( 'NONE', #26541, #871, #34427, .T. ) ;
#28768=FACE_OUTER_BOUND ( 'NONE', #27524, .T. ) ;
#28769=DIRECTION ( 'NONE',  ( 0.000000000000000000, -0.000000000000000000, 1.000000000000000000 ) ) ;
#28770=CARTESIAN_POINT ( 'NONE',  ( 4.458734125000001214, -56.89583333196774362, 2.574251347313718519 ) ) ;
#28771=EDGE_CURVE ( 'NONE', #8963, #26541, #15179, .T. ) ;
#28772=CARTESIAN_POINT ( 'NONE',  ( -3.152801135295367985, -160.0625000013656063, 3.152801135295367096 ) ) ;
#28776=CARTESIAN_POINT ( 'NONE',  ( 5.000000000000000888, -50.45833333060213732, 2.886751345948126879 ) ) ;
#28778=CARTESIAN_POINT ( 'NONE',  ( -4.458734124999999437, 3.354166668032260823, -2.574251347313719407 ) ) ;
#28780=CARTESIAN_POINT ( 'NONE',  ( 0.000000000000000000, -170.0000000000000000, 0.000000000000000000 ) ) ;
#28782=CARTESIAN_POINT ( 'NONE',  ( -8.190561711645485556E-16, -158.6875000013655779, 4.458734124999999437 ) ) ;
#28783=ORIENTED_EDGE ( 'NONE', *, *, #28159, .T. ) ;
#28787=CARTESIAN_POINT ( 'NONE',  ( 2.499999999999998668, -47.20833333060214443, -4.330127018922193649 ) ) ;
#28788=CARTESIAN_POINT ( 'NONE',  ( -2.229367062500000163, -36.72916666530107221, -3.861377020970580443 ) ) ;
#28792=CARTESIAN_POINT ( 'NONE',  ( -3.535533905932737309, -156.7500000027312126, -3.535533905932738197 ) ) ;
#28794=CARTESIAN_POINT ( 'NONE',  ( 4.458734124999998549, -86.97916666530106511, -2.574251347313721627 ) ) ;
#28796=CARTESIAN_POINT ( 'NONE',  ( -5.000000000000000000, 25.12500000273118417, 0.000000000000000000 ) ) ;
#28797=CARTESIAN_POINT ( 'NONE',  ( -6.972266317189433020E-16, -7.249999999999998224, -5.000000000000000000 ) ) ;
#28799=CARTESIAN_POINT ( 'NONE',  ( -2.499999999999996447, -44.70833333060214443, 4.330127018922195425 ) ) ;
#28801=CARTESIAN_POINT ( 'NONE',  ( -6.972266317189433020E-16, -85.12499999726880162, -5.000000000000000000 ) ) ;
#28808=CARTESIAN_POINT ( 'NONE',  ( -2.229367062500000163, -84.72916666530107932, -3.861377020970580443 ) ) ;
#28811=ORIENTED_EDGE ( 'NONE', *, *, #14877, .T. ) ;
#28814=CARTESIAN_POINT ( 'NONE',  ( -5.000000000000000000, -160.6250000027311842, -6.123233995736766282E-16 ) ) ;
#28818=CARTESIAN_POINT ( 'NONE',  ( 0.000000000000000000, -170.0000000000000000, 0.000000000000000000 ) ) ;
#28824=FACE_OUTER_BOUND ( 'NONE', #59830, .T. ) ;
#28825=CARTESIAN_POINT ( 'NONE',  ( -2.229367062500000163, -12.47916666530107044, -3.861377020970580443 ) ) ;
#28827=CARTESIAN_POINT ( 'NONE',  ( 3.535533905932738197, -154.8750000000000000, -3.535533905932738197 ) ) ;
#28829=CARTESIAN_POINT ( 'NONE',  ( -4.458734124999997661, -39.47916666530106511, 2.574251347313722516 ) ) ;
#28831=CARTESIAN_POINT ( 'NONE',  ( -2.499999999999996447, -11.83333333333333393, 4.330127018922195425 ) ) ;
#28835=CARTESIAN_POINT ( 'NONE',  ( -4.458734124999999437, 8.604166668032261711, -2.574251347313719407 ) ) ;
#28837=CARTESIAN_POINT ( 'NONE',  ( -1.339745962155610925, -68.79465819873850307, 5.000000000000000000 ) ) ;
#28840=CARTESIAN_POINT ( 'NONE',  ( 5.000000000000000000, 12.70833333606451809, -2.886751345948129988 ) ) ;
#28843=DIRECTION ( 'NONE',  ( -0.000000000000000000, 1.000000000000000000, -0.000000000000000000 ) ) ;
#28844=ORIENTED_EDGE ( 'NONE', *, *, #52476, .T. ) ;
#28846=CARTESIAN_POINT ( 'NONE',  ( 2.500000000000002220, -85.66666666666667140, 4.330127018922192761 ) ) ;
#28847=CARTESIAN_POINT ( 'NONE',  ( 1.060575238724906964E-15, -29.74999999999999645, 5.773502691896257311 ) ) ;
#28848=CARTESIAN_POINT ( 'NONE',  ( -2.229367062500000163, -34.47916666530107221, -3.861377020970580443 ) ) ;
#28850=CARTESIAN_POINT ( 'NONE',  ( -5.000000000000000000, -31.95833333060214443, -2.886751345948128211 ) ) ;
#28851=CARTESIAN_POINT ( 'NONE',  ( 2.229367062499998831, -64.64583333196773651, -3.861377020970580887 ) ) ;
#28854=CARTESIAN_POINT ( 'NONE',  ( 4.458734125000001214, -13.14583333196774184, 2.574251347313718519 ) ) ;
#28855=ORIENTED_EDGE ( 'NONE', *, *, #37404, .T. ) ;
#28856=CARTESIAN_POINT ( 'NONE',  ( -3.535250795749689387E-16, -79.25000000000000000, -5.773502691896257311 ) ) ;
#28857=CARTESIAN_POINT ( 'NONE',  ( 5.000000000000000888, 28.54166666939784847, 2.886751345948126879 ) ) ;
#28859=CARTESIAN_POINT ( 'NONE',  ( 1.060575238724906964E-15, -80.62499999726881583, 5.773502691896257311 ) ) ;
#28860=CARTESIAN_POINT ( 'NONE',  ( -2.499999999999996447, -31.83333333333333215, 4.330127018922195425 ) ) ;
#28864=CARTESIAN_POINT ( 'NONE',  ( 2.229367062499998831, -23.89583333196773651, -3.861377020970580887 ) ) ;
#28865=CARTESIAN_POINT ( 'NONE',  ( 2.229367062500001939, -60.22916666530106511, 3.861377020970579999 ) ) ;
#28868=CARTESIAN_POINT ( 'NONE',  ( 1.846868145590736310, -166.8750000013655779, 4.458734124999999437 ) ) ;
#28871=VERTEX_POINT ( 'NONE', #36917 ) ;
#28875=CARTESIAN_POINT ( 'NONE',  ( 1.975475456537005874E-15, -58.62499999726880162, 5.000000000000000000 ) ) ;
#28877=( BOUNDED_CURVE ( )  B_SPLINE_CURVE ( 2, ( #34340, #25018, #53965, #30146, #9896, #29505, #24702, #5402, #44628 ),
 .UNSPECIFIED., .F., .F. ) 
 B_SPLINE_CURVE_WITH_KNOTS ( ( 3, 2, 2, 2, 3 ),
 ( 0.8083333333333331261, 0.8124999999999997780, 0.8166666666666664298, 0.8208333333333330817, 0.8249999999999997335 ),
 .UNSPECIFIED. ) 
 CURVE ( )  GEOMETRIC_REPRESENTATION_ITEM ( )  RATIONAL_B_SPLINE_CURVE ( ( 1.000000000000003997, 0.9238795325112826307, 1.000000000000000000, 0.9238795325112867385, 1.000000000000000000, 0.9238795325112867385, 1.000000000000000000, 0.9238795325112908463, 0.9999999999999958922 ) ) 
 REPRESENTATION_ITEM ( '' )  );
#28879=CARTESIAN_POINT ( 'NONE',  ( 3.152801135295367541, -142.5625000013655779, -3.152801135295367541 ) ) ;
#28881=CARTESIAN_POINT ( 'NONE',  ( 5.000000000000000000, -70.50000000000000000, -6.123233995736766282E-16 ) ) ;
#28883=CARTESIAN_POINT ( 'NONE',  ( -3.152548672688508926E-16, -68.81249999863439371, -5.148502694627439702 ) ) ;
#28885=CARTESIAN_POINT ( 'NONE',  ( -1.339745962155613812, -70.20534180126148271, -5.000000000000000000 ) ) ;
#28886=CARTESIAN_POINT ( 'NONE',  ( 3.152801135295367541, -141.3125000013655779, -3.152801135295367541 ) ) ;
#28889=CARTESIAN_POINT ( 'NONE',  ( -1.339745962155610925, -70.66965819600731891, 5.000000000000000000 ) ) ;
#28895=CARTESIAN_POINT ( 'NONE',  ( -4.458734124999999437, 24.35416666803225993, -2.574251347313719407 ) ) ;
#28896=CARTESIAN_POINT ( 'NONE',  ( -6.972266317189433020E-16, -18.25000000000000000, -5.000000000000000000 ) ) ;
#28903=CARTESIAN_POINT ( 'NONE',  ( 4.458734124999999437, -0.8124999986344055847, -5.460374474430324690E-16 ) ) ;
#28904=ORIENTED_EDGE ( 'NONE', *, *, #54153, .F. ) ;
#28905=CARTESIAN_POINT ( 'NONE',  ( 4.458734125000000326, -27.14583333196774717, 2.574251347313718519 ) ) ;
#28906=CARTESIAN_POINT ( 'NONE',  ( 4.458734124999999437, -157.5000000013656063, 1.846868145590737864 ) ) ;
#28907=VECTOR ( 'NONE', #20967, 1000.000000000000000 ) ;
#28911=CARTESIAN_POINT ( 'NONE',  ( 4.458734125000000326, -71.14583333196773651, 2.574251347313718519 ) ) ;
#28915=EDGE_LOOP ( 'NONE', ( #5546, #45487, #45514, #57316 ) ) ;
#28916=CARTESIAN_POINT ( 'NONE',  ( 3.061616997868383141E-16, -140.7500000000000000, -5.000000000000000000 ) ) ;
#28918=CARTESIAN_POINT ( 'NONE',  ( -5.000000000000000000, -15.08333333333333215, -2.886751345948128211 ) ) ;
#28919=CARTESIAN_POINT ( 'NONE',  ( 2.229367062499998831, -16.64583333196773651, -3.861377020970580887 ) ) ;
#28920=CARTESIAN_POINT ( 'NONE',  ( -3.152548672688508926E-16, -78.56249999863440792, -5.148502694627439702 ) ) ;
#28921=CARTESIAN_POINT ( 'NONE',  ( 3.152801135295366208, -167.8125000013656063, 3.152801135295367985 ) ) ;
#28922=CARTESIAN_POINT ( 'NONE',  ( -3.535250795749689387E-16, -16.12499999726881228, -5.773502691896257311 ) ) ;
#28923=CARTESIAN_POINT ( 'NONE',  ( -2.229367062500000163, -48.47916666530106511, -3.861377020970580443 ) ) ;
#28925=CARTESIAN_POINT ( 'NONE',  ( -6.972266317189433020E-16, -15.12499999726881050, -5.000000000000000000 ) ) ;
#28926=CARTESIAN_POINT ( 'NONE',  ( 9.457646018065525792E-16, -0.3124999986344051961, 5.148502694627439702 ) ) ;
#28929=CARTESIAN_POINT ( 'NONE',  ( 1.060575238724906964E-15, -60.75000000000000000, 5.773502691896257311 ) ) ;
#28930=CARTESIAN_POINT ( 'NONE',  ( 3.152801135295366208, -157.8125000013656063, 3.152801135295367985 ) ) ;
#28933=CARTESIAN_POINT ( 'NONE',  ( -5.000000000000000000, -161.5000000000000000, -6.123233995736766282E-16 ) ) ;
#28935=CARTESIAN_POINT ( 'NONE',  ( -2.229367062500000163, -5.729166665301072214, -3.861377020970580443 ) ) ;
#28936=CARTESIAN_POINT ( 'NONE',  ( 2.229367062499998831, -47.89583333196774362, -3.861377020970580887 ) ) ;
#28938=CARTESIAN_POINT ( 'NONE',  ( 2.730187237215162345E-16, -150.1875000013656063, -4.458734124999999437 ) ) ;
#28941=VERTEX_POINT ( 'NONE', #17619 ) ;
#28942=CARTESIAN_POINT ( 'NONE',  ( 5.000000000000000000, -155.1875000027312126, 2.071067811865478614 ) ) ;
#28943=CARTESIAN_POINT ( 'NONE',  ( -4.999999999999998224, -68.79166666393547303, 2.886751345948131764 ) ) ;
#28947=ADVANCED_FACE ( 'NONE', ( #2210 ), #61688, .T. ) ;
#28949=CYLINDRICAL_SURFACE ( 'NONE', #44163, 5.000000000000000000 ) ;
#28952=CARTESIAN_POINT ( 'NONE',  ( -3.152548672688508926E-16, -1.562499998634406140, -5.148502694627439702 ) ) ;
#28954=CARTESIAN_POINT ( 'NONE',  ( -4.458734125000000326, -151.8750000013655779, 1.846868145590734089 ) ) ;
#28958=CARTESIAN_POINT ( 'NONE',  ( 3.061616997868383141E-16, -148.7500000000000284, -5.000000000000000000 ) ) ;
#28959=CARTESIAN_POINT ( 'NONE',  ( 2.499999999999998668, -40.33333333333332860, -4.330127018922193649 ) ) ;
#28968=ORIENTED_EDGE ( 'NONE', *, *, #45520, .F. ) ;
#28969=CARTESIAN_POINT ( 'NONE',  ( 4.458734125000000326, 15.10416666803225993, 2.574251347313718519 ) ) ;
#28971=CARTESIAN_POINT ( 'NONE',  ( 4.458734124999999437, -9.062499998634406140, -5.460374474430324690E-16 ) ) ;
#28972=( BOUNDED_CURVE ( )  B_SPLINE_CURVE ( 2, ( #44459, #11004, #49612, #34479, #5551, #25163, #44777, #6196, #25811 ),
 .UNSPECIFIED., .F., .F. ) 
 B_SPLINE_CURVE_WITH_KNOTS ( ( 3, 2, 2, 2, 3 ),
 ( 0.2562499999999999778, 0.2569444444444444198, 0.2583333333333333592, 0.2597222222222222432, 0.2604166666666666852 ),
 .UNSPECIFIED. ) 
 CURVE ( )  GEOMETRIC_REPRESENTATION_ITEM ( )  RATIONAL_B_SPLINE_CURVE ( ( 0.9330127018922194093, 0.9330127018922194093, 1.000000000000000000, 0.8660254037844387076, 1.000000000000000000, 0.8660254037844387076, 1.000000000000000000, 0.9330127018922194093, 0.9330127018922194093 ) ) 
 REPRESENTATION_ITEM ( '' )  );
#28975=CARTESIAN_POINT ( 'NONE',  ( 4.458734124999999437, -167.4375000013655779, 0.000000000000000000 ) ) ;
#28976=CARTESIAN_POINT ( 'NONE',  ( 2.500000000000002220, -88.66666666666665719, 4.330127018922192761 ) ) ;
#28980=CARTESIAN_POINT ( 'NONE',  ( -6.972266317189433020E-16, -67.25000000000000000, -5.000000000000000000 ) ) ;
#28983=CARTESIAN_POINT ( 'NONE',  ( 2.730187237215162345E-16, -154.4375000013655779, -4.458734124999999437 ) ) ;
#28985=CARTESIAN_POINT ( 'NONE',  ( -9.184850993605147944E-16, -163.2500000000000000, 5.000000000000000000 ) ) ;
#28989=CARTESIAN_POINT ( 'NONE',  ( 3.061616997868383141E-16, -161.7500000000000000, -5.000000000000000000 ) ) ;
#28990=CARTESIAN_POINT ( 'NONE',  ( 5.000000000000000000, 4.583333333333331261, -2.886751345948129988 ) ) ;
#28991=CARTESIAN_POINT ( 'NONE',  ( -4.458734124999999437, -62.39583333196774362, -2.574251347313719407 ) ) ;
#28992=CARTESIAN_POINT ( 'NONE',  ( 1.975475456537005874E-15, 20.24999999999999289, 5.000000000000000000 ) ) ;
#28993=CARTESIAN_POINT ( 'NONE',  ( 1.060575238724906964E-15, -1.624999997268814500, 5.773502691896257311 ) ) ;
#28994=CARTESIAN_POINT ( 'NONE',  ( 9.457646018065525792E-16, -30.06249999863440081, 5.148502694627439702 ) ) ;
#28998=CARTESIAN_POINT ( 'NONE',  ( -5.000000000000000000, -47.08333333333333570, -2.886751345948128211 ) ) ;
#29001=CARTESIAN_POINT ( 'NONE',  ( 1.975475456537005874E-15, -64.74999999999998579, 5.000000000000000000 ) ) ;
#29002=CARTESIAN_POINT ( 'NONE',  ( -2.229367062500000163, -69.47916666530107932, -3.861377020970580443 ) ) ;
#29003=CARTESIAN_POINT ( 'NONE',  ( 4.458734125000000326, -143.6250000013656347, -1.846868145590734978 ) ) ;
#29004=CARTESIAN_POINT ( 'NONE',  ( 4.458734124999999437, -78.81249999863440792, -5.460374474430324690E-16 ) ) ;
#29006=CARTESIAN_POINT ( 'NONE',  ( -2.229367062500000163, -23.72916666530107577, -3.861377020970580443 ) ) ;
#29007=CARTESIAN_POINT ( 'NONE',  ( 2.500000000000002220, -67.54166666393547303, 4.330127018922192761 ) ) ;
#29012=CARTESIAN_POINT ( 'NONE',  ( 3.061616997868383141E-16, -165.7500000000000000, -5.000000000000000000 ) ) ;
#29013=ORIENTED_EDGE ( 'NONE', *, *, #61587, .T. ) ;
#29014=CARTESIAN_POINT ( 'NONE',  ( 1.339745962155612702, 27.70534180126147561, -5.000000000000000000 ) ) ;
#29016=CARTESIAN_POINT ( 'NONE',  ( -6.972266317189433020E-16, -78.12499999726881583, -5.000000000000000000 ) ) ;
#29017=CARTESIAN_POINT ( 'NONE',  ( -2.229367062499996610, -61.39583333196774362, 3.861377020970582219 ) ) ;
#29022=CARTESIAN_POINT ( 'NONE',  ( -6.972266317189433020E-16, -61.12499999726880162, -5.000000000000000000 ) ) ;
#29023=CARTESIAN_POINT ( 'NONE',  ( 9.457646018065525792E-16, 11.93750000136559386, 5.148502694627439702 ) ) ;
#29025=CARTESIAN_POINT ( 'NONE',  ( -8.190561711645485556E-16, -165.6875000013655779, 4.458734124999999437 ) ) ;
#29035=CARTESIAN_POINT ( 'NONE',  ( -1.339745962155610925, 6.205341801261478274, 5.000000000000000000 ) ) ;
#29036=CARTESIAN_POINT ( 'NONE',  ( 5.000000000000000888, -45.58333333333333570, 2.886751345948126879 ) ) ;
#29037=CARTESIAN_POINT ( 'NONE',  ( 5.000000000000000888, -61.58333333333333570, 2.886751345948126879 ) ) ;
#29038=DIRECTION ( 'NONE',  ( -0.000000000000000000, 1.000000000000000000, -0.000000000000000000 ) ) ;
#29042=CARTESIAN_POINT ( 'NONE',  ( 4.458734124999999437, 6.937500001365594748, -5.460374474430324690E-16 ) ) ;
#29044=CARTESIAN_POINT ( 'NONE',  ( 5.000000000000000000, -150.1875000027311842, 2.071067811865478614 ) ) ;
#29050=CARTESIAN_POINT ( 'NONE',  ( 2.071067811865475505, -144.8125000000000000, -5.000000000000000888 ) ) ;
#29052=CARTESIAN_POINT ( 'NONE',  ( 1.846868145590735200, -165.5000000013655779, -4.458734124999999437 ) ) ;
#29053=CARTESIAN_POINT ( 'NONE',  ( -4.458734124999997661, -28.22916666530107221, 2.574251347313722516 ) ) ;
#29055=CARTESIAN_POINT ( 'NONE',  ( 0.000000000000000000, -170.0000000000000000, 0.000000000000000000 ) ) ;
#29057=CARTESIAN_POINT ( 'NONE',  ( -1.846868145590737420, -144.7500000013656063, 4.458734124999999437 ) ) ;
#29059=CARTESIAN_POINT ( 'NONE',  ( -3.152548672688508926E-16, 26.18750000136559564, -5.148502694627439702 ) ) ;
#29061=CARTESIAN_POINT ( 'NONE',  ( 4.458734125000000326, -55.14583333196773651, 2.574251347313718519 ) ) ;
#29064=CARTESIAN_POINT ( 'NONE',  ( -2.500000000000000444, 19.83333333333333570, -4.330127018922193649 ) ) ;
#29066=CARTESIAN_POINT ( 'NONE',  ( -2.229367062499996610, -5.145833331967740065, 3.861377020970582219 ) ) ;
#29069=EDGE_CURVE ( 'NONE', #25740, #61101, #33348, .T. ) ;
#29070=CARTESIAN_POINT ( 'NONE',  ( -5.000000000000000000, -9.083333333333333925, -2.886751345948128211 ) ) ;
#29071=CARTESIAN_POINT ( 'NONE',  ( -6.972266317189433020E-16, -74.12499999726878741, -5.000000000000000000 ) ) ;
#29074=CARTESIAN_POINT ( 'NONE',  ( 2.229367062500001939, -54.97916666530107221, 3.861377020970579999 ) ) ;
#29075=CARTESIAN_POINT ( 'NONE',  ( 4.458734124999999437, -155.7500000013655779, 1.846868145590737864 ) ) ;
#29076=CARTESIAN_POINT ( 'NONE',  ( 5.000000000000000000, -48.37499999726880873, -6.123233995736766282E-16 ) ) ;
#29078=CARTESIAN_POINT ( 'NONE',  ( -3.152548672688508926E-16, 5.187500001365592972, -5.148502694627439702 ) ) ;
#29082=CARTESIAN_POINT ( 'NONE',  ( -4.458734125000001214, -159.8750000013655779, 1.846868145590734089 ) ) ;
#29085=CARTESIAN_POINT ( 'NONE',  ( -6.972266317189433020E-16, -59.25000000000000000, -5.000000000000000000 ) ) ;
#29086=CARTESIAN_POINT ( 'NONE',  ( -4.458734124999999437, -41.56249999863440081, 0.000000000000000000 ) ) ;
#29087=ORIENTED_EDGE ( 'NONE', *, *, #58256, .F. ) ;
#29091=DIRECTION ( 'NONE',  ( -0.000000000000000000, 1.000000000000000000, -0.000000000000000000 ) ) ;
#29093=FACE_OUTER_BOUND ( 'NONE', #40801, .T. ) ;
#29094=ORIENTED_EDGE ( 'NONE', *, *, #32351, .F. ) ;
#29095=CARTESIAN_POINT ( 'NONE',  ( -2.229367062499996610, 26.85416666803225993, 3.861377020970582219 ) ) ;
#29097=CARTESIAN_POINT ( 'NONE',  ( 1.975475456537005874E-15, -35.62499999726880162, 5.000000000000000000 ) ) ;
#29099=CARTESIAN_POINT ( 'NONE',  ( -1.339745962155617365, 24.20534180126148271, 4.999999999999998224 ) ) ;
#29103=EDGE_CURVE ( 'NONE', #11394, #2464, #53902, .T. ) ;
#29107=CYLINDRICAL_SURFACE ( 'NONE', #58173, 5.000000000000000000 ) ;
#29108=EDGE_CURVE ( 'NONE', #63378, #44876, #19299, .T. ) ;
#29110=CARTESIAN_POINT ( 'NONE',  ( -2.229367062499996610, -86.39583333196773651, 3.861377020970582219 ) ) ;
#29113=( BOUNDED_CURVE ( )  B_SPLINE_CURVE ( 2, ( #63157, #48656, #59928, #25493, #27325, #11331, #42110, #54455, #45433 ),
 .UNSPECIFIED., .F., .F. ) 
 B_SPLINE_CURVE_WITH_KNOTS ( ( 3, 2, 2, 2, 3 ),
 ( 0.2020833333333333370, 0.2027777777777777790, 0.2041666666666666630, 0.2055555555555555469, 0.2062499999999999889 ),
 .UNSPECIFIED. ) 
 CURVE ( )  GEOMETRIC_REPRESENTATION_ITEM ( )  RATIONAL_B_SPLINE_CURVE ( ( 0.9330127018922194093, 0.9330127018922194093, 1.000000000000000000, 0.8660254037844387076, 1.000000000000000000, 0.8660254037844387076, 1.000000000000000000, 0.9330127018922194093, 0.9330127018922194093 ) ) 
 REPRESENTATION_ITEM ( '' )  );
#29115=CARTESIAN_POINT ( 'NONE',  ( -5.000000000000000000, -81.08333333333332860, -2.886751345948128211 ) ) ;
#29117=CARTESIAN_POINT ( 'NONE',  ( 3.535533905932738197, -162.0000000027312126, -3.535533905932738197 ) ) ;
#29128=CARTESIAN_POINT ( 'NONE',  ( 4.458734125000000326, -13.89583333196774007, 2.574251347313718519 ) ) ;
#29129=CARTESIAN_POINT ( 'NONE',  ( 0.000000000000000000, -170.0000000000000000, 0.000000000000000000 ) ) ;
#29130=CARTESIAN_POINT ( 'NONE',  ( -5.000000000000000000, -153.5000000000000284, -6.123233995736766282E-16 ) ) ;
#29133=CARTESIAN_POINT ( 'NONE',  ( 2.229367062499998831, -39.89583333196773651, -3.861377020970580887 ) ) ;
#29135=CARTESIAN_POINT ( 'NONE',  ( -1.339745962155610925, -11.79465819873851906, 5.000000000000000000 ) ) ;
#29140=CARTESIAN_POINT ( 'NONE',  ( -4.458734124999999437, 9.687500001365593860, 0.000000000000000000 ) ) ;
#29141=CARTESIAN_POINT ( 'NONE',  ( -1.339745962155610925, -43.79465819873851729, 5.000000000000000000 ) ) ;
#29142=CARTESIAN_POINT ( 'NONE',  ( -2.500000000000000444, -69.16666666666667140, -4.330127018922193649 ) ) ;
#29143=CARTESIAN_POINT ( 'NONE',  ( 2.229367062500001939, -88.22916666530107932, 3.861377020970579999 ) ) ;
#29144=CARTESIAN_POINT ( 'NONE',  ( 4.458734125000001214, 20.85416666803226349, 2.574251347313718519 ) ) ;
#29146=CARTESIAN_POINT ( 'NONE',  ( -2.499999999999996447, 15.29166666939785202, 4.330127018922195425 ) ) ;
#29147=EDGE_LOOP ( 'NONE', ( #58145, #59740, #59299, #40970 ) ) ;
#29151=DIRECTION ( 'NONE',  ( -0.000000000000000000, 1.000000000000000000, -0.000000000000000000 ) ) ;
#29152=CARTESIAN_POINT ( 'NONE',  ( 5.000000000000000888, -34.58333333333332860, 2.886751345948126879 ) ) ;
#29153=CARTESIAN_POINT ( 'NONE',  ( -4.458734124999999437, -36.31249999863440792, 0.000000000000000000 ) ) ;
#29154=CARTESIAN_POINT ( 'NONE',  ( -2.499999999999996447, -32.70833333060215153, 4.330127018922195425 ) ) ;
#29155=CARTESIAN_POINT ( 'NONE',  ( 4.458734124999998549, -66.72916666530106511, -2.574251347313721627 ) ) ;
#29156=ORIENTED_EDGE ( 'NONE', *, *, #44069, .F. ) ;
#29158=CARTESIAN_POINT ( 'NONE',  ( -2.229367062500000163, -11.47916666530107044, -3.861377020970580443 ) ) ;
#29159=CARTESIAN_POINT ( 'NONE',  ( 4.458734124999998549, -11.97916666530107044, -2.574251347313721627 ) ) ;
#29161=CARTESIAN_POINT ( 'NONE',  ( 5.000000000000000000, -83.41666666666667140, -2.886751345948129988 ) ) ;
#29165=CARTESIAN_POINT ( 'NONE',  ( 5.000000000000000000, -83.37499999726881583, -6.123233995736766282E-16 ) ) ;
#29166=CARTESIAN_POINT ( 'NONE',  ( 1.975475456537005874E-15, -18.74999999999999645, 5.000000000000000000 ) ) ;
#29169=CARTESIAN_POINT ( 'NONE',  ( -4.458734124999998549, -28.47916666530107221, 2.574251347313722516 ) ) ;
#29170=ORIENTED_EDGE ( 'NONE', *, *, #20488, .F. ) ;
#29173=CARTESIAN_POINT ( 'NONE',  ( -4.458734125000001214, -166.1250000013655779, 1.846868145590734089 ) ) ;
#29175=CARTESIAN_POINT ( 'NONE',  ( 5.000000000000000888, -8.458333330602144429, 2.886751345948126879 ) ) ;
#29180=LINE ( 'NONE', #48807, #23967 ) ;
#29185=CARTESIAN_POINT ( 'NONE',  ( -4.458734125000000326, -144.2500000013656063, -1.846868145590735644 ) ) ;
#29189=CARTESIAN_POINT ( 'NONE',  ( 4.458734124999999437, -69.06249999863439371, -5.460374474430324690E-16 ) ) ;
#29190=EDGE_CURVE ( 'NONE', #57375, #20078, #62636, .T. ) ;
#29192=CARTESIAN_POINT ( 'NONE',  ( -6.972266317189433020E-16, -1.124999997268814278, -5.000000000000000000 ) ) ;
#29193=CARTESIAN_POINT ( 'NONE',  ( -3.152801135295367985, -139.8125000013655779, 3.152801135295367096 ) ) ;
#29197=ADVANCED_FACE ( 'NONE', ( #53278 ), #8588, .T. ) ;
#29203=CARTESIAN_POINT ( 'NONE',  ( 4.458734124999998549, 25.02083333469892779, -2.574251347313721627 ) ) ;
#29205=ADVANCED_FACE ( 'NONE', ( #13724 ), #8900, .T. ) ;
#29209=CARTESIAN_POINT ( 'NONE',  ( 5.000000000000000000, -60.37499999726880873, -6.123233995736766282E-16 ) ) ;
#29210=CARTESIAN_POINT ( 'NONE',  ( 4.458734124999999437, 2.187500001365593416, -5.460374474430324690E-16 ) ) ;
#29211=ORIENTED_EDGE ( 'NONE', *, *, #59560, .F. ) ;
#29212=CARTESIAN_POINT ( 'NONE',  ( 2.229367062499998831, -25.89583333196773651, -3.861377020970580887 ) ) ;
#29215=CARTESIAN_POINT ( 'NONE',  ( 4.458734125000001214, 27.10416666803225993, 2.574251347313718519 ) ) ;
#29216=CARTESIAN_POINT ( 'NONE',  ( 6.123233995736766282E-16, -170.0000000000000000, -5.000000000000000000 ) ) ;
#29217=LINE ( 'NONE', #39191, #59410 ) ;
#29218=CARTESIAN_POINT ( 'NONE',  ( 2.229367062499998831, -71.89583333196773651, -3.861377020970580887 ) ) ;
#29220=CYLINDRICAL_SURFACE ( 'NONE', #55248, 5.000000000000000000 ) ;
#29221=CARTESIAN_POINT ( 'NONE',  ( -9.184850993605147944E-16, -156.3750000027311842, 5.000000000000000000 ) ) ;
#29225=CARTESIAN_POINT ( 'NONE',  ( 2.500000000000002220, -19.66666666666666430, 4.330127018922192761 ) ) ;
#29226=CARTESIAN_POINT ( 'NONE',  ( 9.457646018065525792E-16, -20.06249999863440081, 5.148502694627439702 ) ) ;
#29227=CARTESIAN_POINT ( 'NONE',  ( 4.458734124999998549, -81.72916666530106511, -2.574251347313721627 ) ) ;
#29228=AXIS2_PLACEMENT_3D ( 'NONE', #19918, #39532, #29883 ) ;
#29229=CARTESIAN_POINT ( 'NONE',  ( 4.458734124999999437, -168.6875000013656063, 0.000000000000000000 ) ) ;
#29230=CARTESIAN_POINT ( 'NONE',  ( -2.499999999999996447, -15.70833333060214443, 4.330127018922195425 ) ) ;
#29231=CARTESIAN_POINT ( 'NONE',  ( -2.229367062500000163, -47.47916666530106511, -3.861377020970580443 ) ) ;
#29232=VERTEX_POINT ( 'NONE', #39104 ) ;
#29234=LINE ( 'NONE', #19909, #19970 ) ;
#29235=CARTESIAN_POINT ( 'NONE',  ( -4.458734124999999437, 1.437500001365592972, 0.000000000000000000 ) ) ;
#29237=CARTESIAN_POINT ( 'NONE',  ( -6.972266317189433020E-16, -87.12499999726880162, -5.000000000000000000 ) ) ;
#29238=CARTESIAN_POINT ( 'NONE',  ( 1.060575238724906964E-15, -59.74999999999999289, 5.773502691896257311 ) ) ;
#29239=CARTESIAN_POINT ( 'NONE',  ( 3.152801135295366208, -155.8125000013656063, 3.152801135295367985 ) ) ;
#29241=CARTESIAN_POINT ( 'NONE',  ( 1.975475456537005874E-15, -6.749999999999999112, 5.000000000000000000 ) ) ;
#29242=CARTESIAN_POINT ( 'NONE',  ( -2.071067811865475061, -162.6875000000000568, -5.000000000000000888 ) ) ;
#29245=CARTESIAN_POINT ( 'NONE',  ( 4.458734125000001214, -5.145833331967740065, 2.574251347313718519 ) ) ;
#29246=CARTESIAN_POINT ( 'NONE',  ( -4.458734124999999437, -48.56249999863440792, 0.000000000000000000 ) ) ;
#29247=( BOUNDED_CURVE ( )  B_SPLINE_CURVE ( 2, ( #36965, #41455, #51449, #30866, #12514, #27309, #61735, #37280, #41774 ),
 .UNSPECIFIED., .F., .F. ) 
 B_SPLINE_CURVE_WITH_KNOTS ( ( 3, 2, 2, 2, 3 ),
 ( 0.3479166666666666519, 0.3486111111111110938, 0.3499999999999999778, 0.3513888888888888618, 0.3520833333333333592 ),
 .UNSPECIFIED. ) 
 CURVE ( )  GEOMETRIC_REPRESENTATION_ITEM ( )  RATIONAL_B_SPLINE_CURVE ( ( 0.9330127018922194093, 0.9330127018922194093, 1.000000000000000000, 0.8660254037844387076, 1.000000000000000000, 0.8660254037844387076, 1.000000000000000000, 0.9330127018922167448, 0.9330127018922194093 ) ) 
 REPRESENTATION_ITEM ( '' )  );
#29248=CARTESIAN_POINT ( 'NONE',  ( 1.975475456537005874E-15, -7.624999997268812280, 5.000000000000000000 ) ) ;
#29249=CARTESIAN_POINT ( 'NONE',  ( 3.152801135295366208, -148.5625000013655779, 3.152801135295367985 ) ) ;
#29251=DIRECTION ( 'NONE',  ( -0.000000000000000000, 1.000000000000000000, -0.000000000000000000 ) ) ;
#29254=CARTESIAN_POINT ( 'NONE',  ( -1.339745962155660663, -5.669658196007336670, 4.999999999999972466 ) ) ;
#29256=CARTESIAN_POINT ( 'NONE',  ( 1.339745962155615144, -30.70534180126147916, 4.999999999999999112 ) ) ;
#29261=CARTESIAN_POINT ( 'NONE',  ( 9.457646018065525792E-16, -2.062499998634407028, 5.148502694627439702 ) ) ;
#29263=CARTESIAN_POINT ( 'NONE',  ( -3.152801135295367985, -154.8125000013656063, 3.152801135295367096 ) ) ;
#29265=ORIENTED_EDGE ( 'NONE', *, *, #53095, .T. ) ;
#29270=CARTESIAN_POINT ( 'NONE',  ( 5.000000000000000000, 8.708333336064518093, -2.886751345948130876 ) ) ;
#29275=CARTESIAN_POINT ( 'NONE',  ( -6.972266317189433020E-16, -72.25000000000000000, -5.000000000000000000 ) ) ;
#29276=ORIENTED_EDGE ( 'NONE', *, *, #38635, .T. ) ;
#29277=CARTESIAN_POINT ( 'NONE',  ( 2.229367062500001939, 20.02083333469892779, 3.861377020970579999 ) ) ;
#29279=CARTESIAN_POINT ( 'NONE',  ( -2.229367062500000163, -7.729166665301073991, -3.861377020970580443 ) ) ;
#29282=CARTESIAN_POINT ( 'NONE',  ( 4.458734124999999437, -166.4375000013655779, 0.000000000000000000 ) ) ;
#29283=CARTESIAN_POINT ( 'NONE',  ( -6.972266317189433020E-16, -24.24999999999999645, -5.000000000000000000 ) ) ;
#29286=CARTESIAN_POINT ( 'NONE',  ( 3.061616997868383141E-16, -151.7500000000000284, -5.000000000000000000 ) ) ;
#29287=CARTESIAN_POINT ( 'NONE',  ( 1.975475456537005874E-15, -49.62499999726880873, 5.000000000000000000 ) ) ;
#29289=CARTESIAN_POINT ( 'NONE',  ( 1.846868145590736310, -153.8750000013655779, 4.458734124999997661 ) ) ;
#29292=CARTESIAN_POINT ( 'NONE',  ( 1.975475456537005874E-15, -46.74999999999999289, 5.000000000000000000 ) ) ;
#29293=CARTESIAN_POINT ( 'NONE',  ( 2.071067811865401787, -162.8124999999999716, -5.000000000000074607 ) ) ;
#29294=VERTEX_POINT ( 'NONE', #4694 ) ;
#29298=CARTESIAN_POINT ( 'NONE',  ( 2.500000000000002220, 3.333333333333333925, 4.330127018922192761 ) ) ;
#29299=CARTESIAN_POINT ( 'NONE',  ( -4.458734124999999437, -68.39583333196773651, -2.574251347313719407 ) ) ;
#29300=CARTESIAN_POINT ( 'NONE',  ( -2.499999999999996447, -30.70833333060214443, 4.330127018922195425 ) ) ;
#29301=CARTESIAN_POINT ( 'NONE',  ( 5.000000000000000888, -1.458333330602149092, 2.886751345948126879 ) ) ;
#29302=CARTESIAN_POINT ( 'NONE',  ( -2.229367062499996610, -36.14583333196773651, 3.861377020970582219 ) ) ;
#29305=DIRECTION ( 'NONE',  ( -0.000000000000000000, 1.000000000000000000, -0.000000000000000000 ) ) ;
#29307=CARTESIAN_POINT ( 'NONE',  ( -2.499999999999996447, -43.83333333333333570, 4.330127018922195425 ) ) ;
#29309=CARTESIAN_POINT ( 'NONE',  ( 4.458734124999999437, -69.81249999863439371, -5.460374474430324690E-16 ) ) ;
#29310=CARTESIAN_POINT ( 'NONE',  ( -3.152801135295367096, -145.3125000013655779, -3.152801135295367541 ) ) ;
#29311=CARTESIAN_POINT ( 'NONE',  ( -2.229367062499996610, -77.14583333196773651, 3.861377020970582219 ) ) ;
#29314=CARTESIAN_POINT ( 'NONE',  ( 9.457646018065525792E-16, -32.31249999863440792, 5.148502694627439702 ) ) ;
#29315=CARTESIAN_POINT ( 'NONE',  ( -5.000000000000000000, -71.95833333060214443, -2.886751345948128211 ) ) ;
#29320=CARTESIAN_POINT ( 'NONE',  ( 3.535533905932736864, -166.1250000000000284, 3.535533905932738641 ) ) ;
#29321=VERTEX_POINT ( 'NONE', #18558 ) ;
#29322=EDGE_CURVE ( 'NONE', #41425, #6544, #9213, .T. ) ;
#29324=CARTESIAN_POINT ( 'NONE',  ( -2.499999999999996447, -2.833333333333333481, 4.330127018922195425 ) ) ;
#29325=CARTESIAN_POINT ( 'NONE',  ( 2.229367062500001939, -59.22916666530106511, 3.861377020970579999 ) ) ;
#29330=CARTESIAN_POINT ( 'NONE',  ( -4.458734124999999437, 14.60416666803226171, -2.574251347313719407 ) ) ;
#29332=CARTESIAN_POINT ( 'NONE',  ( 1.975475456537005874E-15, -32.74999999999999289, 5.000000000000000000 ) ) ;
#29333=CARTESIAN_POINT ( 'NONE',  ( 1.846868145590736310, -164.6250000013656063, 4.458734124999997661 ) ) ;
#29337=CARTESIAN_POINT ( 'NONE',  ( -5.000000000000000000, -51.87499999726881583, 0.000000000000000000 ) ) ;
#29339=DIRECTION ( 'NONE',  ( -0.000000000000000000, 1.000000000000000000, -0.000000000000000000 ) ) ;
#29344=CARTESIAN_POINT ( 'NONE',  ( 1.339745962155612702, -61.29465819873851729, -5.000000000000000000 ) ) ;
#29348=CARTESIAN_POINT ( 'NONE',  ( -3.152548672688508926E-16, 7.187500001365594748, -5.148502694627439702 ) ) ;
#29349=CARTESIAN_POINT ( 'NONE',  ( 5.000000000000000000, -146.1250000027312126, 0.000000000000000000 ) ) ;
#29351=CARTESIAN_POINT ( 'NONE',  ( -3.535533905932737309, -150.7500000027312126, -3.535533905932738197 ) ) ;
#29352=CARTESIAN_POINT ( 'NONE',  ( -2.499999999999996447, 29.16666666666666785, 4.330127018922195425 ) ) ;
#29355=AXIS2_PLACEMENT_3D ( 'NONE', #38269, #7744, #7430 ) ;
#29356=VECTOR ( 'NONE', #45037, 1000.000000000000000 ) ;
#29358=CARTESIAN_POINT ( 'NONE',  ( -2.071067811865478170, -142.3125000000000000, 5.000000000000000000 ) ) ;
#29360=CARTESIAN_POINT ( 'NONE',  ( -8.190561711645485556E-16, -166.9375000013655779, 4.458734124999999437 ) ) ;
#29361=CARTESIAN_POINT ( 'NONE',  ( 4.458734124999998549, -32.72916666530106511, -2.574251347313721627 ) ) ;
#29363=CARTESIAN_POINT ( 'NONE',  ( 0.000000000000000000, -170.0000000000000000, 0.000000000000000000 ) ) ;
#29365=CARTESIAN_POINT ( 'NONE',  ( 2.730187237215162345E-16, -145.1875000013656063, -4.458734124999999437 ) ) ;
#29367=CARTESIAN_POINT ( 'NONE',  ( -4.458734124999999437, 28.35416666803226349, -2.574251347313719407 ) ) ;
#29369=CARTESIAN_POINT ( 'NONE',  ( 4.458734124999998549, -62.97916666530106511, -2.574251347313721627 ) ) ;
#29372=CARTESIAN_POINT ( 'NONE',  ( -5.000000000000000000, 19.00000000000000000, 0.000000000000000000 ) ) ;
#29374=CARTESIAN_POINT ( 'NONE',  ( -5.000000000000000000, -89.00000000000000000, 0.000000000000000000 ) ) ;
#29375=CARTESIAN_POINT ( 'NONE',  ( 9.457646018065525792E-16, -7.062499998634404363, 5.148502694627439702 ) ) ;
#29376=CARTESIAN_POINT ( 'NONE',  ( 3.061616997868383141E-16, -168.7500000000000000, -5.000000000000000000 ) ) ;
#29377=CARTESIAN_POINT ( 'NONE',  ( 0.000000000000000000, -170.0000000000000000, 5.000000000000000000 ) ) ;
#29382=CARTESIAN_POINT ( 'NONE',  ( 4.458734125000001214, -52.89583333196772941, 2.574251347313718519 ) ) ;
#29383=CARTESIAN_POINT ( 'NONE',  ( 4.458734124999999437, -157.7500000013656063, 1.846868145590737864 ) ) ;
#29384=EDGE_CURVE ( 'NONE', #26085, #43575, #43530, .T. ) ;
#29385=CARTESIAN_POINT ( 'NONE',  ( 1.060575238724906964E-15, -47.62499999726881583, 5.773502691896257311 ) ) ;
#29386=ORIENTED_EDGE ( 'NONE', *, *, #59398, .T. ) ;
#29387=CARTESIAN_POINT ( 'NONE',  ( 4.458734124999998549, 4.020833334698926009, -2.574251347313721627 ) ) ;
#29388=ADVANCED_FACE ( 'NONE', ( #59373 ), #54550, .T. ) ;
#29389=VERTEX_POINT ( 'NONE', #45211 ) ;
#29390=FACE_OUTER_BOUND ( 'NONE', #44700, .T. ) ;
#29392=CARTESIAN_POINT ( 'NONE',  ( -1.846868145590737420, -155.7500000013655779, 4.458734124999999437 ) ) ;
#29393=ORIENTED_EDGE ( 'NONE', *, *, #19048, .T. ) ;
#29398=CARTESIAN_POINT ( 'NONE',  ( -4.458734124999998549, -41.47916666530107221, 2.574251347313722516 ) ) ;
#29401=CARTESIAN_POINT ( 'NONE',  ( 5.000000000000000000, 9.625000002731184168, -6.123233995736766282E-16 ) ) ;
#29403=CARTESIAN_POINT ( 'NONE',  ( 6.123233995736766282E-16, -170.0000000000000000, -5.000000000000000000 ) ) ;
#29405=CARTESIAN_POINT ( 'NONE',  ( -4.458734124999999437, -88.56249999863439371, 0.000000000000000000 ) ) ;
#29414=CARTESIAN_POINT ( 'NONE',  ( -4.999999999999998224, -78.79166666393547303, 2.886751345948131764 ) ) ;
#29418=CYLINDRICAL_SURFACE ( 'NONE', #31447, 5.000000000000000000 ) ;
#29424=CARTESIAN_POINT ( 'NONE',  ( -5.000000000000000888, -155.6875000027312126, -2.071067811865475949 ) ) ;
#29426=CARTESIAN_POINT ( 'NONE',  ( 3.535533905932738197, -163.0000000027312126, -3.535533905932738197 ) ) ;
#29432=( BOUNDED_CURVE ( )  B_SPLINE_CURVE ( 2, ( #58408, #37852, #14336, #29424, #23059, #33957, #28184, #53578, #33331 ),
 .UNSPECIFIED., .F., .F. ) 
 B_SPLINE_CURVE_WITH_KNOTS ( ( 3, 2, 2, 2, 3 ),
 ( 0.4416666666666670404, 0.4458333333333337478, 0.4500000000000003997, 0.4541666666666671071, 0.4583333333333337589 ),
 .UNSPECIFIED. ) 
 CURVE ( )  GEOMETRIC_REPRESENTATION_ITEM ( )  RATIONAL_B_SPLINE_CURVE ( ( 0.9999999999999928946, 0.9238795325112938439, 1.000000000000000000, 0.9238795325112867385, 1.000000000000000000, 0.9238795325112867385, 1.000000000000000000, 0.9238795325112786339, 1.000000000000008216 ) ) 
 REPRESENTATION_ITEM ( '' )  );
#29438=CARTESIAN_POINT ( 'NONE',  ( 4.458734124999998549, -12.72916666530106866, -2.574251347313721627 ) ) ;
#29439=CARTESIAN_POINT ( 'NONE',  ( 0.000000000000000000, -170.0000000000000000, 5.000000000000000000 ) ) ;
#29440=CARTESIAN_POINT ( 'NONE',  ( -5.000000000000000000, -156.5000000000000000, -6.123233995736766282E-16 ) ) ;
#29442=VERTEX_POINT ( 'NONE', #1177 ) ;
#29443=CARTESIAN_POINT ( 'NONE',  ( 4.458734125000000326, -42.14583333196773651, 2.574251347313718519 ) ) ;
#29444=AXIS2_PLACEMENT_3D ( 'NONE', #25160, #55079, #30623 ) ;
#29449=VECTOR ( 'NONE', #21521, 1000.000000000000000 ) ;
#29450=CARTESIAN_POINT ( 'NONE',  ( -4.458734124999999437, 7.687500001365594748, 0.000000000000000000 ) ) ;
#29454=AXIS2_PLACEMENT_3D ( 'NONE', #31516, #17375, #41480 ) ;
#29455=CARTESIAN_POINT ( 'NONE',  ( -2.499999999999996447, -68.83333333333332860, 4.330127018922195425 ) ) ;
#29456=CARTESIAN_POINT ( 'NONE',  ( 9.457646018065525792E-16, -86.31249999863439371, 5.148502694627439702 ) ) ;
#29457=CARTESIAN_POINT ( 'NONE',  ( -2.229367062499996610, 20.60416666803225993, 3.861377020970582219 ) ) ;
#29459=CARTESIAN_POINT ( 'NONE',  ( -5.000000000000000000, 12.04166666939785379, -2.886751345948128211 ) ) ;
#29462=ORIENTED_EDGE ( 'NONE', *, *, #27609, .F. ) ;
#29463=CARTESIAN_POINT ( 'NONE',  ( 2.500000000000002220, -35.66666666666666430, 4.330127018922192761 ) ) ;
#29464=CARTESIAN_POINT ( 'NONE',  ( -4.458734124999998549, -40.22916666530107932, 2.574251347313722516 ) ) ;
#29465=CARTESIAN_POINT ( 'NONE',  ( 2.499999999999998668, -33.20833333060215153, -4.330127018922193649 ) ) ;
#29466=CARTESIAN_POINT ( 'NONE',  ( 2.229367062500001939, -64.97916666530106511, 3.861377020970579999 ) ) ;
#29467=VERTEX_POINT ( 'NONE', #35568 ) ;
#29469=CARTESIAN_POINT ( 'NONE',  ( 9.457646018065525792E-16, -11.06249999863440969, 5.148502694627439702 ) ) ;
#29470=EDGE_CURVE ( 'NONE', #43179, #17081, #50196, .T. ) ;
#29471=CARTESIAN_POINT ( 'NONE',  ( -2.229367062500000163, -15.72916666530107399, -3.861377020970580443 ) ) ;
#29473=CARTESIAN_POINT ( 'NONE',  ( -5.000000000000000000, -81.00000000000000000, 0.000000000000000000 ) ) ;
#29474=CARTESIAN_POINT ( 'NONE',  ( 4.458734125000000326, -167.3750000013656347, -1.846868145590734978 ) ) ;
#29476=CARTESIAN_POINT ( 'NONE',  ( 1.060575238724906964E-15, -81.62499999726881583, 5.773502691896257311 ) ) ;
#29477=CARTESIAN_POINT ( 'NONE',  ( -1.339745962155610925, -48.66965819600732601, 5.000000000000000000 ) ) ;
#29478=VERTEX_POINT ( 'NONE', #5343 ) ;
#29480=CARTESIAN_POINT ( 'NONE',  ( 2.229367062499998831, -27.89583333196774007, -3.861377020970580887 ) ) ;
#29482=CARTESIAN_POINT ( 'NONE',  ( -4.458734125000000326, -168.2500000013656063, -1.846868145590735644 ) ) ;
#29484=CARTESIAN_POINT ( 'NONE',  ( 2.500000000000002220, -55.54166666393548013, 4.330127018922192761 ) ) ;
#29485=ORIENTED_EDGE ( 'NONE', *, *, #40609, .T. ) ;
#29489=CARTESIAN_POINT ( 'NONE',  ( 4.458734124999999437, -144.6250000013655779, -1.846868145590734978 ) ) ;
#29494=CARTESIAN_POINT ( 'NONE',  ( -2.500000000000000444, -0.1666666666666656582, -4.330127018922193649 ) ) ;
#29496=VECTOR ( 'NONE', #35510, 1000.000000000000000 ) ;
#29499=CARTESIAN_POINT ( 'NONE',  ( -8.190561711645485556E-16, -140.9375000013656063, 4.458734124999999437 ) ) ;
#29504=CARTESIAN_POINT ( 'NONE',  ( -2.229367062499996610, -71.39583333196773651, 3.861377020970582219 ) ) ;
#29505=CARTESIAN_POINT ( 'NONE',  ( -5.000000000000000888, -144.5625000027311842, 2.071067811865474617 ) ) ;
#29506=CARTESIAN_POINT ( 'NONE',  ( 0.000000000000000000, -170.0000000000000000, 0.000000000000000000 ) ) ;
#29516=CARTESIAN_POINT ( 'NONE',  ( 4.458734125000000326, 21.85416666803225993, 2.574251347313718519 ) ) ;
#29517=CARTESIAN_POINT ( 'NONE',  ( 1.255007937094098239E-14, 22.87500000273118772, -4.999999999999999112 ) ) ;
#29523=CARTESIAN_POINT ( 'NONE',  ( -4.458734124999997661, 0.7708333346989268975, 2.574251347313722516 ) ) ;
#29524=CARTESIAN_POINT ( 'NONE',  ( -3.152548672688508926E-16, -25.81249999863440792, -5.148502694627439702 ) ) ;
#29528=CARTESIAN_POINT ( 'NONE',  ( 2.229367062500001939, 28.02083333469892779, 3.861377020970579999 ) ) ;
#29530=EDGE_CURVE ( 'NONE', #43260, #60995, #15572, .T. ) ;
#29533=CARTESIAN_POINT ( 'NONE',  ( 4.458734124999998549, -72.97916666530107932, -2.574251347313721627 ) ) ;
#29536=CARTESIAN_POINT ( 'NONE',  ( -2.500000000000000444, -11.04166666393547835, -4.330127018922193649 ) ) ;
#29537=ORIENTED_EDGE ( 'NONE', *, *, #12938, .F. ) ;
#29538=CARTESIAN_POINT ( 'NONE',  ( -3.535533905932738641, -140.3750000000000000, 3.535533905932737309 ) ) ;
#29539=EDGE_CURVE ( 'NONE', #25625, #29321, #41640, .T. ) ;
#29541=FACE_OUTER_BOUND ( 'NONE', #53401, .T. ) ;
#29543=CARTESIAN_POINT ( 'NONE',  ( 2.500000000000002220, -16.66666666666666430, 4.330127018922192761 ) ) ;
#29544=CARTESIAN_POINT ( 'NONE',  ( -2.229367062500000163, -23.47916666530107221, -3.861377020970580443 ) ) ;
#29545=EDGE_CURVE ( 'NONE', #40158, #20174, #46379, .T. ) ;
#29546=CARTESIAN_POINT ( 'NONE',  ( -4.458734124999999437, -85.31249999863439371, 0.000000000000000000 ) ) ;
#29548=CARTESIAN_POINT ( 'NONE',  ( -3.152801135295367985, -166.0625000013656063, 3.152801135295367096 ) ) ;
#29549=CARTESIAN_POINT ( 'NONE',  ( 2.499999999999998668, -19.20833333060214798, -4.330127018922193649 ) ) ;
#29550=CARTESIAN_POINT ( 'NONE',  ( 4.458734124999999437, -50.81249999863440792, -5.460374474430324690E-16 ) ) ;
#29551=ORIENTED_EDGE ( 'NONE', *, *, #46424, .F. ) ;
#29554=CARTESIAN_POINT ( 'NONE',  ( 2.229367062499998831, -0.8958333319677401763, -3.861377020970580887 ) ) ;
#29557=CARTESIAN_POINT ( 'NONE',  ( 5.000000000000000000, -66.41666666666667140, -2.886751345948129988 ) ) ;
#29559=CARTESIAN_POINT ( 'NONE',  ( 4.458734125000000326, -157.6250000013655779, -1.846868145590734978 ) ) ;
#29561=CARTESIAN_POINT ( 'NONE',  ( -4.999999999999998224, -80.79166666393547303, 2.886751345948131764 ) ) ;
#29562=CARTESIAN_POINT ( 'NONE',  ( 5.000000000000000000, -164.0625000000000000, 2.071067811865478614 ) ) ;
#29564=EDGE_CURVE ( 'NONE', #24132, #56134, #48420, .T. ) ;
#29567=CARTESIAN_POINT ( 'NONE',  ( 4.458734125000001214, -12.14583333196774007, 2.574251347313718519 ) ) ;
#29568=CARTESIAN_POINT ( 'NONE',  ( 4.458734124999999437, -45.06249999863440081, -5.460374474430324690E-16 ) ) ;
#29569=FACE_OUTER_BOUND ( 'NONE', #44229, .T. ) ;
#29570=CARTESIAN_POINT ( 'NONE',  ( 1.846868145590735200, -150.2500000013656063, -4.458734125000000326 ) ) ;
#29574=CARTESIAN_POINT ( 'NONE',  ( 6.123233995736766282E-16, -170.0000000000000000, -5.000000000000000000 ) ) ;
#29575=CARTESIAN_POINT ( 'NONE',  ( -6.972266317189433020E-16, -45.12499999726880162, -5.000000000000000000 ) ) ;
#29577=CARTESIAN_POINT ( 'NONE',  ( -4.999999999999998224, -61.91666666666666430, 2.886751345948131764 ) ) ;
#29578=ORIENTED_EDGE ( 'NONE', *, *, #20929, .T. ) ;
#29582=CARTESIAN_POINT ( 'NONE',  ( -1.339745962155613812, -51.20534180126148271, -5.000000000000000000 ) ) ;
#29583=CARTESIAN_POINT ( 'NONE',  ( -2.229367062500000163, -3.479166665301069994, -3.861377020970580443 ) ) ;
#29585=CARTESIAN_POINT ( 'NONE',  ( 3.152801135295366208, -149.5625000013655779, 3.152801135295367985 ) ) ;
#29586=VECTOR ( 'NONE', #16478, 1000.000000000000000 ) ;
#29588=VERTEX_POINT ( 'NONE', #47124 ) ;
#29593=CARTESIAN_POINT ( 'NONE',  ( 1.975475456537005874E-15, -81.62499999726881583, 5.000000000000000000 ) ) ;
#29594=DIRECTION ( 'NONE',  ( -0.000000000000000000, 1.000000000000000000, -0.000000000000000000 ) ) ;
#29601=DIRECTION ( 'NONE',  ( 0.000000000000000000, 0.000000000000000000, 1.000000000000000000 ) ) ;
#29602=CARTESIAN_POINT ( 'NONE',  ( 4.458734125000000326, 19.10416666803225638, 2.574251347313718519 ) ) ;
#29604=ORIENTED_EDGE ( 'NONE', *, *, #5971, .F. ) ;
#29605=CARTESIAN_POINT ( 'NONE',  ( 9.457646018065525792E-16, -6.312499998634403475, 5.148502694627439702 ) ) ;
#29608=CARTESIAN_POINT ( 'NONE',  ( -4.458734125000001214, -168.8750000013655779, 1.846868145590734089 ) ) ;
#29609=CARTESIAN_POINT ( 'NONE',  ( 2.500000000000002220, -63.54166666393547303, 4.330127018922192761 ) ) ;
#29613=AXIS2_PLACEMENT_3D ( 'NONE', #45832, #40037, #45190 ) ;
#29614=CARTESIAN_POINT ( 'NONE',  ( -6.972266317189433020E-16, -77.25000000000000000, -5.000000000000000000 ) ) ;
#29615=DIRECTION ( 'NONE',  ( -0.000000000000000000, 1.000000000000000000, -0.000000000000000000 ) ) ;
#29616=LINE ( 'NONE', #24805, #49061 ) ;
#29617=CARTESIAN_POINT ( 'NONE',  ( 4.458734124999999437, -151.6875000013656063, 0.000000000000000000 ) ) ;
#29619=CYLINDRICAL_SURFACE ( 'NONE', #34602, 5.000000000000000000 ) ;
#29621=VERTEX_POINT ( 'NONE', #42289 ) ;
#29625=CARTESIAN_POINT ( 'NONE',  ( -2.499999999999996447, -0.8333333333333317050, 4.330127018922195425 ) ) ;
#29626=CARTESIAN_POINT ( 'NONE',  ( -4.458734124999999437, -64.39583333196773651, -2.574251347313719407 ) ) ;
#29627=( BOUNDED_CURVE ( )  B_SPLINE_CURVE ( 2, ( #53859, #53239, #28787, #9477, #58381, #4976, #48403, #4345, #33930 ),
 .UNSPECIFIED., .F., .F. ) 
 B_SPLINE_CURVE_WITH_KNOTS ( ( 3, 2, 2, 2, 3 ),
 ( 0.6354166666666666297, 0.6361111111111110716, 0.6374999999999999556, 0.6388888888888888395, 0.6395833333333332815 ),
 .UNSPECIFIED. ) 
 CURVE ( )  GEOMETRIC_REPRESENTATION_ITEM ( )  RATIONAL_B_SPLINE_CURVE ( ( 0.9330127018922194093, 0.9330127018922194093, 1.000000000000000000, 0.8660254037844387076, 1.000000000000000000, 0.8660254037844387076, 1.000000000000000000, 0.9330127018922194093, 0.9330127018922194093 ) ) 
 REPRESENTATION_ITEM ( '' )  );
#29628=DIRECTION ( 'NONE',  ( 0.8660254037844410391, -0.4999999999999958367, -0.000000000000000000 ) ) ;
#29629=CARTESIAN_POINT ( 'NONE',  ( 1.060575238724906964E-15, -2.624999997268815388, 5.773502691896257311 ) ) ;
#29630=CARTESIAN_POINT ( 'NONE',  ( 4.458734124999999437, -33.81249999863440792, -5.460374474430324690E-16 ) ) ;
#29632=CARTESIAN_POINT ( 'NONE',  ( 5.000000000000000000, -153.1875000027312126, 2.071067811865478614 ) ) ;
#29633=CARTESIAN_POINT ( 'NONE',  ( -1.339745962155610925, -47.66965819600734022, 5.000000000000000000 ) ) ;
#29636=CARTESIAN_POINT ( 'NONE',  ( -2.499999999999996447, -49.83333333333332860, 4.330127018922195425 ) ) ;
#29637=CYLINDRICAL_SURFACE ( 'NONE', #54166, 5.000000000000000000 ) ;
#29639=CARTESIAN_POINT ( 'NONE',  ( 1.339745962155615144, -32.58034179853029144, 4.999999999999999112 ) ) ;
#29640=CARTESIAN_POINT ( 'NONE',  ( 4.458734125000001214, -69.89583333196773651, 2.574251347313718519 ) ) ;
#29641=CARTESIAN_POINT ( 'NONE',  ( 3.152801135295366208, -142.8125000013655779, 3.152801135295367985 ) ) ;
#29642=CARTESIAN_POINT ( 'NONE',  ( -2.229367062500000163, -82.47916666530106511, -3.861377020970580443 ) ) ;
#29645=CARTESIAN_POINT ( 'NONE',  ( 2.229367062499998831, -28.89583333196774007, -3.861377020970580887 ) ) ;
#29646=CARTESIAN_POINT ( 'NONE',  ( 1.060575238724906964E-15, -72.62499999726880162, 5.773502691896257311 ) ) ;
#29648=ORIENTED_EDGE ( 'NONE', *, *, #2745, .F. ) ;
#29656=CARTESIAN_POINT ( 'NONE',  ( 5.000000000000000000, -12.41666666666666607, -2.886751345948130876 ) ) ;
#29657=CARTESIAN_POINT ( 'NONE',  ( 2.229367062500001939, -57.22916666530107932, 3.861377020970579999 ) ) ;
#29662=CARTESIAN_POINT ( 'NONE',  ( -4.458734124999998549, 13.77083333469892779, 2.574251347313722516 ) ) ;
#29665=CARTESIAN_POINT ( 'NONE',  ( 4.458734124999999437, -163.4375000013655779, 0.000000000000000000 ) ) ;
#29666=ORIENTED_EDGE ( 'NONE', *, *, #52400, .F. ) ;
#29670=CARTESIAN_POINT ( 'NONE',  ( 1.339745962155612702, -40.16965819600733312, -5.000000000000000000 ) ) ;
#29676=( BOUNDED_CURVE ( )  B_SPLINE_CURVE ( 2, ( #8517, #51953, #37166, #7891, #61612, #13341, #27188, #46804, #27811 ),
 .UNSPECIFIED., .F., .F. ) 
 B_SPLINE_CURVE_WITH_KNOTS ( ( 3, 2, 2, 2, 3 ),
 ( 0.1645833333333333315, 0.1652777777777777735, 0.1666666666666666574, 0.1680555555555555691, 0.1687500000000000111 ),
 .UNSPECIFIED. ) 
 CURVE ( )  GEOMETRIC_REPRESENTATION_ITEM ( )  RATIONAL_B_SPLINE_CURVE ( ( 0.9330127018922194093, 0.9330127018922194093, 1.000000000000000000, 0.8660254037844387076, 1.000000000000000000, 0.8660254037844387076, 1.000000000000000000, 0.9330127018922194093, 0.9330127018922194093 ) ) 
 REPRESENTATION_ITEM ( '' )  );
#29680=CARTESIAN_POINT ( 'NONE',  ( 4.458734125000000326, 7.854166668032260823, 2.574251347313718519 ) ) ;
#29682=CARTESIAN_POINT ( 'NONE',  ( -5.000000000000000000, -9.874999997268815832, 0.000000000000000000 ) ) ;
#29684=CARTESIAN_POINT ( 'NONE',  ( 3.535533905932736864, -148.2500000027311842, 3.535533905932738641 ) ) ;
#29688=CARTESIAN_POINT ( 'NONE',  ( 2.071067811865476394, -142.1875000000000284, 5.000000000000000000 ) ) ;
#29690=CARTESIAN_POINT ( 'NONE',  ( 4.458734124999999437, -163.6875000013655779, 0.000000000000000000 ) ) ;
#29691=CARTESIAN_POINT ( 'NONE',  ( -4.458734124999997661, -38.22916666530107932, 2.574251347313722516 ) ) ;
#29692=CARTESIAN_POINT ( 'NONE',  ( -5.000000000000000000, -33.00000000000000000, 0.000000000000000000 ) ) ;
#29695=CARTESIAN_POINT ( 'NONE',  ( 1.846868145590736310, -142.6250000013655779, 4.458734124999999437 ) ) ;
#29697=CARTESIAN_POINT ( 'NONE',  ( -3.152548672688508926E-16, 28.18750000136559564, -5.148502694627439702 ) ) ;
#29698=ORIENTED_EDGE ( 'NONE', *, *, #60875, .T. ) ;
#29699=CARTESIAN_POINT ( 'NONE',  ( -3.152548672688508926E-16, -61.81249999863440081, -5.148502694627439702 ) ) ;
#29701=CARTESIAN_POINT ( 'NONE',  ( 1.975475456537005874E-15, 13.37500000273118417, 5.000000000000000000 ) ) ;
#29702=CARTESIAN_POINT ( 'NONE',  ( -4.999999999999999112, 11.08333333333333393, 2.886751345948131764 ) ) ;
#29703=CARTESIAN_POINT ( 'NONE',  ( 9.457646018065525792E-16, -53.06249999863440792, 5.148502694627439702 ) ) ;
#29704=CARTESIAN_POINT ( 'NONE',  ( -4.458734124999999437, -5.395833331967740953, -2.574251347313719407 ) ) ;
#29705=CARTESIAN_POINT ( 'NONE',  ( 2.071067811865508812, -166.3125000027312126, 4.999999999999968026 ) ) ;
#29707=CARTESIAN_POINT ( 'NONE',  ( 5.000000000000000000, -158.1875000027312126, 2.071067811865478614 ) ) ;
#29708=CARTESIAN_POINT ( 'NONE',  ( 1.062108568985190270E-13, -10.25000000000000355, -4.999999999999999112 ) ) ;
#29712=CARTESIAN_POINT ( 'NONE',  ( -2.229367062500000163, -54.47916666530107221, -3.861377020970580443 ) ) ;
#29713=CARTESIAN_POINT ( 'NONE',  ( 2.730187237215162345E-16, -155.4375000013655779, -4.458734124999999437 ) ) ;
#29714=CARTESIAN_POINT ( 'NONE',  ( -3.535250795749689387E-16, -58.12499999726880162, -5.773502691896257311 ) ) ;
#29716=CARTESIAN_POINT ( 'NONE',  ( 2.229367062499998831, 5.104166668032261711, -3.861377020970580887 ) ) ;
#29719=CARTESIAN_POINT ( 'NONE',  ( 4.458734124999999437, -158.4375000013655779, 0.000000000000000000 ) ) ;
#29720=VERTEX_POINT ( 'NONE', #32322 ) ;
#29723=LINE ( 'NONE', #48713, #27285 ) ;
#29725=CARTESIAN_POINT ( 'NONE',  ( 5.000000000000000000, -153.0000000000000284, 0.000000000000000000 ) ) ;
#29727=CARTESIAN_POINT ( 'NONE',  ( 4.458734125000001214, -45.14583333196774362, 2.574251347313718519 ) ) ;
#29728=VERTEX_POINT ( 'NONE', #51952 ) ;
#29729=CARTESIAN_POINT ( 'NONE',  ( 0.000000000000000000, -170.0000000000000000, 0.000000000000000000 ) ) ;
#29731=CARTESIAN_POINT ( 'NONE',  ( -6.972266317189433020E-16, 3.875000002731185500, -5.000000000000000000 ) ) ;
#29732=ORIENTED_EDGE ( 'NONE', *, *, #57478, .T. ) ;
#29733=CARTESIAN_POINT ( 'NONE',  ( -3.152548672688508926E-16, -88.81249999863439371, -5.148502694627439702 ) ) ;
#29745=CARTESIAN_POINT ( 'NONE',  ( -6.972266317189433020E-16, -42.12499999726880873, -5.000000000000000000 ) ) ;
#29746=CARTESIAN_POINT ( 'NONE',  ( -1.339745962155613812, -67.08034179853029855, -5.000000000000000000 ) ) ;
#29747=CARTESIAN_POINT ( 'NONE',  ( 9.457646018065525792E-16, -90.31249999863439371, 5.148502694627439702 ) ) ;
#29751=CARTESIAN_POINT ( 'NONE',  ( -5.000000000000000888, -143.5625000027311842, 2.071067811865474617 ) ) ;
#29753=CARTESIAN_POINT ( 'NONE',  ( 3.061616997868383141E-16, -161.8750000027311842, -5.000000000000000000 ) ) ;
#29764=CARTESIAN_POINT ( 'NONE',  ( 4.458734124999999437, -19.81249999863440081, -5.460374474430324690E-16 ) ) ;
#29766=CARTESIAN_POINT ( 'NONE',  ( -9.184850993605147944E-16, -156.2500000000000000, 5.000000000000000000 ) ) ;
#29769=CARTESIAN_POINT ( 'NONE',  ( -4.458734124999999437, -44.64583333196773651, -2.574251347313719407 ) ) ;
#29770=CARTESIAN_POINT ( 'NONE',  ( -1.339745962155614034, 26.20534180126147561, 4.999999999999999112 ) ) ;
#29772=CARTESIAN_POINT ( 'NONE',  ( -2.499999999999996447, 27.29166666939785202, 4.330127018922195425 ) ) ;
#29775=VECTOR ( 'NONE', #32975, 1000.000000000000000 ) ;
#29776=CARTESIAN_POINT ( 'NONE',  ( -4.458734124999998549, 11.77083333469892601, 2.574251347313722516 ) ) ;
#29777=CARTESIAN_POINT ( 'NONE',  ( -5.000000000000000000, -44.00000000000000000, 0.000000000000000000 ) ) ;
#29778=CARTESIAN_POINT ( 'NONE',  ( 5.275681513340003914E-14, 11.74999999999999645, -5.000000000000000000 ) ) ;
#29780=CARTESIAN_POINT ( 'NONE',  ( -2.229367062500000163, 19.27083333469892779, -3.861377020970580443 ) ) ;
#29782=CARTESIAN_POINT ( 'NONE',  ( -5.000000000000000000, 7.041666669397851130, -2.886751345948128211 ) ) ;
#29786=DIRECTION ( 'NONE',  ( -0.000000000000000000, 1.000000000000000000, -0.000000000000000000 ) ) ;
#29787=CARTESIAN_POINT ( 'NONE',  ( -4.458734124999999437, -39.31249999863440081, 0.000000000000000000 ) ) ;
#29788=CARTESIAN_POINT ( 'NONE',  ( 5.000000000000000888, -39.45833333060214443, 2.886751345948126879 ) ) ;
#29789=ORIENTED_EDGE ( 'NONE', *, *, #50875, .F. ) ;
#29791=CARTESIAN_POINT ( 'NONE',  ( -4.458734124999998549, -14.22916666530107221, 2.574251347313722516 ) ) ;
#29792=CARTESIAN_POINT ( 'NONE',  ( -3.152548672688508926E-16, -11.81249999863440969, -5.148502694627439702 ) ) ;
#29794=CARTESIAN_POINT ( 'NONE',  ( 1.060575238724906964E-15, -84.74999999999998579, 5.773502691896257311 ) ) ;
#29795=CARTESIAN_POINT ( 'NONE',  ( -4.999999999999998224, 1.208333336064518981, 2.886751345948131764 ) ) ;
#29798=CARTESIAN_POINT ( 'NONE',  ( 5.000000000000000888, -80.45833333060213022, 2.886751345948126879 ) ) ;
#29799=CARTESIAN_POINT ( 'NONE',  ( -5.000000000000000000, -32.08333333333332860, -2.886751345948128211 ) ) ;
#29802=CARTESIAN_POINT ( 'NONE',  ( 4.458734125000001214, -28.14583333196774007, 2.574251347313718519 ) ) ;
#29803=CARTESIAN_POINT ( 'NONE',  ( 1.975475456537005874E-15, -52.75000000000000000, 5.000000000000000000 ) ) ;
#29804=ORIENTED_EDGE ( 'NONE', *, *, #35657, .T. ) ;
#29807=CARTESIAN_POINT ( 'NONE',  ( 3.152801135295367541, -162.5625000013656063, -3.152801135295367541 ) ) ;
#29809=CARTESIAN_POINT ( 'NONE',  ( 3.535533905932738197, -147.8750000000000000, -3.535533905932738197 ) ) ;
#29810=ORIENTED_EDGE ( 'NONE', *, *, #11348, .T. ) ;
#29813=CARTESIAN_POINT ( 'NONE',  ( -2.229367062500000163, -72.72916666530107932, -3.861377020970580443 ) ) ;
#29816=CARTESIAN_POINT ( 'NONE',  ( -1.846868145590737420, -146.0000000013655779, 4.458734124999997661 ) ) ;
#29817=CARTESIAN_POINT ( 'NONE',  ( -1.510657702057710340E-15, 28.25000000000000000, 5.000000000000000000 ) ) ;
#29818=ADVANCED_FACE ( 'NONE', ( #28747 ), #4942, .T. ) ;
#29828=CARTESIAN_POINT ( 'NONE',  ( -4.458734124999999437, -74.64583333196773651, -2.574251347313719407 ) ) ;
#29829=LINE ( 'NONE', #45273, #14775 ) ;
#29831=LINE ( 'NONE', #25337, #60356 ) ;
#29834=LINE ( 'NONE', #54290, #14081 ) ;
#29835=CARTESIAN_POINT ( 'NONE',  ( 2.500000000000002220, -15.66666666666666963, 4.330127018922192761 ) ) ;
#29841=CARTESIAN_POINT ( 'NONE',  ( 4.458734124999998549, 20.02083333469892779, -2.574251347313721627 ) ) ;
#29842=CARTESIAN_POINT ( 'NONE',  ( -1.339745962155611370, 26.79465819873851729, -5.000000000000000888 ) ) ;
#29846=ADVANCED_FACE ( 'NONE', ( #57419 ), #53204, .T. ) ;
#29849=CARTESIAN_POINT ( 'NONE',  ( -2.229367062499996610, 0.8541666680322613781, 3.861377020970582219 ) ) ;
#29850=CARTESIAN_POINT ( 'NONE',  ( -2.229367062499996610, -32.39583333196773651, 3.861377020970582219 ) ) ;
#29853=CARTESIAN_POINT ( 'NONE',  ( 9.457646018065525792E-16, 23.93750000136559564, 5.148502694627439702 ) ) ;
#29856=CARTESIAN_POINT ( 'NONE',  ( -2.229367062499996610, -70.39583333196773651, 3.861377020970582219 ) ) ;
#29858=CARTESIAN_POINT ( 'NONE',  ( -1.339745962155613812, -66.08034179853028434, -5.000000000000000000 ) ) ;
#29859=CARTESIAN_POINT ( 'NONE',  ( -5.000000000000000000, 24.04166666939785202, -2.886751345948128211 ) ) ;
#29861=CARTESIAN_POINT ( 'NONE',  ( 1.975475456537005874E-15, 6.249999999999998224, 5.000000000000000000 ) ) ;
#29863=CARTESIAN_POINT ( 'NONE',  ( 0.000000000000000000, -170.0000000000000000, 5.000000000000000000 ) ) ;
#29864=CARTESIAN_POINT ( 'NONE',  ( -3.535250795749689387E-16, -20.24999999999999645, -5.773502691896257311 ) ) ;
#29865=CARTESIAN_POINT ( 'NONE',  ( 2.229367062500001939, -20.97916666530107221, 3.861377020970579999 ) ) ;
#29867=EDGE_CURVE ( 'NONE', #54415, #31328, #62243, .T. ) ;
#29868=CARTESIAN_POINT ( 'NONE',  ( 4.458734125000000326, -80.89583333196773651, 2.574251347313718519 ) ) ;
#29869=CARTESIAN_POINT ( 'NONE',  ( 5.000000000000000000, -20.37499999726880873, -6.123233995736766282E-16 ) ) ;
#29870=CARTESIAN_POINT ( 'NONE',  ( 9.457646018065525792E-16, -50.06249999863440792, 5.148502694627439702 ) ) ;
#29871=ORIENTED_EDGE ( 'NONE', *, *, #15680, .T. ) ;
#29873=CARTESIAN_POINT ( 'NONE',  ( -5.000000000000000000, -27.95833333060214798, -2.886751345948128211 ) ) ;
#29874=CARTESIAN_POINT ( 'NONE',  ( 2.229367062500001939, 3.770833334698926009, 3.861377020970579999 ) ) ;
#29875=ORIENTED_EDGE ( 'NONE', *, *, #29539, .T. ) ;
#29877=CARTESIAN_POINT ( 'NONE',  ( -4.999999999999999112, -67.91666666666667140, 2.886751345948131764 ) ) ;
#29878=CARTESIAN_POINT ( 'NONE',  ( -1.846868145590737420, -151.0000000013656063, 4.458734124999999437 ) ) ;
#29880=CARTESIAN_POINT ( 'NONE',  ( -2.500000000000000444, -77.04166666393547303, -4.330127018922193649 ) ) ;
#29881=( BOUNDED_CURVE ( )  B_SPLINE_CURVE ( 2, ( #42450, #8377, #17398, #47293, #46656, #37632, #2602, #52442, #37013 ),
 .UNSPECIFIED., .F., .F. ) 
 B_SPLINE_CURVE_WITH_KNOTS ( ( 3, 2, 2, 2, 3 ),
 ( 0.9562500000000000444, 0.9569444444444444864, 0.9583333333333333703, 0.9597222222222222543, 0.9604166666666666963 ),
 .UNSPECIFIED. ) 
 CURVE ( )  GEOMETRIC_REPRESENTATION_ITEM ( )  RATIONAL_B_SPLINE_CURVE ( ( 0.9330127018922194093, 0.9330127018922194093, 1.000000000000000000, 0.8660254037844387076, 1.000000000000000000, 0.8660254037844387076, 1.000000000000000000, 0.9330127018922194093, 0.9330127018922194093 ) ) 
 REPRESENTATION_ITEM ( '' )  );
#29882=CARTESIAN_POINT ( 'NONE',  ( 3.061616997868383141E-16, -161.7500000000000000, -5.000000000000000000 ) ) ;
#29883=DIRECTION ( 'NONE',  ( 0.000000000000000000, 0.000000000000000000, 1.000000000000000000 ) ) ;
#29885=CARTESIAN_POINT ( 'NONE',  ( -4.458734124999999437, -11.64583333196773829, -2.574251347313719407 ) ) ;
#29886=CARTESIAN_POINT ( 'NONE',  ( 9.457646018065525792E-16, -44.31249999863440081, 5.148502694627439702 ) ) ;
#29887=DIRECTION ( 'NONE',  ( -0.000000000000000000, 1.000000000000000000, -0.000000000000000000 ) ) ;
#29888=CARTESIAN_POINT ( 'NONE',  ( -1.846868145590737420, -144.7500000013656063, 4.458734124999999437 ) ) ;
#29893=CARTESIAN_POINT ( 'NONE',  ( 9.457646018065525792E-16, 28.68750000136559208, 5.148502694627439702 ) ) ;
#29895=CARTESIAN_POINT ( 'NONE',  ( 1.975475456537005874E-15, -29.62499999726881228, 5.000000000000000000 ) ) ;
#29904=CARTESIAN_POINT ( 'NONE',  ( 2.229367062500001939, -4.979166665301071326, 3.861377020970579999 ) ) ;
#29906=CARTESIAN_POINT ( 'NONE',  ( -4.458734124999999437, -150.9375000013656063, -5.460374474430324690E-16 ) ) ;
#29907=( BOUNDED_CURVE ( )  B_SPLINE_CURVE ( 2, ( #3327, #61232, #61870, #8459, #36778, #7199, #17786, #22945, #22305 ),
 .UNSPECIFIED., .F., .F. ) 
 B_SPLINE_CURVE_WITH_KNOTS ( ( 3, 2, 2, 2, 3 ),
 ( 0.1770833333333333426, 0.1777777777777777846, 0.1791666666666666685, 0.1805555555555555525, 0.1812499999999999944 ),
 .UNSPECIFIED. ) 
 CURVE ( )  GEOMETRIC_REPRESENTATION_ITEM ( )  RATIONAL_B_SPLINE_CURVE ( ( 0.9330127018922194093, 0.9330127018922194093, 1.000000000000000000, 0.8660254037844387076, 1.000000000000000000, 0.8660254037844387076, 1.000000000000000000, 0.9330127018922194093, 0.9330127018922194093 ) ) 
 REPRESENTATION_ITEM ( '' )  );
#29917=CARTESIAN_POINT ( 'NONE',  ( 1.339745962155615144, 8.419658201469706782, 4.999999999999999112 ) ) ;
#29922=CYLINDRICAL_SURFACE ( 'NONE', #5785, 5.000000000000000000 ) ;
#29924=CARTESIAN_POINT ( 'NONE',  ( 4.458734124999999437, 20.18750000136559208, -5.460374474430324690E-16 ) ) ;
#29926=EDGE_LOOP ( 'NONE', ( #23956, #37508, #31132, #52761 ) ) ;
#29927=CARTESIAN_POINT ( 'NONE',  ( -3.152548672688508926E-16, -6.812499998634404363, -5.148502694627439702 ) ) ;
#29929=CARTESIAN_POINT ( 'NONE',  ( 1.846868145590735200, -163.2500000013655495, -4.458734125000000326 ) ) ;
#29930=CARTESIAN_POINT ( 'NONE',  ( 1.975475456537005874E-15, -88.74999999999998579, 5.000000000000000000 ) ) ;
#29931=EDGE_CURVE ( 'NONE', #5270, #51028, #30385, .T. ) ;
#29936=LINE ( 'NONE', #55, #35774 ) ;
#29937=DIRECTION ( 'NONE',  ( -0.000000000000000000, 1.000000000000000000, -0.000000000000000000 ) ) ;
#29938=CARTESIAN_POINT ( 'NONE',  ( -8.190561711645485556E-16, -153.9375000013655779, 4.458734124999999437 ) ) ;
#29946=CARTESIAN_POINT ( 'NONE',  ( 5.000000000000000888, -1.583333333333332593, 2.886751345948126879 ) ) ;
#29947=CARTESIAN_POINT ( 'NONE',  ( 2.229367062500001939, -66.97916666530106511, 3.861377020970579999 ) ) ;
#29948=CYLINDRICAL_SURFACE ( 'NONE', #2099, 5.000000000000000000 ) ;
#29949=CARTESIAN_POINT ( 'NONE',  ( -5.000000000000000000, -3.874999997268816720, 0.000000000000000000 ) ) ;
#29950=CARTESIAN_POINT ( 'NONE',  ( 4.458734125000001214, -32.89583333196774362, 2.574251347313718519 ) ) ;
#29951=ORIENTED_EDGE ( 'NONE', *, *, #26033, .F. ) ;
#29952=CYLINDRICAL_SURFACE ( 'NONE', #45081, 5.000000000000000000 ) ;
#29953=CARTESIAN_POINT ( 'NONE',  ( -4.999999999999998224, -47.79166666393547303, 2.886751345948131764 ) ) ;
#29954=ORIENTED_EDGE ( 'NONE', *, *, #17376, .T. ) ;
#29956=CARTESIAN_POINT ( 'NONE',  ( 5.000000000000000000, -49.41666666666667140, -2.886751345948129988 ) ) ;
#29957=CARTESIAN_POINT ( 'NONE',  ( 5.000000000000000888, -17.45833333060214443, 2.886751345948126879 ) ) ;
#29959=CARTESIAN_POINT ( 'NONE',  ( -6.972266317189433020E-16, 13.87500000273118594, -5.000000000000000000 ) ) ;
#29960=CARTESIAN_POINT ( 'NONE',  ( -4.458734124999998549, -68.22916666530107932, 2.574251347313722516 ) ) ;
#29961=CARTESIAN_POINT ( 'NONE',  ( 2.730187237215162345E-16, -144.4375000013656063, -4.458734124999999437 ) ) ;
#29962=CARTESIAN_POINT ( 'NONE',  ( 4.458734125000001214, -83.89583333196773651, 2.574251347313718519 ) ) ;
#29964=CARTESIAN_POINT ( 'NONE',  ( -3.152548672688508926E-16, -31.81249999863440792, -5.148502694627439702 ) ) ;
#29965=CARTESIAN_POINT ( 'NONE',  ( -3.535250795749689387E-16, -72.12499999726881583, -5.773502691896257311 ) ) ;
#29974=CARTESIAN_POINT ( 'NONE',  ( -2.499999999999996447, -75.70833333060214443, 4.330127018922195425 ) ) ;
#29975=CARTESIAN_POINT ( 'NONE',  ( 2.229367062499998831, -58.89583333196773651, -3.861377020970580887 ) ) ;
#29981=CARTESIAN_POINT ( 'NONE',  ( -2.229367062499996610, 14.85416666803226171, 3.861377020970582219 ) ) ;
#29983=CARTESIAN_POINT ( 'NONE',  ( 4.458734124999999437, -159.3750000013656063, -1.846868145590734978 ) ) ;
#29984=CYLINDRICAL_SURFACE ( 'NONE', #38867, 5.000000000000000000 ) ;
#29987=DIRECTION ( 'NONE',  ( -0.000000000000000000, 1.000000000000000000, -0.000000000000000000 ) ) ;
#29990=CARTESIAN_POINT ( 'NONE',  ( 5.000000000000000000, -36.50000000000000711, -6.123233995736766282E-16 ) ) ;
#29993=CARTESIAN_POINT ( 'NONE',  ( 5.000000000000000888, 12.54166666939785557, 2.886751345948126879 ) ) ;
#29997=EDGE_CURVE ( 'NONE', #1043, #25291, #25197, .T. ) ;
#30000=CARTESIAN_POINT ( 'NONE',  ( -4.458734124999997661, 5.520833334698926009, 2.574251347313722516 ) ) ;
#30001=CARTESIAN_POINT ( 'NONE',  ( 5.000000000000000888, -146.0625000027312126, -2.071067811865475505 ) ) ;
#30004=CARTESIAN_POINT ( 'NONE',  ( -9.184850993605147944E-16, -150.3750000027312126, 5.000000000000000000 ) ) ;
#30005=CARTESIAN_POINT ( 'NONE',  ( -5.000000000000000000, 28.91666666666666430, -2.886751345948128211 ) ) ;
#30009=( BOUNDED_CURVE ( )  B_SPLINE_CURVE ( 2, ( #3269, #42478, #62116, #18035, #48872, #25073, #38907, #5140, #19289 ),
 .UNSPECIFIED., .F., .F. ) 
 B_SPLINE_CURVE_WITH_KNOTS ( ( 3, 2, 2, 2, 3 ),
 ( 0.5916666666666671182, 0.5958333333333335480, 0.6000000000000000888, 0.6041666666666665186, 0.6083333333333329485 ),
 .UNSPECIFIED. ) 
 CURVE ( )  GEOMETRIC_REPRESENTATION_ITEM ( )  RATIONAL_B_SPLINE_CURVE ( ( 0.9999999999999918954, 0.9238795325112948431, 1.000000000000000000, 0.9238795325112867385, 1.000000000000000000, 0.9238795325112867385, 1.000000000000000000, 0.9238795325112928447, 0.9999999999999938938 ) ) 
 REPRESENTATION_ITEM ( '' )  );
#30011=ADVANCED_FACE ( 'NONE', ( #34511 ), #137, .T. ) ;
#30014=CARTESIAN_POINT ( 'NONE',  ( -1.846868145590737420, -165.0000000013655779, 4.458734124999997661 ) ) ;
#30018=CARTESIAN_POINT ( 'NONE',  ( -4.458734125000001214, -143.8750000013656063, 1.846868145590734089 ) ) ;
#30019=VERTEX_POINT ( 'NONE', #6227 ) ;
#30020=CARTESIAN_POINT ( 'NONE',  ( 5.000000000000000888, -90.45833333060214443, 2.886751345948126879 ) ) ;
#30022=CARTESIAN_POINT ( 'NONE',  ( 4.458734125000000326, -61.14583333196773651, 2.574251347313718519 ) ) ;
#30025=CARTESIAN_POINT ( 'NONE',  ( -2.499999999999996447, 13.16666666666666607, 4.330127018922195425 ) ) ;
#30026=CARTESIAN_POINT ( 'NONE',  ( 4.458734125000000326, -49.89583333196772941, 2.574251347313718519 ) ) ;
#30027=CARTESIAN_POINT ( 'NONE',  ( 4.458734125000001214, -7.895833331967735624, 2.574251347313718519 ) ) ;
#30028=CARTESIAN_POINT ( 'NONE',  ( 5.000000000000000000, -166.1250000027312126, 0.000000000000000000 ) ) ;
#30033=CARTESIAN_POINT ( 'NONE',  ( 1.975475456537005874E-15, -58.75000000000000000, 5.000000000000000000 ) ) ;
#30035=CARTESIAN_POINT ( 'NONE',  ( -6.972266317189433020E-16, -32.12499999726880873, -5.000000000000000000 ) ) ;
#30036=CARTESIAN_POINT ( 'NONE',  ( -4.458734124999999437, -52.31249999863440792, 0.000000000000000000 ) ) ;
#30037=CARTESIAN_POINT ( 'NONE',  ( 1.846868145590735200, -154.5000000013656347, -4.458734125000000326 ) ) ;
#30038=CARTESIAN_POINT ( 'NONE',  ( 1.060575238724906964E-15, -55.62499999726880873, 5.773502691896257311 ) ) ;
#30040=DIRECTION ( 'NONE',  ( -0.000000000000000000, 1.000000000000000000, -0.000000000000000000 ) ) ;
#30041=CARTESIAN_POINT ( 'NONE',  ( 2.229367062500001939, 2.770833334698928674, 3.861377020970579999 ) ) ;
#30045=CARTESIAN_POINT ( 'NONE',  ( 2.730187237215162345E-16, -158.1875000013655779, -4.458734124999999437 ) ) ;
#30047=CARTESIAN_POINT ( 'NONE',  ( -6.972266317189433020E-16, -83.24999999999998579, -5.000000000000000000 ) ) ;
#30049=CARTESIAN_POINT ( 'NONE',  ( 2.071067811865264563, -152.8125000000000000, -5.000000000000211386 ) ) ;
#30050=CARTESIAN_POINT ( 'NONE',  ( -4.458734124999998549, -44.47916666530106511, 2.574251347313722516 ) ) ;
#30052=CARTESIAN_POINT ( 'NONE',  ( 2.499999999999998668, 9.791666669397850242, -4.330127018922193649 ) ) ;
#30055=CARTESIAN_POINT ( 'NONE',  ( 4.458734125000001214, -89.14583333196775072, 2.574251347313718519 ) ) ;
#30058=CARTESIAN_POINT ( 'NONE',  ( 1.975475456537005874E-15, -35.62499999726880162, 5.000000000000000000 ) ) ;
#30059=( BOUNDED_CURVE ( )  B_SPLINE_CURVE ( 2, ( #794, #55772, #35837, #20401, #50623, #44831, #45155, #30684, #31308 ),
 .UNSPECIFIED., .F., .F. ) 
 B_SPLINE_CURVE_WITH_KNOTS ( ( 3, 2, 2, 2, 3 ),
 ( 0.9416666666666665408, 0.9458333333333331927, 0.9499999999999997335, 0.9541666666666664964, 0.9583333333333331483 ),
 .UNSPECIFIED. ) 
 CURVE ( )  GEOMETRIC_REPRESENTATION_ITEM ( )  RATIONAL_B_SPLINE_CURVE ( ( 1.000000000000001998, 0.9238795325112847401, 1.000000000000000000, 0.9238795325112867385, 1.000000000000000000, 0.9238795325112867385, 1.000000000000000000, 0.9238795325112908463, 0.9999999999999958922 ) ) 
 REPRESENTATION_ITEM ( '' )  );
#30060=CARTESIAN_POINT ( 'NONE',  ( -1.339745962155608039, 23.79465819873852084, -5.000000000000004441 ) ) ;
#30063=CYLINDRICAL_SURFACE ( 'NONE', #24684, 5.000000000000000000 ) ;
#30066=CYLINDRICAL_SURFACE ( 'NONE', #59187, 5.000000000000000000 ) ;
#30069=CARTESIAN_POINT ( 'NONE',  ( -1.339745962155589165, 10.91965820146970323, -5.000000000000014211 ) ) ;
#30071=ORIENTED_EDGE ( 'NONE', *, *, #16667, .F. ) ;
#30073=CARTESIAN_POINT ( 'NONE',  ( 3.061616997868383141E-16, -159.8750000027311842, -5.000000000000000000 ) ) ;
#30074=ORIENTED_EDGE ( 'NONE', *, *, #62117, .T. ) ;
#30084=CARTESIAN_POINT ( 'NONE',  ( -5.000000000000000888, -141.5625000027312126, 2.071067811865474617 ) ) ;
#30085=CARTESIAN_POINT ( 'NONE',  ( 2.229367062499998831, -21.64583333196774007, -3.861377020970580887 ) ) ;
#30087=CARTESIAN_POINT ( 'NONE',  ( 2.071067811865476394, -154.1874999999999716, 5.000000000000000000 ) ) ;
#30089=CARTESIAN_POINT ( 'NONE',  ( 3.152801135295367541, -156.3125000013656063, -3.152801135295367541 ) ) ;
#30090=ORIENTED_EDGE ( 'NONE', *, *, #17029, .T. ) ;
#30091=CARTESIAN_POINT ( 'NONE',  ( 4.458734125000000326, -46.14583333196773651, 2.574251347313718519 ) ) ;
#30092=CARTESIAN_POINT ( 'NONE',  ( 2.500000000000002220, -44.54166666393547303, 4.330127018922192761 ) ) ;
#30094=CARTESIAN_POINT ( 'NONE',  ( 4.458734124999998549, -88.72916666530106511, -2.574251347313721627 ) ) ;
#30096=CARTESIAN_POINT ( 'NONE',  ( 2.229367062499998831, 10.35416666803225993, -3.861377020970580887 ) ) ;
#30098=DIRECTION ( 'NONE',  ( 0.000000000000000000, 0.000000000000000000, 1.000000000000000000 ) ) ;
#30100=CARTESIAN_POINT ( 'NONE',  ( -4.458734124999999437, 21.35416666803225993, -2.574251347313719407 ) ) ;
#30102=CARTESIAN_POINT ( 'NONE',  ( 1.060575238724906964E-15, 6.375000002731185056, 5.773502691896257311 ) ) ;
#30104=CARTESIAN_POINT ( 'NONE',  ( 1.975475456537005874E-15, -33.75000000000000000, 5.000000000000000000 ) ) ;
#30105=ORIENTED_EDGE ( 'NONE', *, *, #36244, .F. ) ;
#30106=( BOUNDED_CURVE ( )  B_SPLINE_CURVE ( 2, ( #16251, #3601, #23208, #18384, #38003, #57636, #35871, #13564, #1473 ),
 .UNSPECIFIED., .F., .F. ) 
 B_SPLINE_CURVE_WITH_KNOTS ( ( 3, 2, 2, 2, 3 ),
 ( 0.9770833333333333037, 0.9777777777777777457, 0.9791666666666666297, 0.9805555555555555136, 0.9812499999999999556 ),
 .UNSPECIFIED. ) 
 CURVE ( )  GEOMETRIC_REPRESENTATION_ITEM ( )  RATIONAL_B_SPLINE_CURVE ( ( 0.9330127018922194093, 0.9330127018922194093, 1.000000000000000000, 0.8660254037844387076, 1.000000000000000000, 0.8660254037844387076, 1.000000000000000000, 0.9330127018922194093, 0.9330127018922194093 ) ) 
 REPRESENTATION_ITEM ( '' )  );
#30108=CARTESIAN_POINT ( 'NONE',  ( 9.457646018065525792E-16, -39.06249999863440081, 5.148502694627439702 ) ) ;
#30109=EDGE_CURVE ( 'NONE', #53004, #35151, #26263, .T. ) ;
#30110=CARTESIAN_POINT ( 'NONE',  ( -4.999999999999999112, -38.79166666393548013, 2.886751345948131764 ) ) ;
#30112=CARTESIAN_POINT ( 'NONE',  ( -4.458734124999999437, -10.39583333196773829, -2.574251347313719407 ) ) ;
#30113=CARTESIAN_POINT ( 'NONE',  ( 2.229367062500001939, -18.22916666530106866, 3.861377020970579999 ) ) ;
#30115=CARTESIAN_POINT ( 'NONE',  ( 2.500000000000002220, -84.66666666666667140, 4.330127018922192761 ) ) ;
#30116=CARTESIAN_POINT ( 'NONE',  ( -8.190561711645485556E-16, -168.6875000013656063, 4.458734124999999437 ) ) ;
#30118=CARTESIAN_POINT ( 'NONE',  ( 5.000000000000000888, -88.45833333060214443, 2.886751345948126879 ) ) ;
#30119=CARTESIAN_POINT ( 'NONE',  ( -4.999999999999998224, -48.79166666393547303, 2.886751345948131764 ) ) ;
#30122=CARTESIAN_POINT ( 'NONE',  ( -4.458734124999999437, -27.56249999863440081, 0.000000000000000000 ) ) ;
#30123=CARTESIAN_POINT ( 'NONE',  ( 1.339745962155565406, -5.580341798530294106, 5.000000000000028422 ) ) ;
#30124=ORIENTED_EDGE ( 'NONE', *, *, #13315, .T. ) ;
#30126=CARTESIAN_POINT ( 'NONE',  ( -4.458734125000000326, -164.2500000013656063, -1.846868145590735644 ) ) ;
#30128=CARTESIAN_POINT ( 'NONE',  ( -9.184850993605147944E-16, -156.2500000000000000, 5.000000000000000000 ) ) ;
#30129=VERTEX_POINT ( 'NONE', #44811 ) ;
#30131=CARTESIAN_POINT ( 'NONE',  ( 4.458734125000001214, -75.14583333196775072, 2.574251347313718519 ) ) ;
#30134=CARTESIAN_POINT ( 'NONE',  ( -3.152801135295367096, -146.3125000013655779, -3.152801135295367541 ) ) ;
#30140=CARTESIAN_POINT ( 'NONE',  ( -4.458734125000000326, -142.2500000013656063, -1.846868145590735644 ) ) ;
#30143=DIRECTION ( 'NONE',  ( 0.000000000000000000, 0.000000000000000000, 1.000000000000000000 ) ) ;
#30145=CARTESIAN_POINT ( 'NONE',  ( -2.229367062499996610, -73.39583333196773651, 3.861377020970582219 ) ) ;
#30146=CARTESIAN_POINT ( 'NONE',  ( -5.000000000000000888, -144.6875000027312126, -2.071067811865475949 ) ) ;
#30151=LINE ( 'NONE', #49780, #28464 ) ;
#30157=CARTESIAN_POINT ( 'NONE',  ( -4.458734124999999437, 20.35416666803225993, -2.574251347313719407 ) ) ;
#30158=DIRECTION ( 'NONE',  ( -0.000000000000000000, 1.000000000000000000, -0.000000000000000000 ) ) ;
#30164=CARTESIAN_POINT ( 'NONE',  ( -2.229367062499996610, -6.145833331967740953, 3.861377020970582219 ) ) ;
#30165=ORIENTED_EDGE ( 'NONE', *, *, #61394, .T. ) ;
#30166=CARTESIAN_POINT ( 'NONE',  ( 2.229367062499998831, -29.89583333196773296, -3.861377020970580887 ) ) ;
#30170=CARTESIAN_POINT ( 'NONE',  ( -2.229367062500000163, 23.52083333469892779, -3.861377020970580443 ) ) ;
#30171=CARTESIAN_POINT ( 'NONE',  ( 5.000000000000000888, 26.54166666939784847, 2.886751345948126879 ) ) ;
#30173=CARTESIAN_POINT ( 'NONE',  ( -4.458734124999999437, -80.56249999863440792, 0.000000000000000000 ) ) ;
#30176=CARTESIAN_POINT ( 'NONE',  ( -5.000000000000000000, 22.04166666939785202, -2.886751345948128211 ) ) ;
#30177=ORIENTED_EDGE ( 'NONE', *, *, #19513, .T. ) ;
#30180=CARTESIAN_POINT ( 'NONE',  ( -2.499999999999996447, -15.83333333333333037, 4.330127018922195425 ) ) ;
#30181=CARTESIAN_POINT ( 'NONE',  ( 2.229367062500001939, -23.97916666530107577, 3.861377020970579999 ) ) ;
#30182=EDGE_CURVE ( 'NONE', #21511, #18022, #773, .T. ) ;
#30183=CARTESIAN_POINT ( 'NONE',  ( 9.457646018065525792E-16, -83.06249999863439371, 5.148502694627439702 ) ) ;
#30184=( BOUNDED_CURVE ( )  B_SPLINE_CURVE ( 2, ( #57370, #8781, #47698, #52847, #37738, #47391, #62822, #28392, #13291 ),
 .UNSPECIFIED., .F., .F. ) 
 B_SPLINE_CURVE_WITH_KNOTS ( ( 3, 2, 2, 2, 3 ),
 ( 0.2604166666666666852, 0.2611111111111111271, 0.2625000000000000111, 0.2638888888888888951, 0.2645833333333333370 ),
 .UNSPECIFIED. ) 
 CURVE ( )  GEOMETRIC_REPRESENTATION_ITEM ( )  RATIONAL_B_SPLINE_CURVE ( ( 0.9330127018922194093, 0.9330127018922194093, 1.000000000000000000, 0.8660254037844387076, 1.000000000000000000, 0.8660254037844387076, 1.000000000000000000, 0.9330127018922194093, 0.9330127018922194093 ) ) 
 REPRESENTATION_ITEM ( '' )  );
#30185=CARTESIAN_POINT ( 'NONE',  ( -4.999999999999999112, -23.79166666393548013, 2.886751345948131764 ) ) ;
#30186=CARTESIAN_POINT ( 'NONE',  ( 4.458734124999998549, -49.72916666530106511, -2.574251347313721627 ) ) ;
#30187=ORIENTED_EDGE ( 'NONE', *, *, #11365, .F. ) ;
#30189=CYLINDRICAL_SURFACE ( 'NONE', #35409, 5.000000000000000000 ) ;
#30190=CARTESIAN_POINT ( 'NONE',  ( 4.458734125000001214, 2.854166668032259491, 2.574251347313718519 ) ) ;
#30193=CARTESIAN_POINT ( 'NONE',  ( -3.535250795749689387E-16, -64.25000000000000000, -5.773502691896257311 ) ) ;
#30194=CARTESIAN_POINT ( 'NONE',  ( -4.458734125000001214, -153.1250000013656063, 1.846868145590734089 ) ) ;
#30196=CARTESIAN_POINT ( 'NONE',  ( -1.339745962155610925, -80.66965819600734733, 5.000000000000000000 ) ) ;
#30197=CARTESIAN_POINT ( 'NONE',  ( 5.000000000000000888, -157.9375000000000000, -2.071067811865475505 ) ) ;
#30200=CARTESIAN_POINT ( 'NONE',  ( -2.229367062499996610, -11.39583333196773829, 3.861377020970582219 ) ) ;
#30201=CARTESIAN_POINT ( 'NONE',  ( -4.458734124999998549, -47.47916666530106511, 2.574251347313722516 ) ) ;
#30202=VECTOR ( 'NONE', #26274, 1000.000000000000000 ) ;
#30205=CARTESIAN_POINT ( 'NONE',  ( -4.999999999999998224, -7.791666663935482795, 2.886751345948131764 ) ) ;
#30206=CARTESIAN_POINT ( 'NONE',  ( 3.152801135295367541, -143.3125000013655779, -3.152801135295367541 ) ) ;
#30212=CARTESIAN_POINT ( 'NONE',  ( -1.339745962155613812, -6.080341798530292330, -5.000000000000000000 ) ) ;
#30220=CARTESIAN_POINT ( 'NONE',  ( -2.071067811865644259, -154.8125000027311842, -4.999999999999831246 ) ) ;
#30221=CARTESIAN_POINT ( 'NONE',  ( -4.458734124999998549, -6.229166665301072214, 2.574251347313722516 ) ) ;
#30223=CARTESIAN_POINT ( 'NONE',  ( -3.152801135295367985, -148.8125000013655779, 3.152801135295367096 ) ) ;
#30225=ORIENTED_EDGE ( 'NONE', *, *, #63327, .T. ) ;
#30226=CARTESIAN_POINT ( 'NONE',  ( -1.339745962155613812, -63.08034179853028434, -5.000000000000000000 ) ) ;
#30232=ADVANCED_FACE ( 'NONE', ( #58231 ), #34093, .T. ) ;
#30236=DIRECTION ( 'NONE',  ( -0.000000000000000000, 1.000000000000000000, -0.000000000000000000 ) ) ;
#30238=CARTESIAN_POINT ( 'NONE',  ( -3.152548672688508926E-16, 11.43750000136559564, -5.148502694627439702 ) ) ;
#30240=VERTEX_POINT ( 'NONE', #38303 ) ;
#30241=CARTESIAN_POINT ( 'NONE',  ( 4.458734124999998549, -12.97916666530107399, -2.574251347313721627 ) ) ;
#30243=CARTESIAN_POINT ( 'NONE',  ( 3.152801135295367541, -164.3125000013656063, -3.152801135295367541 ) ) ;
#30244=CARTESIAN_POINT ( 'NONE',  ( 5.000000000000000000, -88.41666666666665719, -2.886751345948130876 ) ) ;
#30253=CARTESIAN_POINT ( 'NONE',  ( 1.846868145590736310, -154.8750000013655779, 4.458734124999997661 ) ) ;
#30257=ORIENTED_EDGE ( 'NONE', *, *, #46409, .T. ) ;
#30261=CARTESIAN_POINT ( 'NONE',  ( 0.000000000000000000, -170.0000000000000000, 0.000000000000000000 ) ) ;
#30262=CARTESIAN_POINT ( 'NONE',  ( -2.500000000000000444, -4.166666666666666075, -4.330127018922193649 ) ) ;
#30263=ADVANCED_FACE ( 'NONE', ( #9028 ), #28949, .T. ) ;
#30264=CARTESIAN_POINT ( 'NONE',  ( 4.458734124999998549, -64.72916666530106511, -2.574251347313721627 ) ) ;
#30265=DIRECTION ( 'NONE',  ( 0.000000000000000000, 0.000000000000000000, 1.000000000000000000 ) ) ;
#30267=ADVANCED_FACE ( 'NONE', ( #33787 ), #8714, .T. ) ;
#30268=CARTESIAN_POINT ( 'NONE',  ( -3.535250795749689387E-16, -5.124999997268809615, -5.773502691896257311 ) ) ;
#30269=CARTESIAN_POINT ( 'NONE',  ( -4.458734124999999437, -33.39583333196772941, -2.574251347313719407 ) ) ;
#30270=ORIENTED_EDGE ( 'NONE', *, *, #45964, .T. ) ;
#30275=CARTESIAN_POINT ( 'NONE',  ( -2.499999999999996447, -50.83333333333332860, 4.330127018922195425 ) ) ;
#30276=FACE_OUTER_BOUND ( 'NONE', #4220, .T. ) ;
#30278=CARTESIAN_POINT ( 'NONE',  ( 1.975475456537005874E-15, -41.62499999726880162, 5.000000000000000000 ) ) ;
#30279=CARTESIAN_POINT ( 'NONE',  ( 2.229367062499998831, -77.64583333196773651, -3.861377020970580887 ) ) ;
#30280=CARTESIAN_POINT ( 'NONE',  ( -1.846868145590734756, -143.3750000013656063, -4.458734125000000326 ) ) ;
#30281=CARTESIAN_POINT ( 'NONE',  ( -2.229367062500000163, -80.47916666530106511, -3.861377020970580443 ) ) ;
#30284=CARTESIAN_POINT ( 'NONE',  ( 9.457646018065525792E-16, -28.31249999863440081, 5.148502694627439702 ) ) ;
#30287=ORIENTED_EDGE ( 'NONE', *, *, #38479, .F. ) ;
#30292=CARTESIAN_POINT ( 'NONE',  ( 6.123233995736766282E-16, -170.0000000000000000, -5.000000000000000000 ) ) ;
#30293=( BOUNDED_CURVE ( )  B_SPLINE_CURVE ( 2, ( #3469, #23082, #42371, #17928, #18250, #27273, #32729, #13425, #47823 ),
 .UNSPECIFIED., .F., .F. ) 
 B_SPLINE_CURVE_WITH_KNOTS ( ( 3, 2, 2, 2, 3 ),
 ( 0.7104166666666666963, 0.7111111111111111382, 0.7125000000000000222, 0.7138888888888889062, 0.7145833333333333481 ),
 .UNSPECIFIED. ) 
 CURVE ( )  GEOMETRIC_REPRESENTATION_ITEM ( )  RATIONAL_B_SPLINE_CURVE ( ( 0.9330127018922194093, 0.9330127018922194093, 1.000000000000000000, 0.8660254037844387076, 1.000000000000000000, 0.8660254037844387076, 1.000000000000000000, 0.9330127018922194093, 0.9330127018922194093 ) ) 
 REPRESENTATION_ITEM ( '' )  );
#30295=CARTESIAN_POINT ( 'NONE',  ( 9.457646018065525792E-16, -63.31249999863440081, 5.148502694627439702 ) ) ;
#30297=ORIENTED_EDGE ( 'NONE', *, *, #37065, .T. ) ;
#30300=CARTESIAN_POINT ( 'NONE',  ( -4.458734124999999437, 15.60416666803225993, -2.574251347313719407 ) ) ;
#30303=CARTESIAN_POINT ( 'NONE',  ( -3.152801135295367096, -161.0625000013656063, -3.152801135295367541 ) ) ;
#30305=VERTEX_POINT ( 'NONE', #53402 ) ;
#30309=LINE ( 'NONE', #59927, #17049 ) ;
#30310=CYLINDRICAL_SURFACE ( 'NONE', #9999, 5.000000000000000000 ) ;
#30313=CARTESIAN_POINT ( 'NONE',  ( 2.500000000000002220, 12.45833333606451809, 4.330127018922192761 ) ) ;
#30316=CARTESIAN_POINT ( 'NONE',  ( 6.123233995736766282E-16, -170.0000000000000000, -5.000000000000000000 ) ) ;
#30319=CARTESIAN_POINT ( 'NONE',  ( 4.458734124999998549, 2.020833334698927786, -2.574251347313721627 ) ) ;
#30320=CARTESIAN_POINT ( 'NONE',  ( -5.000000000000000888, -161.5625000027312126, 2.071067811865474617 ) ) ;
#30322=CARTESIAN_POINT ( 'NONE',  ( 3.061616997868383141E-16, -144.8750000027312126, -5.000000000000000000 ) ) ;
#30323=CARTESIAN_POINT ( 'NONE',  ( 1.975475456537005874E-15, 17.37500000273118417, 5.000000000000000000 ) ) ;
#30330=CARTESIAN_POINT ( 'NONE',  ( -8.190561711645485556E-16, -163.9375000013655779, 4.458734124999999437 ) ) ;
#30332=CARTESIAN_POINT ( 'NONE',  ( -9.184850993605147944E-16, -159.3750000027311842, 5.000000000000000000 ) ) ;
#30334=CARTESIAN_POINT ( 'NONE',  ( -1.846868145590734756, -143.1250000013656063, -4.458734125000000326 ) ) ;
#30335=ORIENTED_EDGE ( 'NONE', *, *, #33623, .F. ) ;
#30336=CARTESIAN_POINT ( 'NONE',  ( 4.458734124999999437, 20.93750000136559208, -5.460374474430324690E-16 ) ) ;
#30337=ORIENTED_EDGE ( 'NONE', *, *, #53182, .T. ) ;
#30338=CARTESIAN_POINT ( 'NONE',  ( 4.458734124999999437, -62.06249999863440792, -5.460374474430324690E-16 ) ) ;
#30340=DIRECTION ( 'NONE',  ( -0.000000000000000000, 1.000000000000000000, -0.000000000000000000 ) ) ;
#30341=CARTESIAN_POINT ( 'NONE',  ( -3.535250795749689387E-16, 13.75000000000000000, -5.773502691896257311 ) ) ;
#30342=CARTESIAN_POINT ( 'NONE',  ( -3.152548672688508926E-16, -51.56249999863440792, -5.148502694627439702 ) ) ;
#30344=CARTESIAN_POINT ( 'NONE',  ( -4.458734124999999437, -10.31249999863440792, 0.000000000000000000 ) ) ;
#30345=CARTESIAN_POINT ( 'NONE',  ( -2.500000000000000444, 3.958333336064518093, -4.330127018922193649 ) ) ;
#30347=CARTESIAN_POINT ( 'NONE',  ( -1.339745962155613812, 13.79465819873852084, -5.000000000000000000 ) ) ;
#30350=DIRECTION ( 'NONE',  ( 0.000000000000000000, 0.000000000000000000, 1.000000000000000000 ) ) ;
#30351=CARTESIAN_POINT ( 'NONE',  ( 1.339745962155612702, 21.83034180399266333, -5.000000000000000000 ) ) ;
#30355=CARTESIAN_POINT ( 'NONE',  ( -4.458734124999999437, -57.39583333196773651, -2.574251347313719407 ) ) ;
#30356=CARTESIAN_POINT ( 'NONE',  ( -4.458734125000000326, -155.2500000013656063, -1.846868145590735644 ) ) ;
#30359=CARTESIAN_POINT ( 'NONE',  ( 5.000000000000000000, -53.29166666393547303, -2.886751345948129988 ) ) ;
#30362=CARTESIAN_POINT ( 'NONE',  ( 4.458734124999999437, 1.937500001365593416, -5.460374474430324690E-16 ) ) ;
#30364=CARTESIAN_POINT ( 'NONE',  ( -5.000000000000000888, -157.5625000027312410, 2.071067811865474617 ) ) ;
#30366=CARTESIAN_POINT ( 'NONE',  ( -1.846868145590737420, -154.7500000013656063, 4.458734124999999437 ) ) ;
#30372=CARTESIAN_POINT ( 'NONE',  ( 2.229367062499998831, -44.89583333196774362, -3.861377020970580887 ) ) ;
#30377=CARTESIAN_POINT ( 'NONE',  ( 2.229367062499998831, 27.35416666803225993, -3.861377020970580887 ) ) ;
#30380=CARTESIAN_POINT ( 'NONE',  ( 2.499999999999998668, -61.20833333060214443, -4.330127018922193649 ) ) ;
#30385=( BOUNDED_CURVE ( )  B_SPLINE_CURVE ( 2, ( #54796, #24565, #45454, #54476, #29692, #44488, #15558, #59626, #5909 ),
 .UNSPECIFIED., .F., .F. ) 
 B_SPLINE_CURVE_WITH_KNOTS ( ( 3, 2, 2, 2, 3 ),
 ( 0.5229166666666666963, 0.5236111111111111382, 0.5250000000000000222, 0.5263888888888889062, 0.5270833333333333481 ),
 .UNSPECIFIED. ) 
 CURVE ( )  GEOMETRIC_REPRESENTATION_ITEM ( )  RATIONAL_B_SPLINE_CURVE ( ( 0.9330127018922194093, 0.9330127018922194093, 1.000000000000000000, 0.8660254037844387076, 1.000000000000000000, 0.8660254037844387076, 1.000000000000000000, 0.9330127018922194093, 0.9330127018922194093 ) ) 
 REPRESENTATION_ITEM ( '' )  );
#30386=DIRECTION ( 'NONE',  ( 0.000000000000000000, 0.000000000000000000, 1.000000000000000000 ) ) ;
#30387=CARTESIAN_POINT ( 'NONE',  ( -9.184850993605147944E-16, -157.2500000000000000, 5.000000000000000000 ) ) ;
#30390=CARTESIAN_POINT ( 'NONE',  ( -2.500000000000000444, 24.83333333333333215, -4.330127018922193649 ) ) ;
#30392=CARTESIAN_POINT ( 'NONE',  ( 4.458734125000001214, -90.14583333196773651, 2.574251347313718519 ) ) ;
#30393=CARTESIAN_POINT ( 'NONE',  ( 0.000000000000000000, -170.0000000000000000, 0.000000000000000000 ) ) ;
#30395=VERTEX_POINT ( 'NONE', #45026 ) ;
#30396=CARTESIAN_POINT ( 'NONE',  ( -6.972266317189433020E-16, -31.24999999999999645, -5.000000000000000000 ) ) ;
#30398=CARTESIAN_POINT ( 'NONE',  ( -5.000000000000000000, -156.6250000027311842, -6.123233995736766282E-16 ) ) ;
#30399=VERTEX_POINT ( 'NONE', #20597 ) ;
#30401=CARTESIAN_POINT ( 'NONE',  ( 2.499999999999998668, -49.20833333060213732, -4.330127018922193649 ) ) ;
#30403=CARTESIAN_POINT ( 'NONE',  ( -1.339745962155610925, -66.79465819873851729, 5.000000000000000000 ) ) ;
#30409=CARTESIAN_POINT ( 'NONE',  ( 2.500000000000002220, -48.54166666393547303, 4.330127018922192761 ) ) ;
#30410=CARTESIAN_POINT ( 'NONE',  ( 4.458734124999998549, -21.72916666530107221, -2.574251347313721627 ) ) ;
#30412=CARTESIAN_POINT ( 'NONE',  ( -3.535533905932737309, -149.6250000000000000, -3.535533905932738197 ) ) ;
#30414=CARTESIAN_POINT ( 'NONE',  ( -1.846868145590734756, -154.1250000013656063, -4.458734125000000326 ) ) ;
#30416=CARTESIAN_POINT ( 'NONE',  ( 9.457646018065525792E-16, -48.31249999863440792, 5.148502694627439702 ) ) ;
#30417=CARTESIAN_POINT ( 'NONE',  ( -2.500000000000000444, 25.83333333333333215, -4.330127018922193649 ) ) ;
#30419=CARTESIAN_POINT ( 'NONE',  ( -4.458734124999999437, -88.39583333196773651, -2.574251347313719407 ) ) ;
#30420=CARTESIAN_POINT ( 'NONE',  ( -4.458734124999998549, 2.770833334698928674, 2.574251347313722516 ) ) ;
#30422=CARTESIAN_POINT ( 'NONE',  ( 2.500000000000002220, 13.33333333333333215, 4.330127018922192761 ) ) ;
#30424=CARTESIAN_POINT ( 'NONE',  ( 4.458734124999999437, 18.93750000136559564, -5.460374474430324690E-16 ) ) ;
#30426=CARTESIAN_POINT ( 'NONE',  ( -3.535250795749689387E-16, 5.875000002731185056, -5.773502691896257311 ) ) ;
#30427=ORIENTED_EDGE ( 'NONE', *, *, #44530, .T. ) ;
#30431=CARTESIAN_POINT ( 'NONE',  ( -2.229367062499996610, -38.14583333196773651, 3.861377020970582219 ) ) ;
#30433=CARTESIAN_POINT ( 'NONE',  ( 5.000000000000000888, -37.45833333060213732, 2.886751345948126879 ) ) ;
#30434=ORIENTED_EDGE ( 'NONE', *, *, #13335, .F. ) ;
#30435=CARTESIAN_POINT ( 'NONE',  ( -4.458734124999999437, -13.31249999863440259, 0.000000000000000000 ) ) ;
#30436=ORIENTED_EDGE ( 'NONE', *, *, #34637, .F. ) ;
#30438=CARTESIAN_POINT ( 'NONE',  ( -2.499999999999996447, -80.83333333333332860, 4.330127018922195425 ) ) ;
#30439=CARTESIAN_POINT ( 'NONE',  ( 1.846868145590736310, -168.6250000013655779, 4.458734124999999437 ) ) ;
#30441=CARTESIAN_POINT ( 'NONE',  ( -3.535250795749689387E-16, -85.12499999726881583, -5.773502691896257311 ) ) ;
#30442=CARTESIAN_POINT ( 'NONE',  ( 3.061616997868383141E-16, -144.8750000027312126, -5.000000000000000000 ) ) ;
#30445=CARTESIAN_POINT ( 'NONE',  ( 2.229367062500001939, -27.22916666530106866, 3.861377020970579999 ) ) ;
#30447=VERTEX_POINT ( 'NONE', #16400 ) ;
#30450=CARTESIAN_POINT ( 'NONE',  ( 4.458734125000000326, -162.6250000013655779, -1.846868145590734978 ) ) ;
#30452=CARTESIAN_POINT ( 'NONE',  ( -1.339745962155613812, -39.08034179853028434, -5.000000000000000000 ) ) ;
#30455=CARTESIAN_POINT ( 'NONE',  ( -4.458734124999999437, -75.64583333196775072, -2.574251347313719407 ) ) ;
#30458=CARTESIAN_POINT ( 'NONE',  ( -4.458734124999999437, -143.1875000013656063, -5.460374474430324690E-16 ) ) ;
#30459=CARTESIAN_POINT ( 'NONE',  ( -2.499999999999996447, 23.16666666666666430, 4.330127018922195425 ) ) ;
#30464=CARTESIAN_POINT ( 'NONE',  ( -9.184850993605147944E-16, -167.2500000000000000, 5.000000000000000000 ) ) ;
#30467=CARTESIAN_POINT ( 'NONE',  ( -2.500000000000000444, -53.16666666666666430, -4.330127018922193649 ) ) ;
#30469=( BOUNDED_CURVE ( )  B_SPLINE_CURVE ( 2, ( #17783, #23568, #43163, #37402, #62802, #57038, #22942, #22302, #8145 ),
 .UNSPECIFIED., .F., .F. ) 
 B_SPLINE_CURVE_WITH_KNOTS ( ( 3, 2, 2, 2, 3 ),
 ( 0.3145833333333333259, 0.3152777777777777679, 0.3166666666666666519, 0.3180555555555555358, 0.3187499999999999778 ),
 .UNSPECIFIED. ) 
 CURVE ( )  GEOMETRIC_REPRESENTATION_ITEM ( )  RATIONAL_B_SPLINE_CURVE ( ( 0.9330127018922194093, 0.9330127018922194093, 1.000000000000000000, 0.8660254037844387076, 1.000000000000000000, 0.8660254037844387076, 1.000000000000000000, 0.9330127018922194093, 0.9330127018922194093 ) ) 
 REPRESENTATION_ITEM ( '' )  );
#30470=CARTESIAN_POINT ( 'NONE',  ( -2.229367062500000163, -72.72916666530107932, -3.861377020970580443 ) ) ;
#30471=CARTESIAN_POINT ( 'NONE',  ( -2.071067811865520358, -139.4375000027311842, 4.999999999999957367 ) ) ;
#30474=ORIENTED_EDGE ( 'NONE', *, *, #16235, .F. ) ;
#30477=CARTESIAN_POINT ( 'NONE',  ( 1.975475456537005874E-15, -15.75000000000000000, 5.000000000000000000 ) ) ;
#30480=CARTESIAN_POINT ( 'NONE',  ( -1.049326080737009628E-13, -4.750000000000003553, 5.000000000000000000 ) ) ;
#30482=CARTESIAN_POINT ( 'NONE',  ( 9.457646018065525792E-16, 15.68750000136559564, 5.148502694627439702 ) ) ;
#30483=DIRECTION ( 'NONE',  ( 0.000000000000000000, 0.000000000000000000, 1.000000000000000000 ) ) ;
#30484=VECTOR ( 'NONE', #44640, 1000.000000000000000 ) ;
#30490=CARTESIAN_POINT ( 'NONE',  ( -4.999999999999998224, -50.79166666393547303, 2.886751345948131764 ) ) ;
#30491=CARTESIAN_POINT ( 'NONE',  ( 4.458734124999998549, -87.72916666530107932, -2.574251347313721627 ) ) ;
#30492=CARTESIAN_POINT ( 'NONE',  ( 2.229367062499998831, -3.645833331967739177, -3.861377020970580887 ) ) ;
#30493=ORIENTED_EDGE ( 'NONE', *, *, #61761, .F. ) ;
#30494=CARTESIAN_POINT ( 'NONE',  ( -4.458734124999997661, -29.47916666530106866, 2.574251347313722516 ) ) ;
#30495=( BOUNDED_CURVE ( )  B_SPLINE_CURVE ( 2, ( #60029, #59379, #15313, #34935, #54556, #10479, #30092, #5668, #25280 ),
 .UNSPECIFIED., .F., .F. ) 
 B_SPLINE_CURVE_WITH_KNOTS ( ( 3, 2, 2, 2, 3 ),
 ( 0.6104166666666667185, 0.6111111111111111605, 0.6125000000000000444, 0.6138888888888889284, 0.6145833333333333703 ),
 .UNSPECIFIED. ) 
 CURVE ( )  GEOMETRIC_REPRESENTATION_ITEM ( )  RATIONAL_B_SPLINE_CURVE ( ( 0.9330127018922194093, 0.9330127018922194093, 1.000000000000000000, 0.8660254037844387076, 1.000000000000000000, 0.8660254037844387076, 1.000000000000000000, 0.9330127018922194093, 0.9330127018922194093 ) ) 
 REPRESENTATION_ITEM ( '' )  );
#30499=CARTESIAN_POINT ( 'NONE',  ( -4.458734124999998549, 21.77083333469892779, 2.574251347313722516 ) ) ;
#30500=CARTESIAN_POINT ( 'NONE',  ( 6.123233995736766282E-16, -170.0000000000000000, -5.000000000000000000 ) ) ;
#30502=CARTESIAN_POINT ( 'NONE',  ( -3.152548672688508926E-16, -76.81249999863440792, -5.148502694627439702 ) ) ;
#30505=CARTESIAN_POINT ( 'NONE',  ( 2.499999999999998668, 21.79166666939785202, -4.330127018922193649 ) ) ;
#30508=FACE_OUTER_BOUND ( 'NONE', #26735, .T. ) ;
#30509=CARTESIAN_POINT ( 'NONE',  ( -3.535250795749689387E-16, -16.25000000000000000, -5.773502691896257311 ) ) ;
#30510=CARTESIAN_POINT ( 'NONE',  ( -4.458734124999999437, -23.31249999863440436, 0.000000000000000000 ) ) ;
#30511=CARTESIAN_POINT ( 'NONE',  ( 4.458734125000000326, -84.89583333196773651, 2.574251347313718519 ) ) ;
#30512=CARTESIAN_POINT ( 'NONE',  ( 5.000000000000000000, -24.29166666393548368, -2.886751345948129988 ) ) ;
#30513=CARTESIAN_POINT ( 'NONE',  ( 4.458734125000001214, -56.89583333196774362, 2.574251347313718519 ) ) ;
#30517=CARTESIAN_POINT ( 'NONE',  ( 2.229367062499998831, -5.895833331967740953, -3.861377020970580887 ) ) ;
#30518=ORIENTED_EDGE ( 'NONE', *, *, #16216, .T. ) ;
#30520=CARTESIAN_POINT ( 'NONE',  ( 5.000000000000000000, -64.41666666666667140, -2.886751345948129988 ) ) ;
#30521=CARTESIAN_POINT ( 'NONE',  ( 1.846868145590735200, -150.5000000013656347, -4.458734125000000326 ) ) ;
#30524=CARTESIAN_POINT ( 'NONE',  ( 3.535533905932736864, -159.1250000000000284, 3.535533905932738641 ) ) ;
#30527=CARTESIAN_POINT ( 'NONE',  ( 4.458734124999999437, -11.06249999863440792, -5.460374474430324690E-16 ) ) ;
#30528=VECTOR ( 'NONE', #60165, 1000.000000000000000 ) ;
#30529=CARTESIAN_POINT ( 'NONE',  ( -4.458734124999999437, -51.64583333196773651, -2.574251347313719407 ) ) ;
#30531=CARTESIAN_POINT ( 'NONE',  ( 3.152801135295367541, -145.3125000013655779, -3.152801135295367541 ) ) ;
#30535=ORIENTED_EDGE ( 'NONE', *, *, #27896, .T. ) ;
#30537=CARTESIAN_POINT ( 'NONE',  ( 9.457646018065525792E-16, 27.68750000136559208, 5.148502694627439702 ) ) ;
#30540=VERTEX_POINT ( 'NONE', #10926 ) ;
#30543=CARTESIAN_POINT ( 'NONE',  ( 5.000000000000000888, 11.54166666939785202, 2.886751345948126879 ) ) ;
#30544=CARTESIAN_POINT ( 'NONE',  ( -3.152548672688508926E-16, -5.562499998634402587, -5.148502694627439702 ) ) ;
#30546=CARTESIAN_POINT ( 'NONE',  ( 2.730187237215162345E-16, -147.1875000013656063, -4.458734124999999437 ) ) ;
#30548=ORIENTED_EDGE ( 'NONE', *, *, #39010, .F. ) ;
#30549=CARTESIAN_POINT ( 'NONE',  ( 3.061616997868383141E-16, -164.8750000027311842, -5.000000000000000000 ) ) ;
#30550=CARTESIAN_POINT ( 'NONE',  ( -9.184850993605147944E-16, -147.3750000027312126, 5.000000000000000000 ) ) ;
#30552=ADVANCED_FACE ( 'NONE', ( #31184 ), #39548, .T. ) ;
#30561=CARTESIAN_POINT ( 'NONE',  ( 4.458734124999999437, 10.18750000136559386, -5.460374474430324690E-16 ) ) ;
#30564=CARTESIAN_POINT ( 'NONE',  ( 2.229367062499998831, -15.89583333196773651, -3.861377020970580887 ) ) ;
#30565=VECTOR ( 'NONE', #340, 1000.000000000000000 ) ;
#30567=CARTESIAN_POINT ( 'NONE',  ( 2.730187237215162345E-16, -164.1875000013655779, -4.458734124999999437 ) ) ;
#30573=( BOUNDED_CURVE ( )  B_SPLINE_CURVE ( 2, ( #15168, #44108, #39599, #43791, #4560, #53454, #25134, #34792, #14523 ),
 .UNSPECIFIED., .F., .F. ) 
 B_SPLINE_CURVE_WITH_KNOTS ( ( 3, 2, 2, 2, 3 ),
 ( 0.4250000000000003220, 0.4291666666666669738, 0.4333333333333336812, 0.4375000000000003886, 0.4416666666666670404 ),
 .UNSPECIFIED. ) 
 CURVE ( )  GEOMETRIC_REPRESENTATION_ITEM ( )  RATIONAL_B_SPLINE_CURVE ( ( 0.9999999999999938938, 0.9238795325112928447, 1.000000000000000000, 0.9238795325112867385, 1.000000000000000000, 0.9238795325112867385, 1.000000000000000000, 0.9238795325112796331, 1.000000000000007105 ) ) 
 REPRESENTATION_ITEM ( '' )  );
#30574=CARTESIAN_POINT ( 'NONE',  ( 0.000000000000000000, -170.0000000000000000, 5.000000000000000000 ) ) ;
#30575=EDGE_CURVE ( 'NONE', #24664, #6571, #24196, .T. ) ;
#30577=CARTESIAN_POINT ( 'NONE',  ( -6.972266317189433020E-16, -69.24999999999998579, -5.000000000000000000 ) ) ;
#30580=CARTESIAN_POINT ( 'NONE',  ( 3.152801135295366208, -148.8125000013655779, 3.152801135295367985 ) ) ;
#30587=FACE_OUTER_BOUND ( 'NONE', #22616, .T. ) ;
#30588=CARTESIAN_POINT ( 'NONE',  ( -4.999999999999999112, -2.916666666666664742, 2.886751345948131764 ) ) ;
#30589=CARTESIAN_POINT ( 'NONE',  ( -3.152548672688508926E-16, -67.56249999863440792, -5.148502694627439702 ) ) ;
#30590=CYLINDRICAL_SURFACE ( 'NONE', #44143, 5.000000000000000000 ) ;
#30592=CARTESIAN_POINT ( 'NONE',  ( 5.000000000000000000, -9.291666663935483683, -2.886751345948129988 ) ) ;
#30593=CARTESIAN_POINT ( 'NONE',  ( 4.458734124999998549, -35.72916666530107221, -2.574251347313721627 ) ) ;
#30595=FACE_OUTER_BOUND ( 'NONE', #55725, .T. ) ;
#30596=CARTESIAN_POINT ( 'NONE',  ( 0.000000000000000000, -170.0000000000000000, 0.000000000000000000 ) ) ;
#30597=CARTESIAN_POINT ( 'NONE',  ( -2.229367062500000163, 14.27083333469892601, -3.861377020970580443 ) ) ;
#30598=ORIENTED_EDGE ( 'NONE', *, *, #50916, .F. ) ;
#30599=CARTESIAN_POINT ( 'NONE',  ( -6.972266317189433020E-16, -36.12499999726880162, -5.000000000000000000 ) ) ;
#30600=CARTESIAN_POINT ( 'NONE',  ( 5.000000000000000000, -52.50000000000000711, -6.123233995736766282E-16 ) ) ;
#30602=CARTESIAN_POINT ( 'NONE',  ( -2.500000000000000444, -42.04166666393548013, -4.330127018922193649 ) ) ;
#30603=CARTESIAN_POINT ( 'NONE',  ( -2.229367062499996610, -75.14583333196773651, 3.861377020970582219 ) ) ;
#30604=CARTESIAN_POINT ( 'NONE',  ( -1.846868145590734756, -140.3750000013656063, -4.458734125000000326 ) ) ;
#30605=CARTESIAN_POINT ( 'NONE',  ( 4.458734124999999437, -81.81249999863440792, -5.460374474430324690E-16 ) ) ;
#30607=CARTESIAN_POINT ( 'NONE',  ( -4.458734124999999437, -31.64583333196773651, -2.574251347313719407 ) ) ;
#30608=ORIENTED_EDGE ( 'NONE', *, *, #53434, .F. ) ;
#30611=VERTEX_POINT ( 'NONE', #30935 ) ;
#30615=CARTESIAN_POINT ( 'NONE',  ( 4.729367062499999719, -169.8437500006828031, 0.000000000000000000 ) ) ;
#30616=VECTOR ( 'NONE', #29038, 1000.000000000000000 ) ;
#30618=CARTESIAN_POINT ( 'NONE',  ( 2.229367062499998831, -62.89583333196774362, -3.861377020970580887 ) ) ;
#30619=AXIS2_PLACEMENT_3D ( 'NONE', #34616, #14053, #59396 ) ;
#30621=ORIENTED_EDGE ( 'NONE', *, *, #9223, .T. ) ;
#30623=DIRECTION ( 'NONE',  ( 0.000000000000000000, 0.000000000000000000, 1.000000000000000000 ) ) ;
#30624=CARTESIAN_POINT ( 'NONE',  ( -4.458734124999999437, 6.604166668032259047, -2.574251347313719407 ) ) ;
#30626=CARTESIAN_POINT ( 'NONE',  ( 1.975475456537005874E-15, -27.62499999726881228, 5.000000000000000000 ) ) ;
#30627=CARTESIAN_POINT ( 'NONE',  ( -4.458734124999999437, -163.0000000013655779, -1.846868145590735644 ) ) ;
#30628=CARTESIAN_POINT ( 'NONE',  ( -2.499999999999996447, 19.29166666939785202, 4.330127018922195425 ) ) ;
#30634=DIRECTION ( 'NONE',  ( -0.000000000000000000, 1.000000000000000000, -0.000000000000000000 ) ) ;
#30635=CARTESIAN_POINT ( 'NONE',  ( 1.975475456537005874E-15, -67.74999999999998579, 5.000000000000000000 ) ) ;
#30638=CARTESIAN_POINT ( 'NONE',  ( 1.975475456537005874E-15, -28.74999999999999645, 5.000000000000000000 ) ) ;
#30641=CARTESIAN_POINT ( 'NONE',  ( 4.458734125000000326, 27.10416666803225993, 2.574251347313718519 ) ) ;
#30644=CARTESIAN_POINT ( 'NONE',  ( 2.229367062500001939, 1.770833334698927786, 3.861377020970579999 ) ) ;
#30646=CYLINDRICAL_SURFACE ( 'NONE', #43186, 5.000000000000000000 ) ;
#30648=CARTESIAN_POINT ( 'NONE',  ( 2.071067811865476394, -145.3125000027312126, 5.000000000000000000 ) ) ;
#30649=CARTESIAN_POINT ( 'NONE',  ( 1.339745962155615144, -33.58034179853029144, 4.999999999999999112 ) ) ;
#30654=CARTESIAN_POINT ( 'NONE',  ( -6.972266317189433020E-16, -76.12499999726880162, -5.000000000000000000 ) ) ;
#30655=CARTESIAN_POINT ( 'NONE',  ( -6.972266317189433020E-16, 3.749999999999999556, -5.000000000000000000 ) ) ;
#30656=ADVANCED_FACE ( 'NONE', ( #17100 ), #11627, .F. ) ;
#30658=CARTESIAN_POINT ( 'NONE',  ( 4.458734124999999437, -162.6250000013656063, -1.846868145590734978 ) ) ;
#30659=CARTESIAN_POINT ( 'NONE',  ( 6.123233995736766282E-16, -170.0000000000000000, -5.000000000000000000 ) ) ;
#30662=CARTESIAN_POINT ( 'NONE',  ( 3.152801135295366208, -140.5625000013655779, 3.152801135295367985 ) ) ;
#30664=CARTESIAN_POINT ( 'NONE',  ( -4.458734124999998549, 20.52083333469892423, 2.574251347313722516 ) ) ;
#30665=ORIENTED_EDGE ( 'NONE', *, *, #25677, .F. ) ;
#30667=CARTESIAN_POINT ( 'NONE',  ( -4.458734124999999437, -59.64583333196775072, -2.574251347313719407 ) ) ;
#30670=CARTESIAN_POINT ( 'NONE',  ( -5.000000000000000000, -2.874999997268815832, 0.000000000000000000 ) ) ;
#30671=CARTESIAN_POINT ( 'NONE',  ( -4.999999999999999112, 15.08333333333333215, 2.886751345948131764 ) ) ;
#30673=CARTESIAN_POINT ( 'NONE',  ( -2.229367062499996610, -52.14583333196773651, 3.861377020970582219 ) ) ;
#30674=CARTESIAN_POINT ( 'NONE',  ( -4.458734124999998549, -9.229166665301068662, 2.574251347313722516 ) ) ;
#30676=DIRECTION ( 'NONE',  ( -0.000000000000000000, 1.000000000000000000, -0.000000000000000000 ) ) ;
#30679=CARTESIAN_POINT ( 'NONE',  ( 2.500000000000002220, -32.66666666666666430, 4.330127018922192761 ) ) ;
#30680=CARTESIAN_POINT ( 'NONE',  ( 5.000000000000000888, -66.45833333060213022, 2.886751345948126879 ) ) ;
#30684=CARTESIAN_POINT ( 'NONE',  ( -2.071067811865562991, -140.4375000027311842, 4.999999999999913847 ) ) ;
#30685=CARTESIAN_POINT ( 'NONE',  ( 4.458734124999998549, -58.72916666530106511, -2.574251347313721627 ) ) ;
#30686=CARTESIAN_POINT ( 'NONE',  ( 3.152801135295366208, -153.8125000013656063, 3.152801135295367985 ) ) ;
#30688=CARTESIAN_POINT ( 'NONE',  ( -2.229367062499996610, -66.14583333196773651, 3.861377020970582219 ) ) ;
#30689=CARTESIAN_POINT ( 'NONE',  ( -5.000000000000000000, -53.95833333060214443, -2.886751345948128211 ) ) ;
#30690=VERTEX_POINT ( 'NONE', #45737 ) ;
#30692=CARTESIAN_POINT ( 'NONE',  ( -2.229367062500000163, -0.7291666653010709931, -3.861377020970580443 ) ) ;
#30695=CARTESIAN_POINT ( 'NONE',  ( -4.458734125000000326, -158.0000000013655779, -1.846868145590735644 ) ) ;
#30697=DIRECTION ( 'NONE',  ( 0.000000000000000000, 0.000000000000000000, 1.000000000000000000 ) ) ;
#30699=CARTESIAN_POINT ( 'NONE',  ( -4.458734124999998549, -50.47916666530107221, 2.574251347313722516 ) ) ;
#30701=CARTESIAN_POINT ( 'NONE',  ( 5.275681513340003914E-14, 10.87500000273118239, -5.000000000000000000 ) ) ;
#30703=CARTESIAN_POINT ( 'NONE',  ( 2.229367062499998831, 22.35416666803225993, -3.861377020970580887 ) ) ;
#30705=LINE ( 'NONE', #11402, #41830 ) ;
#30706=AXIS2_PLACEMENT_3D ( 'NONE', #52665, #47214, #62650 ) ;
#30708=CARTESIAN_POINT ( 'NONE',  ( -1.339745962155613812, 0.7946581987385198387, -5.000000000000000000 ) ) ;
#30712=EDGE_CURVE ( 'NONE', #51645, #30540, #11310, .T. ) ;
#30713=CARTESIAN_POINT ( 'NONE',  ( 1.975475456537005874E-15, -26.74999999999999645, 5.000000000000000000 ) ) ;
#30717=CARTESIAN_POINT ( 'NONE',  ( 5.000000000000000000, -42.37499999726880873, -6.123233995736766282E-16 ) ) ;
#30718=CARTESIAN_POINT ( 'NONE',  ( -4.458734124999998549, -87.47916666530107932, 2.574251347313722516 ) ) ;
#30725=CARTESIAN_POINT ( 'NONE',  ( -2.071067811865478170, -158.4375000027312126, 5.000000000000000000 ) ) ;
#30726=ORIENTED_EDGE ( 'NONE', *, *, #10507, .T. ) ;
#30730=EDGE_CURVE ( 'NONE', #12628, #55786, #59527, .T. ) ;
#30734=EDGE_CURVE ( 'NONE', #48784, #52220, #61605, .T. ) ;
#30737=CARTESIAN_POINT ( 'NONE',  ( -4.458734124999999437, -19.39583333196774007, -2.574251347313719407 ) ) ;
#30738=CARTESIAN_POINT ( 'NONE',  ( 1.339745962155615144, -75.70534180126148271, 4.999999999999999112 ) ) ;
#30739=CARTESIAN_POINT ( 'NONE',  ( -5.000000000000000000, -152.5000000000000284, -6.123233995736766282E-16 ) ) ;
#30741=EDGE_CURVE ( 'NONE', #10944, #35151, #2631, .T. ) ;
#30742=CARTESIAN_POINT ( 'NONE',  ( 1.846868145590736310, -150.6250000013655779, 4.458734124999999437 ) ) ;
#30744=CARTESIAN_POINT ( 'NONE',  ( 2.229367062499998831, -47.89583333196774362, -3.861377020970580887 ) ) ;
#30748=CARTESIAN_POINT ( 'NONE',  ( 5.000000000000000888, 29.41666666666666785, 2.886751345948126879 ) ) ;
#30749=CARTESIAN_POINT ( 'NONE',  ( -2.229367062499996610, 3.854166668032260823, 3.861377020970582219 ) ) ;
#30751=CARTESIAN_POINT ( 'NONE',  ( 1.975475456537005874E-15, -41.62499999726880162, 5.000000000000000000 ) ) ;
#30752=CARTESIAN_POINT ( 'NONE',  ( -6.972266317189433020E-16, -17.25000000000000000, -5.000000000000000000 ) ) ;
#30753=CARTESIAN_POINT ( 'NONE',  ( 9.457646018065525792E-16, 13.68750000136559208, 5.148502694627439702 ) ) ;
#30755=CARTESIAN_POINT ( 'NONE',  ( -5.000000000000000000, 9.041666669397852019, -2.886751345948128211 ) ) ;
#30756=VERTEX_POINT ( 'NONE', #62441 ) ;
#30757=CARTESIAN_POINT ( 'NONE',  ( -6.972266317189433020E-16, 7.750000000000000000, -5.000000000000000000 ) ) ;
#30758=ORIENTED_EDGE ( 'NONE', *, *, #62201, .F. ) ;
#30760=CARTESIAN_POINT ( 'NONE',  ( -3.152548672688508926E-16, -42.56249999863440792, -5.148502694627439702 ) ) ;
#30761=CARTESIAN_POINT ( 'NONE',  ( -1.846868145590737420, -169.0000000013655779, 4.458734124999999437 ) ) ;
#30762=CARTESIAN_POINT ( 'NONE',  ( -3.535250795749689387E-16, -39.12499999726880162, -5.773502691896257311 ) ) ;
#30764=CARTESIAN_POINT ( 'NONE',  ( 2.229367062499998831, -20.64583333196774007, -3.861377020970580887 ) ) ;
#30765=EDGE_LOOP ( 'NONE', ( #9712, #62661, #21384, #6823 ) ) ;
#30766=CARTESIAN_POINT ( 'NONE',  ( 5.000000000000000000, -85.41666666666665719, -2.886751345948129988 ) ) ;
#30767=CARTESIAN_POINT ( 'NONE',  ( -5.000000000000000000, 1.125000002731184390, 0.000000000000000000 ) ) ;
#30768=CARTESIAN_POINT ( 'NONE',  ( -2.499999999999996447, -86.70833333060214443, 4.330127018922195425 ) ) ;
#30772=CARTESIAN_POINT ( 'NONE',  ( -4.458734124999999437, -32.64583333196774362, -2.574251347313719407 ) ) ;
#30779=CARTESIAN_POINT ( 'NONE',  ( 1.339745962155615144, -23.70534180126148271, 4.999999999999999112 ) ) ;
#30781=CARTESIAN_POINT ( 'NONE',  ( -9.184850993605147944E-16, -161.2500000000000000, 5.000000000000000000 ) ) ;
#30783=CARTESIAN_POINT ( 'NONE',  ( 2.229367062500001939, -77.22916666530106511, 3.861377020970579999 ) ) ;
#30786=CARTESIAN_POINT ( 'NONE',  ( -4.458734124999999437, -141.1875000013656063, -5.460374474430324690E-16 ) ) ;
#30787=LINE ( 'NONE', #2483, #49726 ) ;
#30789=CARTESIAN_POINT ( 'NONE',  ( -4.458734124999999437, -45.31249999863440081, 0.000000000000000000 ) ) ;
#30793=CARTESIAN_POINT ( 'NONE',  ( -4.458734125000000326, -140.2500000013656063, -1.846868145590735644 ) ) ;
#30796=CARTESIAN_POINT ( 'NONE',  ( -5.000000000000000000, -39.87499999726880162, 0.000000000000000000 ) ) ;
#30798=CARTESIAN_POINT ( 'NONE',  ( 9.457646018065525792E-16, -72.31249999863440792, 5.148502694627439702 ) ) ;
#30799=DIRECTION ( 'NONE',  ( 0.000000000000000000, 0.000000000000000000, 1.000000000000000000 ) ) ;
#30802=ORIENTED_EDGE ( 'NONE', *, *, #4992, .F. ) ;
#30809=CARTESIAN_POINT ( 'NONE',  ( -4.458734124999997661, 15.52083333469892779, 2.574251347313722516 ) ) ;
#30810=FACE_OUTER_BOUND ( 'NONE', #42461, .T. ) ;
#30815=CARTESIAN_POINT ( 'NONE',  ( -2.499999999999996447, -50.70833333060213732, 4.330127018922195425 ) ) ;
#30816=CARTESIAN_POINT ( 'NONE',  ( -4.458734124999998549, -87.22916666530107932, 2.574251347313722516 ) ) ;
#30817=CARTESIAN_POINT ( 'NONE',  ( 9.457646018065525792E-16, -1.062499998634405696, 5.148502694627439702 ) ) ;
#30818=CARTESIAN_POINT ( 'NONE',  ( 3.061616997868383141E-16, -168.8750000027312126, -5.000000000000000000 ) ) ;
#30819=EDGE_CURVE ( 'NONE', #55230, #37557, #45995, .T. ) ;
#30821=CARTESIAN_POINT ( 'NONE',  ( -4.458734124999999437, -28.56249999863440081, 0.000000000000000000 ) ) ;
#30826=CARTESIAN_POINT ( 'NONE',  ( 2.229367062500001939, 19.02083333469892779, 3.861377020970579999 ) ) ;
#30829=CARTESIAN_POINT ( 'NONE',  ( -6.972266317189433020E-16, 1.750000000000000444, -5.000000000000000000 ) ) ;
#30830=CARTESIAN_POINT ( 'NONE',  ( 4.458734125000000326, -77.14583333196775072, 2.574251347313718519 ) ) ;
#30832=CARTESIAN_POINT ( 'NONE',  ( -5.000000000000000000, 23.04166666939785557, -2.886751345948128211 ) ) ;
#30833=EDGE_LOOP ( 'NONE', ( #17531, #21078, #24366, #10750 ) ) ;
#30834=CARTESIAN_POINT ( 'NONE',  ( 2.500000000000002220, -1.541666663935480130, 4.330127018922192761 ) ) ;
#30838=CARTESIAN_POINT ( 'NONE',  ( 5.000000000000000888, -25.58333333333333215, 2.886751345948126879 ) ) ;
#30839=CARTESIAN_POINT ( 'NONE',  ( -4.458734124999999437, -26.31249999863440792, 0.000000000000000000 ) ) ;
#30840=CARTESIAN_POINT ( 'NONE',  ( -4.458734124999997661, -88.22916666530107932, 2.574251347313722516 ) ) ;
#30841=CARTESIAN_POINT ( 'NONE',  ( -5.000000000000000000, -21.87499999726881228, 0.000000000000000000 ) ) ;
#30842=CARTESIAN_POINT ( 'NONE',  ( 2.229367062500001939, -55.97916666530107221, 3.861377020970579999 ) ) ;
#30844=CARTESIAN_POINT ( 'NONE',  ( 1.975475456537005874E-15, -49.74999999999999289, 5.000000000000000000 ) ) ;
#30845=CARTESIAN_POINT ( 'NONE',  ( -3.152548672688508926E-16, -2.812499998634407028, -5.148502694627439702 ) ) ;
#30847=CARTESIAN_POINT ( 'NONE',  ( 2.499999999999998668, -64.33333333333332860, -4.330127018922193649 ) ) ;
#30848=CARTESIAN_POINT ( 'NONE',  ( -8.190561711645485556E-16, -153.9375000013655779, 4.458734124999999437 ) ) ;
#30852=CARTESIAN_POINT ( 'NONE',  ( 3.535533905932736864, -160.1250000000000284, 3.535533905932738641 ) ) ;
#30856=CARTESIAN_POINT ( 'NONE',  ( -3.152548672688508926E-16, -13.81249999863440436, -5.148502694627439702 ) ) ;
#30857=CARTESIAN_POINT ( 'NONE',  ( 4.458734124999998549, -50.97916666530107221, -2.574251347313721627 ) ) ;
#30859=CARTESIAN_POINT ( 'NONE',  ( -3.152801135295367096, -143.0625000013655779, -3.152801135295367541 ) ) ;
#30862=VERTEX_POINT ( 'NONE', #22430 ) ;
#30864=CARTESIAN_POINT ( 'NONE',  ( -2.229367062499996610, 25.60416666803225993, 3.861377020970582219 ) ) ;
#30866=CARTESIAN_POINT ( 'NONE',  ( -4.999999999999998224, -12.79166666393547835, 2.886751345948131764 ) ) ;
#30867=ORIENTED_EDGE ( 'NONE', *, *, #16065, .T. ) ;
#30869=ADVANCED_FACE ( 'NONE', ( #42027 ), #17601, .T. ) ;
#30873=CARTESIAN_POINT ( 'NONE',  ( 4.458734124999998549, -5.729166665301072214, -2.574251347313721627 ) ) ;
#30874=CARTESIAN_POINT ( 'NONE',  ( 5.000000000000000000, 6.708333336064521646, -2.886751345948130876 ) ) ;
#30875=CARTESIAN_POINT ( 'NONE',  ( -4.458734124999999437, -147.9375000013656063, -5.460374474430324690E-16 ) ) ;
#30878=EDGE_LOOP ( 'NONE', ( #37091, #10600, #26219, #17084 ) ) ;
#30889=CARTESIAN_POINT ( 'NONE',  ( -4.458734124999997661, 9.770833334698927786, 2.574251347313722516 ) ) ;
#30892=CARTESIAN_POINT ( 'NONE',  ( -3.152548672688508926E-16, -15.81249999863440436, -5.148502694627439702 ) ) ;
#30894=CARTESIAN_POINT ( 'NONE',  ( -3.152801135295367985, -164.8125000013656063, 3.152801135295367096 ) ) ;
#30899=LINE ( 'NONE', #30574, #54500 ) ;
#30901=CARTESIAN_POINT ( 'NONE',  ( -1.339745962155613812, -36.20534180126147561, -5.000000000000000000 ) ) ;
#30902=CARTESIAN_POINT ( 'NONE',  ( 9.457646018065525792E-16, -36.06249999863440792, 5.148502694627439702 ) ) ;
#30903=CARTESIAN_POINT ( 'NONE',  ( 1.975475456537005874E-15, 19.37500000273118772, 5.000000000000000000 ) ) ;
#30907=ORIENTED_EDGE ( 'NONE', *, *, #28252, .F. ) ;
#30911=CARTESIAN_POINT ( 'NONE',  ( 2.500000000000002220, -0.6666666666666660745, 4.330127018922192761 ) ) ;
#30912=CARTESIAN_POINT ( 'NONE',  ( -4.458734124999999437, -72.31249999863439371, 0.000000000000000000 ) ) ;
#30914=CARTESIAN_POINT ( 'NONE',  ( -5.000000000000000000, -7.958333330602145317, -2.886751345948128211 ) ) ;
#30915=CARTESIAN_POINT ( 'NONE',  ( -4.458734124999999437, -40.31249999863440081, 0.000000000000000000 ) ) ;
#30917=DIRECTION ( 'NONE',  ( 0.000000000000000000, 0.000000000000000000, 1.000000000000000000 ) ) ;
#30918=CARTESIAN_POINT ( 'NONE',  ( -4.458734124999998549, 10.52083333469892779, 2.574251347313722516 ) ) ;
#30920=CARTESIAN_POINT ( 'NONE',  ( -2.499999999999996447, -47.83333333333332149, 4.330127018922195425 ) ) ;
#30922=CARTESIAN_POINT ( 'NONE',  ( -1.339745962155610925, -34.79465819873851729, 5.000000000000000000 ) ) ;
#30923=CARTESIAN_POINT ( 'NONE',  ( 4.458734125000001214, -76.89583333196775072, 2.574251347313718519 ) ) ;
#30924=CARTESIAN_POINT ( 'NONE',  ( -5.000000000000000000, -169.5000000000000000, -6.123233995736766282E-16 ) ) ;
#30925=CARTESIAN_POINT ( 'NONE',  ( -4.458734124999998549, -87.22916666530107932, 2.574251347313722516 ) ) ;
#30928=CARTESIAN_POINT ( 'NONE',  ( 4.458734124999998549, -37.97916666530107932, -2.574251347313721627 ) ) ;
#30929=ORIENTED_EDGE ( 'NONE', *, *, #37056, .F. ) ;
#30930=CARTESIAN_POINT ( 'NONE',  ( -4.999999999999998224, 24.20833333606451987, 2.886751345948131764 ) ) ;
#30935=CARTESIAN_POINT ( 'NONE',  ( 1.975475456537005874E-15, -22.62499999726880873, 5.000000000000000000 ) ) ;
#30938=CARTESIAN_POINT ( 'NONE',  ( 4.458734124999998549, -62.97916666530107221, -2.574251347313721627 ) ) ;
#30940=EDGE_LOOP ( 'NONE', ( #1694, #59520, #23635, #45409 ) ) ;
#30942=CARTESIAN_POINT ( 'NONE',  ( 1.975475456537005874E-15, -19.62499999726881228, 5.000000000000000000 ) ) ;
#30945=CARTESIAN_POINT ( 'NONE',  ( 2.229367062500001939, 6.020833334698927786, 3.861377020970579999 ) ) ;
#30947=CARTESIAN_POINT ( 'NONE',  ( 3.152801135295366208, -159.5625000013656063, 3.152801135295367985 ) ) ;
#30948=LINE ( 'NONE', #60556, #29586 ) ;
#30953=CARTESIAN_POINT ( 'NONE',  ( 5.000000000000000000, 25.70833333606452342, -2.886751345948130876 ) ) ;
#30955=CARTESIAN_POINT ( 'NONE',  ( -6.972266317189433020E-16, -68.24999999999998579, -5.000000000000000000 ) ) ;
#30958=CARTESIAN_POINT ( 'NONE',  ( -2.499999999999996447, -28.83333333333333570, 4.330127018922195425 ) ) ;
#30961=CARTESIAN_POINT ( 'NONE',  ( 4.458734124999998549, 26.27083333469892423, -2.574251347313721627 ) ) ;
#30964=CARTESIAN_POINT ( 'NONE',  ( -3.152548672688508926E-16, 1.187500001365596081, -5.148502694627439702 ) ) ;
#30965=CARTESIAN_POINT ( 'NONE',  ( -3.535533905932738641, -149.5000000027311842, 3.535533905932737309 ) ) ;
#30967=CARTESIAN_POINT ( 'NONE',  ( -5.000000000000000888, -145.6875000027312126, -2.071067811865475949 ) ) ;
#30968=CARTESIAN_POINT ( 'NONE',  ( -9.184850993605147944E-16, -155.3750000027311842, 5.000000000000000000 ) ) ;
#30972=CARTESIAN_POINT ( 'NONE',  ( -2.071067811865475061, -140.6875000000000568, -5.000000000000000888 ) ) ;
#30973=CARTESIAN_POINT ( 'NONE',  ( 1.975475456537005874E-15, -87.75000000000001421, 5.000000000000000000 ) ) ;
#30975=CARTESIAN_POINT ( 'NONE',  ( -3.152801135295367985, -161.0625000013656063, 3.152801135295367096 ) ) ;
#30978=CARTESIAN_POINT ( 'NONE',  ( -4.458734125000000326, -141.0000000013656063, -1.846868145590735644 ) ) ;
#30979=EDGE_LOOP ( 'NONE', ( #45076, #5059, #17104, #22480 ) ) ;
#30980=CARTESIAN_POINT ( 'NONE',  ( 4.458734124999999437, 23.93750000136559564, -5.460374474430324690E-16 ) ) ;
#30981=VERTEX_POINT ( 'NONE', #27551 ) ;
#30985=CARTESIAN_POINT ( 'NONE',  ( 1.060575238724906964E-15, 16.25000000000000000, 5.773502691896257311 ) ) ;
#30986=CARTESIAN_POINT ( 'NONE',  ( -2.229367062500000163, -52.47916666530107221, -3.861377020970580443 ) ) ;
#30987=CARTESIAN_POINT ( 'NONE',  ( 4.458734125000001214, -13.89583333196774007, 2.574251347313718519 ) ) ;
#30990=FACE_OUTER_BOUND ( 'NONE', #3815, .T. ) ;
#30993=CARTESIAN_POINT ( 'NONE',  ( -5.000000000000000000, -33.08333333333332149, -2.886751345948128211 ) ) ;
#30994=CARTESIAN_POINT ( 'NONE',  ( 4.458734124999999437, -139.6875000013656063, 0.000000000000000000 ) ) ;
#30995=CARTESIAN_POINT ( 'NONE',  ( -6.972266317189433020E-16, -59.25000000000000000, -5.000000000000000000 ) ) ;
#30997=CARTESIAN_POINT ( 'NONE',  ( -2.229367062499996610, -57.14583333196773651, 3.861377020970582219 ) ) ;
#30998=CARTESIAN_POINT ( 'NONE',  ( 3.152801135295366208, -152.8125000013656063, 3.152801135295367985 ) ) ;
#30999=CARTESIAN_POINT ( 'NONE',  ( -4.458734124999998549, -66.22916666530107932, 2.574251347313722516 ) ) ;
#31000=EDGE_CURVE ( 'NONE', #62942, #27799, #56202, .T. ) ;
#31002=CARTESIAN_POINT ( 'NONE',  ( 1.060575238724906964E-15, -57.62499999726880873, 5.773502691896257311 ) ) ;
#31003=ORIENTED_EDGE ( 'NONE', *, *, #47630, .T. ) ;
#31007=CARTESIAN_POINT ( 'NONE',  ( -8.190561711645485556E-16, -151.6875000013656063, 4.458734124999999437 ) ) ;
#31009=CARTESIAN_POINT ( 'NONE',  ( 1.339745962155612702, -54.29465819873851729, -5.000000000000000000 ) ) ;
#31012=CARTESIAN_POINT ( 'NONE',  ( -4.458734124999999437, -47.56249999863440792, 0.000000000000000000 ) ) ;
#31013=ORIENTED_EDGE ( 'NONE', *, *, #28709, .T. ) ;
#31015=EDGE_CURVE ( 'NONE', #21097, #25291, #26653, .T. ) ;
#31017=CARTESIAN_POINT ( 'NONE',  ( 9.457646018065525792E-16, 25.93750000136559564, 5.148502694627439702 ) ) ;
#31020=CARTESIAN_POINT ( 'NONE',  ( 1.975475456537005874E-15, -61.62499999726880873, 5.000000000000000000 ) ) ;
#31021=( BOUNDED_CURVE ( )  B_SPLINE_CURVE ( 2, ( #32075, #51080, #51712, #55907, #31129, #56858, #32398, #52024, #6697 ),
 .UNSPECIFIED., .F., .F. ) 
 B_SPLINE_CURVE_WITH_KNOTS ( ( 3, 2, 2, 2, 3 ),
 ( 0.2083333333333335091, 0.2125000000000001610, 0.2166666666666668406, 0.2208333333333335202, 0.2250000000000001998 ),
 .UNSPECIFIED. ) 
 CURVE ( )  GEOMETRIC_REPRESENTATION_ITEM ( )  RATIONAL_B_SPLINE_CURVE ( ( 0.9999999999999970024, 0.9238795325112897361, 1.000000000000000000, 0.9238795325112867385, 1.000000000000000000, 0.9238795325112867385, 1.000000000000000000, 0.9238795325112831858, 1.000000000000003553 ) ) 
 REPRESENTATION_ITEM ( '' )  );
#31022=ORIENTED_EDGE ( 'NONE', *, *, #18867, .F. ) ;
#31028=CARTESIAN_POINT ( 'NONE',  ( -3.535533905932738641, -157.3750000000000284, 3.535533905932737309 ) ) ;
#31031=CARTESIAN_POINT ( 'NONE',  ( 1.975475456537005874E-15, -42.62499999726880873, 5.000000000000000000 ) ) ;
#31034=CYLINDRICAL_SURFACE ( 'NONE', #25472, 5.000000000000000000 ) ;
#31036=ORIENTED_EDGE ( 'NONE', *, *, #14231, .T. ) ;
#31039=CARTESIAN_POINT ( 'NONE',  ( -5.000000000000000000, -155.6250000027311842, -6.123233995736766282E-16 ) ) ;
#31040=ORIENTED_EDGE ( 'NONE', *, *, #48347, .T. ) ;
#31050=CARTESIAN_POINT ( 'NONE',  ( -4.458734124999999437, -21.31249999863440436, 0.000000000000000000 ) ) ;
#31051=CARTESIAN_POINT ( 'NONE',  ( 0.000000000000000000, -170.0000000000000000, 0.000000000000000000 ) ) ;
#31052=CARTESIAN_POINT ( 'NONE',  ( 3.535533905932736864, -152.1250000000000000, 3.535533905932738641 ) ) ;
#31054=CARTESIAN_POINT ( 'NONE',  ( -4.458734125000000326, -150.0000000013655779, -1.846868145590735644 ) ) ;
#31056=CARTESIAN_POINT ( 'NONE',  ( -4.458734124999997661, -45.47916666530106511, 2.574251347313722516 ) ) ;
#31060=CARTESIAN_POINT ( 'NONE',  ( 2.229367062500001939, -89.97916666530106511, 3.861377020970579999 ) ) ;
#31061=CARTESIAN_POINT ( 'NONE',  ( -3.152548672688508926E-16, 2.437500001365594304, -5.148502694627439702 ) ) ;
#31062=CARTESIAN_POINT ( 'NONE',  ( 3.061616997868383141E-16, -160.8750000027311842, -5.000000000000000000 ) ) ;
#31063=CARTESIAN_POINT ( 'NONE',  ( 1.339745962155615144, -11.58034179853029499, 4.999999999999999112 ) ) ;
#31065=CARTESIAN_POINT ( 'NONE',  ( -4.458734124999998549, 17.52083333469892779, 2.574251347313722516 ) ) ;
#31067=CARTESIAN_POINT ( 'NONE',  ( -2.500000000000000444, 9.958333336064519870, -4.330127018922193649 ) ) ;
#31069=CARTESIAN_POINT ( 'NONE',  ( -9.184850993605147944E-16, -162.3750000027311842, 5.000000000000000000 ) ) ;
#31070=ORIENTED_EDGE ( 'NONE', *, *, #12302, .F. ) ;
#31071=CARTESIAN_POINT ( 'NONE',  ( 1.975475456537005874E-15, -34.62499999726880873, 5.000000000000000000 ) ) ;
#31072=CARTESIAN_POINT ( 'NONE',  ( 2.229367062500001939, -40.97916666530107221, 3.861377020970579999 ) ) ;
#31073=CARTESIAN_POINT ( 'NONE',  ( 1.846868145590735200, -162.5000000013655779, -4.458734125000000326 ) ) ;
#31076=CARTESIAN_POINT ( 'NONE',  ( 5.000000000000000000, -37.29166666393548013, -2.886751345948129988 ) ) ;
#31077=ADVANCED_FACE ( 'NONE', ( #10140 ), #33952, .T. ) ;
#31079=CARTESIAN_POINT ( 'NONE',  ( -2.229367062499996610, -18.14583333196773651, 3.861377020970582219 ) ) ;
#31081=CARTESIAN_POINT ( 'NONE',  ( -2.499999999999996447, -85.83333333333332860, 4.330127018922195425 ) ) ;
#31082=CARTESIAN_POINT ( 'NONE',  ( 4.458734125000000326, -166.3750000013655779, -1.846868145590734978 ) ) ;
#31083=CARTESIAN_POINT ( 'NONE',  ( -2.500000000000000444, -85.04166666393547303, -4.330127018922193649 ) ) ;
#31084=CARTESIAN_POINT ( 'NONE',  ( -5.000000000000000000, -34.87499999726881583, 0.000000000000000000 ) ) ;
#31087=CARTESIAN_POINT ( 'NONE',  ( -3.152548672688508926E-16, -31.81249999863440792, -5.148502694627439702 ) ) ;
#31088=CARTESIAN_POINT ( 'NONE',  ( -1.339745962155613812, -50.20534180126148271, -5.000000000000000000 ) ) ;
#31089=EDGE_CURVE ( 'NONE', #25310, #19310, #52579, .T. ) ;
#31090=VERTEX_POINT ( 'NONE', #33640 ) ;
#31092=EDGE_CURVE ( 'NONE', #16051, #45174, #36990, .T. ) ;
#31095=EDGE_LOOP ( 'NONE', ( #29666, #54182, #62670, #38054 ) ) ;
#31098=CARTESIAN_POINT ( 'NONE',  ( 9.457646018065525792E-16, -82.31249999863440792, 5.148502694627439702 ) ) ;
#31101=CARTESIAN_POINT ( 'NONE',  ( -3.152801135295367985, -141.0625000013655779, 3.152801135295367096 ) ) ;
#31102=CARTESIAN_POINT ( 'NONE',  ( -2.500000000000000444, -58.16666666666665719, -4.330127018922193649 ) ) ;
#31104=CARTESIAN_POINT ( 'NONE',  ( 9.457646018065525792E-16, -43.06249999863440081, 5.148502694627439702 ) ) ;
#31110=CARTESIAN_POINT ( 'NONE',  ( 1.975475456537005874E-15, -39.62499999726880162, 5.000000000000000000 ) ) ;
#31112=CARTESIAN_POINT ( 'NONE',  ( -4.458734124999998549, -80.47916666530106511, 2.574251347313722516 ) ) ;
#31115=LINE ( 'NONE', #22671, #4867 ) ;
#31118=CARTESIAN_POINT ( 'NONE',  ( 2.071067811865392461, -146.1875000000000284, 5.000000000000084377 ) ) ;
#31121=CARTESIAN_POINT ( 'NONE',  ( -5.000000000000000000, -168.6250000027312126, -6.123233995736766282E-16 ) ) ;
#31123=CARTESIAN_POINT ( 'NONE',  ( -4.458734124999999437, 17.35416666803225993, -2.574251347313719407 ) ) ;
#31124=DIRECTION ( 'NONE',  ( -0.000000000000000000, 1.000000000000000000, -0.000000000000000000 ) ) ;
#31129=CARTESIAN_POINT ( 'NONE',  ( -5.000000000000000000, -163.5000000000000000, -6.123233995736766282E-16 ) ) ;
#31130=CARTESIAN_POINT ( 'NONE',  ( 9.457646018065525792E-16, -83.06249999863439371, 5.148502694627439702 ) ) ;
#31131=CARTESIAN_POINT ( 'NONE',  ( -4.458734124999997661, -1.229166665301071548, 2.574251347313722516 ) ) ;
#31132=ORIENTED_EDGE ( 'NONE', *, *, #654, .T. ) ;
#31133=CARTESIAN_POINT ( 'NONE',  ( -4.458734124999997661, -32.47916666530106511, 2.574251347313722516 ) ) ;
#31138=CARTESIAN_POINT ( 'NONE',  ( -4.458734124999999437, 21.60416666803225993, -2.574251347313719407 ) ) ;
#31140=CARTESIAN_POINT ( 'NONE',  ( 1.339745962155612702, 1.705341801261480272, -5.000000000000000000 ) ) ;
#31141=CARTESIAN_POINT ( 'NONE',  ( -4.458734124999999437, -78.56249999863440792, 0.000000000000000000 ) ) ;
#31144=CARTESIAN_POINT ( 'NONE',  ( -2.500000000000000444, 26.95833333606451632, -4.330127018922193649 ) ) ;
#31147=CARTESIAN_POINT ( 'NONE',  ( -2.071067811865306307, -149.6874999999999716, -5.000000000000171418 ) ) ;
#31148=CARTESIAN_POINT ( 'NONE',  ( -2.499999999999996447, -23.83333333333333215, 4.330127018922195425 ) ) ;
#31149=CARTESIAN_POINT ( 'NONE',  ( 2.229367062499998831, -27.64583333196774007, -3.861377020970580887 ) ) ;
#31150=CARTESIAN_POINT ( 'NONE',  ( 4.458734124999999437, -88.81249999863439371, -5.460374474430324690E-16 ) ) ;
#31152=EDGE_CURVE ( 'NONE', #52220, #2151, #53260, .T. ) ;
#31153=CARTESIAN_POINT ( 'NONE',  ( -2.500000000000000444, -22.04166666393548013, -4.330127018922193649 ) ) ;
#31154=CARTESIAN_POINT ( 'NONE',  ( 4.458734125000001214, -52.89583333196772941, 2.574251347313718519 ) ) ;
#31157=CARTESIAN_POINT ( 'NONE',  ( 0.000000000000000000, -170.0000000000000000, 0.000000000000000000 ) ) ;
#31158=CARTESIAN_POINT ( 'NONE',  ( -2.229367062499996610, -5.395833331967740953, 3.861377020970582219 ) ) ;
#31160=CARTESIAN_POINT ( 'NONE',  ( -5.000000000000000000, -70.08333333333332860, -2.886751345948128211 ) ) ;
#31161=CARTESIAN_POINT ( 'NONE',  ( 1.846868145590735200, -152.5000000013656347, -4.458734125000000326 ) ) ;
#31163=LINE ( 'NONE', #7374, #52260 ) ;
#31164=CARTESIAN_POINT ( 'NONE',  ( -9.184850993605147944E-16, -160.2500000000000000, 5.000000000000000000 ) ) ;
#31165=CARTESIAN_POINT ( 'NONE',  ( 5.000000000000000000, -71.29166666393547303, -2.886751345948129988 ) ) ;
#31169=CARTESIAN_POINT ( 'NONE',  ( -2.229367062500000163, -17.72916666530106866, -3.861377020970580443 ) ) ;
#31170=CARTESIAN_POINT ( 'NONE',  ( 2.229367062499998831, -51.89583333196773651, -3.861377020970580887 ) ) ;
#31172=CARTESIAN_POINT ( 'NONE',  ( 4.458734124999999437, -146.5000000013656347, 1.846868145590737864 ) ) ;
#31175=ORIENTED_EDGE ( 'NONE', *, *, #10172, .F. ) ;
#31177=DIRECTION ( 'NONE',  ( 0.000000000000000000, 0.000000000000000000, 1.000000000000000000 ) ) ;
#31178=CARTESIAN_POINT ( 'NONE',  ( -4.458734124999998549, 25.52083333469893134, 2.574251347313722516 ) ) ;
#31180=EDGE_CURVE ( 'NONE', #59835, #42312, #41474, .T. ) ;
#31181=CARTESIAN_POINT ( 'NONE',  ( 5.000000000000000000, -50.41666666666666430, -2.886751345948130876 ) ) ;
#31184=FACE_OUTER_BOUND ( 'NONE', #32926, .T. ) ;
#31187=CARTESIAN_POINT ( 'NONE',  ( -4.458734124999999437, -8.312499998634406140, 0.000000000000000000 ) ) ;
#31189=CARTESIAN_POINT ( 'NONE',  ( -4.458734124999999437, -145.0000000013656063, -1.846868145590735644 ) ) ;
#31192=CARTESIAN_POINT ( 'NONE',  ( 6.123233995736766282E-16, -170.0000000000000000, -5.000000000000000000 ) ) ;
#31197=CARTESIAN_POINT ( 'NONE',  ( 1.339745962155615144, -88.58034179853028434, 4.999999999999999112 ) ) ;
#31204=CARTESIAN_POINT ( 'NONE',  ( -4.458734124999999437, 14.60416666803226171, -2.574251347313719407 ) ) ;
#31206=CARTESIAN_POINT ( 'NONE',  ( 9.457646018065525792E-16, -12.31249999863440259, 5.148502694627439702 ) ) ;
#31207=( BOUNDED_CURVE ( )  B_SPLINE_CURVE ( 2, ( #6230, #50602, #11990, #31616, #26795 ),
 .UNSPECIFIED., .F., .F. ) 
 B_SPLINE_CURVE_WITH_KNOTS ( ( 3, 2, 3 ),
 ( 0.9979166666666666741, 0.9986111111111111160, 1.000000000000000000 ),
 .UNSPECIFIED. ) 
 CURVE ( )  GEOMETRIC_REPRESENTATION_ITEM ( )  RATIONAL_B_SPLINE_CURVE ( ( 0.9330127018922194093, 0.9330127018922194093, 1.000000000000000000, 0.8660254037844387076, 1.000000000000000000 ) ) 
 REPRESENTATION_ITEM ( '' )  );
#31209=CARTESIAN_POINT ( 'NONE',  ( 4.458734125000000326, -164.3750000013656063, -1.846868145590734978 ) ) ;
#31214=CARTESIAN_POINT ( 'NONE',  ( -6.972266317189433020E-16, -89.12499999726880162, -5.000000000000000000 ) ) ;
#31215=CARTESIAN_POINT ( 'NONE',  ( 9.457646018065525792E-16, -37.06249999863440792, 5.148502694627439702 ) ) ;
#31218=CARTESIAN_POINT ( 'NONE',  ( -5.000000000000000000, -13.99999999999999822, 0.000000000000000000 ) ) ;
#31222=CARTESIAN_POINT ( 'NONE',  ( 1.975475456537005874E-15, 12.24999999999999822, 5.000000000000000000 ) ) ;
#31223=CARTESIAN_POINT ( 'NONE',  ( -5.000000000000000000, -6.999999999999999112, 0.000000000000000000 ) ) ;
#31224=CARTESIAN_POINT ( 'NONE',  ( -4.458734124999999437, -73.31249999863439371, 0.000000000000000000 ) ) ;
#31227=CARTESIAN_POINT ( 'NONE',  ( 5.000000000000000888, -8.458333330602146205, 2.886751345948126879 ) ) ;
#31228=CARTESIAN_POINT ( 'NONE',  ( 9.457646018065525792E-16, -39.06249999863440081, 5.148502694627439702 ) ) ;
#31231=CARTESIAN_POINT ( 'NONE',  ( 9.457646018065525792E-16, 13.68750000136559208, 5.148502694627439702 ) ) ;
#31234=CARTESIAN_POINT ( 'NONE',  ( -2.500000000000000444, -53.16666666666666430, -4.330127018922193649 ) ) ;
#31237=CARTESIAN_POINT ( 'NONE',  ( -4.458734124999999437, -74.39583333196775072, -2.574251347313719407 ) ) ;
#31238=CARTESIAN_POINT ( 'NONE',  ( 1.846868145590736310, -139.8750000013656063, 4.458734124999999437 ) ) ;
#31239=CARTESIAN_POINT ( 'NONE',  ( 4.458734124999999437, -84.81249999863439371, -5.460374474430324690E-16 ) ) ;
#31241=CARTESIAN_POINT ( 'NONE',  ( 9.457646018065525792E-16, -38.31249999863441502, 5.148502694627439702 ) ) ;
#31242=CARTESIAN_POINT ( 'NONE',  ( 5.000000000000000000, -72.50000000000000000, -6.123233995736766282E-16 ) ) ;
#31247=( BOUNDED_CURVE ( )  B_SPLINE_CURVE ( 2, ( #39998, #15578, #36149, #56415, #32584, #50941, #12959, #56087, #56728 ),
 .UNSPECIFIED., .F., .F. ) 
 B_SPLINE_CURVE_WITH_KNOTS ( ( 3, 2, 2, 2, 3 ),
 ( 0.1229166666666666741, 0.1236111111111111160, 0.1250000000000000000, 0.1263888888888888840, 0.1270833333333333259 ),
 .UNSPECIFIED. ) 
 CURVE ( )  GEOMETRIC_REPRESENTATION_ITEM ( )  RATIONAL_B_SPLINE_CURVE ( ( 0.9330127018922194093, 0.9330127018922200755, 1.000000000000000000, 0.8660254037844387076, 1.000000000000000000, 0.8660254037844387076, 1.000000000000000000, 0.9330127018922194093, 0.9330127018922194093 ) ) 
 REPRESENTATION_ITEM ( '' )  );
#31248=CARTESIAN_POINT ( 'NONE',  ( 2.071067811865602959, -151.8125000000000284, -4.999999999999874767 ) ) ;
#31249=CARTESIAN_POINT ( 'NONE',  ( -2.229367062500000163, -65.72916666530106511, -3.861377020970580443 ) ) ;
#31253=CARTESIAN_POINT ( 'NONE',  ( 5.000000000000000888, -62.58333333333333570, 2.886751345948126879 ) ) ;
#31256=AXIS2_PLACEMENT_3D ( 'NONE', #170, #24276, #43880 ) ;
#31257=CARTESIAN_POINT ( 'NONE',  ( 4.458734124999998549, 6.270833334698928674, -2.574251347313721627 ) ) ;
#31259=CARTESIAN_POINT ( 'NONE',  ( 1.846868145590736310, -160.6250000013656063, 4.458734124999997661 ) ) ;
#31261=ORIENTED_EDGE ( 'NONE', *, *, #60913, .T. ) ;
#31264=CARTESIAN_POINT ( 'NONE',  ( 1.339745962155615144, -71.58034179853027013, 4.999999999999999112 ) ) ;
#31267=CYLINDRICAL_SURFACE ( 'NONE', #18072, 5.000000000000000000 ) ;
#31269=CARTESIAN_POINT ( 'NONE',  ( -6.972266317189433020E-16, -83.12499999726878741, -5.000000000000000000 ) ) ;
#31270=CARTESIAN_POINT ( 'NONE',  ( 2.500000000000002220, -58.66666666666665719, 4.330127018922192761 ) ) ;
#31273=CARTESIAN_POINT ( 'NONE',  ( -4.458734124999999437, 2.437500001365593860, 0.000000000000000000 ) ) ;
#31274=CARTESIAN_POINT ( 'NONE',  ( -2.071067811865604735, -149.4375000027312410, 4.999999999999872990 ) ) ;
#31276=CARTESIAN_POINT ( 'NONE',  ( 5.000000000000000888, -144.0625000027311842, -2.071067811865475505 ) ) ;
#31281=CYLINDRICAL_SURFACE ( 'NONE', #23695, 5.000000000000000000 ) ;
#31282=CARTESIAN_POINT ( 'NONE',  ( -5.000000000000000000, -88.08333333333332860, -2.886751345948128211 ) ) ;
#31284=CARTESIAN_POINT ( 'NONE',  ( -3.152801135295367096, -160.3125000013656063, -3.152801135295367541 ) ) ;
#31288=ORIENTED_EDGE ( 'NONE', *, *, #23528, .T. ) ;
#31289=CARTESIAN_POINT ( 'NONE',  ( -4.458734124999998549, 23.52083333469892779, 2.574251347313722516 ) ) ;
#31294=CARTESIAN_POINT ( 'NONE',  ( -4.999999999999998224, -2.791666663935478354, 2.886751345948131764 ) ) ;
#31295=CARTESIAN_POINT ( 'NONE',  ( -3.535250795749689387E-16, 8.750000000000000000, -5.773502691896257311 ) ) ;
#31296=CARTESIAN_POINT ( 'NONE',  ( 2.229367062500001939, -57.97916666530107932, 3.861377020970579999 ) ) ;
#31297=CARTESIAN_POINT ( 'NONE',  ( 2.229367062500001939, -13.97916666530107221, 3.861377020970579999 ) ) ;
#31298=CARTESIAN_POINT ( 'NONE',  ( -6.972266317189433020E-16, -6.249999999999999112, -5.000000000000000000 ) ) ;
#31300=CARTESIAN_POINT ( 'NONE',  ( -2.500000000000000444, 13.83333333333333215, -4.330127018922193649 ) ) ;
#31303=CARTESIAN_POINT ( 'NONE',  ( 1.060575238724906964E-15, -35.75000000000000711, 5.773502691896257311 ) ) ;
#31304=LINE ( 'NONE', #52205, #63371 ) ;
#31305=EDGE_CURVE ( 'NONE', #16219, #35844, #36188, .T. ) ;
#31308=CARTESIAN_POINT ( 'NONE',  ( -9.184850993605147944E-16, -140.3750000027312126, 5.000000000000000000 ) ) ;
#31309=CARTESIAN_POINT ( 'NONE',  ( 4.458734124999999437, -59.81249999863440081, -5.460374474430324690E-16 ) ) ;
#31310=CARTESIAN_POINT ( 'NONE',  ( 4.458734125000000326, -150.6250000013655779, -1.846868145590734978 ) ) ;
#31311=CARTESIAN_POINT ( 'NONE',  ( -2.229367062500000163, -72.47916666530107932, -3.861377020970580443 ) ) ;
#31313=VECTOR ( 'NONE', #13534, 1000.000000000000000 ) ;
#31314=CARTESIAN_POINT ( 'NONE',  ( 2.229367062499998831, -21.89583333196774007, -3.861377020970580887 ) ) ;
#31315=CARTESIAN_POINT ( 'NONE',  ( 2.499999999999998668, -62.20833333060214443, -4.330127018922193649 ) ) ;
#31317=CARTESIAN_POINT ( 'NONE',  ( 2.500000000000002220, -31.54166666393548724, 4.330127018922192761 ) ) ;
#31322=CARTESIAN_POINT ( 'NONE',  ( -1.846868145590734756, -151.1250000013655779, -4.458734125000000326 ) ) ;
#31323=ORIENTED_EDGE ( 'NONE', *, *, #33581, .F. ) ;
#31324=CYLINDRICAL_SURFACE ( 'NONE', #53942, 5.000000000000000000 ) ;
#31326=CARTESIAN_POINT ( 'NONE',  ( 0.000000000000000000, -170.0000000000000000, 0.000000000000000000 ) ) ;
#31327=CARTESIAN_POINT ( 'NONE',  ( -2.229367062499996610, -48.39583333196772941, 3.861377020970582219 ) ) ;
#31328=VERTEX_POINT ( 'NONE', #6288 ) ;
#31329=( BOUNDED_CURVE ( )  B_SPLINE_CURVE ( 2, ( #54362, #5466, #20593, #50160, #54675, #49840, #54028, #29256, #6115 ),
 .UNSPECIFIED., .F., .F. ) 
 B_SPLINE_CURVE_WITH_KNOTS ( ( 3, 2, 2, 2, 3 ),
 ( 0.5020833333333333259, 0.5027777777777777679, 0.5041666666666666519, 0.5055555555555555358, 0.5062499999999999778 ),
 .UNSPECIFIED. ) 
 CURVE ( )  GEOMETRIC_REPRESENTATION_ITEM ( )  RATIONAL_B_SPLINE_CURVE ( ( 0.9330127018922194093, 0.9330127018922194093, 1.000000000000000000, 0.8660254037844387076, 1.000000000000000000, 0.8660254037844387076, 1.000000000000000000, 0.9330127018922194093, 0.9330127018922194093 ) ) 
 REPRESENTATION_ITEM ( '' )  );
#31331=CARTESIAN_POINT ( 'NONE',  ( 4.458734124999999437, 25.18750000136559208, -5.460374474430324690E-16 ) ) ;
#31333=CARTESIAN_POINT ( 'NONE',  ( 1.339745962155615144, -61.58034179853027723, 4.999999999999999112 ) ) ;
#31334=ORIENTED_EDGE ( 'NONE', *, *, #28640, .F. ) ;
#31342=FACE_OUTER_BOUND ( 'NONE', #7877, .T. ) ;
#31345=FACE_OUTER_BOUND ( 'NONE', #5679, .T. ) ;
#31347=CARTESIAN_POINT ( 'NONE',  ( 2.071067811865476394, -159.3125000027311842, 5.000000000000000000 ) ) ;
#31350=ADVANCED_FACE ( 'NONE', ( #5966 ), #11413, .T. ) ;
#31359=CARTESIAN_POINT ( 'NONE',  ( -3.152548672688508926E-16, -26.56249999863440436, -5.148502694627439702 ) ) ;
#31361=CARTESIAN_POINT ( 'NONE',  ( 3.535533905932738197, -150.8750000000000000, -3.535533905932738197 ) ) ;
#31363=CARTESIAN_POINT ( 'NONE',  ( -4.458734125000001214, -152.8750000013655779, 1.846868145590734089 ) ) ;
#31365=CARTESIAN_POINT ( 'NONE',  ( 2.229367062499998831, -50.89583333196772941, -3.861377020970580887 ) ) ;
#31368=CARTESIAN_POINT ( 'NONE',  ( 2.500000000000002220, 22.33333333333333215, 4.330127018922192761 ) ) ;
#31369=CARTESIAN_POINT ( 'NONE',  ( 0.000000000000000000, -170.0000000000000000, 5.000000000000000000 ) ) ;
#31370=CARTESIAN_POINT ( 'NONE',  ( 4.458734125000001214, 4.104166668032260823, 2.574251347313718519 ) ) ;
#31371=ADVANCED_FACE ( 'NONE', ( #35549 ), #54531, .T. ) ;
#31372=LINE ( 'NONE', #26239, #15433 ) ;
#31373=ADVANCED_FACE ( 'NONE', ( #40679 ), #55809, .T. ) ;
#31376=CARTESIAN_POINT ( 'NONE',  ( 4.458734124999998549, 13.02083333469892779, -2.574251347313721627 ) ) ;
#31377=( BOUNDED_CURVE ( )  B_SPLINE_CURVE ( 2, ( #36215, #45540, #60990, #11123, #25922, #11755, #46817, #16280, #35898 ),
 .UNSPECIFIED., .F., .F. ) 
 B_SPLINE_CURVE_WITH_KNOTS ( ( 3, 2, 2, 2, 3 ),
 ( 0.8562499999999999556, 0.8569444444444443976, 0.8583333333333332815, 0.8597222222222222765, 0.8604166666666667185 ),
 .UNSPECIFIED. ) 
 CURVE ( )  GEOMETRIC_REPRESENTATION_ITEM ( )  RATIONAL_B_SPLINE_CURVE ( ( 0.9330127018922194093, 0.9330127018922194093, 1.000000000000000000, 0.8660254037844387076, 1.000000000000000000, 0.8660254037844387076, 1.000000000000000000, 0.9330127018922194093, 0.9330127018922194093 ) ) 
 REPRESENTATION_ITEM ( '' )  );
#31378=CARTESIAN_POINT ( 'NONE',  ( -3.535250795749689387E-16, 0.8750000027311874984, -5.773502691896257311 ) ) ;
#31381=ORIENTED_EDGE ( 'NONE', *, *, #61823, .F. ) ;
#31382=CARTESIAN_POINT ( 'NONE',  ( 2.499999999999998668, 27.79166666939785202, -4.330127018922193649 ) ) ;
#31383=CARTESIAN_POINT ( 'NONE',  ( -2.229367062499996610, -41.14583333196773651, 3.861377020970582219 ) ) ;
#31384=CARTESIAN_POINT ( 'NONE',  ( 4.458734124999999437, -164.7500000013656063, 1.846868145590737864 ) ) ;
#31386=CARTESIAN_POINT ( 'NONE',  ( 5.000000000000000000, -43.29166666393548724, -2.886751345948129988 ) ) ;
#31388=CARTESIAN_POINT ( 'NONE',  ( -4.458734124999998549, -19.22916666530106866, 2.574251347313722516 ) ) ;
#31389=ORIENTED_EDGE ( 'NONE', *, *, #2353, .F. ) ;
#31390=CARTESIAN_POINT ( 'NONE',  ( 5.000000000000000888, -88.58333333333332860, 2.886751345948126879 ) ) ;
#31391=CARTESIAN_POINT ( 'NONE',  ( -1.846868145590734756, -164.1250000013656063, -4.458734125000000326 ) ) ;
#31392=CARTESIAN_POINT ( 'NONE',  ( 1.062108568985190270E-13, -28.12499999726880873, -4.999999999999999112 ) ) ;
#31393=ORIENTED_EDGE ( 'NONE', *, *, #52689, .F. ) ;
#31395=CARTESIAN_POINT ( 'NONE',  ( 4.458734124999998549, -30.97916666530107577, -2.574251347313721627 ) ) ;
#31402=VERTEX_POINT ( 'NONE', #503 ) ;
#31405=CARTESIAN_POINT ( 'NONE',  ( -2.229367062500000163, -82.72916666530106511, -3.861377020970580443 ) ) ;
#31407=CARTESIAN_POINT ( 'NONE',  ( 5.000000000000000000, -143.0000000000000284, 0.000000000000000000 ) ) ;
#31408=CARTESIAN_POINT ( 'NONE',  ( -4.458734124999999437, -142.1875000013656063, -5.460374474430324690E-16 ) ) ;
#31409=CARTESIAN_POINT ( 'NONE',  ( 5.000000000000000888, 24.41666666666666785, 2.886751345948126879 ) ) ;
#31411=CARTESIAN_POINT ( 'NONE',  ( 4.458734124999999437, -45.81249999863440081, -5.460374474430324690E-16 ) ) ;
#31417=LINE ( 'NONE', #7635, #41729 ) ;
#31419=CARTESIAN_POINT ( 'NONE',  ( 4.458734124999998549, -77.97916666530106511, -2.574251347313721627 ) ) ;
#31422=( BOUNDED_CURVE ( )  B_SPLINE_CURVE ( 2, ( #33629, #52933, #53248, #9184, #28796, #39074, #58392, #18210, #48412 ),
 .UNSPECIFIED., .F., .F. ) 
 B_SPLINE_CURVE_WITH_KNOTS ( ( 3, 2, 2, 2, 3 ),
 ( 0.03125000000000000000, 0.03194444444444444198, 0.03333333333333333287, 0.03472222222222222376, 0.03541666666666666574 ),
 .UNSPECIFIED. ) 
 CURVE ( )  GEOMETRIC_REPRESENTATION_ITEM ( )  RATIONAL_B_SPLINE_CURVE ( ( 0.9330127018922194093, 0.9330127018922195203, 1.000000000000000000, 0.8660254037844387076, 1.000000000000000000, 0.8660254037844387076, 1.000000000000000000, 0.9330127018922194093, 0.9330127018922194093 ) ) 
 REPRESENTATION_ITEM ( '' )  );
#31428=FACE_OUTER_BOUND ( 'NONE', #51255, .T. ) ;
#31430=ADVANCED_FACE ( 'NONE', ( #10452 ), #49696, .T. ) ;
#31431=CARTESIAN_POINT ( 'NONE',  ( -3.152548672688508926E-16, 13.18750000136559208, -5.148502694627439702 ) ) ;
#31437=CARTESIAN_POINT ( 'NONE',  ( -1.339745962155610925, -15.66965819600733134, 5.000000000000000000 ) ) ;
#31438=CARTESIAN_POINT ( 'NONE',  ( -2.229367062500000163, -84.47916666530107932, -3.861377020970580443 ) ) ;
#31439=CARTESIAN_POINT ( 'NONE',  ( 2.229367062499998831, -5.645833331967740953, -3.861377020970580887 ) ) ;
#31441=CARTESIAN_POINT ( 'NONE',  ( 4.458734124999998549, -36.97916666530107221, -2.574251347313721627 ) ) ;
#31446=AXIS2_PLACEMENT_3D ( 'NONE', #50184, #45043, #35719 ) ;
#31447=AXIS2_PLACEMENT_3D ( 'NONE', #48425, #13394, #33017 ) ;
#31448=CARTESIAN_POINT ( 'NONE',  ( -3.152548672688508926E-16, 22.43750000136559208, -5.148502694627439702 ) ) ;
#31450=EDGE_CURVE ( 'NONE', #49754, #18888, #44870, .T. ) ;
#31451=CARTESIAN_POINT ( 'NONE',  ( -1.339745962155610925, -25.66965819600733312, 5.000000000000000000 ) ) ;
#31452=CARTESIAN_POINT ( 'NONE',  ( 4.458734124999998549, -75.97916666530106511, -2.574251347313721627 ) ) ;
#31454=CARTESIAN_POINT ( 'NONE',  ( 0.000000000000000000, -170.0000000000000000, 0.000000000000000000 ) ) ;
#31455=CARTESIAN_POINT ( 'NONE',  ( -2.500000000000000444, 18.95833333606451632, -4.330127018922193649 ) ) ;
#31457=CYLINDRICAL_SURFACE ( 'NONE', #52036, 5.000000000000000000 ) ;
#31459=CARTESIAN_POINT ( 'NONE',  ( -5.000000000000000888, -149.4375000000000000, 2.071067811865474617 ) ) ;
#31460=CARTESIAN_POINT ( 'NONE',  ( -3.535250795749689387E-16, -23.25000000000000000, -5.773502691896257311 ) ) ;
#31461=CARTESIAN_POINT ( 'NONE',  ( 4.458734124999999437, -26.81249999863440081, -5.460374474430324690E-16 ) ) ;
#31463=CARTESIAN_POINT ( 'NONE',  ( -2.500000000000000444, -26.04166666393547658, -4.330127018922193649 ) ) ;
#31464=CARTESIAN_POINT ( 'NONE',  ( 4.458734125000001214, -54.89583333196773651, 2.574251347313718519 ) ) ;
#31468=CARTESIAN_POINT ( 'NONE',  ( -3.152548672688508926E-16, -3.812499998634408360, -5.148502694627439702 ) ) ;
#31470=CARTESIAN_POINT ( 'NONE',  ( 5.000000000000000888, -71.58333333333332860, 2.886751345948126879 ) ) ;
#31474=CARTESIAN_POINT ( 'NONE',  ( -2.499999999999996447, -70.70833333060214443, 4.330127018922195425 ) ) ;
#31477=CARTESIAN_POINT ( 'NONE',  ( -4.458734124999998549, -18.47916666530106866, 2.574251347313722516 ) ) ;
#31478=CARTESIAN_POINT ( 'NONE',  ( -4.458734124999999437, -53.56249999863439371, 0.000000000000000000 ) ) ;
#31480=CARTESIAN_POINT ( 'NONE',  ( 4.458734124999999437, -139.4375000013656063, 0.000000000000000000 ) ) ;
#31483=ORIENTED_EDGE ( 'NONE', *, *, #40513, .T. ) ;
#31485=CARTESIAN_POINT ( 'NONE',  ( 4.458734124999998549, 24.02083333469892423, -2.574251347313721627 ) ) ;
#31487=CARTESIAN_POINT ( 'NONE',  ( 5.000000000000000888, -50.58333333333332860, 2.886751345948126879 ) ) ;
#31492=CARTESIAN_POINT ( 'NONE',  ( 4.458734124999999437, -147.6875000013656063, 0.000000000000000000 ) ) ;
#31495=CARTESIAN_POINT ( 'NONE',  ( -4.458734124999999437, -64.64583333196772230, -2.574251347313719407 ) ) ;
#31496=FACE_OUTER_BOUND ( 'NONE', #565, .T. ) ;
#31497=CARTESIAN_POINT ( 'NONE',  ( -3.152548672688508926E-16, -9.562499998634406140, -5.148502694627439702 ) ) ;
#31499=CARTESIAN_POINT ( 'NONE',  ( 4.458734124999997661, -144.5000000013656063, 1.846868145590737864 ) ) ;
#31502=CARTESIAN_POINT ( 'NONE',  ( -5.000000000000000888, -164.5625000027312126, 2.071067811865474617 ) ) ;
#31503=CARTESIAN_POINT ( 'NONE',  ( -6.972266317189433020E-16, -8.249999999999998224, -5.000000000000000000 ) ) ;
#31506=CARTESIAN_POINT ( 'NONE',  ( 9.457646018065525792E-16, 28.68750000136559208, 5.148502694627439702 ) ) ;
#31507=CARTESIAN_POINT ( 'NONE',  ( -1.339745962155610925, -5.794658198738521726, 5.000000000000000000 ) ) ;
#31515=CARTESIAN_POINT ( 'NONE',  ( 2.499999999999998668, -56.20833333060214443, -4.330127018922193649 ) ) ;
#31516=CARTESIAN_POINT ( 'NONE',  ( 0.000000000000000000, -170.0000000000000000, 0.000000000000000000 ) ) ;
#31518=CARTESIAN_POINT ( 'NONE',  ( 4.458734124999999437, 14.18750000136559386, -5.460374474430324690E-16 ) ) ;
#31520=CARTESIAN_POINT ( 'NONE',  ( 2.229367062499998831, -11.89583333196774007, -3.861377020970580887 ) ) ;
#31523=CARTESIAN_POINT ( 'NONE',  ( -4.458734125000001214, -159.8750000013655779, 1.846868145590734089 ) ) ;
#31524=CARTESIAN_POINT ( 'NONE',  ( -1.339745962155610925, -37.79465819873851729, 5.000000000000000000 ) ) ;
#31528=EDGE_CURVE ( 'NONE', #2792, #61933, #11050, .T. ) ;
#31530=CARTESIAN_POINT ( 'NONE',  ( -4.999999999999998224, -27.91666666666666430, 2.886751345948131764 ) ) ;
#31532=CARTESIAN_POINT ( 'NONE',  ( 2.229367062500001939, -33.97916666530107221, 3.861377020970579999 ) ) ;
#31537=CARTESIAN_POINT ( 'NONE',  ( 5.000000000000000000, -36.37499999726881583, -6.123233995736766282E-16 ) ) ;
#31538=ORIENTED_EDGE ( 'NONE', *, *, #22841, .F. ) ;
#31542=DIRECTION ( 'NONE',  ( 0.000000000000000000, 0.000000000000000000, 1.000000000000000000 ) ) ;
#31543=EDGE_CURVE ( 'NONE', #60982, #43179, #34770, .T. ) ;
#31544=CARTESIAN_POINT ( 'NONE',  ( 2.499999999999998668, -8.333333333333332149, -4.330127018922193649 ) ) ;
#31546=( GEOMETRIC_REPRESENTATION_CONTEXT ( 3 ) GLOBAL_UNCERTAINTY_ASSIGNED_CONTEXT ( ( #38183 ) ) GLOBAL_UNIT_ASSIGNED_CONTEXT ( ( #22932, #61856, #57027 ) ) REPRESENTATION_CONTEXT ( 'NONE', 'WORKASPACE' ) );
#31547=CARTESIAN_POINT ( 'NONE',  ( -2.229367062500000163, -74.47916666530106511, -3.861377020970580443 ) ) ;
#31548=VECTOR ( 'NONE', #4595, 1000.000000000000000 ) ;
#31549=CARTESIAN_POINT ( 'NONE',  ( -2.500000000000000444, -17.16666666666666430, -4.330127018922193649 ) ) ;
#31550=CARTESIAN_POINT ( 'NONE',  ( 1.060575238724906964E-15, -7.624999997268813168, 5.773502691896257311 ) ) ;
#31551=CARTESIAN_POINT ( 'NONE',  ( 4.458734124999999437, -38.81249999863440081, -5.460374474430324690E-16 ) ) ;
#31552=ORIENTED_EDGE ( 'NONE', *, *, #44054, .F. ) ;
#31553=CLOSED_SHELL ( 'NONE', ( #35762, #39545, #12175, #17728, #14684, #30011, #47212, #34532, #63119, #42319, #51670, #3665, #36257, #40034, #41635, #37865, #16217, #35465, #43693, #1621, #44523, #48290, #54832, #5607, #59711, #20849, #36707, #47231, #23265, #29197, #61013, #15398, #14516, #40893, #11834, #10526, #41959, #28691, #57764, #34137, #43556, #30263, #45982, #51573, #40818, #19316, #41286, #53516, #24397, #35095, #47634, #53878, #40008, #40588, #53373, #23624, #23205, #27701, #43367, #53541, #43724, #52997, #47479, #47558, #39276, #32693, #42793, #44834, #5981, #9933, #26028, #46787, #3675, #4442, #31350, #28029, #17032, #40180, #59508, #3575, #31077, #43730, #4, #30267, #41760, #33154, #24053, #7102, #12997, #21930, #47057, #40256, #42006, #22084, #17026, #12969, #43560, #47908, #23627, #33505, #7792, #15399, #5531, #63326, #2872, #9012, #47163, #3510, #31373, #6798, #19688, #53163, #59877, #62280, #50401, #29818, #8381, #46121, #31430, #15837, #24030, #44902, #52723, #9019, #36187, #18720, #60685, #5859, #20642, #9279, #45313, #45539, #22473, #55462, #4021, #22555, #57471, #61126, #36088, #38642, #32174, #12221, #9045, #23899, #30552, #35096, #52742, #55231, #43278, #12043, #51588, #53964, #55850, #49973, #39991, #28234, #38554, #14527, #55341, #25576, #14601, #62843, #57104, #61851, #61316, #24333, #17997, #46841, #60581, #62256, #24490, #41241, #34179, #6656, #19766, #2852, #40844, #6796, #7596, #57429, #49619, #20116, #12155, #48701, #30869, #20800, #33134, #23184, #31371, #8, #20588, #549, #5960, #7602, #59032, #29388, #907, #19453, #32234, #45788, #62175, #42779, #52230, #28947, #22908, #42443, #20592, #20511, #25557, #45679, #29846, #52696, #61380, #61680, #23247, #51522, #55126, #1187, #58614, #2067, #2623, #34974, #62627, #7441, #52032, #26836, #17729, #29205, #2773, #39797, #50845, #52380, #38906, #58690, #17670, #22906, #46864, #44268, #45696, #62863, #62190, #58265, #25290, #36107, #46430, #24852, #61711, #60604, #60687, #7067, #45710, #2489, #44864, #39638, #63645, #4290, #20112, #9793, #45882, #35010, #366, #41982, #4781, #5150, #54327, #17002, #10776, #32349, #26019, #8562, #26683, #50442, #62988, #38297, #45158, #44866, #48645, #6783, #27261, #56663, #46068, #32259, #11579, #3586, #474, #57666, #58385, #30232, #55602, #49060, #26772, #14148, #26331, #58445, #11928, #49257, #16637, #28060, #19772, #56957, #36105, #51948, #2083, #37430, #19142, #10561, #41275, #52738, #12640, #30656, #38065, #20501, #25299, #7494 ) ) ;
#31556=CARTESIAN_POINT ( 'NONE',  ( -4.458734124999998549, 13.52083333469892779, 2.574251347313722516 ) ) ;
#31558=DIRECTION ( 'NONE',  ( 0.000000000000000000, 0.000000000000000000, 1.000000000000000000 ) ) ;
#31559=CARTESIAN_POINT ( 'NONE',  ( -3.535250795749689387E-16, -54.24999999999999289, -5.773502691896257311 ) ) ;
#31560=CARTESIAN_POINT ( 'NONE',  ( -4.458734125000001214, -160.1250000013655779, 1.846868145590734089 ) ) ;
#31563=CARTESIAN_POINT ( 'NONE',  ( 4.458734125000001214, -73.89583333196773651, 2.574251347313718519 ) ) ;
#31564=CARTESIAN_POINT ( 'NONE',  ( -1.846868145590737420, -141.0000000013656063, 4.458734124999999437 ) ) ;
#31565=CARTESIAN_POINT ( 'NONE',  ( -4.458734124999999437, -85.31249999863439371, 0.000000000000000000 ) ) ;
#31567=CARTESIAN_POINT ( 'NONE',  ( 9.457646018065525792E-16, -34.31249999863440792, 5.148502694627439702 ) ) ;
#31569=ORIENTED_EDGE ( 'NONE', *, *, #4672, .F. ) ;
#31571=CARTESIAN_POINT ( 'NONE',  ( 1.339745962155612702, -84.29465819873850307, -5.000000000000000000 ) ) ;
#31574=DIRECTION ( 'NONE',  ( -0.000000000000000000, 1.000000000000000000, -0.000000000000000000 ) ) ;
#31575=CARTESIAN_POINT ( 'NONE',  ( -4.458734124999999437, -62.56249999863440792, 0.000000000000000000 ) ) ;
#31577=ORIENTED_EDGE ( 'NONE', *, *, #4033, .T. ) ;
#31583=CARTESIAN_POINT ( 'NONE',  ( -4.458734124999999437, 9.687500001365593860, 0.000000000000000000 ) ) ;
#31584=DIRECTION ( 'NONE',  ( -0.000000000000000000, 1.000000000000000000, -0.000000000000000000 ) ) ;
#31585=CARTESIAN_POINT ( 'NONE',  ( 3.152801135295367541, -158.3125000013656063, -3.152801135295367541 ) ) ;
#31586=( BOUNDED_CURVE ( )  B_SPLINE_CURVE ( 2, ( #28360, #47364, #52512, #41891, #8132, #7500, #62163, #51561, #13260 ),
 .UNSPECIFIED., .F., .F. ) 
 B_SPLINE_CURVE_WITH_KNOTS ( ( 3, 2, 2, 2, 3 ),
 ( 0.7416666666666664742, 0.7458333333333331261, 0.7499999999999997780, 0.7541666666666664298, 0.7583333333333330817 ),
 .UNSPECIFIED. ) 
 CURVE ( )  GEOMETRIC_REPRESENTATION_ITEM ( )  RATIONAL_B_SPLINE_CURVE ( ( 1.000000000000003997, 0.9238795325112826307, 1.000000000000000000, 0.9238795325112867385, 1.000000000000000000, 0.9238795325112867385, 1.000000000000000000, 0.9238795325112908463, 0.9999999999999958922 ) ) 
 REPRESENTATION_ITEM ( '' )  );
#31588=ORIENTED_EDGE ( 'NONE', *, *, #9380, .T. ) ;
#31590=FACE_OUTER_BOUND ( 'NONE', #46726, .T. ) ;
#31593=CARTESIAN_POINT ( 'NONE',  ( 2.499999999999998668, -71.20833333060214443, -4.330127018922193649 ) ) ;
#31596=CARTESIAN_POINT ( 'NONE',  ( -6.972266317189433020E-16, -73.12499999726878741, -5.000000000000000000 ) ) ;
#31599=CARTESIAN_POINT ( 'NONE',  ( 9.457646018065525792E-16, 27.93750000136559208, 5.148502694627439702 ) ) ;
#31602=CARTESIAN_POINT ( 'NONE',  ( 4.458734125000000326, -0.1458333319677394824, 2.574251347313718519 ) ) ;
#31603=CARTESIAN_POINT ( 'NONE',  ( 5.000000000000000000, -0.3749999972688135008, -6.123233995736766282E-16 ) ) ;
#31605=CARTESIAN_POINT ( 'NONE',  ( 3.061616997868383141E-16, -145.8750000027312126, -5.000000000000000000 ) ) ;
#31606=CARTESIAN_POINT ( 'NONE',  ( 1.339745962155612702, -75.16965819600731891, -5.000000000000000000 ) ) ;
#31610=DIRECTION ( 'NONE',  ( -0.000000000000000000, 1.000000000000000000, -0.000000000000000000 ) ) ;
#31613=CARTESIAN_POINT ( 'NONE',  ( 4.458734124999999437, -162.6875000013655779, 0.000000000000000000 ) ) ;
#31616=CARTESIAN_POINT ( 'NONE',  ( -4.999999999999998224, -90.79166666393547303, 2.886751345948131764 ) ) ;
#31619=CARTESIAN_POINT ( 'NONE',  ( 2.229367062500001939, 21.77083333469892779, 3.861377020970579999 ) ) ;
#31625=CARTESIAN_POINT ( 'NONE',  ( 2.499999999999998668, 7.666666666666665186, -4.330127018922193649 ) ) ;
#31626=CARTESIAN_POINT ( 'NONE',  ( 4.458734124999999437, -58.81249999863440081, -5.460374474430324690E-16 ) ) ;
#31630=DIRECTION ( 'NONE',  ( 0.000000000000000000, 0.000000000000000000, 1.000000000000000000 ) ) ;
#31633=CARTESIAN_POINT ( 'NONE',  ( -2.499999999999996447, -37.83333333333332860, 4.330127018922195425 ) ) ;
#31634=CARTESIAN_POINT ( 'NONE',  ( -2.499999999999996447, -44.83333333333333570, 4.330127018922195425 ) ) ;
#31637=CARTESIAN_POINT ( 'NONE',  ( 0.000000000000000000, -170.0000000000000000, 5.000000000000000000 ) ) ;
#31638=CARTESIAN_POINT ( 'NONE',  ( 2.229367062499998831, -58.64583333196773651, -3.861377020970580887 ) ) ;
#31639=( BOUNDED_CURVE ( )  B_SPLINE_CURVE ( 2, ( #58872, #9662, #35, #19634, #39245, #14802, #34415, #1005, #40526 ),
 .UNSPECIFIED., .F., .F. ) 
 B_SPLINE_CURVE_WITH_KNOTS ( ( 3, 2, 2, 2, 3 ),
 ( 0.002083333333333333738, 0.002777777777777777884, 0.004166666666666666609, 0.005555555555555555768, 0.006250000000000000347 ),
 .UNSPECIFIED. ) 
 CURVE ( )  GEOMETRIC_REPRESENTATION_ITEM ( )  RATIONAL_B_SPLINE_CURVE ( ( 0.9330127018922194093, 0.9330127018922194093, 1.000000000000000000, 0.8660254037844387076, 1.000000000000000000, 0.8660254037844387076, 1.000000000000000000, 0.9330127018922192983, 0.9330127018922194093 ) ) 
 REPRESENTATION_ITEM ( '' )  );
#31640=CARTESIAN_POINT ( 'NONE',  ( -3.152801135295367096, -153.3125000013656063, -3.152801135295367541 ) ) ;
#31641=CARTESIAN_POINT ( 'NONE',  ( -4.458734124999999437, -70.39583333196773651, -2.574251347313719407 ) ) ;
#31644=CARTESIAN_POINT ( 'NONE',  ( 2.229367062500001939, -19.22916666530106866, 3.861377020970579999 ) ) ;
#31645=CARTESIAN_POINT ( 'NONE',  ( 5.000000000000000888, -63.45833333060215153, 2.886751345948126879 ) ) ;
#31646=ORIENTED_EDGE ( 'NONE', *, *, #8635, .F. ) ;
#31650=DIRECTION ( 'NONE',  ( 0.000000000000000000, 0.000000000000000000, 1.000000000000000000 ) ) ;
#31652=CARTESIAN_POINT ( 'NONE',  ( 3.152801135295366208, -151.5625000013655779, 3.152801135295367985 ) ) ;
#31656=CARTESIAN_POINT ( 'NONE',  ( -2.229367062499996610, -49.39583333196772941, 3.861377020970582219 ) ) ;
#31658=CARTESIAN_POINT ( 'NONE',  ( 2.499999999999998668, 10.79166666939785202, -4.330127018922193649 ) ) ;
#31660=CARTESIAN_POINT ( 'NONE',  ( 9.457646018065525792E-16, 23.93750000136559564, 5.148502694627439702 ) ) ;
#31663=CARTESIAN_POINT ( 'NONE',  ( 1.846868145590736310, -168.6250000013656063, 4.458734124999997661 ) ) ;
#31664=VERTEX_POINT ( 'NONE', #119 ) ;
#31669=CARTESIAN_POINT ( 'NONE',  ( 2.071067811865348940, -156.9375000027312410, -5.000000000000127898 ) ) ;
#31674=CARTESIAN_POINT ( 'NONE',  ( -2.499999999999996447, 19.16666666666666430, 4.330127018922195425 ) ) ;
#31679=CARTESIAN_POINT ( 'NONE',  ( 3.535533905932738197, -159.0000000027312126, -3.535533905932738197 ) ) ;
#31680=VERTEX_POINT ( 'NONE', #8806 ) ;
#31686=CARTESIAN_POINT ( 'NONE',  ( 5.000000000000000000, -149.0000000000000284, 0.000000000000000000 ) ) ;
#31690=CARTESIAN_POINT ( 'NONE',  ( 2.229367062499998831, -27.64583333196774007, -3.861377020970580887 ) ) ;
#31691=CARTESIAN_POINT ( 'NONE',  ( 5.000000000000000888, 14.41666666666666430, 2.886751345948126879 ) ) ;
#31692=CARTESIAN_POINT ( 'NONE',  ( 3.061616997868383141E-16, -152.7500000000000000, -5.000000000000000000 ) ) ;
#31694=CARTESIAN_POINT ( 'NONE',  ( 3.152801135295366208, -150.5625000013655779, 3.152801135295367985 ) ) ;
#31697=CARTESIAN_POINT ( 'NONE',  ( 9.457646018065525792E-16, -50.31249999863440792, 5.148502694627439702 ) ) ;
#31700=CARTESIAN_POINT ( 'NONE',  ( -3.535250795749689387E-16, 26.75000000000000000, -5.773502691896257311 ) ) ;
#31701=AXIS2_PLACEMENT_3D ( 'NONE', #5640, #59679, #25253 ) ;
#31702=FACE_OUTER_BOUND ( 'NONE', #33163, .T. ) ;
#31703=CARTESIAN_POINT ( 'NONE',  ( 9.457646018065525792E-16, 5.937500001365592972, 5.148502694627439702 ) ) ;
#31704=CARTESIAN_POINT ( 'NONE',  ( 2.499999999999998668, 19.66666666666666430, -4.330127018922193649 ) ) ;
#31707=CARTESIAN_POINT ( 'NONE',  ( -3.152548672688508926E-16, 16.18750000136559564, -5.148502694627439702 ) ) ;
#31708=CARTESIAN_POINT ( 'NONE',  ( 1.060575238724906964E-15, 3.375000002731186388, 5.773502691896257311 ) ) ;
#31709=EDGE_LOOP ( 'NONE', ( #37661, #16860, #48194, #44399 ) ) ;
#31711=ORIENTED_EDGE ( 'NONE', *, *, #35445, .F. ) ;
#31713=CARTESIAN_POINT ( 'NONE',  ( -4.458734124999999437, -43.39583333196774362, -2.574251347313719407 ) ) ;
#31714=CARTESIAN_POINT ( 'NONE',  ( 1.846868145590736310, -163.8750000013655779, 4.458734124999999437 ) ) ;
#31716=CARTESIAN_POINT ( 'NONE',  ( 2.499999999999998668, -47.20833333060214443, -4.330127018922193649 ) ) ;
#31718=CARTESIAN_POINT ( 'NONE',  ( -3.152548672688508926E-16, -16.56249999863440792, -5.148502694627439702 ) ) ;
#31720=CARTESIAN_POINT ( 'NONE',  ( 1.060575238724906964E-15, -86.75000000000000000, 5.773502691896257311 ) ) ;
#31721=CARTESIAN_POINT ( 'NONE',  ( -3.152801135295367096, -166.0625000013656063, -3.152801135295367541 ) ) ;
#31723=CARTESIAN_POINT ( 'NONE',  ( 2.499999999999998668, -20.20833333060214798, -4.330127018922193649 ) ) ;
#31724=ORIENTED_EDGE ( 'NONE', *, *, #23697, .T. ) ;
#31726=EDGE_CURVE ( 'NONE', #16689, #23906, #58643, .T. ) ;
#31728=CARTESIAN_POINT ( 'NONE',  ( -4.458734124999998549, -33.47916666530107221, 2.574251347313722516 ) ) ;
#31733=CARTESIAN_POINT ( 'NONE',  ( -5.000000000000000000, -28.87499999726881228, 0.000000000000000000 ) ) ;
#31734=ORIENTED_EDGE ( 'NONE', *, *, #48070, .T. ) ;
#31737=CARTESIAN_POINT ( 'NONE',  ( -2.229367062499996610, -80.39583333196773651, 3.861377020970582219 ) ) ;
#31739=CARTESIAN_POINT ( 'NONE',  ( 3.152801135295367541, -143.5625000013655779, -3.152801135295367541 ) ) ;
#31740=CARTESIAN_POINT ( 'NONE',  ( 1.339745962155615144, -84.58034179853028434, 4.999999999999999112 ) ) ;
#31742=CARTESIAN_POINT ( 'NONE',  ( -4.458734124999999437, -44.39583333196774362, -2.574251347313719407 ) ) ;
#31746=CARTESIAN_POINT ( 'NONE',  ( 3.535533905932736864, -154.2500000027312126, 3.535533905932738641 ) ) ;
#31750=CARTESIAN_POINT ( 'NONE',  ( 4.458734124999999437, -79.06249999863440792, -5.460374474430324690E-16 ) ) ;
#31755=CARTESIAN_POINT ( 'NONE',  ( -5.000000000000000000, -14.95833333060214621, -2.886751345948128211 ) ) ;
#31757=CARTESIAN_POINT ( 'NONE',  ( 3.535533905932736864, -168.2500000027312126, 3.535533905932738641 ) ) ;
#31759=CARTESIAN_POINT ( 'NONE',  ( -2.229367062499996610, 13.60416666803226171, 3.861377020970582219 ) ) ;
#31767=CARTESIAN_POINT ( 'NONE',  ( -4.458734124999998549, -83.22916666530106511, 2.574251347313722516 ) ) ;
#31768=CARTESIAN_POINT ( 'NONE',  ( 9.457646018065525792E-16, -9.062499998634407916, 5.148502694627439702 ) ) ;
#31770=CARTESIAN_POINT ( 'NONE',  ( 2.229367062500001939, -36.22916666530107221, 3.861377020970579999 ) ) ;
#31775=CARTESIAN_POINT ( 'NONE',  ( 1.846868145590735200, -149.5000000013656063, -4.458734124999999437 ) ) ;
#31776=CARTESIAN_POINT ( 'NONE',  ( -4.458734124999999437, 19.68750000136559208, 0.000000000000000000 ) ) ;
#31777=DIRECTION ( 'NONE',  ( -0.000000000000000000, 1.000000000000000000, -0.000000000000000000 ) ) ;
#31778=CYLINDRICAL_SURFACE ( 'NONE', #48104, 5.000000000000000000 ) ;
#31779=CARTESIAN_POINT ( 'NONE',  ( -2.229367062499996610, -81.39583333196773651, 3.861377020970582219 ) ) ;
#31781=CARTESIAN_POINT ( 'NONE',  ( -6.972266317189433020E-16, -72.12499999726878741, -5.000000000000000000 ) ) ;
#31782=CARTESIAN_POINT ( 'NONE',  ( 1.060575238724906964E-15, 19.37500000273118772, 5.773502691896257311 ) ) ;
#31785=DIRECTION ( 'NONE',  ( 0.000000000000000000, 0.000000000000000000, 1.000000000000000000 ) ) ;
#31787=CARTESIAN_POINT ( 'NONE',  ( -4.999999999999999112, -21.91666666666666785, 2.886751345948131764 ) ) ;
#31788=CARTESIAN_POINT ( 'NONE',  ( 2.229367062500001939, -25.97916666530106866, 3.861377020970579999 ) ) ;
#31789=CARTESIAN_POINT ( 'NONE',  ( 2.229367062499998831, -89.64583333196773651, -3.861377020970580887 ) ) ;
#31790=CARTESIAN_POINT ( 'NONE',  ( -3.535250795749689387E-16, -28.12499999726880873, -5.773502691896257311 ) ) ;
#31791=CARTESIAN_POINT ( 'NONE',  ( -3.152548672688508926E-16, -55.56249999863440081, -5.148502694627439702 ) ) ;
#31792=ORIENTED_EDGE ( 'NONE', *, *, #45714, .F. ) ;
#31794=CARTESIAN_POINT ( 'NONE',  ( 4.458734125000001214, -1.145833331967740509, 2.574251347313718519 ) ) ;
#31796=CARTESIAN_POINT ( 'NONE',  ( -3.535250795749689387E-16, -70.25000000000000000, -5.773502691896257311 ) ) ;
#31800=CARTESIAN_POINT ( 'NONE',  ( -4.999999999999999112, -74.79166666393547303, 2.886751345948131764 ) ) ;
#31801=CARTESIAN_POINT ( 'NONE',  ( -2.500000000000000444, -54.04166666393548013, -4.330127018922193649 ) ) ;
#31803=EDGE_CURVE ( 'NONE', #25841, #1596, #52563, .T. ) ;
#31804=CARTESIAN_POINT ( 'NONE',  ( -4.458734124999999437, -18.56249999863440792, 0.000000000000000000 ) ) ;
#31805=CARTESIAN_POINT ( 'NONE',  ( 2.229367062499998831, -49.89583333196772941, -3.861377020970580887 ) ) ;
#31806=CARTESIAN_POINT ( 'NONE',  ( 2.499999999999998668, 10.66666666666666430, -4.330127018922193649 ) ) ;
#31807=SURFACE_STYLE_USAGE ( .BOTH. , #47244 ) ;
#31808=CARTESIAN_POINT ( 'NONE',  ( -3.152801135295367096, -141.0625000013655779, -3.152801135295367541 ) ) ;
#31810=CARTESIAN_POINT ( 'NONE',  ( 2.071067811865644703, -147.9375000027312126, -4.999999999999831246 ) ) ;
#31815=( BOUNDED_CURVE ( )  B_SPLINE_CURVE ( 2, ( #40909, #46385, #2642, #37054, #32211, #6834, #51840, #60554, #36096 ),
 .UNSPECIFIED., .F., .F. ) 
 B_SPLINE_CURVE_WITH_KNOTS ( ( 3, 2, 2, 2, 3 ),
 ( 0.5145833333333332815, 0.5152777777777777235, 0.5166666666666667185, 0.5180555555555556024, 0.5187500000000000444 ),
 .UNSPECIFIED. ) 
 CURVE ( )  GEOMETRIC_REPRESENTATION_ITEM ( )  RATIONAL_B_SPLINE_CURVE ( ( 0.9330127018922194093, 0.9330127018922194093, 1.000000000000000000, 0.8660254037844387076, 1.000000000000000000, 0.8660254037844387076, 1.000000000000000000, 0.9330127018922194093, 0.9330127018922194093 ) ) 
 REPRESENTATION_ITEM ( '' )  );
#31817=CARTESIAN_POINT ( 'NONE',  ( 2.499999999999998668, -50.33333333333332860, -4.330127018922193649 ) ) ;
#31818=VECTOR ( 'NONE', #4397, 1000.000000000000000 ) ;
#31821=CARTESIAN_POINT ( 'NONE',  ( -1.846868145590737420, -147.0000000013655779, 4.458734124999999437 ) ) ;
#31826=CARTESIAN_POINT ( 'NONE',  ( -4.458734124999998549, -62.47916666530106511, 2.574251347313722516 ) ) ;
#31829=CARTESIAN_POINT ( 'NONE',  ( 1.846868145590735200, -146.2500000013656347, -4.458734124999999437 ) ) ;
#31842=DIRECTION ( 'NONE',  ( -0.000000000000000000, 1.000000000000000000, -0.000000000000000000 ) ) ;
#31844=CARTESIAN_POINT ( 'NONE',  ( -2.229367062500000163, 7.520833334698929562, -3.861377020970580443 ) ) ;
#31846=CARTESIAN_POINT ( 'NONE',  ( 4.458734125000000326, -22.14583333196773296, 2.574251347313718519 ) ) ;
#31848=CARTESIAN_POINT ( 'NONE',  ( 4.458734124999999437, -161.5000000013656063, 1.846868145590737864 ) ) ;
#31849=CARTESIAN_POINT ( 'NONE',  ( 0.000000000000000000, -170.0000000000000000, 5.000000000000000000 ) ) ;
#31852=CARTESIAN_POINT ( 'NONE',  ( -3.152548672688508926E-16, -37.56249999863440792, -5.148502694627439702 ) ) ;
#31853=EDGE_CURVE ( 'NONE', #34317, #25633, #8983, .T. ) ;
#31854=CARTESIAN_POINT ( 'NONE',  ( 2.500000000000002220, -51.54166666393547303, 4.330127018922192761 ) ) ;
#31855=CARTESIAN_POINT ( 'NONE',  ( 4.458734124999998549, -67.97916666530106511, -2.574251347313721627 ) ) ;
#31858=CARTESIAN_POINT ( 'NONE',  ( 5.000000000000000000, -68.37499999726881583, -6.123233995736766282E-16 ) ) ;
#31859=ORIENTED_EDGE ( 'NONE', *, *, #22115, .T. ) ;
#31862=CARTESIAN_POINT ( 'NONE',  ( 5.000000000000000888, -144.0625000027311273, -2.071067811865475505 ) ) ;
#31863=CARTESIAN_POINT ( 'NONE',  ( -2.500000000000000444, -10.16666666666666430, -4.330127018922193649 ) ) ;
#31865=CARTESIAN_POINT ( 'NONE',  ( 2.229367062500001939, -69.97916666530107932, 3.861377020970579999 ) ) ;
#31867=CARTESIAN_POINT ( 'NONE',  ( 2.499999999999998668, -11.20833333060214798, -4.330127018922193649 ) ) ;
#31868=CARTESIAN_POINT ( 'NONE',  ( 9.457646018065525792E-16, -41.06249999863440792, 5.148502694627439702 ) ) ;
#31869=ORIENTED_EDGE ( 'NONE', *, *, #6302, .F. ) ;
#31871=CARTESIAN_POINT ( 'NONE',  ( 2.229367062500001939, 10.77083333469892956, 3.861377020970579999 ) ) ;
#31874=CARTESIAN_POINT ( 'NONE',  ( -2.500000000000000444, -55.16666666666667140, -4.330127018922193649 ) ) ;
#31875=CARTESIAN_POINT ( 'NONE',  ( -1.846868145590737420, -161.0000000013656063, 4.458734124999999437 ) ) ;
#31878=CARTESIAN_POINT ( 'NONE',  ( 2.229367062499998831, -80.64583333196773651, -3.861377020970580887 ) ) ;
#31879=CARTESIAN_POINT ( 'NONE',  ( 2.071067811865476394, -169.1875000000000000, 5.000000000000000000 ) ) ;
#31880=CARTESIAN_POINT ( 'NONE',  ( 4.458734124999999437, -86.81249999863439371, -5.460374474430324690E-16 ) ) ;
#31882=CARTESIAN_POINT ( 'NONE',  ( -2.229367062500000163, 0.2708333346989263979, -3.861377020970580443 ) ) ;
#31883=CARTESIAN_POINT ( 'NONE',  ( -2.229367062500000163, -36.72916666530107221, -3.861377020970580443 ) ) ;
#31885=EDGE_CURVE ( 'NONE', #9668, #20741, #50887, .T. ) ;
#31886=CARTESIAN_POINT ( 'NONE',  ( -2.499999999999996447, 24.29166666939785202, 4.330127018922195425 ) ) ;
#31889=EDGE_CURVE ( 'NONE', #32568, #30305, #48051, .T. ) ;
#31893=CARTESIAN_POINT ( 'NONE',  ( -4.458734124999999437, -71.64583333196773651, -2.574251347313719407 ) ) ;
#31896=EDGE_CURVE ( 'NONE', #35368, #33079, #24868, .T. ) ;
#31897=( BOUNDED_CURVE ( )  B_SPLINE_CURVE ( 2, ( #30752, #21427, #60676, #10811, #16599, #36217, #15321, #54881, #16282 ),
 .UNSPECIFIED., .F., .F. ) 
 B_SPLINE_CURVE_WITH_KNOTS ( ( 3, 2, 2, 2, 3 ),
 ( 0.3937499999999999889, 0.3944444444444444309, 0.3958333333333333148, 0.3972222222222221988, 0.3979166666666666963 ),
 .UNSPECIFIED. ) 
 CURVE ( )  GEOMETRIC_REPRESENTATION_ITEM ( )  RATIONAL_B_SPLINE_CURVE ( ( 0.9330127018922194093, 0.9330127018922194093, 1.000000000000000000, 0.8660254037844387076, 1.000000000000000000, 0.8660254037844387076, 1.000000000000000000, 0.9330127018922167448, 0.9330127018922194093 ) ) 
 REPRESENTATION_ITEM ( '' )  );
#31898=CARTESIAN_POINT ( 'NONE',  ( 5.000000000000000000, -164.0625000000000000, 2.071067811865478614 ) ) ;
#31900=EDGE_CURVE ( 'NONE', #25633, #5644, #28700, .T. ) ;
#31901=CARTESIAN_POINT ( 'NONE',  ( -4.729367062499999719, 29.84375000068279604, 0.000000000000000000 ) ) ;
#31902=CARTESIAN_POINT ( 'NONE',  ( -2.229367062499996610, 7.854166668032260823, 3.861377020970582219 ) ) ;
#31903=AXIS2_PLACEMENT_3D ( 'NONE', #13415, #46571, #52027 ) ;
#31904=CARTESIAN_POINT ( 'NONE',  ( 1.846868145590735200, -156.2500000013656063, -4.458734124999999437 ) ) ;
#31906=EDGE_LOOP ( 'NONE', ( #49418, #8929, #7685, #11116 ) ) ;
#31908=EDGE_CURVE ( 'NONE', #44350, #45572, #44790, .T. ) ;
#31914=LINE ( 'NONE', #61519, #9057 ) ;
#31917=CARTESIAN_POINT ( 'NONE',  ( 2.229367062499998831, 28.35416666803225993, -3.861377020970580887 ) ) ;
#31920=CARTESIAN_POINT ( 'NONE',  ( -4.458734124999999437, -3.562499998634407916, 0.000000000000000000 ) ) ;
#31921=CARTESIAN_POINT ( 'NONE',  ( 1.339745962155615144, -0.5803417985302927740, 4.999999999999999112 ) ) ;
#31923=CARTESIAN_POINT ( 'NONE',  ( 3.061616997868383141E-16, -141.8750000027312126, -5.000000000000000000 ) ) ;
#31924=CARTESIAN_POINT ( 'NONE',  ( 3.535533905932736864, -159.1250000000000284, 3.535533905932738641 ) ) ;
#31928=CARTESIAN_POINT ( 'NONE',  ( 0.000000000000000000, -170.0000000000000000, 0.000000000000000000 ) ) ;
#31929=CARTESIAN_POINT ( 'NONE',  ( 2.500000000000002220, -22.66666666666666785, 4.330127018922192761 ) ) ;
#31931=CARTESIAN_POINT ( 'NONE',  ( 4.458734124999997661, -159.7500000013656063, 1.846868145590737864 ) ) ;
#31933=CARTESIAN_POINT ( 'NONE',  ( -6.972266317189433020E-16, -57.25000000000000000, -5.000000000000000000 ) ) ;
#31935=CARTESIAN_POINT ( 'NONE',  ( -4.458734124999999437, 18.43750000136559564, 0.000000000000000000 ) ) ;
#31940=CARTESIAN_POINT ( 'NONE',  ( -6.972266317189433020E-16, -16.25000000000000000, -5.000000000000000000 ) ) ;
#31941=CARTESIAN_POINT ( 'NONE',  ( 2.499999999999998668, 10.66666666666666430, -4.330127018922193649 ) ) ;
#31942=CARTESIAN_POINT ( 'NONE',  ( -2.229367062500000163, -56.47916666530107221, -3.861377020970580443 ) ) ;
#31943=LINE ( 'NONE', #42536, #40018 ) ;
#31945=CARTESIAN_POINT ( 'NONE',  ( 5.275681513340003914E-14, 9.875000002731184168, -5.000000000000000000 ) ) ;
#31947=CARTESIAN_POINT ( 'NONE',  ( -3.535533905932738641, -151.5000000027312126, 3.535533905932737309 ) ) ;
#31948=CARTESIAN_POINT ( 'NONE',  ( -3.535250795749689387E-16, -40.24999999999998579, -5.773502691896257311 ) ) ;
#31952=CARTESIAN_POINT ( 'NONE',  ( 9.457646018065525792E-16, -64.06249999863440792, 5.148502694627439702 ) ) ;
#31953=CARTESIAN_POINT ( 'NONE',  ( -4.458734124999999437, -152.1875000013656063, -5.460374474430324690E-16 ) ) ;
#31954=CARTESIAN_POINT ( 'NONE',  ( -4.458734124999999437, -69.31249999863439371, 0.000000000000000000 ) ) ;
#31956=CARTESIAN_POINT ( 'NONE',  ( -4.458734124999999437, -19.64583333196774362, -2.574251347313719407 ) ) ;
#31957=CARTESIAN_POINT ( 'NONE',  ( -3.535250795749689387E-16, -60.12499999726880162, -5.773502691896257311 ) ) ;
#31959=VERTEX_POINT ( 'NONE', #1399 ) ;
#31960=CARTESIAN_POINT ( 'NONE',  ( 0.000000000000000000, -170.0000000000000000, 0.000000000000000000 ) ) ;
#31963=CARTESIAN_POINT ( 'NONE',  ( -6.972266317189433020E-16, -21.12499999726881228, -5.000000000000000000 ) ) ;
#31964=CARTESIAN_POINT ( 'NONE',  ( -4.458734124999999437, -150.9375000013656063, -5.460374474430324690E-16 ) ) ;
#31966=( BOUNDED_CURVE ( )  B_SPLINE_CURVE ( 2, ( #59151, #15083, #9616, #4177, #14123, #4478, #34697, #10260, #29861 ),
 .UNSPECIFIED., .F., .F. ) 
 B_SPLINE_CURVE_WITH_KNOTS ( ( 3, 2, 2, 2, 3 ),
 ( 0.1937500000000000056, 0.1944444444444444475, 0.1958333333333333315, 0.1972222222222222154, 0.1979166666666666574 ),
 .UNSPECIFIED. ) 
 CURVE ( )  GEOMETRIC_REPRESENTATION_ITEM ( )  RATIONAL_B_SPLINE_CURVE ( ( 0.9330127018922194093, 0.9330127018922194093, 1.000000000000000000, 0.8660254037844387076, 1.000000000000000000, 0.8660254037844387076, 1.000000000000000000, 0.9330127018922194093, 0.9330127018922194093 ) ) 
 REPRESENTATION_ITEM ( '' )  );
#31967=CARTESIAN_POINT ( 'NONE',  ( 5.000000000000000000, -155.1250000027311842, 0.000000000000000000 ) ) ;
#31970=CARTESIAN_POINT ( 'NONE',  ( 4.458734125000001214, -47.14583333196774362, 2.574251347313718519 ) ) ;
#31974=EDGE_CURVE ( 'NONE', #49174, #28941, #57096, .T. ) ;
#31975=CARTESIAN_POINT ( 'NONE',  ( -4.458734124999999437, 21.60416666803225993, -2.574251347313719407 ) ) ;
#31978=CARTESIAN_POINT ( 'NONE',  ( 2.730187237215162345E-16, -169.1875000013656063, -4.458734124999999437 ) ) ;
#31984=EDGE_CURVE ( 'NONE', #20487, #38204, #63656, .T. ) ;
#31985=CYLINDRICAL_SURFACE ( 'NONE', #26503, 5.000000000000000000 ) ;
#31995=CARTESIAN_POINT ( 'NONE',  ( 2.071067811865475505, -154.9375000027311842, -5.000000000000000888 ) ) ;
#31996=ORIENTED_EDGE ( 'NONE', *, *, #26751, .F. ) ;
#32002=CARTESIAN_POINT ( 'NONE',  ( 5.000000000000000000, -148.0000000000000284, 0.000000000000000000 ) ) ;
#32006=CARTESIAN_POINT ( 'NONE',  ( -3.152548672688508926E-16, -22.56249999863440436, -5.148502694627439702 ) ) ;
#32010=CARTESIAN_POINT ( 'NONE',  ( 1.846868145590735200, -153.2500000013655779, -4.458734125000000326 ) ) ;
#32011=ORIENTED_EDGE ( 'NONE', *, *, #55941, .F. ) ;
#32012=CARTESIAN_POINT ( 'NONE',  ( -6.972266317189433020E-16, 17.75000000000000355, -5.000000000000000000 ) ) ;
#32013=CARTESIAN_POINT ( 'NONE',  ( 9.457646018065525792E-16, -49.31249999863440792, 5.148502694627439702 ) ) ;
#32014=CARTESIAN_POINT ( 'NONE',  ( 1.339745962155615144, -58.58034179853029855, 4.999999999999999112 ) ) ;
#32016=CARTESIAN_POINT ( 'NONE',  ( 5.000000000000000888, 22.41666666666666785, 2.886751345948126879 ) ) ;
#32018=CARTESIAN_POINT ( 'NONE',  ( -4.458734124999998549, -2.229166665301068662, 2.574251347313722516 ) ) ;
#32020=CARTESIAN_POINT ( 'NONE',  ( -4.458734124999998549, 15.52083333469892779, 2.574251347313722516 ) ) ;
#32021=CARTESIAN_POINT ( 'NONE',  ( 2.499999999999998668, 4.791666669397852907, -4.330127018922193649 ) ) ;
#32023=CARTESIAN_POINT ( 'NONE',  ( 1.975475456537005874E-15, -42.75000000000000000, 5.000000000000000000 ) ) ;
#32024=VERTEX_POINT ( 'NONE', #22596 ) ;
#32025=CARTESIAN_POINT ( 'NONE',  ( 2.500000000000002220, 27.45833333606451632, 4.330127018922192761 ) ) ;
#32026=CARTESIAN_POINT ( 'NONE',  ( -4.458734124999998549, -42.22916666530107932, 2.574251347313722516 ) ) ;
#32027=CARTESIAN_POINT ( 'NONE',  ( -1.846868145590734756, -164.3750000013656063, -4.458734125000000326 ) ) ;
#32028=EDGE_CURVE ( 'NONE', #56895, #9036, #54635, .T. ) ;
#32029=CARTESIAN_POINT ( 'NONE',  ( 5.000000000000000000, -46.29166666393547303, -2.886751345948129988 ) ) ;
#32030=ORIENTED_EDGE ( 'NONE', *, *, #17388, .T. ) ;
#32031=CARTESIAN_POINT ( 'NONE',  ( 9.457646018065525792E-16, -22.06249999863440436, 5.148502694627439702 ) ) ;
#32033=CARTESIAN_POINT ( 'NONE',  ( 2.499999999999998668, -89.33333333333332860, -4.330127018922193649 ) ) ;
#32034=CARTESIAN_POINT ( 'NONE',  ( 4.458734124999999437, -164.5000000013655779, 1.846868145590737864 ) ) ;
#32035=CARTESIAN_POINT ( 'NONE',  ( 2.500000000000002220, -39.54166666393548013, 4.330127018922192761 ) ) ;
#32037=CARTESIAN_POINT ( 'NONE',  ( 2.229367062500001939, -34.22916666530107221, 3.861377020970579999 ) ) ;
#32039=ORIENTED_EDGE ( 'NONE', *, *, #16092, .T. ) ;
#32044=CARTESIAN_POINT ( 'NONE',  ( -2.071067811865496378, -166.8125000027312410, -4.999999999999979572 ) ) ;
#32046=CARTESIAN_POINT ( 'NONE',  ( -4.458734124999998549, -79.47916666530106511, 2.574251347313722516 ) ) ;
#32049=CARTESIAN_POINT ( 'NONE',  ( -5.000000000000000888, -158.6875000027312126, -2.071067811865475949 ) ) ;
#32050=CARTESIAN_POINT ( 'NONE',  ( 2.500000000000002220, 20.33333333333333215, 4.330127018922192761 ) ) ;
#32052=CARTESIAN_POINT ( 'NONE',  ( 4.458734125000000326, -47.89583333196774362, 2.574251347313718519 ) ) ;
#32055=CARTESIAN_POINT ( 'NONE',  ( 3.061616997868383141E-16, -153.8750000027311842, -5.000000000000000000 ) ) ;
#32058=CARTESIAN_POINT ( 'NONE',  ( 0.000000000000000000, -170.0000000000000000, 0.000000000000000000 ) ) ;
#32060=CARTESIAN_POINT ( 'NONE',  ( 2.229367062499998831, -78.89583333196773651, -3.861377020970580887 ) ) ;
#32064=ORIENTED_EDGE ( 'NONE', *, *, #55598, .T. ) ;
#32065=CARTESIAN_POINT ( 'NONE',  ( -1.510657702057710340E-15, 28.25000000000000000, 5.000000000000000000 ) ) ;
#32067=CARTESIAN_POINT ( 'NONE',  ( -5.000000000000000000, -5.083333333333334814, -2.886751345948128211 ) ) ;
#32069=CARTESIAN_POINT ( 'NONE',  ( -4.458734124999999437, 10.43750000136559386, 0.000000000000000000 ) ) ;
#32075=CARTESIAN_POINT ( 'NONE',  ( 3.061616997868383141E-16, -163.7500000000000000, -5.000000000000000000 ) ) ;
#32077=CARTESIAN_POINT ( 'NONE',  ( 2.229367062500001939, -7.979166665301073991, 3.861377020970579999 ) ) ;
#32080=CARTESIAN_POINT ( 'NONE',  ( 4.458734125000000326, -37.14583333196773651, 2.574251347313718519 ) ) ;
#32087=CARTESIAN_POINT ( 'NONE',  ( -3.152801135295367985, -151.0625000013655779, 3.152801135295367096 ) ) ;
#32088=CARTESIAN_POINT ( 'NONE',  ( -4.458734124999999437, 12.60416666803225993, -2.574251347313719407 ) ) ;
#32091=CARTESIAN_POINT ( 'NONE',  ( -4.458734124999997661, -85.47916666530107932, 2.574251347313722516 ) ) ;
#32094=CARTESIAN_POINT ( 'NONE',  ( 5.000000000000000000, 20.62500000273118772, -6.123233995736766282E-16 ) ) ;
#32095=VERTEX_POINT ( 'NONE', #12609 ) ;
#32097=CARTESIAN_POINT ( 'NONE',  ( 1.975475456537005874E-15, -55.74999999999999289, 5.000000000000000000 ) ) ;
#32099=CARTESIAN_POINT ( 'NONE',  ( 2.499999999999998668, -22.33333333333332860, -4.330127018922193649 ) ) ;
#32100=CARTESIAN_POINT ( 'NONE',  ( -4.458734124999999437, -28.39583333196774007, -2.574251347313719407 ) ) ;
#32101=CARTESIAN_POINT ( 'NONE',  ( -2.229367062499996610, -90.14583333196773651, 3.861377020970582219 ) ) ;
#32102=CARTESIAN_POINT ( 'NONE',  ( 5.000000000000000000, -27.37499999726880873, -6.123233995736766282E-16 ) ) ;
#32103=CARTESIAN_POINT ( 'NONE',  ( -4.458734124999999437, -59.39583333196773651, -2.574251347313719407 ) ) ;
#32104=ORIENTED_EDGE ( 'NONE', *, *, #6790, .T. ) ;
#32106=CARTESIAN_POINT ( 'NONE',  ( -4.458734124999998549, -10.47916666530107044, 2.574251347313722516 ) ) ;
#32107=VERTEX_POINT ( 'NONE', #57006 ) ;
#32108=CARTESIAN_POINT ( 'NONE',  ( -2.500000000000000444, -74.16666666666665719, -4.330127018922193649 ) ) ;
#32111=CARTESIAN_POINT ( 'NONE',  ( -2.500000000000000444, -75.04166666393547303, -4.330127018922193649 ) ) ;
#32112=CARTESIAN_POINT ( 'NONE',  ( 1.339745962155612702, -10.16965819600733312, -5.000000000000000000 ) ) ;
#32115=CARTESIAN_POINT ( 'NONE',  ( 4.458734124999999437, -16.06249999863440436, -5.460374474430324690E-16 ) ) ;
#32116=CARTESIAN_POINT ( 'NONE',  ( -4.458734124999999437, -56.64583333196773651, -2.574251347313719407 ) ) ;
#32117=CARTESIAN_POINT ( 'NONE',  ( -5.000000000000000000, -29.87499999726881228, 0.000000000000000000 ) ) ;
#32119=CARTESIAN_POINT ( 'NONE',  ( 2.730187237215162345E-16, -140.1875000013656063, -4.458734124999999437 ) ) ;
#32121=CARTESIAN_POINT ( 'NONE',  ( 3.535533905932736864, -158.1250000000000284, 3.535533905932738641 ) ) ;
#32125=CARTESIAN_POINT ( 'NONE',  ( 0.000000000000000000, -170.0000000000000000, 0.000000000000000000 ) ) ;
#32128=CARTESIAN_POINT ( 'NONE',  ( -4.458734125000000326, -148.2500000013656063, -1.846868145590735644 ) ) ;
#32132=( BOUNDED_CURVE ( )  B_SPLINE_CURVE ( 2, ( #52839, #33534, #53149, #16135, #21278, #45724, #35126, #10982, #29959 ),
 .UNSPECIFIED., .F., .F. ) 
 B_SPLINE_CURVE_WITH_KNOTS ( ( 3, 2, 2, 2, 3 ),
 ( 0.1229166666666666741, 0.1236111111111111160, 0.1250000000000000000, 0.1263888888888888840, 0.1270833333333333259 ),
 .UNSPECIFIED. ) 
 CURVE ( )  GEOMETRIC_REPRESENTATION_ITEM ( )  RATIONAL_B_SPLINE_CURVE ( ( 0.9330127018922194093, 0.9330127018922200755, 1.000000000000000000, 0.8660254037844387076, 1.000000000000000000, 0.8660254037844387076, 1.000000000000000000, 0.9330127018922194093, 0.9330127018922194093 ) ) 
 REPRESENTATION_ITEM ( '' )  );
#32133=CARTESIAN_POINT ( 'NONE',  ( 4.458734124999999437, -62.06249999863440792, -5.460374474430324690E-16 ) ) ;
#32136=CARTESIAN_POINT ( 'NONE',  ( -3.152801135295367096, -146.0625000013655779, -3.152801135295367541 ) ) ;
#32140=CARTESIAN_POINT ( 'NONE',  ( -5.000000000000000000, -144.5000000000000284, -6.123233995736766282E-16 ) ) ;
#32143=CARTESIAN_POINT ( 'NONE',  ( -5.000000000000000000, -67.99999999999998579, 0.000000000000000000 ) ) ;
#32145=DIRECTION ( 'NONE',  ( -0.000000000000000000, 1.000000000000000000, -0.000000000000000000 ) ) ;
#32150=CARTESIAN_POINT ( 'NONE',  ( 2.499999999999998668, 21.66666666666666785, -4.330127018922193649 ) ) ;
#32151=CARTESIAN_POINT ( 'NONE',  ( 4.458734124999998549, 6.270833334698928674, -2.574251347313721627 ) ) ;
#32153=CARTESIAN_POINT ( 'NONE',  ( 4.458734125000000326, -17.14583333196773651, 2.574251347313718519 ) ) ;
#32155=CARTESIAN_POINT ( 'NONE',  ( -4.458734125000001214, -158.8750000013655779, 1.846868145590734089 ) ) ;
#32156=DIRECTION ( 'NONE',  ( 0.000000000000000000, 0.000000000000000000, 1.000000000000000000 ) ) ;
#32159=EDGE_CURVE ( 'NONE', #46199, #7616, #17119, .T. ) ;
#32161=CARTESIAN_POINT ( 'NONE',  ( 4.458734124999998549, -41.72916666530107932, -2.574251347313721627 ) ) ;
#32162=CARTESIAN_POINT ( 'NONE',  ( 2.500000000000002220, 19.45833333606451632, 4.330127018922192761 ) ) ;
#32163=CARTESIAN_POINT ( 'NONE',  ( 2.229367062500001939, -68.22916666530106511, 3.861377020970579999 ) ) ;
#32164=( BOUNDED_CURVE ( )  B_SPLINE_CURVE ( 2, ( #12952, #38035, #32254, #27427, #3009, #37718, #52829, #37101, #51884 ),
 .UNSPECIFIED., .F., .F. ) 
 B_SPLINE_CURVE_WITH_KNOTS ( ( 3, 2, 2, 2, 3 ),
 ( 0.6812500000000000222, 0.6819444444444444642, 0.6833333333333333481, 0.6847222222222222321, 0.6854166666666666741 ),
 .UNSPECIFIED. ) 
 CURVE ( )  GEOMETRIC_REPRESENTATION_ITEM ( )  RATIONAL_B_SPLINE_CURVE ( ( 0.9330127018922194093, 0.9330127018922194093, 1.000000000000000000, 0.8660254037844387076, 1.000000000000000000, 0.8660254037844387076, 1.000000000000000000, 0.9330127018922194093, 0.9330127018922194093 ) ) 
 REPRESENTATION_ITEM ( '' )  );
#32167=CARTESIAN_POINT ( 'NONE',  ( 5.000000000000000888, -89.58333333333332860, 2.886751345948126879 ) ) ;
#32168=ORIENTED_EDGE ( 'NONE', *, *, #30712, .F. ) ;
#32171=CARTESIAN_POINT ( 'NONE',  ( -4.999999999999999112, -8.916666666666664298, 2.886751345948131764 ) ) ;
#32172=CARTESIAN_POINT ( 'NONE',  ( -4.458734124999997661, -72.22916666530107932, 2.574251347313722516 ) ) ;
#32174=ADVANCED_FACE ( 'NONE', ( #42193 ), #2032, .T. ) ;
#32175=CARTESIAN_POINT ( 'NONE',  ( 5.000000000000000000, -14.29166666393548191, -2.886751345948129988 ) ) ;
#32176=CARTESIAN_POINT ( 'NONE',  ( 4.458734124999998549, -41.72916666530107932, -2.574251347313721627 ) ) ;
#32180=CARTESIAN_POINT ( 'NONE',  ( -2.229367062500000163, 8.270833334698926009, -3.861377020970580443 ) ) ;
#32182=CARTESIAN_POINT ( 'NONE',  ( 1.339745962155612702, -34.16965819600732601, -5.000000000000000000 ) ) ;
#32183=CARTESIAN_POINT ( 'NONE',  ( 1.060575238724906964E-15, -55.74999999999999289, 5.773502691896257311 ) ) ;
#32184=CARTESIAN_POINT ( 'NONE',  ( -1.846868145590737420, -160.0000000013656063, 4.458734124999999437 ) ) ;
#32187=CARTESIAN_POINT ( 'NONE',  ( -4.458734124999998549, -80.22916666530106511, 2.574251347313722516 ) ) ;
#32189=CARTESIAN_POINT ( 'NONE',  ( -2.071067811865475061, -167.6875000000000000, -5.000000000000000888 ) ) ;
#32190=CARTESIAN_POINT ( 'NONE',  ( -4.458734124999999437, -89.39583333196773651, -2.574251347313719407 ) ) ;
#32192=CARTESIAN_POINT ( 'NONE',  ( 9.457646018065525792E-16, -1.312499998634405918, 5.148502694627439702 ) ) ;
#32193=EDGE_CURVE ( 'NONE', #40991, #13039, #31914, .T. ) ;
#32194=CARTESIAN_POINT ( 'NONE',  ( 4.458734125000001214, -33.14583333196774362, 2.574251347313718519 ) ) ;
#32195=VECTOR ( 'NONE', #5710, 1000.000000000000000 ) ;
#32198=CARTESIAN_POINT ( 'NONE',  ( 1.975475456537005874E-15, -54.62499999726880873, 5.000000000000000000 ) ) ;
#32201=CARTESIAN_POINT ( 'NONE',  ( -1.339745962155613812, -19.08034179853029144, -5.000000000000000000 ) ) ;
#32202=CARTESIAN_POINT ( 'NONE',  ( -3.152548672688508926E-16, -67.81249999863440792, -5.148502694627439702 ) ) ;
#32207=CARTESIAN_POINT ( 'NONE',  ( -5.000000000000000000, -146.6250000027312126, -6.123233995736766282E-16 ) ) ;
#32210=CARTESIAN_POINT ( 'NONE',  ( 2.229367062499998831, 4.354166668032260823, -3.861377020970580887 ) ) ;
#32211=CARTESIAN_POINT ( 'NONE',  ( -5.000000000000000000, -32.87499999726880873, 0.000000000000000000 ) ) ;
#32212=CARTESIAN_POINT ( 'NONE',  ( -8.190561711645485556E-16, -155.6875000013655779, 4.458734124999999437 ) ) ;
#32216=CARTESIAN_POINT ( 'NONE',  ( 1.975475456537005874E-15, -24.74999999999999645, 5.000000000000000000 ) ) ;
#32218=DIRECTION ( 'NONE',  ( -0.000000000000000000, 1.000000000000000000, -0.000000000000000000 ) ) ;
#32219=CARTESIAN_POINT ( 'NONE',  ( -6.972266317189433020E-16, -23.12499999726880873, -5.000000000000000000 ) ) ;
#32220=CARTESIAN_POINT ( 'NONE',  ( -6.972266317189433020E-16, -67.25000000000000000, -5.000000000000000000 ) ) ;
#32225=CARTESIAN_POINT ( 'NONE',  ( 4.458734124999998549, 21.27083333469892779, -2.574251347313721627 ) ) ;
#32227=CARTESIAN_POINT ( 'NONE',  ( 4.458734125000000326, -2.145833331967737845, 2.574251347313718519 ) ) ;
#32230=CARTESIAN_POINT ( 'NONE',  ( -9.184850993605147944E-16, -143.3750000027312126, 5.000000000000000000 ) ) ;
#32231=DIRECTION ( 'NONE',  ( 0.000000000000000000, 0.000000000000000000, 1.000000000000000000 ) ) ;
#32234=ADVANCED_FACE ( 'NONE', ( #46707 ), #31267, .T. ) ;
#32242=CARTESIAN_POINT ( 'NONE',  ( -1.846868145590737420, -157.0000000013655779, 4.458734124999997661 ) ) ;
#32245=EDGE_LOOP ( 'NONE', ( #2813, #15487, #41669, #33869 ) ) ;
#32246=CARTESIAN_POINT ( 'NONE',  ( 4.458734124999999437, 19.93750000136559208, -5.460374474430324690E-16 ) ) ;
#32247=ORIENTED_EDGE ( 'NONE', *, *, #46960, .T. ) ;
#32252=CARTESIAN_POINT ( 'NONE',  ( 5.000000000000000000, 9.583333333333333925, -2.886751345948129988 ) ) ;
#32253=CARTESIAN_POINT ( 'NONE',  ( -4.458734124999999437, -57.39583333196773651, -2.574251347313719407 ) ) ;
#32254=CARTESIAN_POINT ( 'NONE',  ( -2.499999999999996447, -52.70833333060213732, 4.330127018922195425 ) ) ;
#32256=DIRECTION ( 'NONE',  ( 0.000000000000000000, 0.000000000000000000, 1.000000000000000000 ) ) ;
#32258=DIRECTION ( 'NONE',  ( 0.000000000000000000, 0.000000000000000000, 1.000000000000000000 ) ) ;
#32259=ADVANCED_FACE ( 'NONE', ( #42506 ), #16487, .T. ) ;
#32260=CARTESIAN_POINT ( 'NONE',  ( -2.071067811865686448, -151.8125000027311842, -4.999999999999789502 ) ) ;
#32261=CARTESIAN_POINT ( 'NONE',  ( -2.500000000000000444, -41.16666666666667140, -4.330127018922193649 ) ) ;
#32265=DIRECTION ( 'NONE',  ( 0.000000000000000000, 0.000000000000000000, 1.000000000000000000 ) ) ;
#32266=CARTESIAN_POINT ( 'NONE',  ( -4.458734124999999437, -62.31249999863440792, 0.000000000000000000 ) ) ;
#32267=CARTESIAN_POINT ( 'NONE',  ( -4.458734124999999437, -149.1875000013656063, -5.460374474430324690E-16 ) ) ;
#32269=CARTESIAN_POINT ( 'NONE',  ( 4.458734124999999437, -73.81249999863440792, -5.460374474430324690E-16 ) ) ;
#32271=( BOUNDED_SURFACE ( )  B_SPLINE_SURFACE ( 1, 2, ( 
 ( #63380, #59180, #43737, #49523, #19295, #34731, #59505, #34398, #54358, #29893, #5464, #54673, #20262, #10597, #38913, #45020, #987, #57377, #10919, #55325, #16070, #30537, #40823, #6433, #41138, #35698, #36013, #11240, #1308, #40196, #50158, #6745, #21858, #21542, #20904, #59832, #26044, #6113, #15754, #55645, #21215, #25728, #16394, #45339, #41453, #40507, #30864, #31178, #45659, #26353, #54993, #50493, #60469, #60149, #45975, #11559, #50808, #1940, #60786, #1616, #16711, #36327, #55955, #35370, #11869, #31485, #51130, #7065, #26678, #46297, #2254, #61102, #34294, #24653, #49088, #20150, #54882, #14673, #24336, #39118, #53916, #49731, #44259, #53606, #15645, #10812, #63584, #19821, #49412, #59716, #58745, #19505, #15322, #4711, #5356, #5034, #9540, #30100, #40073, #44582, #39747, #9842, #25611, #29144, #48766, #10177, #29457, #5676, #43937, #54236, #223, #39430, #59071, #54565, #868, #14996, #45225, #25287, #44912, #34609, #20471, #539, #29780, #24975, #59389, #35261, #30424, #50051, #40394, #34946, #10487, #6009, #1192, #20792, #60035, #33986, #21105, #46508, #56162, #41656, #6959, #2453, #6632, #31065, #16283, #51657, #61307, #41031, #16600, #51014, #16913, #26568, #40710, #15960, #26891, #36530, #50373, #46820, #12084, #31707, #27202, #7280, #11446, #36857, #22064, #11758, #17232, #32020, #56486, #7594, #12408, #60677, #45544, #2764, #22386, #21428, #46187, #51341, #41987, #35582, #55209, #50689, #55842, #2147, #21752, #41347, #60993, #11126, #35901, #30753, #6320, #26241, #25925, #1504, #55536, #60359, #45861, #31376, #1827, #36218, #4330, #8843, #27826, #18793, #8222, #38418, #56803, #38120, #58044, #13038, #13354, #52597, #47449, #28456, #3401, #47141, #23330, #37179, #23017, #17561, #61944, #43240, #13974, #52284, #32341, #62577, #57122, #57434, #27511, #48072, #23948, #42620, #28141, #57743, #33601, #4026, #62881, #32657, #37806, #32977, #47758, #3714, #8531, #53221, #17863, #42934, #13668, #62258, #9153, #23645, #37484, #61626, #12721, #18498, #28765, #33288, #51967, #48388, #18177, #7906, #52907, #3088, #22706, #42304, #38734, #19442, #59001, #33612, #9469, #9781, #43559, #39370, #4968, #24590, #14929, #34536, #4645, #63204, #9162, #162, #40007, #53544, #54172, #20080, #49670, #44197, #19759, #10111, #43872, #14299, #24266, #29078, #29716, #34882, #58372, #4337, #19115, #33919, #49349, #63518, #53230, #59324, #54504, #48705, #39055, #29387, #39685, #58683, #14612, #5294, #48395, #49023, #34225, #28778, #24912, #15257, #44516, #10428, #53852, #478, #30041, #802, #13982, #5613, #23955, #25227, #44838, #20408, #27367, #10752, #30362, #35519, #12892, #37035, #51516, #55142, #45162, #36717, #32511, #47001, #59977, #1447, #56661, #2949, #47315, #1130, #7453, #54821, #51822, #25544, #31882, #61800, #11068, #61489, #17421, #50309, #12270, #56348, #20731, #21921, #41842, #15586, #30692, #27061, #40335, #22243, #46679, #2625, #12579, #32192, #6258, #15900, #49984, #7764, #22879, #25867, #22566, #42164, #52143, #17726, #37342, #56975, #45482, #41519, #61171, #17094, #8085, #27689, #3267, #5938, #59654, #35204, #58217, #33156, #62114, #24126, #63372, #8400, #28312, #57916, #4498, #3573, #28000, #23812, #13213, #13837, #57609, #18032, #38585, #48559, #53076, #38903, #62746, #38289, #43105, #29245, #4817, #9322, #32835, #43727, #37978, #43415, #28935, #57297, #52464, #18353, #58538, #18970, #33457, #13536, #47619, #18667, #14460, #19287, #42792, #47928, #14145, #34082, #48870, #23181, #9015, #37655, #33771, #62435, #28626, #53705, #52770, #63058, #53391, #8699, #9637, #48243, #3883, #23502, #42473, #4199, #60140, #34392, #34721, #59172, #14773, #59496, #5453, #54983, #15105, #10589, #10280, #44359, #24437, #54018, #45012, #35689, #15745, #24755, #50485, #49515, #58844, #44040, #15435, #25071, #39219, #39853, #19607, #20252, #322, #25392, #30527, #16060, #35053, #54665, #30200, #54350, #19920, #29885, #39534, #49829, #45330, #5138, #9951, #29567, #44681, #40188, #642, #5, #6105, #1300, #49198, #5773, #978, #50150, #20581, #59824, #35361, #10912, #25720, #20896, #40498, #55317, #11231, #30856, #2871, #26668, #2245, #7056, #56897, #32438, #36955, #40813, #7693, #1928, #51437, #56584, #21207, #60460, #45966, #22488, #46605, #61094, #21533, #55636, #46288, #42084, #12503, #6736, #11861, #2550, #32115, #12817, #11551, #17018, #1608, #61411, #36005, #41445, #27299, #41130, #7378, #26986, #60777, #46924, #21849, #26345, #16386, #61726, #36633, #17655, #31169, #16702, #36320, #50800, #56266, #51119, #51751, #55947, #12189, #31477, #31804, #6424, #22165, #41761, #37270, #17334, #26036, #45650, #13456, #22803, #8007, #43032, #52690, #3186, #3807, #47241, #47849, #23431, #62672, #13138, #57532, #33382, #27610, #47543, #18593, #17954, #13760, #38219, #57841, #52998, #8937, #42711, #37578, #42397, #28551, #14385, #37902, #57218, #48170, #62037, #33077, #32757, #52385, #33697, #48486, #62353, #8322, #4123, #3494, #23745, #43338, #27922, #43649, #23107, #18277, #28235, #8625, #62982, #18896, #38510, #58138, #14069, #53315, #9249, #28864, #4422, #63289, #24048, #19207, #38823, #58462, #52067, #34635, #9870, #563, #20496, #15664, #44933, #40414, #59416, #9563, #54262, #5058, #40095, #48793, #890, #39143, #59738, #10508, #35282, #24995, #54903, #24678, #49114, #34316, #6029, #10831, #59094, #10201, #5378, #34970, #44603, #58769, #34009, #30445, #54586, #4735, #1214, #30122, #49752, #45246, #25312, #29480, #50072, #25632, #29802, #20811, #60054, #53632, #29169, #24360, #15020, #63609, #43962, #19528, #39459, #20172, #5697, #14699, #53940, #44285, #247, #49436, #39768, #15346, #19844, #6977, #61328, #16303, #26588, #12102, #50710, #27219, #2470, #35925, #42003, #55228, #55864, #56504, #31395, #22405, #26909, #45883, #36874, #26259, #21451, #15977, #36549, #55554, #31087, #51034, #46205, #1845, #46528, #35604, #11151, #11777, #11466, #51358, #30772, #36236, #6653, #41050, #60697, #56181, #22080, #16617, #7614, #7298, #31728, #2166, #41677, #21772, #41365, #61009, #16935, #17250, #12426, #32037, #50393, #51673, #6342, #46836, #2784, #25949, #45564, #1522, #21126, #40732, #60379, #23663, #52612, #28476, #52306, #13056, #61959, #33621, #43259, #23033, #62278, #32995, #62595, #8547, #22722, #61644, #8860, #18515, #32360, #28788, #38137, #57762, #9175, #52923, #57139, #18813, #4046, #57451, #62899, #13993, #48090, #53240, #38435, #42636, #27529, #58062, #4346, #3417, #28160, #13685, #48404, #23965, #17577, #32673, #37821, #47775, #3730, #23352, #42952, #37195, #17881, #33304, #56820, #8240, #12737, #51982, #37501, #7924, #47160, #13374, #3105, #42320, #27842, #47464, #18200, #811, #53860, #49033, #43568, #487, #43881, #58693, #59010, #34547, #9790, #10437, #29398, #29086, #5303, #19126, #4977, #63213, #63529, #25236, #40019, #34234, #14310, #44527, #39065, #39379, #49358, #19451, #35212, #14938, #20089, #54181, #4655, #38745, #54514, #39694, #33931, #10761, #59334, #15267, #54830, #34892, #14622, #20418, #49679, #10120, #5624, #59663, #30050, #15595, #44848, #24600, #9478, #30372, #49994, #44206, #29727, #5947, #58382, #53554, #48715, #171, #19770, #24921, #24277, #11708, #16546, #7227, #25876, #36169, #21701, #60303, #36803, #12028, #45492, #51606, #1140, #1773, #2400, #40983, #31970, #36482, #55478, #46455, #35852, #31012, #25553, #46132, #1455, #40663, #60627, #55790, #11392, #56107, #50641, #31327, #50320, #50962, #6903, #26516, #16232, #11077, #20740, #2100, #45173, #21056, #41292, #31656, #61255, #60941, #16859, #51292, #6579, #26194, #45813, #21375, #26841, #22010, #6269, #15909, #30699, #41603, #17178, #56435, #40343, #12357, #59986, #55153, #35529, #22966, #33236, #32284, #56748, #52547, #41932, #42563, #22654, #46766, #3659, #13618, #18122, #3972, #27773, #3349, #8172, #57996, #33548, #38062, #61574, #8788, #3035, #8479, #57691, #22331, #17509, #47087, #28088, #52855, #42252, #62829, #42876, #23273, #37435, #62522, #37747, #47398, #61893, #57379, #28400, #48021, #18440, #13923, #32924, #2711, #62206, #17809, #23592, #37128, #43188, #12672, #18745, #47705, #38370, #13299, #7538, #57067, #12979, #7852, #27150, #51912, #32602, #27455, #52227, #54104, #24527, #14233, #53166, #412, #10043, #23896, #20341, #29657, #49288, #730, #44452, #48642, #10366, #59259, #48955, #15190, #5544, #20014, #25156, #54438, #34165, #19055, #39620, #59588, #58626, #19696, #5226, #29975, #34815, #49602, #4583, #29325, #44130, #39306, #58933, #97, #44770, #53479, #14860, #24845, #24207, #39941, #15522, #9408, #9102, #28710, #4907, #48333, #34472, #4278, #43499, #19377, #63143, #63458, #14546, #38673, #58311, #29017, #43813, #33859, #38991, #53787, #9720, #50564, #16784, #6507, #10681, #40584, #54756, #35449, #36401, #31575, #25804, #5867, #36087, #30618, #30938, #40900, #10996, #26758, #30295, #49913, #11312, #55075, #6826, #25474, #55396, #50240, #6190, #45416, #26119, #60545, #1383, #46375, #45097, #1062, #45739, #20983, #26432, #20669, #1692, #60228, #16148, #35773, #55716, #2015, #21295, #2323, #46053, #31249, #16467, #50883, #11629, #21618, #41212, #60857, #56031, #11948, #51209, #41529, #7143, #40275, #21929, #61179, #35141, #59913, #15834, #22253, #47627, #57305, #42803, #8093, #3583, #7772, #32202, #17429, #52780, #62444, #42172, #17735, #52151, #18040, #27697, #41850, #17102, #28010, #37663, #51525, #47940, #13222, #32844, #28323, #8408, #12589, #37986, #23190, #12899, #18362, #33166, #57618, #8709, #13545, #61809, #46686, #3893, #23513, #22575, #47325, #52472, #43114, #36726, #56358, #51831, #56983, #3276, #22887, #42484, #62123, #12278, #37044, #31893, #7462, #27376, #27070, #2633, #56671, #61498, #47009, #32522, #2958, #37353, #6354, #10839, #29813, #20823, #10210, #5387, #62755, #20506, #63070, #15030, #15355, #54595, #49445, #34646, #34980, #45258, #10517, #38300, #25002, #18675, #18983, #1224, #60064, #54270, #33467, #899, #59103, #35292, #59748, #44612, #15673, #30131, #572, #38595, #49760, #50080, #40424, #30455, #25958, #25321, #57928, #20181, #39779, #6037, #13846, #25642, #4210, #15988, #40105, #35613, #5706, #55239, #59426, #44941, #54912, #11161, #30783, #50406, #53090, #9026, #28636, #48253, #23822, #43427, #56513, #2478, #16314, #12748, #22091, #41690, #56830, #36883, #41060, #2795, #51682, #41374, #7623, #61653, #12434, #17587, #46848, #26598, #11478, #32046, #51992, #51043, #12110, #61337, #22414, #27227, #42013, #60707, #21782, #16946, #31737, #51367, #36559, #37204, #45892, #56190, #17260, #16627, #32368, #7936, #1854, #45575, #21136, #61020, #1531, #7308, #40741, #60388, #11787, #35935, #55875, #6986, #55563, #31098, #21460, #36248, #26921, #46537, #31405, #46214, #50719, #6663, #26270, #2177, #33003, #47170, #27851, #9182, #23974, #18208, #61969, #28483, #23042, #23360, #33311, #3426, #19134, #3113, #22731, #3739, #47472, #62909, #42329, #47782, #42645, #62286, #37829, #48099, #58068, #57463, #38751, #42959, #4354, #62602, #33938, #38441, #13382, #48410, #52620, #8554, #27538, #4053, #28167, #18525, #38145, #57770, #13692, #52931, #8868, #28794, #23671, #17890, #43269, #37510, #18822, #43576, #63219, #14000, #57150, #33627, #53246, #58390, #14316, #53559, #13065, #32685, #52316, #8251, #29405, #44855, #48722, #29733, #24606, #49038, #44212, #30055, #40023, #177, #1144, #818, #5629, #39385, #25240, #20095, #10126, #4983, #39701, #59667, #54836, #20423, #15913, #34896, #4662 ),
 ( #10441, #19777, #10766, #49365, #59016, #43887, #45178, #5309, #20744, #19458, #14947, #34557, #63535, #44535, #54188, #15598, #24927, #59341, #492, #15272, #9484, #39072, #49684, #40348, #35216, #9797, #35534, #54518, #30377, #58700, #50000, #25561, #5951, #59990, #29095, #24284, #14628, #34241, #53870, #46138, #50328, #46459, #21061, #26520, #56439, #31017, #56111, #12035, #45818, #12361, #55796, #11399, #25880, #27155, #31331, #46771, #1460, #1780, #26198, #45496, #2104, #36175, #22015, #21380, #41297, #40987, #50645, #55162, #40666, #31660, #2717, #2403, #55483, #17513, #16551, #60310, #11081, #21705, #11713, #6274, #6909, #16238, #50966, #60946, #16867, #35857, #60631, #36485, #30703, #6583, #51296, #7232, #26846, #41609, #61259, #17183, #36809, #31975, #51610, #7543, #22339, #41937, #61578, #38069, #43193, #9107, #28093, #47711, #3666, #3353, #37440, #27778, #52234, #23279, #58001, #17815, #27463, #42256, #57071, #52861, #47402, #56753, #18750, #13927, #3040, #22970, #52552, #62835, #61897, #22658, #18446, #7857, #8484, #8176, #12676, #33241, #38374, #42882, #33552, #57385, #32929, #37753, #23903, #63148, #3976, #47092, #53173, #32608, #57697, #23596, #51916, #12983, #42570, #28714, #13623, #48337, #4284, #43503, #62210, #13306, #62527, #8794, #28406, #48026, #37133, #18126, #32290, #15196, #53793, #30300, #5549, #19383, #45102, #58316, #58939, #59593, #34477, #25481, #29981, #48960, #39945, #29330, #24532, #19059, #39626, #38999, #34170, #54109, #10049, #4912, #9727, #29662, #737, #49293, #14241, #44135, #38677, #58631, #20346, #15526, #105, #53484, #20020, #14551, #14868, #24853, #19701, #10690, #33864, #9412, #5233, #39311, #54444, #29023, #44457, #417, #59264, #34821, #10372, #49610, #25161, #49920, #44775, #35146, #54762, #5873, #48647, #4589, #24212, #43818, #63464, #46384, #11956, #7468, #26440, #40280, #21304, #35782, #51217, #15840, #31583, #6194, #7154, #41219, #26764, #55723, #2330, #55404, #16155, #1387, #36732, #21937, #26126, #1700, #36095, #2022, #11636, #25809, #1067, #41535, #21626, #35459, #31902, #60866, #16792, #12286, #56040, #60237, #61187, #17109, #60553, #56364, #51531, #27077, #20674, #59919, #45746, #30624, #55080, #11002, #6514, #31257, #36410, #50891, #30945, #20988, #11320, #50571, #6833, #50246, #45422, #40591, #40908, #16474, #46062, #37362, #2641, #28332, #3900, #12597, #32530, #62130, #8718, #7782, #32210, #28017, #17436, #18048, #61820, #22260, #42809, #52786, #57312, #43120, #3282, #42493, #47332, #33475, #9031, #13552, #37052, #47946, #42180, #47636, #33172, #61506, #56681, #22583, #62760, #23196, #37670, #17745, #51839, #22898, #18680, #23519, #47017, #52158, #62449, #38306, #53097, #27385, #13229, #41859, #37992, #2967, #32852, #57933, #56992, #3591, #18371, #12907, #13852, #52480, #8101, #27705, #46694, #8415, #57624, #38602, #38920, #63388, #18987, #24, #9652, #59192, #19306, #14793, #14475, #48575, #28643, #58235, #49215, #39869, #19939, #28952, #54685, #53721, #63077, #48258, #19625, #29261, #43432, #44060, #23829, #24453, #39235, #58861, #53406, #34096, #9972, #4216, #24141, #4515, #43744, #34405, #9338, #54034, #29583, #5155, #58555, #14162, #33790, #24775, #48889, #4834, #44378, #34741, #661, #339, #39551, #15122, #5473, #54369, #35068, #10296, #29904, #49532, #25088, #44697, #20270, #59516, #15451, #30544, #55332, #30873, #25736, #50168, #11249, #26365, #50501, #30221, #20912, #49846, #35380, #45985, #41147, #6123, #25409, #21227, #10929, #35705, #45667, #45350, #16720, #5792, #45029, #16081, #55001, #36021, #996, #60159, #1317, #40517, #6444, #40833, #31187, #26053, #60794, #55653, #60478, #1626, #16403, #11567, #50816, #6753, #1950, #21551, #36336, #55967, #11878, #31497, #20600, #10607, #40204, #59840, #15765, #34958, #9553, #54575, #44593, #30112, #59084, #10497, #58759, #19518, #4724, #40083, #49742, #29469, #5048, #39447, #5368, #15010, #29158, #4412, #15335, #24986, #38810, #35272, #553, #20162, #15654, #59403, #63598, #25302, #5686, #236, #44923, #20485, #878, #59727, #54894, #49102, #33999, #10823, #30435, #9859, #34624, #39758, #24036, #43638, #63280, #39132, #44274, #54249, #10191, #29791, #49424, #19197, #24350, #58452, #14375, #14689, #53622, #48782, #43950, #34307, #53930, #19834, #24666, #61002, #16294, #7291, #60371, #55546, #50064, #6969, #50385, #1514, #1837, #41043, #35917, #21117, #21439, #31718, #60690, #25624, #11457, #6019, #6333, #51352, #46521, #40724, #20803, #51027, #45556, #45874, #55856, #25937, #41670, #45238, #1203, #26251, #31079, #21765, #40406, #6644, #50701, #16610, #36229, #26579, #16926, #11769, #61319, #41358, #46198, #31388, #2158, #36541, #56174, #12095, #26901, #2463, #22074, #17243, #56497, #36867, #60045, #12418, #15969, #35596, #55220, #11140, #30764, #62585, #8540, #57753, #23026, #18508, #22716, #47151, #32354, #4036, #13677, #57134, #32667, #3410, #32987, #42629, #56813, #32031, #42944, #52606, #2778, #62890, #28152, #47767, #43249, #23343, #27523, #52914, #38129, #27836, #33296, #48081, #8851, #23655, #28468, #13050, #61638, #18803, #38426, #37493, #62268, #3722, #58052, #51666, #7608, #3099, #8233, #18193, #37815, #57443, #13366, #27213, #51976, #46830, #22397, #42313, #41997, #17570, #7917, #37189, #12730, #47458, #61953, #17874, #52297, #42538, #62176, #53453, #38650, #18416, #3326, #4257, #43788, #42854, #3947, #33527, #14207, #43477, #58288, #52523, #13595, #8766, #23570, #43165, #28374, #19033, #37720, #47995, #53142, #8458, #48618, #23872, #57355, #63435, #12954, #33214, #33836, #52832, #37406, #48306, #3633, #9384, #47682, #62498, #57041, #57974, #13274, #28065, #62804, #18724, #23244, #38037, #38348, #28994, #13900, #32578, #57669, #52200, #32898, #4557, #24182, #9077, #8147, #28686, #63122, #27747, #47376, #22944, #18096, #38964, #58602, #59232, #39280, #54732, #14520, #39596, #34449, #58908, #54081, #39915, #49889, #10019, #10972, #10653, #15495, #49264, #35118, #29950, #19988, #14835, #49575, #5840, #1039, #30269, #25781, #44743, #34142, #15165, #29630, #25452, #53761, #45072, #24502, #20645, #59563, #40249, #10341, #59889, #5201, #24819, #19669, #55049, #15809, #44425, #34789, #54411, #20314, #5518, #44105, #19350, #35425, #30593, #9695, #50214, #6164, #45392, #29302, #48932, #385, #4880, #25131, #69, #704, #60204, #60835, #16761, #36378, #26095, #6802, #46349, #20961, #60519, #21270, #16446, #11922, #45716, #56008, #26734, #2305, #55694, #50541, #16126, #51186, #27353, #40877, #21907, #7438, #37021, #31551, #7118, #41504, #31228, #1668, #11608, #36065, #61157, #22228, #50858, #55374, #6485, #26410, #17080, #46028, #40561, #46665, #41828, #30915, #1991, #36699, #27047, #21595, #41190, #56334, #35748, #12254, #31868, #11289, #51501, #2610, #61472, #17406, #56648, #12564, #32176, #51808, #1357, #7750, #17713, #48228, #42457, #28299, #13825, #61786, #37328, #22866, #63046, #23489, #37962, #62100, #32497, #23167, #18956, #33444, #47299, #52450, #43091, #53061, #33757, #52129, #57596, #42150, #38276, #38572, #47912, #27672, #12879, #3869, #62732, #37640, #4185, #47605, #3253, #56959, #58203, #42776, #14130, #8071, #57283, #18017, #13199, #18340, #27986, #9001, #32821, #33142, #8385, #3559, #46986, #62421, #18654, #53375, #57901, #13524, #9309, #52757, #8686, #2935, #28612, #23799, #43401, #22548, #15417, #29231, #54970, #4485, #5122, #5759, #44345, #35349, #39839, #58829, #49814, #39205, #34377, #28923, #49500, #48857, #44026, #308, #19906, #14759, #63673, #39521, #10575, #59158, #24114, #54005, #48546, #4800, #30186, #25377, #19593, #63356, #29870, #24424, #24742, #34707, #9935, #20566, #43712, #19272, #15091, #29550, #627, #38888, #49184, #54332, #10266, #5439, #25057, #59482, #44667, #40171, #20237, #35039, #54651, #44999, #964, #59809, #15731, #58522, #14447, #34068, #53691, #9623, #36307, #50136, #31154, #45637, #61082, #25704, #41433, #16046, #17004, #51105, #36619, #1914, #56252, #1595, #26021, #11218, #46593, #12176, #35991, #11537, #45949, #11846, #21519, #35675, #10898, #21836, #31464, #45315, #41747, #7043, #26655, #22153, #2232, #6411, #31791, #51423, #7366, #55622, #55302, #30842, #26974, #2537, #50782, #40484, #61396, #17321, #16372, #41115, #46273, #36944, #30513, #6091, #21193, #6722, #60763, #16688, #55931, #1282, #20881, #50472, #60125, #40800, #60447, #26332, #56885, #18883, #17941, #27287, #12491, #47531, #57206, #7681, #8308, #51739, #52371, #27909, #3481, #17641, #62024, #37890, #32103, #52055, #12805, #7993, #23095, #37257, #42698, #18263, #57520, #47228, #42071, #46912, #62342, #56569, #32426, #13439, #62660, #28538, #33064, #52678, #8613, #22791, #27595, #3171, #42384, #28221, #13748, #37566, #2854, #61712, #13125, #47837, #32743, #22476, #38203, #33370, #3796, #23417, #43020, #18580, #57828, #52984, #8925, #48158, #4111, #23731, #43326, #62967, #45478, #49099, #35840, #58756, #34304, #39129, #26180, #1759, #6253, #9237, #40651, #33996, #19831, #25862, #53303, #28851, #14372, #55463, #15895, #29466, #53619, #24033, #14686, #11379, #1442, #38807, #43947, #35515, #21044, #45799, #43635, #5045, #33682, #30688, #30999, #39444, #19194, #4409, #59081, #55136, #29155, #60290, #53927, #58449, #48473, #50627, #9856, #6565, #63277, #48779, #9550, #4721, #24663, #19515, #16214, #24347, #44271, #63595, #233, #38498, #11063, #50304, #58126, #14057, #7524, #47386, #60925, #22315, #27439, #57053, #12343, #31954, #51586, #51276, #21686, #12012, #36465, #27135, #42237, #2080, #11692, #26502, #41276, #37115, #31641, #40965, #3022, #61879, #50947, #7209, #36787, #47073, #46117, #6888, #2695, #55775, #56420, #56092, #60613, #17493, #22638, #46750, #17795, #41589, #17163, #21996, #8159, #21361, #51897, #31311, #37419, #16844, #41916, #7838, #36155, #26821, #46440, #12964, #61559, #56733, #2386, #61241, #12653, #32589, #52212, #32269, #27758, #16532, #33845, #53774, #8468, #57984, #62188, #58299, #38975, #4267, #47693, #32911, #23884, #43487, #57680, #4569, #3958, #23257, #37731, #58612, #43175, #14533, #13285, #13606, #38047, #57364, #38358, #48005, #53464, #33223, #53152, #52842, #42864, #3337, #52534, #63132, #34152, #14218, #3645, #29311, #28386, #28076, #22953, #13909, #23579, #18109, #18733, #62509, #62816, #33537, #9088, #18426, #8776, #48317, #42549, #28697, #19043, #38660, #9394, #29004, #48629, #24192, #43799, #63446, #19363, #9706, #45085, #55061, #59575, #45404, #5529, #44755, #49587, #35760, #11301, #15822, #19680, #50228, #44437, #30281, #35435, #80, #39292, #24831, #1371, #25463, #39928, #398, #34460, #25144, #20972, #10985, #49276, #54424, #1051, #30605, #55384, #54091, #15508, #44116, #40261, #40573, #49901, #29642, #14848, #5855, #20657, #39608, #6176, #716, #5212, #58919, #60214, #20326, #16138, #10030, #59245, #20000, #15176, #35129, #29962, #25793, #34801, #54745, #10353, #10665, #48943, #59901, #4891, #24514, #22240, #31239, #56973, #56021, #1679, #50552, #21919, #31565, #45728, #46362, #26108, #26746, #2316, #41516, #55705, #36390, #12267, #6496, #26422, #50871, #46039, #61169, #11619, #17092, #56346, #31880, #21607, #16457, #21281, #36715, #30925, #6815, #51514, #37033, #2947, #7451, #27059, #46677, #60846, #2003, #41202, #16772, #2622, #51820, #11936, #40888, #36076, #51198, #41840, #7130, #60533, #12577, #7762, #61487, #17418, #56659, #32190, #27365, #46999, #22563, #42162, #61798, #17724, #37340, #27998, #62744, #33769, #57295 ) ),
 .UNSPECIFIED., .F., .F., .F. ) 
 B_SPLINE_SURFACE_WITH_KNOTS ( ( 2, 2 ),
 ( 3, 2, 2, 2, 2, 2, 2, 2, 2, 2, 2, 2, 2, 2, 2, 2, 2, 2, 2, 2, 2, 2, 2, 2, 2, 2, 2, 2, 2, 2, 2, 2, 2, 2, 2, 2, 2, 2, 2, 2, 2, 2, 2, 2, 2, 2, 2, 2, 2, 2, 2, 2, 2, 2, 2, 2, 2, 2, 2, 2, 2, 2, 2, 2, 2, 2, 2, 2, 2, 2, 2, 2, 2, 2, 2, 2, 2, 2, 2, 2, 2, 2, 2, 2, 2, 2, 2, 2, 2, 2, 2, 2, 2, 2, 2, 2, 2, 2, 2, 2, 2, 2, 2, 2, 2, 2, 2, 2, 2, 2, 2, 2, 2, 2, 2, 2, 2, 2, 2, 2, 2, 2, 2, 2, 2, 2, 2, 2, 2, 2, 2, 2, 2, 2, 2, 2, 2, 2, 2, 2, 2, 2, 2, 2, 2, 2, 2, 2, 2, 2, 2, 2, 2, 2, 2, 2, 2, 2, 2, 2, 2, 2, 2, 2, 2, 2, 2, 2, 2, 2, 2, 2, 2, 2, 2, 2, 2, 2, 2, 2, 2, 2, 2, 2, 2, 2, 2, 2, 2, 2, 2, 2, 2, 2, 2, 2, 2, 2, 2, 2, 2, 2, 2, 2, 2, 2, 2, 2, 2, 2, 2, 2, 2, 2, 2, 2, 2, 2, 2, 2, 2, 2, 2, 2, 2, 2, 2, 2, 2, 2, 2, 2, 2, 2, 2, 2, 2, 2, 2, 2, 2, 2, 2, 2, 2, 2, 2, 2, 2, 2, 2, 2, 2, 2, 2, 2, 2, 2, 2, 2, 2, 2, 2, 2, 2, 2, 2, 2, 2, 2, 2, 2, 2, 2, 2, 2, 2, 2, 2, 2, 2, 2, 2, 2, 2, 2, 2, 2, 2, 2, 2, 2, 2, 2, 2, 2, 2, 2, 2, 2, 2, 2, 2, 2, 2, 2, 2, 2, 2, 2, 2, 2, 2, 2, 2, 2, 2, 2, 2, 2, 2, 2, 2, 2, 2, 2, 2, 2, 2, 2, 2, 2, 2, 2, 2, 2, 2, 2, 2, 2, 2, 2, 2, 2, 2, 2, 2, 2, 2, 2, 2, 2, 2, 2, 2, 2, 2, 2, 2, 2, 2, 2, 2, 2, 2, 2, 2, 2, 2, 2, 2, 2, 2, 2, 2, 2, 2, 2, 2, 2, 2, 2, 2, 2, 2, 2, 2, 2, 2, 2, 2, 2, 2, 2, 2, 2, 2, 2, 2, 2, 2, 2, 2, 2, 2, 2, 2, 2, 2, 2, 2, 2, 2, 2, 2, 2, 2, 2, 2, 2, 2, 2, 2, 2, 2, 2, 2, 2, 2, 2, 2, 2, 2, 2, 2, 2, 2, 2, 2, 2, 2, 2, 2, 2, 2, 2, 2, 2, 2, 2, 2, 2, 2, 2, 2, 2, 2, 2, 2, 2, 2, 2, 2, 2, 2, 2, 2, 2, 2, 2, 2, 2, 2, 2, 2, 2, 2, 2, 2, 2, 2, 2, 2, 2, 2, 2, 2, 2, 2, 2, 2, 2, 2, 2, 2, 2, 2, 2, 2, 2, 2, 2, 2, 2, 2, 2, 2, 2, 2, 2, 2, 2, 2, 2, 2, 2, 2, 2, 2, 2, 2, 2, 2, 2, 2, 2, 2, 2, 2, 2, 2, 2, 2, 2, 2, 2, 2, 2, 2, 2, 2, 2, 2, 2, 2, 2, 2, 2, 2, 2, 2, 2, 2, 2, 2, 2, 2, 2, 2, 2, 2, 2, 2, 2, 2, 2, 2, 2, 2, 2, 2, 2, 2, 2, 2, 2, 2, 2, 2, 2, 2, 2, 2, 2, 2, 2, 2, 2, 2, 2, 2, 2, 2, 2, 2, 2, 2, 2, 2, 2, 2, 2, 2, 2, 2, 2, 2, 2, 2, 2, 2, 2, 2, 2, 2, 2, 2, 2, 2, 2, 2, 2, 2, 2, 2, 2, 2, 2, 2, 2, 2, 2, 2, 2, 2, 2, 2, 2, 2, 2, 2, 2, 2, 2, 2, 2, 2, 2, 2, 2, 2, 2, 2, 2, 2, 2, 2, 2, 2, 2, 2, 2, 2, 2, 2, 2, 2, 2, 2, 2, 2, 2, 2, 2, 2, 2, 2, 2, 2, 2, 2, 2, 2, 2, 2, 2, 2, 2, 2, 2, 2, 2, 2, 2, 2, 2, 2, 2, 2, 2, 2, 2, 2, 2, 2, 2, 2, 2, 2, 2, 2, 2, 2, 2, 2, 2, 2, 2, 2, 2, 3 ),
 ( 0.000000000000000000, 1.000000000000000000 ),
 ( 0.000000000000000000, 0.001388888888888888942, 0.002777777777777777884, 0.004166666666666666609, 0.005555555555555555768, 0.006944444444444444059, 0.008333333333333333218, 0.009722222222222222376, 0.01111111111111111154, 0.01250000000000000069, 0.01388888888888888812, 0.01527777777777777728, 0.01666666666666666644, 0.01805555555555555386, 0.01944444444444444475, 0.02083333333333333218, 0.02222222222222222307, 0.02361111111111111049, 0.02500000000000000139, 0.02638888888888888881, 0.02777777777777777624, 0.02916666666666666713, 0.03055555555555555455, 0.03194444444444444198, 0.03333333333333333287, 0.03472222222222222376, 0.03611111111111110772, 0.03749999999999999861, 0.03888888888888888951, 0.04027777777777778040, 0.04166666666666666435, 0.04305555555555555525, 0.04444444444444444614, 0.04583333333333333010, 0.04722222222222222099, 0.04861111111111111188, 0.05000000000000000278, 0.05138888888888888673, 0.05277777777777777762, 0.05416666666666666852, 0.05555555555555555247, 0.05694444444444444337, 0.05833333333333333426, 0.05972222222222222515, 0.06111111111111110911, 0.06250000000000000000, 0.06388888888888888395, 0.06527777777777778179, 0.06666666666666666574, 0.06805555555555554970, 0.06944444444444444753, 0.07083333333333333148, 0.07222222222222221544, 0.07361111111111111327, 0.07499999999999999722, 0.07638888888888889506, 0.07777777777777777901, 0.07916666666666666297, 0.08055555555555556080, 0.08194444444444444475, 0.08333333333333332871, 0.08472222222222222654, 0.08611111111111111049, 0.08749999999999999445, 0.08888888888888889228, 0.09027777777777777624, 0.09166666666666666019, 0.09305555555555555802, 0.09444444444444444198, 0.09583333333333333981, 0.09722222222222222376, 0.09861111111111110772, 0.1000000000000000056, 0.1013888888888888895, 0.1027777777777777735, 0.1041666666666666713, 0.1055555555555555552, 0.1069444444444444392, 0.1083333333333333370, 0.1097222222222222210, 0.1111111111111111049, 0.1125000000000000028, 0.1138888888888888867, 0.1152777777777777846, 0.1166666666666666685, 0.1180555555555555525, 0.1194444444444444503, 0.1208333333333333343, 0.1222222222222222182, 0.1236111111111111160, 0.1250000000000000000, 0.1263888888888888840, 0.1277777777777777679, 0.1291666666666666796, 0.1305555555555555636, 0.1319444444444444475, 0.1333333333333333315, 0.1347222222222222154, 0.1361111111111110994, 0.1375000000000000111, 0.1388888888888888951, 0.1402777777777777790, 0.1416666666666666630, 0.1430555555555555469, 0.1444444444444444309, 0.1458333333333333426, 0.1472222222222222265, 0.1486111111111111105, 0.1499999999999999944, 0.1513888888888888784, 0.1527777777777777901, 0.1541666666666666741, 0.1555555555555555580, 0.1569444444444444420, 0.1583333333333333259, 0.1597222222222222099, 0.1611111111111111216, 0.1625000000000000056, 0.1638888888888888895, 0.1652777777777777735, 0.1666666666666666574, 0.1680555555555555691, 0.1694444444444444531, 0.1708333333333333370, 0.1722222222222222210, 0.1736111111111111049, 0.1749999999999999889, 0.1763888888888889006, 0.1777777777777777846, 0.1791666666666666685, 0.1805555555555555525, 0.1819444444444444364, 0.1833333333333333204, 0.1847222222222222321, 0.1861111111111111160, 0.1875000000000000000, 0.1888888888888888840, 0.1902777777777777679, 0.1916666666666666796, 0.1930555555555555636, 0.1944444444444444475, 0.1958333333333333315, 0.1972222222222222154, 0.1986111111111110994, 0.2000000000000000111, 0.2013888888888888951, 0.2027777777777777790, 0.2041666666666666630, 0.2055555555555555469, 0.2069444444444444309, 0.2083333333333333426, 0.2097222222222222265, 0.2111111111111111105, 0.2124999999999999944, 0.2138888888888888784, 0.2152777777777777901, 0.2166666666666666741, 0.2180555555555555580, 0.2194444444444444420, 0.2208333333333333259, 0.2222222222222222099, 0.2236111111111111216, 0.2250000000000000056, 0.2263888888888888895, 0.2277777777777777735, 0.2291666666666666574, 0.2305555555555555691, 0.2319444444444444531, 0.2333333333333333370, 0.2347222222222222210, 0.2361111111111111049, 0.2374999999999999889, 0.2388888888888889006, 0.2402777777777777846, 0.2416666666666666685, 0.2430555555555555525, 0.2444444444444444364, 0.2458333333333333204, 0.2472222222222222321, 0.2486111111111111160, 0.2500000000000000000, 0.2513888888888888840, 0.2527777777777777679, 0.2541666666666666519, 0.2555555555555555358, 0.2569444444444444198, 0.2583333333333333592, 0.2597222222222222432, 0.2611111111111111271, 0.2625000000000000111, 0.2638888888888888951, 0.2652777777777777790, 0.2666666666666666630, 0.2680555555555555469, 0.2694444444444444309, 0.2708333333333333148, 0.2722222222222221988, 0.2736111111111111382, 0.2750000000000000222, 0.2763888888888889062, 0.2777777777777777901, 0.2791666666666666741, 0.2805555555555555580, 0.2819444444444444420, 0.2833333333333333259, 0.2847222222222222099, 0.2861111111111110938, 0.2874999999999999778, 0.2888888888888888618, 0.2902777777777778012, 0.2916666666666666852, 0.2930555555555555691, 0.2944444444444444531, 0.2958333333333333370, 0.2972222222222222210, 0.2986111111111111049, 0.2999999999999999889, 0.3013888888888888729, 0.3027777777777777568, 0.3041666666666666408, 0.3055555555555555802, 0.3069444444444444642, 0.3083333333333333481, 0.3097222222222222321, 0.3111111111111111160, 0.3125000000000000000, 0.3138888888888888840, 0.3152777777777777679, 0.3166666666666666519, 0.3180555555555555358, 0.3194444444444444198, 0.3208333333333333592, 0.3222222222222222432, 0.3236111111111111271, 0.3250000000000000111, 0.3263888888888888951, 0.3277777777777777790, 0.3291666666666666630, 0.3305555555555555469, 0.3319444444444444309, 0.3333333333333333148, 0.3347222222222221988, 0.3361111111111111382, 0.3375000000000000222, 0.3388888888888889062, 0.3402777777777777901, 0.3416666666666666741, 0.3430555555555555580, 0.3444444444444444420, 0.3458333333333333259, 0.3472222222222222099, 0.3486111111111110938, 0.3499999999999999778, 0.3513888888888888618, 0.3527777777777778012, 0.3541666666666666852, 0.3555555555555555691, 0.3569444444444444531, 0.3583333333333333370, 0.3597222222222222210, 0.3611111111111111049, 0.3624999999999999889, 0.3638888888888888729, 0.3652777777777777568, 0.3666666666666666408, 0.3680555555555555802, 0.3694444444444444642, 0.3708333333333333481, 0.3722222222222222321, 0.3736111111111111160, 0.3750000000000000000, 0.3763888888888888840, 0.3777777777777777679, 0.3791666666666666519, 0.3805555555555555358, 0.3819444444444444198, 0.3833333333333333592, 0.3847222222222222432, 0.3861111111111111271, 0.3875000000000000111, 0.3888888888888888951, 0.3902777777777777790, 0.3916666666666666630, 0.3930555555555555469, 0.3944444444444444309, 0.3958333333333333148, 0.3972222222222221988, 0.3986111111111111382, 0.4000000000000000222, 0.4013888888888889062, 0.4027777777777777901, 0.4041666666666666741, 0.4055555555555555580, 0.4069444444444444420, 0.4083333333333333259, 0.4097222222222222099, 0.4111111111111110938, 0.4124999999999999778, 0.4138888888888888618, 0.4152777777777778012, 0.4166666666666666852, 0.4180555555555555691, 0.4194444444444444531, 0.4208333333333333370, 0.4222222222222222210, 0.4236111111111111049, 0.4249999999999999889, 0.4263888888888888729, 0.4277777777777777568, 0.4291666666666666408, 0.4305555555555555802, 0.4319444444444444642, 0.4333333333333333481, 0.4347222222222222321, 0.4361111111111111160, 0.4375000000000000000, 0.4388888888888888840, 0.4402777777777777679, 0.4416666666666666519, 0.4430555555555555358, 0.4444444444444444198, 0.4458333333333333592, 0.4472222222222222432, 0.4486111111111111271, 0.4500000000000000111, 0.4513888888888888951, 0.4527777777777777790, 0.4541666666666666630, 0.4555555555555555469, 0.4569444444444444309, 0.4583333333333333148, 0.4597222222222221988, 0.4611111111111111382, 0.4625000000000000222, 0.4638888888888889062, 0.4652777777777777901, 0.4666666666666666741, 0.4680555555555555580, 0.4694444444444444420, 0.4708333333333333259, 0.4722222222222222099, 0.4736111111111110938, 0.4749999999999999778, 0.4763888888888888618, 0.4777777777777778012, 0.4791666666666666852, 0.4805555555555555691, 0.4819444444444444531, 0.4833333333333333370, 0.4847222222222222210, 0.4861111111111111049, 0.4874999999999999889, 0.4888888888888888729, 0.4902777777777777568, 0.4916666666666666408, 0.4930555555555555802, 0.4944444444444444642, 0.4958333333333333481, 0.4972222222222222321, 0.4986111111111111160, 0.5000000000000000000, 0.5013888888888888840, 0.5027777777777777679, 0.5041666666666666519, 0.5055555555555555358, 0.5069444444444444198, 0.5083333333333333037, 0.5097222222222221877, 0.5111111111111110716, 0.5124999999999999556, 0.5138888888888888395, 0.5152777777777777235, 0.5166666666666667185, 0.5180555555555556024, 0.5194444444444444864, 0.5208333333333333703, 0.5222222222222222543, 0.5236111111111111382, 0.5250000000000000222, 0.5263888888888889062, 0.5277777777777777901, 0.5291666666666666741, 0.5305555555555555580, 0.5319444444444444420, 0.5333333333333333259, 0.5347222222222222099, 0.5361111111111110938, 0.5374999999999999778, 0.5388888888888888618, 0.5402777777777777457, 0.5416666666666666297, 0.5430555555555555136, 0.5444444444444443976, 0.5458333333333332815, 0.5472222222222222765, 0.5486111111111111605, 0.5500000000000000444, 0.5513888888888889284, 0.5527777777777778123, 0.5541666666666666963, 0.5555555555555555802, 0.5569444444444444642, 0.5583333333333333481, 0.5597222222222222321, 0.5611111111111111160, 0.5625000000000000000, 0.5638888888888888840, 0.5652777777777777679, 0.5666666666666666519, 0.5680555555555555358, 0.5694444444444444198, 0.5708333333333333037, 0.5722222222222221877, 0.5736111111111110716, 0.5749999999999999556, 0.5763888888888888395, 0.5777777777777777235, 0.5791666666666667185, 0.5805555555555556024, 0.5819444444444444864, 0.5833333333333333703, 0.5847222222222222543, 0.5861111111111111382, 0.5875000000000000222, 0.5888888888888889062, 0.5902777777777777901, 0.5916666666666666741, 0.5930555555555555580, 0.5944444444444444420, 0.5958333333333333259, 0.5972222222222222099, 0.5986111111111110938, 0.5999999999999999778, 0.6013888888888888618, 0.6027777777777777457, 0.6041666666666666297, 0.6055555555555555136, 0.6069444444444443976, 0.6083333333333332815, 0.6097222222222222765, 0.6111111111111111605, 0.6125000000000000444, 0.6138888888888889284, 0.6152777777777778123, 0.6166666666666666963, 0.6180555555555555802, 0.6194444444444444642, 0.6208333333333333481, 0.6222222222222222321, 0.6236111111111111160, 0.6250000000000000000, 0.6263888888888888840, 0.6277777777777777679, 0.6291666666666666519, 0.6305555555555555358, 0.6319444444444444198, 0.6333333333333333037, 0.6347222222222221877, 0.6361111111111110716, 0.6374999999999999556, 0.6388888888888888395, 0.6402777777777777235, 0.6416666666666667185, 0.6430555555555556024, 0.6444444444444444864, 0.6458333333333333703, 0.6472222222222222543, 0.6486111111111111382, 0.6500000000000000222, 0.6513888888888889062, 0.6527777777777777901, 0.6541666666666666741, 0.6555555555555555580, 0.6569444444444444420, 0.6583333333333333259, 0.6597222222222222099, 0.6611111111111110938, 0.6624999999999999778, 0.6638888888888888618, 0.6652777777777777457, 0.6666666666666666297, 0.6680555555555555136, 0.6694444444444443976, 0.6708333333333332815, 0.6722222222222222765, 0.6736111111111111605, 0.6750000000000000444, 0.6763888888888889284, 0.6777777777777778123, 0.6791666666666666963, 0.6805555555555555802, 0.6819444444444444642, 0.6833333333333333481, 0.6847222222222222321, 0.6861111111111111160, 0.6875000000000000000, 0.6888888888888888840, 0.6902777777777777679, 0.6916666666666666519, 0.6930555555555555358, 0.6944444444444444198, 0.6958333333333333037, 0.6972222222222221877, 0.6986111111111110716, 0.6999999999999999556, 0.7013888888888888395, 0.7027777777777777235, 0.7041666666666667185, 0.7055555555555556024, 0.7069444444444444864, 0.7083333333333333703, 0.7097222222222222543, 0.7111111111111111382, 0.7125000000000000222, 0.7138888888888889062, 0.7152777777777777901, 0.7166666666666666741, 0.7180555555555555580, 0.7194444444444444420, 0.7208333333333333259, 0.7222222222222222099, 0.7236111111111110938, 0.7249999999999999778, 0.7263888888888888618, 0.7277777777777777457, 0.7291666666666666297, 0.7305555555555555136, 0.7319444444444443976, 0.7333333333333332815, 0.7347222222222222765, 0.7361111111111111605, 0.7375000000000000444, 0.7388888888888889284, 0.7402777777777778123, 0.7416666666666666963, 0.7430555555555555802, 0.7444444444444444642, 0.7458333333333333481, 0.7472222222222222321, 0.7486111111111111160, 0.7500000000000000000, 0.7513888888888888840, 0.7527777777777777679, 0.7541666666666666519, 0.7555555555555555358, 0.7569444444444444198, 0.7583333333333333037, 0.7597222222222221877, 0.7611111111111110716, 0.7624999999999999556, 0.7638888888888888395, 0.7652777777777777235, 0.7666666666666667185, 0.7680555555555556024, 0.7694444444444444864, 0.7708333333333333703, 0.7722222222222222543, 0.7736111111111111382, 0.7750000000000000222, 0.7763888888888889062, 0.7777777777777777901, 0.7791666666666666741, 0.7805555555555555580, 0.7819444444444444420, 0.7833333333333333259, 0.7847222222222222099, 0.7861111111111110938, 0.7874999999999999778, 0.7888888888888888618, 0.7902777777777777457, 0.7916666666666666297, 0.7930555555555555136, 0.7944444444444443976, 0.7958333333333332815, 0.7972222222222222765, 0.7986111111111111605, 0.8000000000000000444, 0.8013888888888889284, 0.8027777777777778123, 0.8041666666666666963, 0.8055555555555555802, 0.8069444444444444642, 0.8083333333333333481, 0.8097222222222222321, 0.8111111111111111160, 0.8125000000000000000, 0.8138888888888888840, 0.8152777777777777679, 0.8166666666666666519, 0.8180555555555555358, 0.8194444444444444198, 0.8208333333333333037, 0.8222222222222221877, 0.8236111111111110716, 0.8249999999999999556, 0.8263888888888888395, 0.8277777777777777235, 0.8291666666666667185, 0.8305555555555556024, 0.8319444444444444864, 0.8333333333333333703, 0.8347222222222222543, 0.8361111111111111382, 0.8375000000000000222, 0.8388888888888889062, 0.8402777777777777901, 0.8416666666666666741, 0.8430555555555555580, 0.8444444444444444420, 0.8458333333333333259, 0.8472222222222222099, 0.8486111111111110938, 0.8499999999999999778, 0.8513888888888888618, 0.8527777777777777457, 0.8541666666666666297, 0.8555555555555555136, 0.8569444444444443976, 0.8583333333333332815, 0.8597222222222222765, 0.8611111111111111605, 0.8625000000000000444, 0.8638888888888889284, 0.8652777777777778123, 0.8666666666666666963, 0.8680555555555555802, 0.8694444444444444642, 0.8708333333333333481, 0.8722222222222222321, 0.8736111111111111160, 0.8750000000000000000, 0.8763888888888888840, 0.8777777777777777679, 0.8791666666666666519, 0.8805555555555555358, 0.8819444444444444198, 0.8833333333333333037, 0.8847222222222221877, 0.8861111111111110716, 0.8874999999999999556, 0.8888888888888888395, 0.8902777777777777235, 0.8916666666666667185, 0.8930555555555556024, 0.8944444444444444864, 0.8958333333333333703, 0.8972222222222222543, 0.8986111111111111382, 0.9000000000000000222, 0.9013888888888889062, 0.9027777777777777901, 0.9041666666666666741, 0.9055555555555555580, 0.9069444444444444420, 0.9083333333333333259, 0.9097222222222222099, 0.9111111111111110938, 0.9124999999999999778, 0.9138888888888888618, 0.9152777777777777457, 0.9166666666666666297, 0.9180555555555555136, 0.9194444444444443976, 0.9208333333333332815, 0.9222222222222222765, 0.9236111111111111605, 0.9250000000000000444, 0.9263888888888889284, 0.9277777777777778123, 0.9291666666666666963, 0.9305555555555555802, 0.9319444444444444642, 0.9333333333333333481, 0.9347222222222222321, 0.9361111111111111160, 0.9375000000000000000, 0.9388888888888888840, 0.9402777777777777679, 0.9416666666666666519, 0.9430555555555555358, 0.9444444444444444198, 0.9458333333333333037, 0.9472222222222221877, 0.9486111111111110716, 0.9499999999999999556, 0.9513888888888888395, 0.9527777777777777235, 0.9541666666666667185, 0.9555555555555556024, 0.9569444444444444864, 0.9583333333333333703, 0.9597222222222222543, 0.9611111111111111382, 0.9625000000000000222, 0.9638888888888889062, 0.9652777777777777901, 0.9666666666666666741, 0.9680555555555555580, 0.9694444444444444420, 0.9708333333333333259, 0.9722222222222222099, 0.9736111111111110938, 0.9749999999999999778, 0.9763888888888888618, 0.9777777777777777457, 0.9791666666666666297, 0.9805555555555555136, 0.9819444444444443976, 0.9833333333333332815, 0.9847222222222222765, 0.9861111111111111605, 0.9875000000000000444, 0.9888888888888889284, 0.9902777777777778123, 0.9916666666666666963, 0.9930555555555555802, 0.9944444444444444642, 0.9958333333333333481, 0.9972222222222222321, 0.9986111111111111160, 1.000000000000000000 ),
 .UNSPECIFIED. ) 
 GEOMETRIC_REPRESENTATION_ITEM ( )  RATIONAL_B_SPLINE_SURFACE ( (
 ( 1.000000000000000000, 0.8660254037844387076, 1.000000000000000000, 0.8660254037844387076, 1.000000000000000000, 0.8660254037844387076, 1.000000000000000000, 0.8660254037844387076, 1.000000000000000000, 0.8660254037844387076, 1.000000000000000000, 0.8660254037844387076, 1.000000000000000000, 0.8660254037844387076, 1.000000000000000000, 0.8660254037844387076, 1.000000000000000000, 0.8660254037844387076, 1.000000000000000000, 0.8660254037844387076, 1.000000000000000000, 0.8660254037844387076, 1.000000000000000000, 0.8660254037844387076, 1.000000000000000000, 0.8660254037844387076, 1.000000000000000000, 0.8660254037844387076, 1.000000000000000000, 0.8660254037844387076, 1.000000000000000000, 0.8660254037844387076, 1.000000000000000000, 0.8660254037844387076, 1.000000000000000000, 0.8660254037844387076, 1.000000000000000000, 0.8660254037844387076, 1.000000000000000000, 0.8660254037844387076, 1.000000000000000000, 0.8660254037844387076, 1.000000000000000000, 0.8660254037844387076, 1.000000000000000000, 0.8660254037844387076, 1.000000000000000000, 0.8660254037844387076, 1.000000000000000000, 0.8660254037844387076, 1.000000000000000000, 0.8660254037844387076, 1.000000000000000000, 0.8660254037844387076, 1.000000000000000000, 0.8660254037844387076, 1.000000000000000000, 0.8660254037844387076, 1.000000000000000000, 0.8660254037844387076, 1.000000000000000000, 0.8660254037844387076, 1.000000000000000000, 0.8660254037844387076, 1.000000000000000000, 0.8660254037844387076, 1.000000000000000000, 0.8660254037844387076, 1.000000000000000000, 0.8660254037844387076, 1.000000000000000000, 0.8660254037844387076, 1.000000000000000000, 0.8660254037844387076, 1.000000000000000000, 0.8660254037844387076, 1.000000000000000000, 0.8660254037844387076, 1.000000000000000000, 0.8660254037844387076, 1.000000000000000000, 0.8660254037844387076, 1.000000000000000000, 0.8660254037844387076, 1.000000000000000000, 0.8660254037844387076, 1.000000000000000000, 0.8660254037844387076, 1.000000000000000000, 0.8660254037844387076, 1.000000000000000000, 0.8660254037844387076, 1.000000000000000000, 0.8660254037844387076, 1.000000000000000000, 0.8660254037844387076, 1.000000000000000000, 0.8660254037844387076, 1.000000000000000000, 0.8660254037844387076, 1.000000000000000000, 0.8660254037844387076, 1.000000000000000000, 0.8660254037844387076, 1.000000000000000000, 0.8660254037844387076, 1.000000000000000000, 0.8660254037844387076, 1.000000000000000000, 0.8660254037844387076, 1.000000000000000000, 0.8660254037844387076, 1.000000000000000000, 0.8660254037844387076, 1.000000000000000000, 0.8660254037844387076, 1.000000000000000000, 0.8660254037844387076, 1.000000000000000000, 0.8660254037844387076, 1.000000000000000000, 0.8660254037844387076, 1.000000000000000000, 0.8660254037844387076, 1.000000000000000000, 0.8660254037844387076, 1.000000000000000000, 0.8660254037844387076, 1.000000000000000000, 0.8660254037844387076, 1.000000000000000000, 0.8660254037844387076, 1.000000000000000000, 0.8660254037844387076, 1.000000000000000000, 0.8660254037844387076, 1.000000000000000000, 0.8660254037844387076, 1.000000000000000000, 0.8660254037844387076, 1.000000000000000000, 0.8660254037844387076, 1.000000000000000000, 0.8660254037844387076, 1.000000000000000000, 0.8660254037844387076, 1.000000000000000000, 0.8660254037844387076, 1.000000000000000000, 0.8660254037844387076, 1.000000000000000000, 0.8660254037844387076, 1.000000000000000000, 0.8660254037844387076, 1.000000000000000000, 0.8660254037844387076, 1.000000000000000000, 0.8660254037844387076, 1.000000000000000000, 0.8660254037844387076, 1.000000000000000000, 0.8660254037844387076, 1.000000000000000000, 0.8660254037844387076, 1.000000000000000000, 0.8660254037844387076, 1.000000000000000000, 0.8660254037844387076, 1.000000000000000000, 0.8660254037844387076, 1.000000000000000000, 0.8660254037844387076, 1.000000000000000000, 0.8660254037844387076, 1.000000000000000000, 0.8660254037844387076, 1.000000000000000000, 0.8660254037844387076, 1.000000000000000000, 0.8660254037844387076, 1.000000000000000000, 0.8660254037844387076, 1.000000000000000000, 0.8660254037844387076, 1.000000000000000000, 0.8660254037844387076, 1.000000000000000000, 0.8660254037844387076, 1.000000000000000000, 0.8660254037844387076, 1.000000000000000000, 0.8660254037844387076, 1.000000000000000000, 0.8660254037844387076, 1.000000000000000000, 0.8660254037844387076, 1.000000000000000000, 0.8660254037844387076, 1.000000000000000000, 0.8660254037844387076, 1.000000000000000000, 0.8660254037844387076, 1.000000000000000000, 0.8660254037844387076, 1.000000000000000000, 0.8660254037844387076, 1.000000000000000000, 0.8660254037844387076, 1.000000000000000000, 0.8660254037844387076, 1.000000000000000000, 0.8660254037844387076, 1.000000000000000000, 0.8660254037844387076, 1.000000000000000000, 0.8660254037844387076, 1.000000000000000000, 0.8660254037844387076, 1.000000000000000000, 0.8660254037844387076, 1.000000000000000000, 0.8660254037844387076, 1.000000000000000000, 0.8660254037844387076, 1.000000000000000000, 0.8660254037844387076, 1.000000000000000000, 0.8660254037844387076, 1.000000000000000000, 0.8660254037844387076, 1.000000000000000000, 0.8660254037844387076, 1.000000000000000000, 0.8660254037844387076, 1.000000000000000000, 0.8660254037844387076, 1.000000000000000000, 0.8660254037844387076, 1.000000000000000000, 0.8660254037844387076, 1.000000000000000000, 0.8660254037844387076, 1.000000000000000000, 0.8660254037844387076, 1.000000000000000000, 0.8660254037844387076, 1.000000000000000000, 0.8660254037844387076, 1.000000000000000000, 0.8660254037844387076, 1.000000000000000000, 0.8660254037844387076, 1.000000000000000000, 0.8660254037844387076, 1.000000000000000000, 0.8660254037844387076, 1.000000000000000000, 0.8660254037844387076, 1.000000000000000000, 0.8660254037844387076, 1.000000000000000000, 0.8660254037844387076, 1.000000000000000000, 0.8660254037844387076, 1.000000000000000000, 0.8660254037844387076, 1.000000000000000000, 0.8660254037844387076, 1.000000000000000000, 0.8660254037844387076, 1.000000000000000000, 0.8660254037844387076, 1.000000000000000000, 0.8660254037844387076, 1.000000000000000000, 0.8660254037844387076, 1.000000000000000000, 0.8660254037844387076, 1.000000000000000000, 0.8660254037844387076, 1.000000000000000000, 0.8660254037844387076, 1.000000000000000000, 0.8660254037844387076, 1.000000000000000000, 0.8660254037844387076, 1.000000000000000000, 0.8660254037844387076, 1.000000000000000000, 0.8660254037844387076, 1.000000000000000000, 0.8660254037844387076, 1.000000000000000000, 0.8660254037844387076, 1.000000000000000000, 0.8660254037844387076, 1.000000000000000000, 0.8660254037844387076, 1.000000000000000000, 0.8660254037844387076, 1.000000000000000000, 0.8660254037844387076, 1.000000000000000000, 0.8660254037844387076, 1.000000000000000000, 0.8660254037844387076, 1.000000000000000000, 0.8660254037844387076, 1.000000000000000000, 0.8660254037844387076, 1.000000000000000000, 0.8660254037844387076, 1.000000000000000000, 0.8660254037844387076, 1.000000000000000000, 0.8660254037844387076, 1.000000000000000000, 0.8660254037844387076, 1.000000000000000000, 0.8660254037844387076, 1.000000000000000000, 0.8660254037844387076, 1.000000000000000000, 0.8660254037844387076, 1.000000000000000000, 0.8660254037844387076, 1.000000000000000000, 0.8660254037844387076, 1.000000000000000000, 0.8660254037844387076, 1.000000000000000000, 0.8660254037844387076, 1.000000000000000000, 0.8660254037844387076, 1.000000000000000000, 0.8660254037844387076, 1.000000000000000000, 0.8660254037844387076, 1.000000000000000000, 0.8660254037844387076, 1.000000000000000000, 0.8660254037844387076, 1.000000000000000000, 0.8660254037844387076, 1.000000000000000000, 0.8660254037844387076, 1.000000000000000000, 0.8660254037844387076, 1.000000000000000000, 0.8660254037844387076, 1.000000000000000000, 0.8660254037844387076, 1.000000000000000000, 0.8660254037844387076, 1.000000000000000000, 0.8660254037844387076, 1.000000000000000000, 0.8660254037844387076, 1.000000000000000000, 0.8660254037844387076, 1.000000000000000000, 0.8660254037844387076, 1.000000000000000000, 0.8660254037844387076, 1.000000000000000000, 0.8660254037844387076, 1.000000000000000000, 0.8660254037844387076, 1.000000000000000000, 0.8660254037844387076, 1.000000000000000000, 0.8660254037844387076, 1.000000000000000000, 0.8660254037844387076, 1.000000000000000000, 0.8660254037844387076, 1.000000000000000000, 0.8660254037844387076, 1.000000000000000000, 0.8660254037844387076, 1.000000000000000000, 0.8660254037844387076, 1.000000000000000000, 0.8660254037844387076, 1.000000000000000000, 0.8660254037844387076, 1.000000000000000000, 0.8660254037844387076, 1.000000000000000000, 0.8660254037844387076, 1.000000000000000000, 0.8660254037844387076, 1.000000000000000000, 0.8660254037844387076, 1.000000000000000000, 0.8660254037844387076, 1.000000000000000000, 0.8660254037844387076, 1.000000000000000000, 0.8660254037844387076, 1.000000000000000000, 0.8660254037844387076, 1.000000000000000000, 0.8660254037844387076, 1.000000000000000000, 0.8660254037844387076, 1.000000000000000000, 0.8660254037844387076, 1.000000000000000000, 0.8660254037844387076, 1.000000000000000000, 0.8660254037844387076, 1.000000000000000000, 0.8660254037844387076, 1.000000000000000000, 0.8660254037844387076, 1.000000000000000000, 0.8660254037844387076, 1.000000000000000000, 0.8660254037844387076, 1.000000000000000000, 0.8660254037844387076, 1.000000000000000000, 0.8660254037844387076, 1.000000000000000000, 0.8660254037844387076, 1.000000000000000000, 0.8660254037844387076, 1.000000000000000000, 0.8660254037844387076, 1.000000000000000000, 0.8660254037844387076, 1.000000000000000000, 0.8660254037844387076, 1.000000000000000000, 0.8660254037844387076, 1.000000000000000000, 0.8660254037844387076, 1.000000000000000000, 0.8660254037844387076, 1.000000000000000000, 0.8660254037844387076, 1.000000000000000000, 0.8660254037844387076, 1.000000000000000000, 0.8660254037844387076, 1.000000000000000000, 0.8660254037844387076, 1.000000000000000000, 0.8660254037844387076, 1.000000000000000000, 0.8660254037844387076, 1.000000000000000000, 0.8660254037844387076, 1.000000000000000000, 0.8660254037844387076, 1.000000000000000000, 0.8660254037844387076, 1.000000000000000000, 0.8660254037844387076, 1.000000000000000000, 0.8660254037844387076, 1.000000000000000000, 0.8660254037844387076, 1.000000000000000000, 0.8660254037844387076, 1.000000000000000000, 0.8660254037844387076, 1.000000000000000000, 0.8660254037844387076, 1.000000000000000000, 0.8660254037844387076, 1.000000000000000000, 0.8660254037844387076, 1.000000000000000000, 0.8660254037844387076, 1.000000000000000000, 0.8660254037844387076, 1.000000000000000000, 0.8660254037844387076, 1.000000000000000000, 0.8660254037844387076, 1.000000000000000000, 0.8660254037844387076, 1.000000000000000000, 0.8660254037844387076, 1.000000000000000000, 0.8660254037844387076, 1.000000000000000000, 0.8660254037844387076, 1.000000000000000000, 0.8660254037844387076, 1.000000000000000000, 0.8660254037844387076, 1.000000000000000000, 0.8660254037844387076, 1.000000000000000000, 0.8660254037844387076, 1.000000000000000000, 0.8660254037844387076, 1.000000000000000000, 0.8660254037844387076, 1.000000000000000000, 0.8660254037844387076, 1.000000000000000000, 0.8660254037844387076, 1.000000000000000000, 0.8660254037844387076, 1.000000000000000000, 0.8660254037844387076, 1.000000000000000000, 0.8660254037844387076, 1.000000000000000000, 0.8660254037844387076, 1.000000000000000000, 0.8660254037844387076, 1.000000000000000000, 0.8660254037844387076, 1.000000000000000000, 0.8660254037844387076, 1.000000000000000000, 0.8660254037844387076, 1.000000000000000000, 0.8660254037844387076, 1.000000000000000000, 0.8660254037844387076, 1.000000000000000000, 0.8660254037844387076, 1.000000000000000000, 0.8660254037844387076, 1.000000000000000000, 0.8660254037844387076, 1.000000000000000000, 0.8660254037844387076, 1.000000000000000000, 0.8660254037844387076, 1.000000000000000000, 0.8660254037844387076, 1.000000000000000000, 0.8660254037844387076, 1.000000000000000000, 0.8660254037844387076, 1.000000000000000000, 0.8660254037844387076, 1.000000000000000000, 0.8660254037844387076, 1.000000000000000000, 0.8660254037844387076, 1.000000000000000000, 0.8660254037844387076, 1.000000000000000000, 0.8660254037844387076, 1.000000000000000000, 0.8660254037844387076, 1.000000000000000000, 0.8660254037844387076, 1.000000000000000000, 0.8660254037844387076, 1.000000000000000000, 0.8660254037844387076, 1.000000000000000000, 0.8660254037844387076, 1.000000000000000000, 0.8660254037844387076, 1.000000000000000000, 0.8660254037844387076, 1.000000000000000000, 0.8660254037844387076, 1.000000000000000000, 0.8660254037844387076, 1.000000000000000000, 0.8660254037844387076, 1.000000000000000000, 0.8660254037844387076, 1.000000000000000000, 0.8660254037844387076, 1.000000000000000000, 0.8660254037844387076, 1.000000000000000000, 0.8660254037844387076, 1.000000000000000000, 0.8660254037844387076, 1.000000000000000000, 0.8660254037844387076, 1.000000000000000000, 0.8660254037844387076, 1.000000000000000000, 0.8660254037844387076, 1.000000000000000000, 0.8660254037844387076, 1.000000000000000000, 0.8660254037844387076, 1.000000000000000000, 0.8660254037844387076, 1.000000000000000000, 0.8660254037844387076, 1.000000000000000000, 0.8660254037844387076, 1.000000000000000000, 0.8660254037844387076, 1.000000000000000000, 0.8660254037844387076, 1.000000000000000000, 0.8660254037844387076, 1.000000000000000000, 0.8660254037844387076, 1.000000000000000000, 0.8660254037844387076, 1.000000000000000000, 0.8660254037844387076, 1.000000000000000000, 0.8660254037844387076, 1.000000000000000000, 0.8660254037844387076, 1.000000000000000000, 0.8660254037844387076, 1.000000000000000000, 0.8660254037844387076, 1.000000000000000000, 0.8660254037844387076, 1.000000000000000000, 0.8660254037844387076, 1.000000000000000000, 0.8660254037844387076, 1.000000000000000000, 0.8660254037844387076, 1.000000000000000000, 0.8660254037844387076, 1.000000000000000000, 0.8660254037844387076, 1.000000000000000000, 0.8660254037844387076, 1.000000000000000000, 0.8660254037844387076, 1.000000000000000000, 0.8660254037844387076, 1.000000000000000000, 0.8660254037844387076, 1.000000000000000000, 0.8660254037844387076, 1.000000000000000000, 0.8660254037844387076, 1.000000000000000000, 0.8660254037844387076, 1.000000000000000000, 0.8660254037844387076, 1.000000000000000000, 0.8660254037844387076, 1.000000000000000000, 0.8660254037844387076, 1.000000000000000000, 0.8660254037844387076, 1.000000000000000000, 0.8660254037844387076, 1.000000000000000000, 0.8660254037844387076, 1.000000000000000000, 0.8660254037844387076, 1.000000000000000000, 0.8660254037844387076, 1.000000000000000000, 0.8660254037844387076, 1.000000000000000000, 0.8660254037844387076, 1.000000000000000000, 0.8660254037844387076, 1.000000000000000000, 0.8660254037844387076, 1.000000000000000000, 0.8660254037844387076, 1.000000000000000000, 0.8660254037844387076, 1.000000000000000000, 0.8660254037844387076, 1.000000000000000000, 0.8660254037844387076, 1.000000000000000000, 0.8660254037844387076, 1.000000000000000000, 0.8660254037844387076, 1.000000000000000000, 0.8660254037844387076, 1.000000000000000000, 0.8660254037844387076, 1.000000000000000000, 0.8660254037844387076, 1.000000000000000000, 0.8660254037844387076, 1.000000000000000000, 0.8660254037844387076, 1.000000000000000000, 0.8660254037844387076, 1.000000000000000000, 0.8660254037844387076, 1.000000000000000000, 0.8660254037844387076, 1.000000000000000000, 0.8660254037844387076, 1.000000000000000000, 0.8660254037844387076, 1.000000000000000000, 0.8660254037844387076, 1.000000000000000000, 0.8660254037844387076, 1.000000000000000000, 0.8660254037844387076, 1.000000000000000000, 0.8660254037844387076, 1.000000000000000000, 0.8660254037844387076, 1.000000000000000000, 0.8660254037844387076, 1.000000000000000000, 0.8660254037844387076, 1.000000000000000000, 0.8660254037844387076, 1.000000000000000000, 0.8660254037844387076, 1.000000000000000000, 0.8660254037844387076, 1.000000000000000000, 0.8660254037844387076, 1.000000000000000000, 0.8660254037844387076, 1.000000000000000000, 0.8660254037844387076, 1.000000000000000000, 0.8660254037844387076, 1.000000000000000000, 0.8660254037844387076, 1.000000000000000000, 0.8660254037844387076, 1.000000000000000000, 0.8660254037844387076, 1.000000000000000000, 0.8660254037844387076, 1.000000000000000000, 0.8660254037844387076, 1.000000000000000000, 0.8660254037844387076, 1.000000000000000000, 0.8660254037844387076, 1.000000000000000000, 0.8660254037844387076, 1.000000000000000000, 0.8660254037844387076, 1.000000000000000000, 0.8660254037844387076, 1.000000000000000000, 0.8660254037844387076, 1.000000000000000000, 0.8660254037844387076, 1.000000000000000000, 0.8660254037844387076, 1.000000000000000000, 0.8660254037844387076, 1.000000000000000000, 0.8660254037844387076, 1.000000000000000000, 0.8660254037844387076, 1.000000000000000000, 0.8660254037844387076, 1.000000000000000000, 0.8660254037844387076, 1.000000000000000000, 0.8660254037844387076, 1.000000000000000000, 0.8660254037844387076, 1.000000000000000000, 0.8660254037844387076, 1.000000000000000000, 0.8660254037844387076, 1.000000000000000000, 0.8660254037844387076, 1.000000000000000000, 0.8660254037844387076, 1.000000000000000000, 0.8660254037844387076, 1.000000000000000000, 0.8660254037844387076, 1.000000000000000000, 0.8660254037844387076, 1.000000000000000000, 0.8660254037844387076, 1.000000000000000000, 0.8660254037844387076, 1.000000000000000000, 0.8660254037844387076, 1.000000000000000000, 0.8660254037844387076, 1.000000000000000000, 0.8660254037844387076, 1.000000000000000000, 0.8660254037844387076, 1.000000000000000000, 0.8660254037844387076, 1.000000000000000000, 0.8660254037844387076, 1.000000000000000000, 0.8660254037844387076, 1.000000000000000000, 0.8660254037844387076, 1.000000000000000000, 0.8660254037844387076, 1.000000000000000000, 0.8660254037844387076, 1.000000000000000000, 0.8660254037844387076, 1.000000000000000000, 0.8660254037844387076, 1.000000000000000000, 0.8660254037844387076, 1.000000000000000000, 0.8660254037844387076, 1.000000000000000000, 0.8660254037844387076, 1.000000000000000000, 0.8660254037844387076, 1.000000000000000000, 0.8660254037844387076, 1.000000000000000000, 0.8660254037844387076, 1.000000000000000000, 0.8660254037844387076, 1.000000000000000000, 0.8660254037844387076, 1.000000000000000000, 0.8660254037844387076, 1.000000000000000000, 0.8660254037844387076, 1.000000000000000000, 0.8660254037844387076, 1.000000000000000000, 0.8660254037844387076, 1.000000000000000000, 0.8660254037844387076, 1.000000000000000000, 0.8660254037844387076, 1.000000000000000000, 0.8660254037844387076, 1.000000000000000000, 0.8660254037844387076, 1.000000000000000000, 0.8660254037844387076, 1.000000000000000000, 0.8660254037844387076, 1.000000000000000000, 0.8660254037844387076, 1.000000000000000000, 0.8660254037844387076, 1.000000000000000000, 0.8660254037844387076, 1.000000000000000000, 0.8660254037844387076, 1.000000000000000000, 0.8660254037844387076, 1.000000000000000000, 0.8660254037844387076, 1.000000000000000000, 0.8660254037844387076, 1.000000000000000000, 0.8660254037844387076, 1.000000000000000000, 0.8660254037844387076, 1.000000000000000000, 0.8660254037844387076, 1.000000000000000000, 0.8660254037844387076, 1.000000000000000000, 0.8660254037844387076, 1.000000000000000000, 0.8660254037844387076, 1.000000000000000000, 0.8660254037844387076, 1.000000000000000000, 0.8660254037844387076, 1.000000000000000000, 0.8660254037844387076, 1.000000000000000000, 0.8660254037844387076, 1.000000000000000000, 0.8660254037844387076, 1.000000000000000000, 0.8660254037844387076, 1.000000000000000000, 0.8660254037844387076, 1.000000000000000000, 0.8660254037844387076, 1.000000000000000000, 0.8660254037844387076, 1.000000000000000000, 0.8660254037844387076, 1.000000000000000000, 0.8660254037844387076, 1.000000000000000000, 0.8660254037844387076, 1.000000000000000000, 0.8660254037844387076, 1.000000000000000000, 0.8660254037844387076, 1.000000000000000000, 0.8660254037844387076, 1.000000000000000000, 0.8660254037844387076, 1.000000000000000000, 0.8660254037844387076, 1.000000000000000000, 0.8660254037844387076, 1.000000000000000000, 0.8660254037844387076, 1.000000000000000000, 0.8660254037844387076, 1.000000000000000000, 0.8660254037844387076, 1.000000000000000000, 0.8660254037844387076, 1.000000000000000000, 0.8660254037844387076, 1.000000000000000000, 0.8660254037844387076, 1.000000000000000000, 0.8660254037844387076, 1.000000000000000000, 0.8660254037844387076, 1.000000000000000000, 0.8660254037844387076, 1.000000000000000000, 0.8660254037844387076, 1.000000000000000000, 0.8660254037844387076, 1.000000000000000000, 0.8660254037844387076, 1.000000000000000000, 0.8660254037844387076, 1.000000000000000000, 0.8660254037844387076, 1.000000000000000000, 0.8660254037844387076, 1.000000000000000000, 0.8660254037844387076, 1.000000000000000000, 0.8660254037844387076, 1.000000000000000000, 0.8660254037844387076, 1.000000000000000000, 0.8660254037844387076, 1.000000000000000000, 0.8660254037844387076, 1.000000000000000000, 0.8660254037844387076, 1.000000000000000000, 0.8660254037844387076, 1.000000000000000000, 0.8660254037844387076, 1.000000000000000000, 0.8660254037844387076, 1.000000000000000000, 0.8660254037844387076, 1.000000000000000000, 0.8660254037844387076, 1.000000000000000000, 0.8660254037844387076, 1.000000000000000000, 0.8660254037844387076, 1.000000000000000000, 0.8660254037844387076, 1.000000000000000000, 0.8660254037844387076, 1.000000000000000000, 0.8660254037844387076, 1.000000000000000000, 0.8660254037844387076, 1.000000000000000000, 0.8660254037844387076, 1.000000000000000000, 0.8660254037844387076, 1.000000000000000000, 0.8660254037844387076, 1.000000000000000000, 0.8660254037844387076, 1.000000000000000000, 0.8660254037844387076, 1.000000000000000000, 0.8660254037844387076, 1.000000000000000000, 0.8660254037844387076, 1.000000000000000000, 0.8660254037844387076, 1.000000000000000000, 0.8660254037844387076, 1.000000000000000000, 0.8660254037844387076, 1.000000000000000000, 0.8660254037844387076, 1.000000000000000000, 0.8660254037844387076, 1.000000000000000000, 0.8660254037844387076, 1.000000000000000000, 0.8660254037844387076, 1.000000000000000000, 0.8660254037844387076, 1.000000000000000000, 0.8660254037844387076, 1.000000000000000000, 0.8660254037844387076, 1.000000000000000000, 0.8660254037844387076, 1.000000000000000000, 0.8660254037844387076, 1.000000000000000000, 0.8660254037844387076, 1.000000000000000000, 0.8660254037844387076, 1.000000000000000000, 0.8660254037844387076, 1.000000000000000000, 0.8660254037844387076, 1.000000000000000000, 0.8660254037844387076, 1.000000000000000000, 0.8660254037844387076, 1.000000000000000000, 0.8660254037844387076, 1.000000000000000000, 0.8660254037844387076, 1.000000000000000000, 0.8660254037844387076, 1.000000000000000000, 0.8660254037844387076, 1.000000000000000000, 0.8660254037844387076, 1.000000000000000000, 0.8660254037844387076, 1.000000000000000000, 0.8660254037844387076, 1.000000000000000000, 0.8660254037844387076, 1.000000000000000000, 0.8660254037844387076, 1.000000000000000000, 0.8660254037844387076, 1.000000000000000000, 0.8660254037844387076, 1.000000000000000000, 0.8660254037844387076, 1.000000000000000000, 0.8660254037844387076, 1.000000000000000000, 0.8660254037844387076, 1.000000000000000000, 0.8660254037844387076, 1.000000000000000000, 0.8660254037844387076, 1.000000000000000000, 0.8660254037844387076, 1.000000000000000000, 0.8660254037844387076, 1.000000000000000000, 0.8660254037844387076, 1.000000000000000000, 0.8660254037844387076, 1.000000000000000000, 0.8660254037844387076, 1.000000000000000000, 0.8660254037844387076, 1.000000000000000000, 0.8660254037844387076, 1.000000000000000000, 0.8660254037844387076, 1.000000000000000000, 0.8660254037844387076, 1.000000000000000000, 0.8660254037844387076, 1.000000000000000000, 0.8660254037844387076, 1.000000000000000000, 0.8660254037844387076, 1.000000000000000000, 0.8660254037844387076, 1.000000000000000000, 0.8660254037844387076, 1.000000000000000000, 0.8660254037844387076, 1.000000000000000000, 0.8660254037844387076, 1.000000000000000000, 0.8660254037844387076, 1.000000000000000000, 0.8660254037844387076, 1.000000000000000000, 0.8660254037844387076, 1.000000000000000000, 0.8660254037844387076, 1.000000000000000000, 0.8660254037844387076, 1.000000000000000000, 0.8660254037844387076, 1.000000000000000000, 0.8660254037844387076, 1.000000000000000000, 0.8660254037844387076, 1.000000000000000000, 0.8660254037844387076, 1.000000000000000000, 0.8660254037844387076, 1.000000000000000000, 0.8660254037844387076, 1.000000000000000000, 0.8660254037844387076, 1.000000000000000000, 0.8660254037844387076, 1.000000000000000000, 0.8660254037844387076, 1.000000000000000000, 0.8660254037844387076, 1.000000000000000000, 0.8660254037844387076, 1.000000000000000000, 0.8660254037844387076, 1.000000000000000000, 0.8660254037844387076, 1.000000000000000000, 0.8660254037844387076, 1.000000000000000000, 0.8660254037844387076, 1.000000000000000000, 0.8660254037844387076, 1.000000000000000000, 0.8660254037844387076, 1.000000000000000000, 0.8660254037844387076, 1.000000000000000000, 0.8660254037844387076, 1.000000000000000000, 0.8660254037844387076, 1.000000000000000000, 0.8660254037844387076, 1.000000000000000000, 0.8660254037844387076, 1.000000000000000000, 0.8660254037844387076, 1.000000000000000000, 0.8660254037844387076, 1.000000000000000000, 0.8660254037844387076, 1.000000000000000000, 0.8660254037844387076, 1.000000000000000000, 0.8660254037844387076, 1.000000000000000000, 0.8660254037844387076, 1.000000000000000000, 0.8660254037844387076, 1.000000000000000000, 0.8660254037844387076, 1.000000000000000000, 0.8660254037844387076, 1.000000000000000000, 0.8660254037844387076, 1.000000000000000000, 0.8660254037844387076, 1.000000000000000000, 0.8660254037844387076, 1.000000000000000000, 0.8660254037844387076, 1.000000000000000000, 0.8660254037844387076, 1.000000000000000000, 0.8660254037844387076, 1.000000000000000000, 0.8660254037844387076, 1.000000000000000000, 0.8660254037844387076, 1.000000000000000000, 0.8660254037844387076, 1.000000000000000000, 0.8660254037844387076, 1.000000000000000000, 0.8660254037844387076, 1.000000000000000000, 0.8660254037844387076, 1.000000000000000000, 0.8660254037844387076, 1.000000000000000000, 0.8660254037844387076, 1.000000000000000000, 0.8660254037844387076, 1.000000000000000000, 0.8660254037844387076, 1.000000000000000000, 0.8660254037844387076, 1.000000000000000000, 0.8660254037844387076, 1.000000000000000000, 0.8660254037844387076, 1.000000000000000000, 0.8660254037844387076, 1.000000000000000000, 0.8660254037844387076, 1.000000000000000000, 0.8660254037844387076, 1.000000000000000000, 0.8660254037844387076, 1.000000000000000000, 0.8660254037844387076, 1.000000000000000000, 0.8660254037844387076, 1.000000000000000000, 0.8660254037844387076, 1.000000000000000000, 0.8660254037844387076, 1.000000000000000000, 0.8660254037844387076, 1.000000000000000000, 0.8660254037844387076, 1.000000000000000000, 0.8660254037844387076, 1.000000000000000000, 0.8660254037844387076, 1.000000000000000000, 0.8660254037844387076, 1.000000000000000000, 0.8660254037844387076, 1.000000000000000000, 0.8660254037844387076, 1.000000000000000000, 0.8660254037844387076, 1.000000000000000000, 0.8660254037844387076, 1.000000000000000000, 0.8660254037844387076, 1.000000000000000000, 0.8660254037844387076, 1.000000000000000000, 0.8660254037844387076, 1.000000000000000000, 0.8660254037844387076, 1.000000000000000000, 0.8660254037844387076, 1.000000000000000000, 0.8660254037844387076, 1.000000000000000000, 0.8660254037844387076, 1.000000000000000000, 0.8660254037844387076, 1.000000000000000000, 0.8660254037844387076, 1.000000000000000000, 0.8660254037844387076, 1.000000000000000000, 0.8660254037844387076, 1.000000000000000000, 0.8660254037844387076, 1.000000000000000000, 0.8660254037844387076, 1.000000000000000000, 0.8660254037844387076, 1.000000000000000000, 0.8660254037844387076, 1.000000000000000000, 0.8660254037844387076, 1.000000000000000000, 0.8660254037844387076, 1.000000000000000000, 0.8660254037844387076, 1.000000000000000000, 0.8660254037844387076, 1.000000000000000000, 0.8660254037844387076, 1.000000000000000000, 0.8660254037844387076, 1.000000000000000000, 0.8660254037844387076, 1.000000000000000000, 0.8660254037844387076, 1.000000000000000000, 0.8660254037844387076, 1.000000000000000000, 0.8660254037844387076, 1.000000000000000000, 0.8660254037844387076, 1.000000000000000000, 0.8660254037844387076, 1.000000000000000000, 0.8660254037844387076, 1.000000000000000000, 0.8660254037844387076, 1.000000000000000000, 0.8660254037844387076, 1.000000000000000000, 0.8660254037844387076, 1.000000000000000000, 0.8660254037844387076, 1.000000000000000000, 0.8660254037844387076, 1.000000000000000000, 0.8660254037844387076, 1.000000000000000000, 0.8660254037844387076, 1.000000000000000000, 0.8660254037844387076, 1.000000000000000000, 0.8660254037844387076, 1.000000000000000000, 0.8660254037844387076, 1.000000000000000000, 0.8660254037844387076, 1.000000000000000000, 0.8660254037844387076, 1.000000000000000000, 0.8660254037844387076, 1.000000000000000000, 0.8660254037844387076, 1.000000000000000000, 0.8660254037844387076, 1.000000000000000000, 0.8660254037844387076, 1.000000000000000000, 0.8660254037844387076, 1.000000000000000000, 0.8660254037844387076, 1.000000000000000000, 0.8660254037844387076, 1.000000000000000000, 0.8660254037844387076, 1.000000000000000000, 0.8660254037844387076, 1.000000000000000000, 0.8660254037844387076, 1.000000000000000000, 0.8660254037844387076, 1.000000000000000000, 0.8660254037844387076, 1.000000000000000000, 0.8660254037844387076, 1.000000000000000000, 0.8660254037844387076, 1.000000000000000000, 0.8660254037844387076, 1.000000000000000000, 0.8660254037844387076, 1.000000000000000000, 0.8660254037844387076, 1.000000000000000000, 0.8660254037844387076, 1.000000000000000000, 0.8660254037844387076, 1.000000000000000000, 0.8660254037844387076, 1.000000000000000000, 0.8660254037844387076, 1.000000000000000000, 0.8660254037844387076, 1.000000000000000000, 0.8660254037844387076, 1.000000000000000000, 0.8660254037844387076, 1.000000000000000000, 0.8660254037844387076, 1.000000000000000000, 0.8660254037844387076, 1.000000000000000000, 0.8660254037844387076, 1.000000000000000000, 0.8660254037844387076, 1.000000000000000000, 0.8660254037844387076, 1.000000000000000000, 0.8660254037844387076, 1.000000000000000000, 0.8660254037844387076, 1.000000000000000000, 0.8660254037844387076, 1.000000000000000000, 0.8660254037844387076, 1.000000000000000000, 0.8660254037844387076, 1.000000000000000000, 0.8660254037844387076, 1.000000000000000000, 0.8660254037844387076, 1.000000000000000000, 0.8660254037844387076, 1.000000000000000000, 0.8660254037844387076, 1.000000000000000000, 0.8660254037844387076, 1.000000000000000000, 0.8660254037844387076, 1.000000000000000000, 0.8660254037844387076, 1.000000000000000000, 0.8660254037844387076, 1.000000000000000000, 0.8660254037844387076, 1.000000000000000000, 0.8660254037844387076, 1.000000000000000000, 0.8660254037844387076, 1.000000000000000000, 0.8660254037844387076, 1.000000000000000000, 0.8660254037844387076, 1.000000000000000000, 0.8660254037844387076, 1.000000000000000000, 0.8660254037844387076, 1.000000000000000000, 0.8660254037844387076, 1.000000000000000000, 0.8660254037844387076, 1.000000000000000000, 0.8660254037844387076, 1.000000000000000000, 0.8660254037844387076, 1.000000000000000000, 0.8660254037844387076, 1.000000000000000000, 0.8660254037844387076, 1.000000000000000000, 0.8660254037844387076, 1.000000000000000000, 0.8660254037844387076, 1.000000000000000000, 0.8660254037844387076, 1.000000000000000000, 0.8660254037844387076, 1.000000000000000000, 0.8660254037844387076, 1.000000000000000000, 0.8660254037844387076, 1.000000000000000000, 0.8660254037844387076, 1.000000000000000000, 0.8660254037844387076, 1.000000000000000000, 0.8660254037844387076, 1.000000000000000000, 0.8660254037844387076, 1.000000000000000000),
 ( 1.000000000000000000, 0.8660254037844387076, 1.000000000000000000, 0.8660254037844387076, 1.000000000000000000, 0.8660254037844387076, 1.000000000000000000, 0.8660254037844387076, 1.000000000000000000, 0.8660254037844387076, 1.000000000000000000, 0.8660254037844387076, 1.000000000000000000, 0.8660254037844387076, 1.000000000000000000, 0.8660254037844387076, 1.000000000000000000, 0.8660254037844387076, 1.000000000000000000, 0.8660254037844387076, 1.000000000000000000, 0.8660254037844387076, 1.000000000000000000, 0.8660254037844387076, 1.000000000000000000, 0.8660254037844387076, 1.000000000000000000, 0.8660254037844387076, 1.000000000000000000, 0.8660254037844387076, 1.000000000000000000, 0.8660254037844387076, 1.000000000000000000, 0.8660254037844387076, 1.000000000000000000, 0.8660254037844387076, 1.000000000000000000, 0.8660254037844387076, 1.000000000000000000, 0.8660254037844387076, 1.000000000000000000, 0.8660254037844387076, 1.000000000000000000, 0.8660254037844387076, 1.000000000000000000, 0.8660254037844387076, 1.000000000000000000, 0.8660254037844387076, 1.000000000000000000, 0.8660254037844387076, 1.000000000000000000, 0.8660254037844387076, 1.000000000000000000, 0.8660254037844387076, 1.000000000000000000, 0.8660254037844387076, 1.000000000000000000, 0.8660254037844387076, 1.000000000000000000, 0.8660254037844387076, 1.000000000000000000, 0.8660254037844387076, 1.000000000000000000, 0.8660254037844387076, 1.000000000000000000, 0.8660254037844387076, 1.000000000000000000, 0.8660254037844387076, 1.000000000000000000, 0.8660254037844387076, 1.000000000000000000, 0.8660254037844387076, 1.000000000000000000, 0.8660254037844387076, 1.000000000000000000, 0.8660254037844387076, 1.000000000000000000, 0.8660254037844387076, 1.000000000000000000, 0.8660254037844387076, 1.000000000000000000, 0.8660254037844387076, 1.000000000000000000, 0.8660254037844387076, 1.000000000000000000, 0.8660254037844387076, 1.000000000000000000, 0.8660254037844387076, 1.000000000000000000, 0.8660254037844387076, 1.000000000000000000, 0.8660254037844387076, 1.000000000000000000, 0.8660254037844387076, 1.000000000000000000, 0.8660254037844387076, 1.000000000000000000, 0.8660254037844387076, 1.000000000000000000, 0.8660254037844387076, 1.000000000000000000, 0.8660254037844387076, 1.000000000000000000, 0.8660254037844387076, 1.000000000000000000, 0.8660254037844387076, 1.000000000000000000, 0.8660254037844387076, 1.000000000000000000, 0.8660254037844387076, 1.000000000000000000, 0.8660254037844387076, 1.000000000000000000, 0.8660254037844387076, 1.000000000000000000, 0.8660254037844387076, 1.000000000000000000, 0.8660254037844387076, 1.000000000000000000, 0.8660254037844387076, 1.000000000000000000, 0.8660254037844387076, 1.000000000000000000, 0.8660254037844387076, 1.000000000000000000, 0.8660254037844387076, 1.000000000000000000, 0.8660254037844387076, 1.000000000000000000, 0.8660254037844387076, 1.000000000000000000, 0.8660254037844387076, 1.000000000000000000, 0.8660254037844387076, 1.000000000000000000, 0.8660254037844387076, 1.000000000000000000, 0.8660254037844387076, 1.000000000000000000, 0.8660254037844387076, 1.000000000000000000, 0.8660254037844387076, 1.000000000000000000, 0.8660254037844387076, 1.000000000000000000, 0.8660254037844387076, 1.000000000000000000, 0.8660254037844387076, 1.000000000000000000, 0.8660254037844387076, 1.000000000000000000, 0.8660254037844387076, 1.000000000000000000, 0.8660254037844387076, 1.000000000000000000, 0.8660254037844387076, 1.000000000000000000, 0.8660254037844387076, 1.000000000000000000, 0.8660254037844387076, 1.000000000000000000, 0.8660254037844387076, 1.000000000000000000, 0.8660254037844387076, 1.000000000000000000, 0.8660254037844387076, 1.000000000000000000, 0.8660254037844387076, 1.000000000000000000, 0.8660254037844387076, 1.000000000000000000, 0.8660254037844387076, 1.000000000000000000, 0.8660254037844387076, 1.000000000000000000, 0.8660254037844387076, 1.000000000000000000, 0.8660254037844387076, 1.000000000000000000, 0.8660254037844387076, 1.000000000000000000, 0.8660254037844387076, 1.000000000000000000, 0.8660254037844387076, 1.000000000000000000, 0.8660254037844387076, 1.000000000000000000, 0.8660254037844387076, 1.000000000000000000, 0.8660254037844387076, 1.000000000000000000, 0.8660254037844387076, 1.000000000000000000, 0.8660254037844387076, 1.000000000000000000, 0.8660254037844387076, 1.000000000000000000, 0.8660254037844387076, 1.000000000000000000, 0.8660254037844387076, 1.000000000000000000, 0.8660254037844387076, 1.000000000000000000, 0.8660254037844387076, 1.000000000000000000, 0.8660254037844387076, 1.000000000000000000, 0.8660254037844387076, 1.000000000000000000, 0.8660254037844387076, 1.000000000000000000, 0.8660254037844387076, 1.000000000000000000, 0.8660254037844387076, 1.000000000000000000, 0.8660254037844387076, 1.000000000000000000, 0.8660254037844387076, 1.000000000000000000, 0.8660254037844387076, 1.000000000000000000, 0.8660254037844387076, 1.000000000000000000, 0.8660254037844387076, 1.000000000000000000, 0.8660254037844387076, 1.000000000000000000, 0.8660254037844387076, 1.000000000000000000, 0.8660254037844387076, 1.000000000000000000, 0.8660254037844387076, 1.000000000000000000, 0.8660254037844387076, 1.000000000000000000, 0.8660254037844387076, 1.000000000000000000, 0.8660254037844387076, 1.000000000000000000, 0.8660254037844387076, 1.000000000000000000, 0.8660254037844387076, 1.000000000000000000, 0.8660254037844387076, 1.000000000000000000, 0.8660254037844387076, 1.000000000000000000, 0.8660254037844387076, 1.000000000000000000, 0.8660254037844387076, 1.000000000000000000, 0.8660254037844387076, 1.000000000000000000, 0.8660254037844387076, 1.000000000000000000, 0.8660254037844387076, 1.000000000000000000, 0.8660254037844387076, 1.000000000000000000, 0.8660254037844387076, 1.000000000000000000, 0.8660254037844387076, 1.000000000000000000, 0.8660254037844387076, 1.000000000000000000, 0.8660254037844387076, 1.000000000000000000, 0.8660254037844387076, 1.000000000000000000, 0.8660254037844387076, 1.000000000000000000, 0.8660254037844387076, 1.000000000000000000, 0.8660254037844387076, 1.000000000000000000, 0.8660254037844387076, 1.000000000000000000, 0.8660254037844387076, 1.000000000000000000, 0.8660254037844387076, 1.000000000000000000, 0.8660254037844387076, 1.000000000000000000, 0.8660254037844387076, 1.000000000000000000, 0.8660254037844387076, 1.000000000000000000, 0.8660254037844387076, 1.000000000000000000, 0.8660254037844387076, 1.000000000000000000, 0.8660254037844387076, 1.000000000000000000, 0.8660254037844387076, 1.000000000000000000, 0.8660254037844387076, 1.000000000000000000, 0.8660254037844387076, 1.000000000000000000, 0.8660254037844387076, 1.000000000000000000, 0.8660254037844387076, 1.000000000000000000, 0.8660254037844387076, 1.000000000000000000, 0.8660254037844387076, 1.000000000000000000, 0.8660254037844387076, 1.000000000000000000, 0.8660254037844387076, 1.000000000000000000, 0.8660254037844387076, 1.000000000000000000, 0.8660254037844387076, 1.000000000000000000, 0.8660254037844387076, 1.000000000000000000, 0.8660254037844387076, 1.000000000000000000, 0.8660254037844387076, 1.000000000000000000, 0.8660254037844387076, 1.000000000000000000, 0.8660254037844387076, 1.000000000000000000, 0.8660254037844387076, 1.000000000000000000, 0.8660254037844387076, 1.000000000000000000, 0.8660254037844387076, 1.000000000000000000, 0.8660254037844387076, 1.000000000000000000, 0.8660254037844387076, 1.000000000000000000, 0.8660254037844387076, 1.000000000000000000, 0.8660254037844387076, 1.000000000000000000, 0.8660254037844387076, 1.000000000000000000, 0.8660254037844387076, 1.000000000000000000, 0.8660254037844387076, 1.000000000000000000, 0.8660254037844387076, 1.000000000000000000, 0.8660254037844387076, 1.000000000000000000, 0.8660254037844387076, 1.000000000000000000, 0.8660254037844387076, 1.000000000000000000, 0.8660254037844387076, 1.000000000000000000, 0.8660254037844387076, 1.000000000000000000, 0.8660254037844387076, 1.000000000000000000, 0.8660254037844387076, 1.000000000000000000, 0.8660254037844387076, 1.000000000000000000, 0.8660254037844387076, 1.000000000000000000, 0.8660254037844387076, 1.000000000000000000, 0.8660254037844387076, 1.000000000000000000, 0.8660254037844387076, 1.000000000000000000, 0.8660254037844387076, 1.000000000000000000, 0.8660254037844387076, 1.000000000000000000, 0.8660254037844387076, 1.000000000000000000, 0.8660254037844387076, 1.000000000000000000, 0.8660254037844387076, 1.000000000000000000, 0.8660254037844387076, 1.000000000000000000, 0.8660254037844387076, 1.000000000000000000, 0.8660254037844387076, 1.000000000000000000, 0.8660254037844387076, 1.000000000000000000, 0.8660254037844387076, 1.000000000000000000, 0.8660254037844387076, 1.000000000000000000, 0.8660254037844387076, 1.000000000000000000, 0.8660254037844387076, 1.000000000000000000, 0.8660254037844387076, 1.000000000000000000, 0.8660254037844387076, 1.000000000000000000, 0.8660254037844387076, 1.000000000000000000, 0.8660254037844387076, 1.000000000000000000, 0.8660254037844387076, 1.000000000000000000, 0.8660254037844387076, 1.000000000000000000, 0.8660254037844387076, 1.000000000000000000, 0.8660254037844387076, 1.000000000000000000, 0.8660254037844387076, 1.000000000000000000, 0.8660254037844387076, 1.000000000000000000, 0.8660254037844387076, 1.000000000000000000, 0.8660254037844387076, 1.000000000000000000, 0.8660254037844387076, 1.000000000000000000, 0.8660254037844387076, 1.000000000000000000, 0.8660254037844387076, 1.000000000000000000, 0.8660254037844387076, 1.000000000000000000, 0.8660254037844387076, 1.000000000000000000, 0.8660254037844387076, 1.000000000000000000, 0.8660254037844387076, 1.000000000000000000, 0.8660254037844387076, 1.000000000000000000, 0.8660254037844387076, 1.000000000000000000, 0.8660254037844387076, 1.000000000000000000, 0.8660254037844387076, 1.000000000000000000, 0.8660254037844387076, 1.000000000000000000, 0.8660254037844387076, 1.000000000000000000, 0.8660254037844387076, 1.000000000000000000, 0.8660254037844387076, 1.000000000000000000, 0.8660254037844387076, 1.000000000000000000, 0.8660254037844387076, 1.000000000000000000, 0.8660254037844387076, 1.000000000000000000, 0.8660254037844387076, 1.000000000000000000, 0.8660254037844387076, 1.000000000000000000, 0.8660254037844387076, 1.000000000000000000, 0.8660254037844387076, 1.000000000000000000, 0.8660254037844387076, 1.000000000000000000, 0.8660254037844387076, 1.000000000000000000, 0.8660254037844387076, 1.000000000000000000, 0.8660254037844387076, 1.000000000000000000, 0.8660254037844387076, 1.000000000000000000, 0.8660254037844387076, 1.000000000000000000, 0.8660254037844387076, 1.000000000000000000, 0.8660254037844387076, 1.000000000000000000, 0.8660254037844387076, 1.000000000000000000, 0.8660254037844387076, 1.000000000000000000, 0.8660254037844387076, 1.000000000000000000, 0.8660254037844387076, 1.000000000000000000, 0.8660254037844387076, 1.000000000000000000, 0.8660254037844387076, 1.000000000000000000, 0.8660254037844387076, 1.000000000000000000, 0.8660254037844387076, 1.000000000000000000, 0.8660254037844387076, 1.000000000000000000, 0.8660254037844387076, 1.000000000000000000, 0.8660254037844387076, 1.000000000000000000, 0.8660254037844387076, 1.000000000000000000, 0.8660254037844387076, 1.000000000000000000, 0.8660254037844387076, 1.000000000000000000, 0.8660254037844387076, 1.000000000000000000, 0.8660254037844387076, 1.000000000000000000, 0.8660254037844387076, 1.000000000000000000, 0.8660254037844387076, 1.000000000000000000, 0.8660254037844387076, 1.000000000000000000, 0.8660254037844387076, 1.000000000000000000, 0.8660254037844387076, 1.000000000000000000, 0.8660254037844387076, 1.000000000000000000, 0.8660254037844387076, 1.000000000000000000, 0.8660254037844387076, 1.000000000000000000, 0.8660254037844387076, 1.000000000000000000, 0.8660254037844387076, 1.000000000000000000, 0.8660254037844387076, 1.000000000000000000, 0.8660254037844387076, 1.000000000000000000, 0.8660254037844387076, 1.000000000000000000, 0.8660254037844387076, 1.000000000000000000, 0.8660254037844387076, 1.000000000000000000, 0.8660254037844387076, 1.000000000000000000, 0.8660254037844387076, 1.000000000000000000, 0.8660254037844387076, 1.000000000000000000, 0.8660254037844387076, 1.000000000000000000, 0.8660254037844387076, 1.000000000000000000, 0.8660254037844387076, 1.000000000000000000, 0.8660254037844387076, 1.000000000000000000, 0.8660254037844387076, 1.000000000000000000, 0.8660254037844387076, 1.000000000000000000, 0.8660254037844387076, 1.000000000000000000, 0.8660254037844387076, 1.000000000000000000, 0.8660254037844387076, 1.000000000000000000, 0.8660254037844387076, 1.000000000000000000, 0.8660254037844387076, 1.000000000000000000, 0.8660254037844387076, 1.000000000000000000, 0.8660254037844387076, 1.000000000000000000, 0.8660254037844387076, 1.000000000000000000, 0.8660254037844387076, 1.000000000000000000, 0.8660254037844387076, 1.000000000000000000, 0.8660254037844387076, 1.000000000000000000, 0.8660254037844387076, 1.000000000000000000, 0.8660254037844387076, 1.000000000000000000, 0.8660254037844387076, 1.000000000000000000, 0.8660254037844387076, 1.000000000000000000, 0.8660254037844387076, 1.000000000000000000, 0.8660254037844387076, 1.000000000000000000, 0.8660254037844387076, 1.000000000000000000, 0.8660254037844387076, 1.000000000000000000, 0.8660254037844387076, 1.000000000000000000, 0.8660254037844387076, 1.000000000000000000, 0.8660254037844387076, 1.000000000000000000, 0.8660254037844387076, 1.000000000000000000, 0.8660254037844387076, 1.000000000000000000, 0.8660254037844387076, 1.000000000000000000, 0.8660254037844387076, 1.000000000000000000, 0.8660254037844387076, 1.000000000000000000, 0.8660254037844387076, 1.000000000000000000, 0.8660254037844387076, 1.000000000000000000, 0.8660254037844387076, 1.000000000000000000, 0.8660254037844387076, 1.000000000000000000, 0.8660254037844387076, 1.000000000000000000, 0.8660254037844387076, 1.000000000000000000, 0.8660254037844387076, 1.000000000000000000, 0.8660254037844387076, 1.000000000000000000, 0.8660254037844387076, 1.000000000000000000, 0.8660254037844387076, 1.000000000000000000, 0.8660254037844387076, 1.000000000000000000, 0.8660254037844387076, 1.000000000000000000, 0.8660254037844387076, 1.000000000000000000, 0.8660254037844387076, 1.000000000000000000, 0.8660254037844387076, 1.000000000000000000, 0.8660254037844387076, 1.000000000000000000, 0.8660254037844387076, 1.000000000000000000, 0.8660254037844387076, 1.000000000000000000, 0.8660254037844387076, 1.000000000000000000, 0.8660254037844387076, 1.000000000000000000, 0.8660254037844387076, 1.000000000000000000, 0.8660254037844387076, 1.000000000000000000, 0.8660254037844387076, 1.000000000000000000, 0.8660254037844387076, 1.000000000000000000, 0.8660254037844387076, 1.000000000000000000, 0.8660254037844387076, 1.000000000000000000, 0.8660254037844387076, 1.000000000000000000, 0.8660254037844387076, 1.000000000000000000, 0.8660254037844387076, 1.000000000000000000, 0.8660254037844387076, 1.000000000000000000, 0.8660254037844387076, 1.000000000000000000, 0.8660254037844387076, 1.000000000000000000, 0.8660254037844387076, 1.000000000000000000, 0.8660254037844387076, 1.000000000000000000, 0.8660254037844387076, 1.000000000000000000, 0.8660254037844387076, 1.000000000000000000, 0.8660254037844387076, 1.000000000000000000, 0.8660254037844387076, 1.000000000000000000, 0.8660254037844387076, 1.000000000000000000, 0.8660254037844387076, 1.000000000000000000, 0.8660254037844387076, 1.000000000000000000, 0.8660254037844387076, 1.000000000000000000, 0.8660254037844387076, 1.000000000000000000, 0.8660254037844387076, 1.000000000000000000, 0.8660254037844387076, 1.000000000000000000, 0.8660254037844387076, 1.000000000000000000, 0.8660254037844387076, 1.000000000000000000, 0.8660254037844387076, 1.000000000000000000, 0.8660254037844387076, 1.000000000000000000, 0.8660254037844387076, 1.000000000000000000, 0.8660254037844387076, 1.000000000000000000, 0.8660254037844387076, 1.000000000000000000, 0.8660254037844387076, 1.000000000000000000, 0.8660254037844387076, 1.000000000000000000, 0.8660254037844387076, 1.000000000000000000, 0.8660254037844387076, 1.000000000000000000, 0.8660254037844387076, 1.000000000000000000, 0.8660254037844387076, 1.000000000000000000, 0.8660254037844387076, 1.000000000000000000, 0.8660254037844387076, 1.000000000000000000, 0.8660254037844387076, 1.000000000000000000, 0.8660254037844387076, 1.000000000000000000, 0.8660254037844387076, 1.000000000000000000, 0.8660254037844387076, 1.000000000000000000, 0.8660254037844387076, 1.000000000000000000, 0.8660254037844387076, 1.000000000000000000, 0.8660254037844387076, 1.000000000000000000, 0.8660254037844387076, 1.000000000000000000, 0.8660254037844387076, 1.000000000000000000, 0.8660254037844387076, 1.000000000000000000, 0.8660254037844387076, 1.000000000000000000, 0.8660254037844387076, 1.000000000000000000, 0.8660254037844387076, 1.000000000000000000, 0.8660254037844387076, 1.000000000000000000, 0.8660254037844387076, 1.000000000000000000, 0.8660254037844387076, 1.000000000000000000, 0.8660254037844387076, 1.000000000000000000, 0.8660254037844387076, 1.000000000000000000, 0.8660254037844387076, 1.000000000000000000, 0.8660254037844387076, 1.000000000000000000, 0.8660254037844387076, 1.000000000000000000, 0.8660254037844387076, 1.000000000000000000, 0.8660254037844387076, 1.000000000000000000, 0.8660254037844387076, 1.000000000000000000, 0.8660254037844387076, 1.000000000000000000, 0.8660254037844387076, 1.000000000000000000, 0.8660254037844387076, 1.000000000000000000, 0.8660254037844387076, 1.000000000000000000, 0.8660254037844387076, 1.000000000000000000, 0.8660254037844387076, 1.000000000000000000, 0.8660254037844387076, 1.000000000000000000, 0.8660254037844387076, 1.000000000000000000, 0.8660254037844387076, 1.000000000000000000, 0.8660254037844387076, 1.000000000000000000, 0.8660254037844387076, 1.000000000000000000, 0.8660254037844387076, 1.000000000000000000, 0.8660254037844387076, 1.000000000000000000, 0.8660254037844387076, 1.000000000000000000, 0.8660254037844387076, 1.000000000000000000, 0.8660254037844387076, 1.000000000000000000, 0.8660254037844387076, 1.000000000000000000, 0.8660254037844387076, 1.000000000000000000, 0.8660254037844387076, 1.000000000000000000, 0.8660254037844387076, 1.000000000000000000, 0.8660254037844387076, 1.000000000000000000, 0.8660254037844387076, 1.000000000000000000, 0.8660254037844387076, 1.000000000000000000, 0.8660254037844387076, 1.000000000000000000, 0.8660254037844387076, 1.000000000000000000, 0.8660254037844387076, 1.000000000000000000, 0.8660254037844387076, 1.000000000000000000, 0.8660254037844387076, 1.000000000000000000, 0.8660254037844387076, 1.000000000000000000, 0.8660254037844387076, 1.000000000000000000, 0.8660254037844387076, 1.000000000000000000, 0.8660254037844387076, 1.000000000000000000, 0.8660254037844387076, 1.000000000000000000, 0.8660254037844387076, 1.000000000000000000, 0.8660254037844387076, 1.000000000000000000, 0.8660254037844387076, 1.000000000000000000, 0.8660254037844387076, 1.000000000000000000, 0.8660254037844387076, 1.000000000000000000, 0.8660254037844387076, 1.000000000000000000, 0.8660254037844387076, 1.000000000000000000, 0.8660254037844387076, 1.000000000000000000, 0.8660254037844387076, 1.000000000000000000, 0.8660254037844387076, 1.000000000000000000, 0.8660254037844387076, 1.000000000000000000, 0.8660254037844387076, 1.000000000000000000, 0.8660254037844387076, 1.000000000000000000, 0.8660254037844387076, 1.000000000000000000, 0.8660254037844387076, 1.000000000000000000, 0.8660254037844387076, 1.000000000000000000, 0.8660254037844387076, 1.000000000000000000, 0.8660254037844387076, 1.000000000000000000, 0.8660254037844387076, 1.000000000000000000, 0.8660254037844387076, 1.000000000000000000, 0.8660254037844387076, 1.000000000000000000, 0.8660254037844387076, 1.000000000000000000, 0.8660254037844387076, 1.000000000000000000, 0.8660254037844387076, 1.000000000000000000, 0.8660254037844387076, 1.000000000000000000, 0.8660254037844387076, 1.000000000000000000, 0.8660254037844387076, 1.000000000000000000, 0.8660254037844387076, 1.000000000000000000, 0.8660254037844387076, 1.000000000000000000, 0.8660254037844387076, 1.000000000000000000, 0.8660254037844387076, 1.000000000000000000, 0.8660254037844387076, 1.000000000000000000, 0.8660254037844387076, 1.000000000000000000, 0.8660254037844387076, 1.000000000000000000, 0.8660254037844387076, 1.000000000000000000, 0.8660254037844387076, 1.000000000000000000, 0.8660254037844387076, 1.000000000000000000, 0.8660254037844387076, 1.000000000000000000, 0.8660254037844387076, 1.000000000000000000, 0.8660254037844387076, 1.000000000000000000, 0.8660254037844387076, 1.000000000000000000, 0.8660254037844387076, 1.000000000000000000, 0.8660254037844387076, 1.000000000000000000, 0.8660254037844387076, 1.000000000000000000, 0.8660254037844387076, 1.000000000000000000, 0.8660254037844387076, 1.000000000000000000, 0.8660254037844387076, 1.000000000000000000, 0.8660254037844387076, 1.000000000000000000, 0.8660254037844387076, 1.000000000000000000, 0.8660254037844387076, 1.000000000000000000, 0.8660254037844387076, 1.000000000000000000, 0.8660254037844387076, 1.000000000000000000, 0.8660254037844387076, 1.000000000000000000, 0.8660254037844387076, 1.000000000000000000, 0.8660254037844387076, 1.000000000000000000, 0.8660254037844387076, 1.000000000000000000, 0.8660254037844387076, 1.000000000000000000, 0.8660254037844387076, 1.000000000000000000, 0.8660254037844387076, 1.000000000000000000, 0.8660254037844387076, 1.000000000000000000, 0.8660254037844387076, 1.000000000000000000, 0.8660254037844387076, 1.000000000000000000, 0.8660254037844387076, 1.000000000000000000, 0.8660254037844387076, 1.000000000000000000, 0.8660254037844387076, 1.000000000000000000, 0.8660254037844387076, 1.000000000000000000, 0.8660254037844387076, 1.000000000000000000, 0.8660254037844387076, 1.000000000000000000, 0.8660254037844387076, 1.000000000000000000, 0.8660254037844387076, 1.000000000000000000, 0.8660254037844387076, 1.000000000000000000, 0.8660254037844387076, 1.000000000000000000, 0.8660254037844387076, 1.000000000000000000, 0.8660254037844387076, 1.000000000000000000, 0.8660254037844387076, 1.000000000000000000, 0.8660254037844387076, 1.000000000000000000, 0.8660254037844387076, 1.000000000000000000, 0.8660254037844387076, 1.000000000000000000, 0.8660254037844387076, 1.000000000000000000, 0.8660254037844387076, 1.000000000000000000, 0.8660254037844387076, 1.000000000000000000, 0.8660254037844387076, 1.000000000000000000, 0.8660254037844387076, 1.000000000000000000, 0.8660254037844387076, 1.000000000000000000, 0.8660254037844387076, 1.000000000000000000, 0.8660254037844387076, 1.000000000000000000, 0.8660254037844387076, 1.000000000000000000, 0.8660254037844387076, 1.000000000000000000, 0.8660254037844387076, 1.000000000000000000, 0.8660254037844387076, 1.000000000000000000, 0.8660254037844387076, 1.000000000000000000, 0.8660254037844387076, 1.000000000000000000, 0.8660254037844387076, 1.000000000000000000, 0.8660254037844387076, 1.000000000000000000, 0.8660254037844387076, 1.000000000000000000, 0.8660254037844387076, 1.000000000000000000, 0.8660254037844387076, 1.000000000000000000, 0.8660254037844387076, 1.000000000000000000, 0.8660254037844387076, 1.000000000000000000, 0.8660254037844387076, 1.000000000000000000, 0.8660254037844387076, 1.000000000000000000, 0.8660254037844387076, 1.000000000000000000, 0.8660254037844387076, 1.000000000000000000, 0.8660254037844387076, 1.000000000000000000, 0.8660254037844387076, 1.000000000000000000, 0.8660254037844387076, 1.000000000000000000, 0.8660254037844387076, 1.000000000000000000, 0.8660254037844387076, 1.000000000000000000, 0.8660254037844387076, 1.000000000000000000, 0.8660254037844387076, 1.000000000000000000, 0.8660254037844387076, 1.000000000000000000, 0.8660254037844387076, 1.000000000000000000, 0.8660254037844387076, 1.000000000000000000, 0.8660254037844387076, 1.000000000000000000, 0.8660254037844387076, 1.000000000000000000, 0.8660254037844387076, 1.000000000000000000, 0.8660254037844387076, 1.000000000000000000, 0.8660254037844387076, 1.000000000000000000, 0.8660254037844387076, 1.000000000000000000, 0.8660254037844387076, 1.000000000000000000, 0.8660254037844387076, 1.000000000000000000, 0.8660254037844387076, 1.000000000000000000, 0.8660254037844387076, 1.000000000000000000, 0.8660254037844387076, 1.000000000000000000, 0.8660254037844387076, 1.000000000000000000, 0.8660254037844387076, 1.000000000000000000, 0.8660254037844387076, 1.000000000000000000, 0.8660254037844387076, 1.000000000000000000, 0.8660254037844387076, 1.000000000000000000, 0.8660254037844387076, 1.000000000000000000, 0.8660254037844387076, 1.000000000000000000, 0.8660254037844387076, 1.000000000000000000, 0.8660254037844387076, 1.000000000000000000, 0.8660254037844387076, 1.000000000000000000, 0.8660254037844387076, 1.000000000000000000, 0.8660254037844387076, 1.000000000000000000, 0.8660254037844387076, 1.000000000000000000, 0.8660254037844387076, 1.000000000000000000, 0.8660254037844387076, 1.000000000000000000, 0.8660254037844387076, 1.000000000000000000, 0.8660254037844387076, 1.000000000000000000, 0.8660254037844387076, 1.000000000000000000, 0.8660254037844387076, 1.000000000000000000, 0.8660254037844387076, 1.000000000000000000, 0.8660254037844387076, 1.000000000000000000, 0.8660254037844387076, 1.000000000000000000, 0.8660254037844387076, 1.000000000000000000, 0.8660254037844387076, 1.000000000000000000, 0.8660254037844387076, 1.000000000000000000, 0.8660254037844387076, 1.000000000000000000, 0.8660254037844387076, 1.000000000000000000, 0.8660254037844387076, 1.000000000000000000, 0.8660254037844387076, 1.000000000000000000, 0.8660254037844387076, 1.000000000000000000, 0.8660254037844387076, 1.000000000000000000, 0.8660254037844387076, 1.000000000000000000, 0.8660254037844387076, 1.000000000000000000, 0.8660254037844387076, 1.000000000000000000, 0.8660254037844387076, 1.000000000000000000, 0.8660254037844387076, 1.000000000000000000, 0.8660254037844387076, 1.000000000000000000, 0.8660254037844387076, 1.000000000000000000, 0.8660254037844387076, 1.000000000000000000, 0.8660254037844387076, 1.000000000000000000, 0.8660254037844387076, 1.000000000000000000, 0.8660254037844387076, 1.000000000000000000, 0.8660254037844387076, 1.000000000000000000, 0.8660254037844387076, 1.000000000000000000, 0.8660254037844387076, 1.000000000000000000, 0.8660254037844387076, 1.000000000000000000, 0.8660254037844387076, 1.000000000000000000, 0.8660254037844387076, 1.000000000000000000, 0.8660254037844387076, 1.000000000000000000, 0.8660254037844387076, 1.000000000000000000, 0.8660254037844387076, 1.000000000000000000, 0.8660254037844387076, 1.000000000000000000, 0.8660254037844387076, 1.000000000000000000, 0.8660254037844387076, 1.000000000000000000, 0.8660254037844387076, 1.000000000000000000, 0.8660254037844387076, 1.000000000000000000, 0.8660254037844387076, 1.000000000000000000, 0.8660254037844387076, 1.000000000000000000, 0.8660254037844387076, 1.000000000000000000, 0.8660254037844387076, 1.000000000000000000, 0.8660254037844387076, 1.000000000000000000, 0.8660254037844387076, 1.000000000000000000, 0.8660254037844387076, 1.000000000000000000, 0.8660254037844387076, 1.000000000000000000, 0.8660254037844387076, 1.000000000000000000, 0.8660254037844387076, 1.000000000000000000, 0.8660254037844387076, 1.000000000000000000, 0.8660254037844387076, 1.000000000000000000, 0.8660254037844387076, 1.000000000000000000, 0.8660254037844387076, 1.000000000000000000, 0.8660254037844387076, 1.000000000000000000, 0.8660254037844387076, 1.000000000000000000, 0.8660254037844387076, 1.000000000000000000, 0.8660254037844387076, 1.000000000000000000, 0.8660254037844387076, 1.000000000000000000, 0.8660254037844387076, 1.000000000000000000, 0.8660254037844387076, 1.000000000000000000, 0.8660254037844387076, 1.000000000000000000, 0.8660254037844387076, 1.000000000000000000, 0.8660254037844387076, 1.000000000000000000, 0.8660254037844387076, 1.000000000000000000, 0.8660254037844387076, 1.000000000000000000, 0.8660254037844387076, 1.000000000000000000, 0.8660254037844387076, 1.000000000000000000, 0.8660254037844387076, 1.000000000000000000, 0.8660254037844387076, 1.000000000000000000, 0.8660254037844387076, 1.000000000000000000, 0.8660254037844387076, 1.000000000000000000, 0.8660254037844387076, 1.000000000000000000, 0.8660254037844387076, 1.000000000000000000, 0.8660254037844387076, 1.000000000000000000, 0.8660254037844387076, 1.000000000000000000, 0.8660254037844387076, 1.000000000000000000, 0.8660254037844387076, 1.000000000000000000, 0.8660254037844387076, 1.000000000000000000, 0.8660254037844387076, 1.000000000000000000, 0.8660254037844387076, 1.000000000000000000, 0.8660254037844387076, 1.000000000000000000, 0.8660254037844387076, 1.000000000000000000, 0.8660254037844387076, 1.000000000000000000, 0.8660254037844387076, 1.000000000000000000, 0.8660254037844387076, 1.000000000000000000, 0.8660254037844387076, 1.000000000000000000, 0.8660254037844387076, 1.000000000000000000, 0.8660254037844387076, 1.000000000000000000, 0.8660254037844387076, 1.000000000000000000, 0.8660254037844387076, 1.000000000000000000, 0.8660254037844387076, 1.000000000000000000, 0.8660254037844387076, 1.000000000000000000, 0.8660254037844387076, 1.000000000000000000, 0.8660254037844387076, 1.000000000000000000, 0.8660254037844387076, 1.000000000000000000, 0.8660254037844387076, 1.000000000000000000, 0.8660254037844387076, 1.000000000000000000, 0.8660254037844387076, 1.000000000000000000, 0.8660254037844387076, 1.000000000000000000, 0.8660254037844387076, 1.000000000000000000, 0.8660254037844387076, 1.000000000000000000, 0.8660254037844387076, 1.000000000000000000, 0.8660254037844387076, 1.000000000000000000, 0.8660254037844387076, 1.000000000000000000, 0.8660254037844387076, 1.000000000000000000, 0.8660254037844387076, 1.000000000000000000, 0.8660254037844387076, 1.000000000000000000, 0.8660254037844387076, 1.000000000000000000, 0.8660254037844387076, 1.000000000000000000, 0.8660254037844387076, 1.000000000000000000, 0.8660254037844387076, 1.000000000000000000, 0.8660254037844387076, 1.000000000000000000, 0.8660254037844387076, 1.000000000000000000, 0.8660254037844387076, 1.000000000000000000, 0.8660254037844387076, 1.000000000000000000, 0.8660254037844387076, 1.000000000000000000, 0.8660254037844387076, 1.000000000000000000, 0.8660254037844387076, 1.000000000000000000, 0.8660254037844387076, 1.000000000000000000, 0.8660254037844387076, 1.000000000000000000, 0.8660254037844387076, 1.000000000000000000, 0.8660254037844387076, 1.000000000000000000, 0.8660254037844387076, 1.000000000000000000, 0.8660254037844387076, 1.000000000000000000, 0.8660254037844387076, 1.000000000000000000, 0.8660254037844387076, 1.000000000000000000, 0.8660254037844387076, 1.000000000000000000, 0.8660254037844387076, 1.000000000000000000, 0.8660254037844387076, 1.000000000000000000, 0.8660254037844387076, 1.000000000000000000, 0.8660254037844387076, 1.000000000000000000, 0.8660254037844387076, 1.000000000000000000, 0.8660254037844387076, 1.000000000000000000, 0.8660254037844387076, 1.000000000000000000, 0.8660254037844387076, 1.000000000000000000, 0.8660254037844387076, 1.000000000000000000, 0.8660254037844387076, 1.000000000000000000, 0.8660254037844387076, 1.000000000000000000, 0.8660254037844387076, 1.000000000000000000, 0.8660254037844387076, 1.000000000000000000, 0.8660254037844387076, 1.000000000000000000, 0.8660254037844387076, 1.000000000000000000, 0.8660254037844387076, 1.000000000000000000, 0.8660254037844387076, 1.000000000000000000, 0.8660254037844387076, 1.000000000000000000, 0.8660254037844387076, 1.000000000000000000, 0.8660254037844387076, 1.000000000000000000, 0.8660254037844387076, 1.000000000000000000, 0.8660254037844387076, 1.000000000000000000, 0.8660254037844387076, 1.000000000000000000, 0.8660254037844387076, 1.000000000000000000, 0.8660254037844387076, 1.000000000000000000, 0.8660254037844387076, 1.000000000000000000, 0.8660254037844387076, 1.000000000000000000, 0.8660254037844387076, 1.000000000000000000) ) ) 
 REPRESENTATION_ITEM ( '' )  SURFACE ( )  );
#32272=CARTESIAN_POINT ( 'NONE',  ( -3.152548672688508926E-16, -17.81249999863440792, -5.148502694627439702 ) ) ;
#32273=CARTESIAN_POINT ( 'NONE',  ( 5.000000000000000888, -62.45833333060214443, 2.886751345948126879 ) ) ;
#32278=CARTESIAN_POINT ( 'NONE',  ( -6.972266317189433020E-16, -6.124999997268813168, -5.000000000000000000 ) ) ;
#32281=CARTESIAN_POINT ( 'NONE',  ( -2.499999999999996447, 3.291666669397851575, 4.330127018922195425 ) ) ;
#32283=CARTESIAN_POINT ( 'NONE',  ( -9.184850993605147944E-16, -156.2500000000000000, 5.000000000000000000 ) ) ;
#32284=CARTESIAN_POINT ( 'NONE',  ( -2.229367062499996610, -51.39583333196773651, 3.861377020970582219 ) ) ;
#32286=VECTOR ( 'NONE', #5282, 1000.000000000000000 ) ;
#32287=( BOUNDED_SURFACE ( )  B_SPLINE_SURFACE ( 1, 2, ( 
 ( #39762, #15014, #25627, #54897, #21120, #11143, #54579, #10501, #15972, #50388, #5372, #10826, #30116, #30439, #557, #40727, #6336, #50067, #6022, #45241, #60374, #24990, #25942, #1207, #16297, #59088, #44597, #59408, #5052, #24670, #20806, #35920, #9864, #29474, #49746, #49106, #882, #44278, #10195, #240, #15340, #19838, #5690, #34629, #25306, #20490, #40088, #16930, #2466, #31082, #12422, #36232, #47155, #22401, #31721, #26254, #26904, #55859, #7921, #61323, #56177, #46201, #51030, #61956, #2161, #60693, #21768, #46524, #41046, #17877, #41361, #37192, #3102, #27526, #45877, #17573, #22719, #41673, #50705, #32034, #42316, #32357, #51669, #16613, #7611, #31391, #21443, #56816, #22077, #12733, #11773, #17246, #51979, #6972, #26582, #61005, #36870, #36545, #56500, #12098, #46833, #51355, #55549, #27216, #11460, #6647, #1840, #7294, #2781, #42000, #61641, #14303, #38738, #13053, #52609, #52300, #8237, #13370, #53549, #8854, #47461, #57758, #48709, #37818, #9473, #4040, #8544, #23659, #62590, #32992, #57447, #58376, #33616, #57137, #13681, #47771, #28156, #3726, #9166, #18511, #23347, #42948, #18197, #32670, #19119, #38133, #23959, #53234, #23030, #27839, #33300, #52918, #3414, #29082, #33923, #42633, #62272, #63208, #63522, #37496, #28472, #4650, #48084, #43253, #62894, #18808, #24270, #38430, #4341, #58057, #13986, #43876, #28782, #48399, #43563, #14616, #29719, #25871, #15262, #58687, #30045, #25548, #45486, #30695, #10115, #35207, #14933, #10432, #59658, #4972, #59981, #34228, #53855, #54508, #15904, #19446, #45166, #40012, #39059, #6263, #24916, #44201, #34540, #25231, #44842, #54825, #54176, #49353, #10757, #44520, #5298, #482, #166, #9784, #1135, #20084, #5942, #15590, #24594, #29392, #39688, #59328, #49028, #11072, #20734, #19763, #39374, #40338, #59005, #34886, #49674, #55146, #5617, #806, #20412, #30366, #35523, #49988, #50313, #16541, #46128, #37981, #2092, #11387, #7220, #60298, #11702, #8702, #60936, #40658, #12022, #7533, #28317, #13539, #55785, #17172, #60621, #56102, #41599, #50636, #41927, #16224, #35847, #36476, #61569, #1450, #27145, #22005, #21051, #52774, #6897, #26189, #36164, #26833, #46450, #36798, #55471, #61250, #17503, #57612, #56430, #6574, #12352, #40975, #31007, #46761, #31652, #2706, #21370, #2395, #22325, #45808, #1768, #31322, #51287, #50957, #31964, #26511, #51598, #21696, #33160, #41287, #16854, #49201, #5141, #43732, #3887, #29570, #28938, #24760, #44363, #23505, #63062, #62749, #18670, #23815, #325, #19290, #57921, #4503, #59175, #48246, #19924, #14463, #18974, #34085, #9325, #43419, #4202, #39537, #44043, #43108, #24129, #58221, #29249, #38588, #39223, #28629, #15109, #24440, #38293, #34725, #54353, #63375, #13840, #10283, #48563, #47932, #33460, #53082, #14150, #9018, #33775, #53394, #38908, #58541, #53708, #9641, #48873, #4821, #10, #19610, #58847, #14777, #34394, #54021, #9955, #31172, #26039, #49518, #50154, #40191, #25396, #59827, #1611, #54987, #981, #15749, #10592, #25074, #11554, #10915, #16389, #45654, #15438, #645, #30531, #6108, #20257, #21537, #50804, #5457, #39856, #55639, #55949, #29888, #44684, #1934, #35365, #25723, #45015, #11235, #6740, #16064, #60464, #20584, #45333, #41133, #1303, #59499, #35693, #35056, #20899, #36322, #40502, #54668, #60143, #36008, #30206, #60781, #55320, #21211, #30859, #50488, #6427, #49832, #26348, #5775, #40817, #45970, #16707, #37906, #17958, #32441, #11864, #62358, #17338, #36637, #7382, #17658, #37274, #47245, #7060, #52070, #27926, #52391, #8011, #61098, #27614, #51442, #41448, #37581, #22491, #57222, #31808, #56902, #32761, #17022, #12193, #22168, #61729, #56269, #26672, #46292, #26989, #47547, #46927, #21853, #32119, #23111, #46608, #3497, #42087, #2554, #12820, #36958, #41765, #61415, #13142, #3191, #31480 ),
 ( #56588, #2249, #12507, #51755, #7699, #42715, #8326, #51124, #27302, #18281, #2876, #22807, #42400, #62042, #23749, #53320, #8940, #38827, #14701, #43651, #24362, #28554, #38514, #29482, #58142, #3811, #63291, #52693, #4127, #250, #9253, #33080, #4427, #63611, #19848, #5060, #48175, #9566, #53001, #48490, #34011, #43036, #34320, #8628, #28240, #28868, #53945, #57536, #19531, #14388, #13461, #44288, #62987, #18598, #43344, #19210, #58464, #29173, #47854, #53634, #9874, #49117, #48797, #62676, #4738, #33386, #23435, #39145, #24052, #58772, #13764, #43965, #24680, #38224, #57846, #18900, #14072, #33700, #894, #24998, #35287, #5382, #50075, #40099, #39462, #6033, #25636, #30126, #59098, #45251, #10512, #1218, #20816, #34640, #39774, #567, #49440, #40417, #44936, #60057, #44607, #20500, #15025, #20176, #59420, #34973, #59742, #15350, #15668, #54590, #54265, #49755, #10204, #30450, #29807, #5701, #25316, #54907, #10835, #18025, #17413, #13206, #37647, #11929, #51509, #51193, #7125, #12261, #52457, #7757, #46357, #56654, #47612, #36708, #8392, #2942, #7446, #22556, #61480, #31875, #56341, #57290, #32504, #56016, #12571, #46672, #27054, #2617, #8078, #37028, #22235, #41835, #17087, #31560, #32828, #32184, #22872, #52136, #21914, #26741, #51815, #27360, #2311, #27993, #3566, #41511, #61164, #62106, #62429, #36385, #46994, #23173, #42157, #61793, #17720, #37334, #42784, #56967, #3260, #12886, #27679, #47307, #42465, #28305, #24120, #13530, #28620, #24748, #14137, #57603, #28930, #24432, #44353, #29559, #9008, #34076, #13832, #9316, #58530, #3877, #58838, #33150, #52764, #53383, #14767, #18347, #44034, #38895, #37970, #5130, #23806, #43098, #33451, #43720, #63365, #53699, #8693, #14454, #34385, #54013, #9631, #23496, #29239, #9943, #47919, #38283, #48235, #62739, #18661, #48864, #49192, #4809, #57909, #18964, #53068, #48553, #9216, #4193, #19601, #43408, #63053, #38579, #58210, #39213, #33764, #4492, #19280, #10906, #39528, #20889, #44675, #55629, #30848, #40181, #34715, #35356, #635, #16379, #6099, #972, #54659, #59490, #6729, #10582, #5447, #30194, #54977, #49508, #26339, #49823, #45644, #11544, #35998, #54342, #26029, #31161, #50144, #15426, #21200, #10274, #35047, #45324, #50791, #316, #15739, #20245, #50479, #15098, #6419, #5767, #1292, #19914, #59166, #25712, #1602, #25385, #59817, #16054, #40806, #29878, #60454, #25065, #39847, #45006, #40492, #60133, #20574, #30521, #35682, #55310, #11225, #62052, #51138, #41779, #55963, #21863, #37283, #26686, #47255, #22500, #1946, #3200, #22820, #61425, #21547, #27626, #26998, #42409, #17966, #41142, #61108, #60790, #16716, #41459, #37590, #17348, #11874, #2563, #57233, #46302, #13150, #12517, #17033, #32128, #7391, #36647, #2260, #32770, #42096, #36333, #22177, #51764, #31492, #56278, #52405, #36972, #7071, #56599, #52082, #8336, #45980, #12204, #61741, #31821, #7708, #17668, #51454, #46618, #27312, #46939, #2888, #56912, #12830, #8020, #32450, #27935, #14714, #33398, #52704, #23444, #33711, #53330, #63304, #23120, #4437, #43979, #4750, #48500, #13473, #24067, #3823, #57545, #53645, #38525, #9579, #47864, #9264, #48812, #33089, #28250, #63625, #8638, #23759, #37915, #43046, #19226, #62686, #29185, #43663, #47559, #24378, #19546, #43355, #3508, #39159, #8953, #58784, #34334, #42724, #18607, #62368, #18292, #38235, #53958, #63002, #57855, #48185, #13776, #53012, #28564, #58153, #4138, #14084, #18911, #28879, #38841, #58476, #14402, #34024, #30140, #20190, #5396, #39791, #45267, #34989, #44622, #59437, #54279, #5074, #55251, #54604, #60076, #6046, #59112, #44300, #10527, #49769, #264, #1543, #11170, #29499, #19862, #35623, #35945, #9890, #49131, #45585, #15366, #5715, #25012, #54923, #30793, #59757, #40435, #581, #25330, #21147, #44952, #39476, #912, #15999 ) ),
 .UNSPECIFIED., .F., .F., .F. ) 
 B_SPLINE_SURFACE_WITH_KNOTS ( ( 2, 2 ),
 ( 3, 2, 2, 2, 2, 2, 2, 2, 2, 2, 2, 2, 2, 2, 2, 2, 2, 2, 2, 2, 2, 2, 2, 2, 2, 2, 2, 2, 2, 2, 2, 2, 2, 2, 2, 2, 2, 2, 2, 2, 2, 2, 2, 2, 2, 2, 2, 2, 2, 2, 2, 2, 2, 2, 2, 2, 2, 2, 2, 2, 2, 2, 2, 2, 2, 2, 2, 2, 2, 2, 2, 2, 2, 2, 2, 2, 2, 2, 2, 2, 2, 2, 2, 2, 2, 2, 2, 2, 2, 2, 2, 2, 2, 2, 2, 2, 2, 2, 2, 2, 2, 2, 2, 2, 2, 2, 2, 2, 2, 2, 2, 2, 2, 2, 2, 2, 2, 2, 2, 2, 2, 2, 2, 2, 2, 2, 2, 2, 2, 2, 2, 2, 2, 2, 2, 2, 2, 2, 2, 2, 2, 2, 2, 2, 2, 2, 2, 2, 2, 2, 2, 2, 2, 2, 2, 2, 2, 2, 2, 2, 2, 2, 2, 2, 2, 2, 2, 2, 2, 2, 2, 2, 2, 2, 2, 2, 2, 2, 2, 2, 2, 2, 2, 2, 2, 2, 2, 2, 2, 2, 2, 2, 2, 2, 2, 2, 2, 2, 2, 2, 2, 2, 2, 2, 2, 2, 2, 2, 2, 2, 2, 2, 2, 2, 2, 2, 2, 2, 2, 2, 2, 2, 2, 2, 2, 2, 2, 2, 2, 2, 2, 2, 2, 2, 2, 2, 2, 2, 2, 2, 3 ),
 ( 0.000000000000000000, 1.000000000000000000 ),
 ( 0.000000000000000000, 0.004166666666666666609, 0.008333333333333333218, 0.01250000000000000069, 0.01666666666666666644, 0.02083333333333333218, 0.02500000000000000139, 0.02916666666666666713, 0.03333333333333333287, 0.03749999999999999861, 0.04166666666666666435, 0.04583333333333333010, 0.05000000000000000278, 0.05416666666666666852, 0.05833333333333333426, 0.06250000000000000000, 0.06666666666666666574, 0.07083333333333333148, 0.07499999999999999722, 0.07916666666666666297, 0.08333333333333332871, 0.08749999999999999445, 0.09166666666666666019, 0.09583333333333333981, 0.1000000000000000056, 0.1041666666666666713, 0.1083333333333333370, 0.1125000000000000028, 0.1166666666666666685, 0.1208333333333333343, 0.1250000000000000000, 0.1291666666666666796, 0.1333333333333333315, 0.1375000000000000111, 0.1416666666666666630, 0.1458333333333333426, 0.1499999999999999944, 0.1541666666666666741, 0.1583333333333333259, 0.1625000000000000056, 0.1666666666666666574, 0.1708333333333333370, 0.1749999999999999889, 0.1791666666666666685, 0.1833333333333333204, 0.1875000000000000000, 0.1916666666666666796, 0.1958333333333333315, 0.2000000000000000111, 0.2041666666666666630, 0.2083333333333333426, 0.2124999999999999944, 0.2166666666666666741, 0.2208333333333333259, 0.2250000000000000056, 0.2291666666666666574, 0.2333333333333333370, 0.2374999999999999889, 0.2416666666666666685, 0.2458333333333333204, 0.2500000000000000000, 0.2541666666666666519, 0.2583333333333333592, 0.2625000000000000111, 0.2666666666666666630, 0.2708333333333333148, 0.2750000000000000222, 0.2791666666666666741, 0.2833333333333333259, 0.2874999999999999778, 0.2916666666666666852, 0.2958333333333333370, 0.2999999999999999889, 0.3041666666666666408, 0.3083333333333333481, 0.3125000000000000000, 0.3166666666666666519, 0.3208333333333333592, 0.3250000000000000111, 0.3291666666666666630, 0.3333333333333333148, 0.3375000000000000222, 0.3416666666666666741, 0.3458333333333333259, 0.3499999999999999778, 0.3541666666666666852, 0.3583333333333333370, 0.3624999999999999889, 0.3666666666666666408, 0.3708333333333333481, 0.3750000000000000000, 0.3791666666666666519, 0.3833333333333333592, 0.3875000000000000111, 0.3916666666666666630, 0.3958333333333333148, 0.4000000000000000222, 0.4041666666666666741, 0.4083333333333333259, 0.4124999999999999778, 0.4166666666666666852, 0.4208333333333333370, 0.4249999999999999889, 0.4291666666666666408, 0.4333333333333333481, 0.4375000000000000000, 0.4416666666666666519, 0.4458333333333333592, 0.4500000000000000111, 0.4541666666666666630, 0.4583333333333333148, 0.4625000000000000222, 0.4666666666666666741, 0.4708333333333333259, 0.4749999999999999778, 0.4791666666666666852, 0.4833333333333333370, 0.4874999999999999889, 0.4916666666666666408, 0.4958333333333333481, 0.5000000000000000000, 0.5041666666666666519, 0.5083333333333333037, 0.5124999999999999556, 0.5166666666666667185, 0.5208333333333333703, 0.5250000000000000222, 0.5291666666666666741, 0.5333333333333333259, 0.5374999999999999778, 0.5416666666666666297, 0.5458333333333332815, 0.5500000000000000444, 0.5541666666666666963, 0.5583333333333333481, 0.5625000000000000000, 0.5666666666666666519, 0.5708333333333333037, 0.5749999999999999556, 0.5791666666666667185, 0.5833333333333333703, 0.5875000000000000222, 0.5916666666666666741, 0.5958333333333333259, 0.5999999999999999778, 0.6041666666666666297, 0.6083333333333332815, 0.6125000000000000444, 0.6166666666666666963, 0.6208333333333333481, 0.6250000000000000000, 0.6291666666666666519, 0.6333333333333333037, 0.6374999999999999556, 0.6416666666666667185, 0.6458333333333333703, 0.6500000000000000222, 0.6541666666666666741, 0.6583333333333333259, 0.6624999999999999778, 0.6666666666666666297, 0.6708333333333332815, 0.6750000000000000444, 0.6791666666666666963, 0.6833333333333333481, 0.6875000000000000000, 0.6916666666666666519, 0.6958333333333333037, 0.6999999999999999556, 0.7041666666666667185, 0.7083333333333333703, 0.7125000000000000222, 0.7166666666666666741, 0.7208333333333333259, 0.7249999999999999778, 0.7291666666666666297, 0.7333333333333332815, 0.7375000000000000444, 0.7416666666666666963, 0.7458333333333333481, 0.7500000000000000000, 0.7541666666666666519, 0.7583333333333333037, 0.7624999999999999556, 0.7666666666666667185, 0.7708333333333333703, 0.7750000000000000222, 0.7791666666666666741, 0.7833333333333333259, 0.7874999999999999778, 0.7916666666666666297, 0.7958333333333332815, 0.8000000000000000444, 0.8041666666666666963, 0.8083333333333333481, 0.8125000000000000000, 0.8166666666666666519, 0.8208333333333333037, 0.8249999999999999556, 0.8291666666666667185, 0.8333333333333333703, 0.8375000000000000222, 0.8416666666666666741, 0.8458333333333333259, 0.8499999999999999778, 0.8541666666666666297, 0.8583333333333332815, 0.8625000000000000444, 0.8666666666666666963, 0.8708333333333333481, 0.8750000000000000000, 0.8791666666666666519, 0.8833333333333333037, 0.8874999999999999556, 0.8916666666666667185, 0.8958333333333333703, 0.9000000000000000222, 0.9041666666666666741, 0.9083333333333333259, 0.9124999999999999778, 0.9166666666666666297, 0.9208333333333332815, 0.9250000000000000444, 0.9291666666666666963, 0.9333333333333333481, 0.9375000000000000000, 0.9416666666666666519, 0.9458333333333333037, 0.9499999999999999556, 0.9541666666666667185, 0.9583333333333333703, 0.9625000000000000222, 0.9666666666666666741, 0.9708333333333333259, 0.9749999999999999778, 0.9791666666666666297, 0.9833333333333332815, 0.9875000000000000444, 0.9916666666666666963, 0.9958333333333333481, 1.000000000000000000 ),
 .UNSPECIFIED. ) 
 GEOMETRIC_REPRESENTATION_ITEM ( )  RATIONAL_B_SPLINE_SURFACE ( (
 ( 1.000000000000000000, 0.9238795325112867385, 1.000000000000000000, 0.9238795325112867385, 1.000000000000000000, 0.9238795325112867385, 1.000000000000000000, 0.9238795325112867385, 1.000000000000000000, 0.9238795325112867385, 1.000000000000000000, 0.9238795325112867385, 1.000000000000000000, 0.9238795325112867385, 1.000000000000000000, 0.9238795325112867385, 1.000000000000000000, 0.9238795325112867385, 1.000000000000000000, 0.9238795325112867385, 1.000000000000000000, 0.9238795325112867385, 1.000000000000000000, 0.9238795325112867385, 1.000000000000000000, 0.9238795325112867385, 1.000000000000000000, 0.9238795325112867385, 1.000000000000000000, 0.9238795325112867385, 1.000000000000000000, 0.9238795325112867385, 1.000000000000000000, 0.9238795325112867385, 1.000000000000000000, 0.9238795325112867385, 1.000000000000000000, 0.9238795325112867385, 1.000000000000000000, 0.9238795325112867385, 1.000000000000000000, 0.9238795325112867385, 1.000000000000000000, 0.9238795325112867385, 1.000000000000000000, 0.9238795325112867385, 1.000000000000000000, 0.9238795325112867385, 1.000000000000000000, 0.9238795325112867385, 1.000000000000000000, 0.9238795325112867385, 1.000000000000000000, 0.9238795325112867385, 1.000000000000000000, 0.9238795325112867385, 1.000000000000000000, 0.9238795325112867385, 1.000000000000000000, 0.9238795325112867385, 1.000000000000000000, 0.9238795325112867385, 1.000000000000000000, 0.9238795325112867385, 1.000000000000000000, 0.9238795325112867385, 1.000000000000000000, 0.9238795325112867385, 1.000000000000000000, 0.9238795325112867385, 1.000000000000000000, 0.9238795325112867385, 1.000000000000000000, 0.9238795325112867385, 1.000000000000000000, 0.9238795325112867385, 1.000000000000000000, 0.9238795325112867385, 1.000000000000000000, 0.9238795325112867385, 1.000000000000000000, 0.9238795325112867385, 1.000000000000000000, 0.9238795325112867385, 1.000000000000000000, 0.9238795325112867385, 1.000000000000000000, 0.9238795325112867385, 1.000000000000000000, 0.9238795325112867385, 1.000000000000000000, 0.9238795325112867385, 1.000000000000000000, 0.9238795325112867385, 1.000000000000000000, 0.9238795325112867385, 1.000000000000000000, 0.9238795325112867385, 1.000000000000000000, 0.9238795325112867385, 1.000000000000000000, 0.9238795325112867385, 1.000000000000000000, 0.9238795325112867385, 1.000000000000000000, 0.9238795325112867385, 1.000000000000000000, 0.9238795325112867385, 1.000000000000000000, 0.9238795325112867385, 1.000000000000000000, 0.9238795325112867385, 1.000000000000000000, 0.9238795325112867385, 1.000000000000000000, 0.9238795325112867385, 1.000000000000000000, 0.9238795325112867385, 1.000000000000000000, 0.9238795325112867385, 1.000000000000000000, 0.9238795325112867385, 1.000000000000000000, 0.9238795325112867385, 1.000000000000000000, 0.9238795325112867385, 1.000000000000000000, 0.9238795325112867385, 1.000000000000000000, 0.9238795325112867385, 1.000000000000000000, 0.9238795325112867385, 1.000000000000000000, 0.9238795325112867385, 1.000000000000000000, 0.9238795325112867385, 1.000000000000000000, 0.9238795325112867385, 1.000000000000000000, 0.9238795325112867385, 1.000000000000000000, 0.9238795325112867385, 1.000000000000000000, 0.9238795325112867385, 1.000000000000000000, 0.9238795325112867385, 1.000000000000000000, 0.9238795325112867385, 1.000000000000000000, 0.9238795325112867385, 1.000000000000000000, 0.9238795325112867385, 1.000000000000000000, 0.9238795325112867385, 1.000000000000000000, 0.9238795325112867385, 1.000000000000000000, 0.9238795325112867385, 1.000000000000000000, 0.9238795325112867385, 1.000000000000000000, 0.9238795325112867385, 1.000000000000000000, 0.9238795325112867385, 1.000000000000000000, 0.9238795325112867385, 1.000000000000000000, 0.9238795325112867385, 1.000000000000000000, 0.9238795325112867385, 1.000000000000000000, 0.9238795325112867385, 1.000000000000000000, 0.9238795325112867385, 1.000000000000000000, 0.9238795325112867385, 1.000000000000000000, 0.9238795325112867385, 1.000000000000000000, 0.9238795325112867385, 1.000000000000000000, 0.9238795325112867385, 1.000000000000000000, 0.9238795325112867385, 1.000000000000000000, 0.9238795325112867385, 1.000000000000000000, 0.9238795325112867385, 1.000000000000000000, 0.9238795325112867385, 1.000000000000000000, 0.9238795325112867385, 1.000000000000000000, 0.9238795325112867385, 1.000000000000000000, 0.9238795325112867385, 1.000000000000000000, 0.9238795325112867385, 1.000000000000000000, 0.9238795325112867385, 1.000000000000000000, 0.9238795325112867385, 1.000000000000000000, 0.9238795325112867385, 1.000000000000000000, 0.9238795325112867385, 1.000000000000000000, 0.9238795325112867385, 1.000000000000000000, 0.9238795325112867385, 1.000000000000000000, 0.9238795325112867385, 1.000000000000000000, 0.9238795325112867385, 1.000000000000000000, 0.9238795325112867385, 1.000000000000000000, 0.9238795325112867385, 1.000000000000000000, 0.9238795325112867385, 1.000000000000000000, 0.9238795325112867385, 1.000000000000000000, 0.9238795325112867385, 1.000000000000000000, 0.9238795325112867385, 1.000000000000000000, 0.9238795325112867385, 1.000000000000000000, 0.9238795325112867385, 1.000000000000000000, 0.9238795325112867385, 1.000000000000000000, 0.9238795325112867385, 1.000000000000000000, 0.9238795325112867385, 1.000000000000000000, 0.9238795325112867385, 1.000000000000000000, 0.9238795325112867385, 1.000000000000000000, 0.9238795325112867385, 1.000000000000000000, 0.9238795325112867385, 1.000000000000000000, 0.9238795325112867385, 1.000000000000000000, 0.9238795325112867385, 1.000000000000000000, 0.9238795325112867385, 1.000000000000000000, 0.9238795325112867385, 1.000000000000000000, 0.9238795325112867385, 1.000000000000000000, 0.9238795325112867385, 1.000000000000000000, 0.9238795325112867385, 1.000000000000000000, 0.9238795325112867385, 1.000000000000000000, 0.9238795325112867385, 1.000000000000000000, 0.9238795325112867385, 1.000000000000000000, 0.9238795325112867385, 1.000000000000000000, 0.9238795325112867385, 1.000000000000000000, 0.9238795325112867385, 1.000000000000000000, 0.9238795325112867385, 1.000000000000000000, 0.9238795325112867385, 1.000000000000000000, 0.9238795325112867385, 1.000000000000000000, 0.9238795325112867385, 1.000000000000000000, 0.9238795325112867385, 1.000000000000000000, 0.9238795325112867385, 1.000000000000000000, 0.9238795325112867385, 1.000000000000000000, 0.9238795325112867385, 1.000000000000000000, 0.9238795325112867385, 1.000000000000000000, 0.9238795325112867385, 1.000000000000000000, 0.9238795325112867385, 1.000000000000000000, 0.9238795325112867385, 1.000000000000000000, 0.9238795325112867385, 1.000000000000000000, 0.9238795325112867385, 1.000000000000000000, 0.9238795325112867385, 1.000000000000000000, 0.9238795325112867385, 1.000000000000000000, 0.9238795325112867385, 1.000000000000000000, 0.9238795325112867385, 1.000000000000000000, 0.9238795325112867385, 1.000000000000000000, 0.9238795325112867385, 1.000000000000000000, 0.9238795325112867385, 1.000000000000000000, 0.9238795325112867385, 1.000000000000000000, 0.9238795325112867385, 1.000000000000000000, 0.9238795325112867385, 1.000000000000000000, 0.9238795325112867385, 1.000000000000000000, 0.9238795325112867385, 1.000000000000000000, 0.9238795325112867385, 1.000000000000000000, 0.9238795325112867385, 1.000000000000000000, 0.9238795325112867385, 1.000000000000000000, 0.9238795325112867385, 1.000000000000000000, 0.9238795325112867385, 1.000000000000000000, 0.9238795325112867385, 1.000000000000000000, 0.9238795325112867385, 1.000000000000000000, 0.9238795325112867385, 1.000000000000000000, 0.9238795325112867385, 1.000000000000000000, 0.9238795325112867385, 1.000000000000000000, 0.9238795325112867385, 1.000000000000000000, 0.9238795325112867385, 1.000000000000000000, 0.9238795325112867385, 1.000000000000000000, 0.9238795325112867385, 1.000000000000000000, 0.9238795325112867385, 1.000000000000000000, 0.9238795325112867385, 1.000000000000000000, 0.9238795325112867385, 1.000000000000000000, 0.9238795325112867385, 1.000000000000000000, 0.9238795325112867385, 1.000000000000000000, 0.9238795325112867385, 1.000000000000000000, 0.9238795325112867385, 1.000000000000000000, 0.9238795325112867385, 1.000000000000000000, 0.9238795325112867385, 1.000000000000000000, 0.9238795325112867385, 1.000000000000000000, 0.9238795325112867385, 1.000000000000000000, 0.9238795325112867385, 1.000000000000000000, 0.9238795325112867385, 1.000000000000000000, 0.9238795325112867385, 1.000000000000000000, 0.9238795325112867385, 1.000000000000000000, 0.9238795325112867385, 1.000000000000000000, 0.9238795325112867385, 1.000000000000000000, 0.9238795325112867385, 1.000000000000000000, 0.9238795325112867385, 1.000000000000000000, 0.9238795325112867385, 1.000000000000000000, 0.9238795325112867385, 1.000000000000000000, 0.9238795325112867385, 1.000000000000000000, 0.9238795325112867385, 1.000000000000000000, 0.9238795325112867385, 1.000000000000000000, 0.9238795325112867385, 1.000000000000000000, 0.9238795325112867385, 1.000000000000000000, 0.9238795325112867385, 1.000000000000000000, 0.9238795325112867385, 1.000000000000000000, 0.9238795325112867385, 1.000000000000000000, 0.9238795325112867385, 1.000000000000000000, 0.9238795325112867385, 1.000000000000000000, 0.9238795325112867385, 1.000000000000000000, 0.9238795325112867385, 1.000000000000000000, 0.9238795325112867385, 1.000000000000000000, 0.9238795325112867385, 1.000000000000000000, 0.9238795325112867385, 1.000000000000000000, 0.9238795325112867385, 1.000000000000000000, 0.9238795325112867385, 1.000000000000000000, 0.9238795325112867385, 1.000000000000000000, 0.9238795325112867385, 1.000000000000000000, 0.9238795325112867385, 1.000000000000000000, 0.9238795325112867385, 1.000000000000000000, 0.9238795325112867385, 1.000000000000000000, 0.9238795325112867385, 1.000000000000000000, 0.9238795325112867385, 1.000000000000000000, 0.9238795325112867385, 1.000000000000000000, 0.9238795325112867385, 1.000000000000000000, 0.9238795325112867385, 1.000000000000000000, 0.9238795325112867385, 1.000000000000000000, 0.9238795325112867385, 1.000000000000000000, 0.9238795325112867385, 1.000000000000000000, 0.9238795325112867385, 1.000000000000000000, 0.9238795325112867385, 1.000000000000000000, 0.9238795325112867385, 1.000000000000000000, 0.9238795325112867385, 1.000000000000000000, 0.9238795325112867385, 1.000000000000000000, 0.9238795325112867385, 1.000000000000000000, 0.9238795325112867385, 1.000000000000000000, 0.9238795325112867385, 1.000000000000000000, 0.9238795325112867385, 1.000000000000000000, 0.9238795325112867385, 1.000000000000000000, 0.9238795325112867385, 1.000000000000000000, 0.9238795325112867385, 1.000000000000000000, 0.9238795325112867385, 1.000000000000000000, 0.9238795325112867385, 1.000000000000000000),
 ( 1.000000000000000000, 0.9238795325112867385, 1.000000000000000000, 0.9238795325112867385, 1.000000000000000000, 0.9238795325112867385, 1.000000000000000000, 0.9238795325112867385, 1.000000000000000000, 0.9238795325112867385, 1.000000000000000000, 0.9238795325112867385, 1.000000000000000000, 0.9238795325112867385, 1.000000000000000000, 0.9238795325112867385, 1.000000000000000000, 0.9238795325112867385, 1.000000000000000000, 0.9238795325112867385, 1.000000000000000000, 0.9238795325112867385, 1.000000000000000000, 0.9238795325112867385, 1.000000000000000000, 0.9238795325112867385, 1.000000000000000000, 0.9238795325112867385, 1.000000000000000000, 0.9238795325112867385, 1.000000000000000000, 0.9238795325112867385, 1.000000000000000000, 0.9238795325112867385, 1.000000000000000000, 0.9238795325112867385, 1.000000000000000000, 0.9238795325112867385, 1.000000000000000000, 0.9238795325112867385, 1.000000000000000000, 0.9238795325112867385, 1.000000000000000000, 0.9238795325112867385, 1.000000000000000000, 0.9238795325112867385, 1.000000000000000000, 0.9238795325112867385, 1.000000000000000000, 0.9238795325112867385, 1.000000000000000000, 0.9238795325112867385, 1.000000000000000000, 0.9238795325112867385, 1.000000000000000000, 0.9238795325112867385, 1.000000000000000000, 0.9238795325112867385, 1.000000000000000000, 0.9238795325112867385, 1.000000000000000000, 0.9238795325112867385, 1.000000000000000000, 0.9238795325112867385, 1.000000000000000000, 0.9238795325112867385, 1.000000000000000000, 0.9238795325112867385, 1.000000000000000000, 0.9238795325112867385, 1.000000000000000000, 0.9238795325112867385, 1.000000000000000000, 0.9238795325112867385, 1.000000000000000000, 0.9238795325112867385, 1.000000000000000000, 0.9238795325112867385, 1.000000000000000000, 0.9238795325112867385, 1.000000000000000000, 0.9238795325112867385, 1.000000000000000000, 0.9238795325112867385, 1.000000000000000000, 0.9238795325112867385, 1.000000000000000000, 0.9238795325112867385, 1.000000000000000000, 0.9238795325112867385, 1.000000000000000000, 0.9238795325112867385, 1.000000000000000000, 0.9238795325112867385, 1.000000000000000000, 0.9238795325112867385, 1.000000000000000000, 0.9238795325112867385, 1.000000000000000000, 0.9238795325112867385, 1.000000000000000000, 0.9238795325112867385, 1.000000000000000000, 0.9238795325112867385, 1.000000000000000000, 0.9238795325112867385, 1.000000000000000000, 0.9238795325112867385, 1.000000000000000000, 0.9238795325112867385, 1.000000000000000000, 0.9238795325112867385, 1.000000000000000000, 0.9238795325112867385, 1.000000000000000000, 0.9238795325112867385, 1.000000000000000000, 0.9238795325112867385, 1.000000000000000000, 0.9238795325112867385, 1.000000000000000000, 0.9238795325112867385, 1.000000000000000000, 0.9238795325112867385, 1.000000000000000000, 0.9238795325112867385, 1.000000000000000000, 0.9238795325112867385, 1.000000000000000000, 0.9238795325112867385, 1.000000000000000000, 0.9238795325112867385, 1.000000000000000000, 0.9238795325112867385, 1.000000000000000000, 0.9238795325112867385, 1.000000000000000000, 0.9238795325112867385, 1.000000000000000000, 0.9238795325112867385, 1.000000000000000000, 0.9238795325112867385, 1.000000000000000000, 0.9238795325112867385, 1.000000000000000000, 0.9238795325112867385, 1.000000000000000000, 0.9238795325112867385, 1.000000000000000000, 0.9238795325112867385, 1.000000000000000000, 0.9238795325112867385, 1.000000000000000000, 0.9238795325112867385, 1.000000000000000000, 0.9238795325112867385, 1.000000000000000000, 0.9238795325112867385, 1.000000000000000000, 0.9238795325112867385, 1.000000000000000000, 0.9238795325112867385, 1.000000000000000000, 0.9238795325112867385, 1.000000000000000000, 0.9238795325112867385, 1.000000000000000000, 0.9238795325112867385, 1.000000000000000000, 0.9238795325112867385, 1.000000000000000000, 0.9238795325112867385, 1.000000000000000000, 0.9238795325112867385, 1.000000000000000000, 0.9238795325112867385, 1.000000000000000000, 0.9238795325112867385, 1.000000000000000000, 0.9238795325112867385, 1.000000000000000000, 0.9238795325112867385, 1.000000000000000000, 0.9238795325112867385, 1.000000000000000000, 0.9238795325112867385, 1.000000000000000000, 0.9238795325112867385, 1.000000000000000000, 0.9238795325112867385, 1.000000000000000000, 0.9238795325112867385, 1.000000000000000000, 0.9238795325112867385, 1.000000000000000000, 0.9238795325112867385, 1.000000000000000000, 0.9238795325112867385, 1.000000000000000000, 0.9238795325112867385, 1.000000000000000000, 0.9238795325112867385, 1.000000000000000000, 0.9238795325112867385, 1.000000000000000000, 0.9238795325112867385, 1.000000000000000000, 0.9238795325112867385, 1.000000000000000000, 0.9238795325112867385, 1.000000000000000000, 0.9238795325112867385, 1.000000000000000000, 0.9238795325112867385, 1.000000000000000000, 0.9238795325112867385, 1.000000000000000000, 0.9238795325112867385, 1.000000000000000000, 0.9238795325112867385, 1.000000000000000000, 0.9238795325112867385, 1.000000000000000000, 0.9238795325112867385, 1.000000000000000000, 0.9238795325112867385, 1.000000000000000000, 0.9238795325112867385, 1.000000000000000000, 0.9238795325112867385, 1.000000000000000000, 0.9238795325112867385, 1.000000000000000000, 0.9238795325112867385, 1.000000000000000000, 0.9238795325112867385, 1.000000000000000000, 0.9238795325112867385, 1.000000000000000000, 0.9238795325112867385, 1.000000000000000000, 0.9238795325112867385, 1.000000000000000000, 0.9238795325112867385, 1.000000000000000000, 0.9238795325112867385, 1.000000000000000000, 0.9238795325112867385, 1.000000000000000000, 0.9238795325112867385, 1.000000000000000000, 0.9238795325112867385, 1.000000000000000000, 0.9238795325112867385, 1.000000000000000000, 0.9238795325112867385, 1.000000000000000000, 0.9238795325112867385, 1.000000000000000000, 0.9238795325112867385, 1.000000000000000000, 0.9238795325112867385, 1.000000000000000000, 0.9238795325112867385, 1.000000000000000000, 0.9238795325112867385, 1.000000000000000000, 0.9238795325112867385, 1.000000000000000000, 0.9238795325112867385, 1.000000000000000000, 0.9238795325112867385, 1.000000000000000000, 0.9238795325112867385, 1.000000000000000000, 0.9238795325112867385, 1.000000000000000000, 0.9238795325112867385, 1.000000000000000000, 0.9238795325112867385, 1.000000000000000000, 0.9238795325112867385, 1.000000000000000000, 0.9238795325112867385, 1.000000000000000000, 0.9238795325112867385, 1.000000000000000000, 0.9238795325112867385, 1.000000000000000000, 0.9238795325112867385, 1.000000000000000000, 0.9238795325112867385, 1.000000000000000000, 0.9238795325112867385, 1.000000000000000000, 0.9238795325112867385, 1.000000000000000000, 0.9238795325112867385, 1.000000000000000000, 0.9238795325112867385, 1.000000000000000000, 0.9238795325112867385, 1.000000000000000000, 0.9238795325112867385, 1.000000000000000000, 0.9238795325112867385, 1.000000000000000000, 0.9238795325112867385, 1.000000000000000000, 0.9238795325112867385, 1.000000000000000000, 0.9238795325112867385, 1.000000000000000000, 0.9238795325112867385, 1.000000000000000000, 0.9238795325112867385, 1.000000000000000000, 0.9238795325112867385, 1.000000000000000000, 0.9238795325112867385, 1.000000000000000000, 0.9238795325112867385, 1.000000000000000000, 0.9238795325112867385, 1.000000000000000000, 0.9238795325112867385, 1.000000000000000000, 0.9238795325112867385, 1.000000000000000000, 0.9238795325112867385, 1.000000000000000000, 0.9238795325112867385, 1.000000000000000000, 0.9238795325112867385, 1.000000000000000000, 0.9238795325112867385, 1.000000000000000000, 0.9238795325112867385, 1.000000000000000000, 0.9238795325112867385, 1.000000000000000000, 0.9238795325112867385, 1.000000000000000000, 0.9238795325112867385, 1.000000000000000000, 0.9238795325112867385, 1.000000000000000000, 0.9238795325112867385, 1.000000000000000000, 0.9238795325112867385, 1.000000000000000000, 0.9238795325112867385, 1.000000000000000000, 0.9238795325112867385, 1.000000000000000000, 0.9238795325112867385, 1.000000000000000000, 0.9238795325112867385, 1.000000000000000000, 0.9238795325112867385, 1.000000000000000000, 0.9238795325112867385, 1.000000000000000000, 0.9238795325112867385, 1.000000000000000000, 0.9238795325112867385, 1.000000000000000000, 0.9238795325112867385, 1.000000000000000000, 0.9238795325112867385, 1.000000000000000000, 0.9238795325112867385, 1.000000000000000000, 0.9238795325112867385, 1.000000000000000000, 0.9238795325112867385, 1.000000000000000000, 0.9238795325112867385, 1.000000000000000000, 0.9238795325112867385, 1.000000000000000000, 0.9238795325112867385, 1.000000000000000000, 0.9238795325112867385, 1.000000000000000000, 0.9238795325112867385, 1.000000000000000000, 0.9238795325112867385, 1.000000000000000000, 0.9238795325112867385, 1.000000000000000000, 0.9238795325112867385, 1.000000000000000000, 0.9238795325112867385, 1.000000000000000000, 0.9238795325112867385, 1.000000000000000000, 0.9238795325112867385, 1.000000000000000000, 0.9238795325112867385, 1.000000000000000000, 0.9238795325112867385, 1.000000000000000000, 0.9238795325112867385, 1.000000000000000000, 0.9238795325112867385, 1.000000000000000000, 0.9238795325112867385, 1.000000000000000000, 0.9238795325112867385, 1.000000000000000000, 0.9238795325112867385, 1.000000000000000000, 0.9238795325112867385, 1.000000000000000000, 0.9238795325112867385, 1.000000000000000000, 0.9238795325112867385, 1.000000000000000000, 0.9238795325112867385, 1.000000000000000000, 0.9238795325112867385, 1.000000000000000000, 0.9238795325112867385, 1.000000000000000000, 0.9238795325112867385, 1.000000000000000000, 0.9238795325112867385, 1.000000000000000000, 0.9238795325112867385, 1.000000000000000000, 0.9238795325112867385, 1.000000000000000000, 0.9238795325112867385, 1.000000000000000000, 0.9238795325112867385, 1.000000000000000000, 0.9238795325112867385, 1.000000000000000000, 0.9238795325112867385, 1.000000000000000000, 0.9238795325112867385, 1.000000000000000000, 0.9238795325112867385, 1.000000000000000000, 0.9238795325112867385, 1.000000000000000000, 0.9238795325112867385, 1.000000000000000000, 0.9238795325112867385, 1.000000000000000000, 0.9238795325112867385, 1.000000000000000000, 0.9238795325112867385, 1.000000000000000000, 0.9238795325112867385, 1.000000000000000000, 0.9238795325112867385, 1.000000000000000000, 0.9238795325112867385, 1.000000000000000000, 0.9238795325112867385, 1.000000000000000000, 0.9238795325112867385, 1.000000000000000000, 0.9238795325112867385, 1.000000000000000000, 0.9238795325112867385, 1.000000000000000000, 0.9238795325112867385, 1.000000000000000000, 0.9238795325112867385, 1.000000000000000000, 0.9238795325112867385, 1.000000000000000000, 0.9238795325112867385, 1.000000000000000000, 0.9238795325112867385, 1.000000000000000000, 0.9238795325112867385, 1.000000000000000000) ) ) 
 REPRESENTATION_ITEM ( '' )  SURFACE ( )  );
#32288=CARTESIAN_POINT ( 'NONE',  ( -9.184850993605147944E-16, -157.2500000000000000, 5.000000000000000000 ) ) ;
#32290=CARTESIAN_POINT ( 'NONE',  ( -2.229367062499996610, 15.85416666803226171, 3.861377020970582219 ) ) ;
#32293=CARTESIAN_POINT ( 'NONE',  ( 2.071067811865540342, -165.1875000000000284, 4.999999999999936051 ) ) ;
#32296=CARTESIAN_POINT ( 'NONE',  ( -1.339745962155610925, -85.66965819600731891, 5.000000000000000000 ) ) ;
#32301=CARTESIAN_POINT ( 'NONE',  ( -9.184850993605147944E-16, -139.3750000027312126, 5.000000000000000000 ) ) ;
#32302=CARTESIAN_POINT ( 'NONE',  ( 6.042630808230842148E-15, 25.87500000273118062, -4.999999999999999112 ) ) ;
#32303=DIRECTION ( 'NONE',  ( 0.000000000000000000, 0.000000000000000000, 1.000000000000000000 ) ) ;
#32309=CARTESIAN_POINT ( 'NONE',  ( 3.535533905932736864, -155.2500000027312126, 3.535533905932738641 ) ) ;
#32315=CARTESIAN_POINT ( 'NONE',  ( 2.071067811865475505, -146.8125000000000000, -5.000000000000000888 ) ) ;
#32319=CARTESIAN_POINT ( 'NONE',  ( 1.975475456537005874E-15, -54.74999999999999289, 5.000000000000000000 ) ) ;
#32320=CARTESIAN_POINT ( 'NONE',  ( -4.458734124999997661, -23.22916666530107221, 2.574251347313722516 ) ) ;
#32321=EDGE_CURVE ( 'NONE', #13039, #34762, #6553, .T. ) ;
#32322=CARTESIAN_POINT ( 'NONE',  ( -6.972266317189433020E-16, 6.875000002731185944, -5.000000000000000000 ) ) ;
#32325=CARTESIAN_POINT ( 'NONE',  ( -1.846868145590734756, -147.1250000013656063, -4.458734125000000326 ) ) ;
#32327=CARTESIAN_POINT ( 'NONE',  ( 3.535533905932736864, -150.1250000000000000, 3.535533905932738641 ) ) ;
#32328=CARTESIAN_POINT ( 'NONE',  ( 4.458734124999998549, -51.97916666530107221, -2.574251347313721627 ) ) ;
#32329=EDGE_CURVE ( 'NONE', #30019, #42348, #63402, .T. ) ;
#32330=CARTESIAN_POINT ( 'NONE',  ( 5.000000000000000000, -2.500000000000002220, -6.123233995736766282E-16 ) ) ;
#32332=CARTESIAN_POINT ( 'NONE',  ( -5.000000000000000000, 25.91666666666666430, -2.886751345948128211 ) ) ;
#32335=CYLINDRICAL_SURFACE ( 'NONE', #42734, 5.000000000000000000 ) ;
#32336=VECTOR ( 'NONE', #3881, 1000.000000000000000 ) ;
#32337=CARTESIAN_POINT ( 'NONE',  ( -2.229367062499996610, 0.8541666680322613781, 3.861377020970582219 ) ) ;
#32338=CARTESIAN_POINT ( 'NONE',  ( -6.972266317189433020E-16, -48.24999999999999289, -5.000000000000000000 ) ) ;
#32340=CARTESIAN_POINT ( 'NONE',  ( -4.999999999999998224, -73.91666666666667140, 2.886751345948131764 ) ) ;
#32341=CARTESIAN_POINT ( 'NONE',  ( 2.229367062500001939, 10.77083333469892956, 3.861377020970579999 ) ) ;
#32343=ORIENTED_EDGE ( 'NONE', *, *, #23697, .F. ) ;
#32347=CARTESIAN_POINT ( 'NONE',  ( 5.000000000000000000, -7.374999997268813168, -6.123233995736766282E-16 ) ) ;
#32348=CARTESIAN_POINT ( 'NONE',  ( 4.458734124999999437, -47.81249999863440792, -5.460374474430324690E-16 ) ) ;
#32349=ADVANCED_FACE ( 'NONE', ( #38615 ), #28031, .T. ) ;
#32350=CARTESIAN_POINT ( 'NONE',  ( 4.458734124999999437, -165.6875000013655779, 0.000000000000000000 ) ) ;
#32351=EDGE_CURVE ( 'NONE', #37665, #53636, #38005, .T. ) ;
#32352=CARTESIAN_POINT ( 'NONE',  ( -5.000000000000000000, -43.87499999726880873, 0.000000000000000000 ) ) ;
#32354=CARTESIAN_POINT ( 'NONE',  ( -4.458734124999999437, -21.31249999863440436, 0.000000000000000000 ) ) ;
#32355=ORIENTED_EDGE ( 'NONE', *, *, #52292, .T. ) ;
#32357=CARTESIAN_POINT ( 'NONE',  ( 4.458734125000000326, -164.3750000013656063, -1.846868145590734978 ) ) ;
#32360=CARTESIAN_POINT ( 'NONE',  ( -4.458734124999999437, -36.64583333196773651, -2.574251347313719407 ) ) ;
#32361=ORIENTED_EDGE ( 'NONE', *, *, #48718, .T. ) ;
#32366=CARTESIAN_POINT ( 'NONE',  ( -2.499999999999996447, -59.70833333060214443, 4.330127018922195425 ) ) ;
#32368=CARTESIAN_POINT ( 'NONE',  ( 4.458734124999999437, -81.06249999863440792, -5.460374474430324690E-16 ) ) ;
#32370=CARTESIAN_POINT ( 'NONE',  ( 3.535533905932738197, -142.8750000000000000, -3.535533905932738197 ) ) ;
#32371=CARTESIAN_POINT ( 'NONE',  ( 1.846868145590736310, -139.8750000013656063, 4.458734124999997661 ) ) ;
#32372=( BOUNDED_CURVE ( )  B_SPLINE_CURVE ( 2, ( #57433, #62576, #56801, #57120, #32655, #51965, #7904, #27825, #17230 ),
 .UNSPECIFIED., .F., .F. ) 
 B_SPLINE_CURVE_WITH_KNOTS ( ( 3, 2, 2, 2, 3 ),
 ( 0.9583333333333331483, 0.9624999999999998002, 0.9666666666666665630, 0.9708333333333332149, 0.9749999999999998668 ),
 .UNSPECIFIED. ) 
 CURVE ( )  GEOMETRIC_REPRESENTATION_ITEM ( )  RATIONAL_B_SPLINE_CURVE ( ( 1.000000000000003997, 0.9238795325112826307, 1.000000000000000000, 0.9238795325112867385, 1.000000000000000000, 0.9238795325112867385, 1.000000000000000000, 0.9238795325112887369, 0.9999999999999980016 ) ) 
 REPRESENTATION_ITEM ( '' )  );
#32373=CARTESIAN_POINT ( 'NONE',  ( -4.999999999999998224, -46.79166666393547303, 2.886751345948131764 ) ) ;
#32379=CARTESIAN_POINT ( 'NONE',  ( 5.000000000000000000, -159.1250000027311842, 0.000000000000000000 ) ) ;
#32382=CARTESIAN_POINT ( 'NONE',  ( 1.975475456537005874E-15, 16.37500000273118417, 5.000000000000000000 ) ) ;
#32384=CARTESIAN_POINT ( 'NONE',  ( -4.458734124999999437, -79.56249999863440792, 0.000000000000000000 ) ) ;
#32390=CARTESIAN_POINT ( 'NONE',  ( -5.000000000000000888, -165.6875000027312126, -2.071067811865475949 ) ) ;
#32392=CARTESIAN_POINT ( 'NONE',  ( 9.457646018065525792E-16, 13.68750000136559386, 5.148502694627439702 ) ) ;
#32393=FACE_OUTER_BOUND ( 'NONE', #51353, .T. ) ;
#32398=CARTESIAN_POINT ( 'NONE',  ( -3.535533905932738641, -163.3750000000000284, 3.535533905932737309 ) ) ;
#32399=CARTESIAN_POINT ( 'NONE',  ( -2.499999999999996447, -21.70833333060214798, 4.330127018922195425 ) ) ;
#32400=CARTESIAN_POINT ( 'NONE',  ( 4.458734125000000326, -7.895833331967735624, 2.574251347313718519 ) ) ;
#32402=ORIENTED_EDGE ( 'NONE', *, *, #16200, .T. ) ;
#32403=CARTESIAN_POINT ( 'NONE',  ( -4.458734124999999437, -35.64583333196772941, -2.574251347313719407 ) ) ;
#32408=CARTESIAN_POINT ( 'NONE',  ( 3.152801135295366208, -149.8125000013655779, 3.152801135295367985 ) ) ;
#32409=CARTESIAN_POINT ( 'NONE',  ( -4.458734124999999437, 15.68750000136559564, 0.000000000000000000 ) ) ;
#32412=CARTESIAN_POINT ( 'NONE',  ( 4.458734124999998549, -85.97916666530107932, -2.574251347313721627 ) ) ;
#32415=CARTESIAN_POINT ( 'NONE',  ( 2.500000000000002220, 20.45833333606451987, 4.330127018922192761 ) ) ;
#32417=CARTESIAN_POINT ( 'NONE',  ( 2.499999999999998668, -79.33333333333332860, -4.330127018922193649 ) ) ;
#32420=CARTESIAN_POINT ( 'NONE',  ( 2.500000000000002220, -27.66666666666666430, 4.330127018922192761 ) ) ;
#32421=CARTESIAN_POINT ( 'NONE',  ( 4.458734124999999437, -34.81249999863440792, -5.460374474430324690E-16 ) ) ;
#32422=LINE ( 'NONE', #14603, #44797 ) ;
#32423=VECTOR ( 'NONE', #35390, 1000.000000000000000 ) ;
#32424=EDGE_CURVE ( 'NONE', #37331, #45160, #58570, .T. ) ;
#32425=CARTESIAN_POINT ( 'NONE',  ( -3.535250795749689387E-16, -27.12499999726881583, -5.773502691896257311 ) ) ;
#32426=CARTESIAN_POINT ( 'NONE',  ( -3.152548672688508926E-16, -60.56249999863440792, -5.148502694627439702 ) ) ;
#32427=VERTEX_POINT ( 'NONE', #47960 ) ;
#32429=CARTESIAN_POINT ( 'NONE',  ( 4.458734125000001214, -8.145833331967736513, 2.574251347313718519 ) ) ;
#32431=CARTESIAN_POINT ( 'NONE',  ( -2.500000000000000444, -69.16666666666667140, -4.330127018922193649 ) ) ;
#32434=CARTESIAN_POINT ( 'NONE',  ( -5.000000000000000000, -75.95833333060215864, -2.886751345948128211 ) ) ;
#32435=CARTESIAN_POINT ( 'NONE',  ( 1.339745962155615144, -13.70534180126148094, 4.999999999999999112 ) ) ;
#32438=CARTESIAN_POINT ( 'NONE',  ( 9.457646018065525792E-16, -14.31249999863440259, 5.148502694627439702 ) ) ;
#32439=CARTESIAN_POINT ( 'NONE',  ( 2.229367062499998831, -58.89583333196773651, -3.861377020970580887 ) ) ;
#32440=CARTESIAN_POINT ( 'NONE',  ( 1.975475456537005874E-15, -10.62499999726881228, 5.000000000000000000 ) ) ;
#32441=CARTESIAN_POINT ( 'NONE',  ( 4.458734125000000326, -142.3750000013656063, -1.846868145590734978 ) ) ;
#32443=CARTESIAN_POINT ( 'NONE',  ( 3.535533905932738197, -148.0000000027311842, -3.535533905932738197 ) ) ;
#32444=ORIENTED_EDGE ( 'NONE', *, *, #41778, .T. ) ;
#32450=CARTESIAN_POINT ( 'NONE',  ( -3.152801135295367096, -146.3125000013655779, -3.152801135295367541 ) ) ;
#32454=CARTESIAN_POINT ( 'NONE',  ( -4.458734124999999437, -64.56249999863440792, 0.000000000000000000 ) ) ;
#32457=CARTESIAN_POINT ( 'NONE',  ( 2.730187237215162345E-16, -145.1875000013656063, -4.458734124999999437 ) ) ;
#32466=CARTESIAN_POINT ( 'NONE',  ( 2.229367062500001939, 26.77083333469892423, 3.861377020970579999 ) ) ;
#32468=AXIS2_PLACEMENT_3D ( 'NONE', #23985, #8880, #14638 ) ;
#32469=( BOUNDED_CURVE ( )  B_SPLINE_CURVE ( 2, ( #14621, #62898, #39378, #59009, #14937, #38744, #18812, #63212, #54180 ),
 .UNSPECIFIED., .F., .F. ) 
 B_SPLINE_CURVE_WITH_KNOTS ( ( 3, 2, 2, 2, 3 ),
 ( 0.7312499999999999556, 0.7319444444444443976, 0.7333333333333332815, 0.7347222222222222765, 0.7354166666666667185 ),
 .UNSPECIFIED. ) 
 CURVE ( )  GEOMETRIC_REPRESENTATION_ITEM ( )  RATIONAL_B_SPLINE_CURVE ( ( 0.9330127018922194093, 0.9330127018922194093, 1.000000000000000000, 0.8660254037844387076, 1.000000000000000000, 0.8660254037844387076, 1.000000000000000000, 0.9330127018922194093, 0.9330127018922194093 ) ) 
 REPRESENTATION_ITEM ( '' )  );
#32472=CARTESIAN_POINT ( 'NONE',  ( 5.000000000000000000, -56.37499999726880162, -6.123233995736766282E-16 ) ) ;
#32473=CYLINDRICAL_SURFACE ( 'NONE', #29454, 5.000000000000000000 ) ;
#32474=CARTESIAN_POINT ( 'NONE',  ( -4.458734124999999437, 5.687500001365592972, 0.000000000000000000 ) ) ;
#32476=CARTESIAN_POINT ( 'NONE',  ( 4.458734124999999437, -21.06249999863440436, -5.460374474430324690E-16 ) ) ;
#32478=CARTESIAN_POINT ( 'NONE',  ( 4.458734124999999437, -158.4375000013655779, 0.000000000000000000 ) ) ;
#32479=CARTESIAN_POINT ( 'NONE',  ( 1.339745962155602488, 15.41965820146970323, 5.000000000000007105 ) ) ;
#32483=CARTESIAN_POINT ( 'NONE',  ( -4.458734124999997661, -40.22916666530107932, 2.574251347313722516 ) ) ;
#32485=CARTESIAN_POINT ( 'NONE',  ( 4.458734125000000326, -68.14583333196773651, 2.574251347313718519 ) ) ;
#32487=CARTESIAN_POINT ( 'NONE',  ( -5.000000000000000000, -40.99999999999999289, 0.000000000000000000 ) ) ;
#32488=CARTESIAN_POINT ( 'NONE',  ( 5.000000000000000888, -68.45833333060214443, 2.886751345948126879 ) ) ;
#32489=EDGE_LOOP ( 'NONE', ( #58821, #49185, #27584, #56073 ) ) ;
#32491=CARTESIAN_POINT ( 'NONE',  ( -1.339745962155610925, -67.66965819600733312, 5.000000000000000000 ) ) ;
#32492=CARTESIAN_POINT ( 'NONE',  ( 1.060575238724906964E-15, -14.75000000000000000, 5.773502691896257311 ) ) ;
#32493=CARTESIAN_POINT ( 'NONE',  ( 2.229367062499998831, -14.64583333196773474, -3.861377020970580887 ) ) ;
#32494=CARTESIAN_POINT ( 'NONE',  ( -4.458734124999997661, -78.22916666530106511, 2.574251347313722516 ) ) ;
#32496=CARTESIAN_POINT ( 'NONE',  ( -4.999999999999999112, -11.79166666393547835, 2.886751345948131764 ) ) ;
#32497=CARTESIAN_POINT ( 'NONE',  ( 9.457646018065525792E-16, -43.06249999863440081, 5.148502694627439702 ) ) ;
#32500=CARTESIAN_POINT ( 'NONE',  ( -4.458734124999999437, 8.354166668032261711, -2.574251347313719407 ) ) ;
#32503=CARTESIAN_POINT ( 'NONE',  ( 2.499999999999998668, -54.33333333333332860, -4.330127018922193649 ) ) ;
#32504=CARTESIAN_POINT ( 'NONE',  ( 3.152801135295366208, -160.8125000013656063, 3.152801135295367985 ) ) ;
#32507=CARTESIAN_POINT ( 'NONE',  ( 4.458734124999999437, -81.81249999863440792, -5.460374474430324690E-16 ) ) ;
#32508=CARTESIAN_POINT ( 'NONE',  ( 2.071067811865476394, -168.1875000000000284, 5.000000000000000000 ) ) ;
#32511=CARTESIAN_POINT ( 'NONE',  ( -2.229367062500000163, 1.270833334698927342, -3.861377020970580443 ) ) ;
#32513=CARTESIAN_POINT ( 'NONE',  ( -4.458734124999998549, -42.47916666530107932, 2.574251347313722516 ) ) ;
#32516=CARTESIAN_POINT ( 'NONE',  ( 0.000000000000000000, -170.0000000000000000, 0.000000000000000000 ) ) ;
#32520=( BOUNDED_CURVE ( )  B_SPLINE_CURVE ( 2, ( #46014, #36363, #16746, #21254, #7737 ),
 .UNSPECIFIED., .F., .F. ) 
 B_SPLINE_CURVE_WITH_KNOTS ( ( 3, 2, 3 ),
 ( 0.9916666666666665853, 0.9958333333333333481, 1.000000000000000000 ),
 .UNSPECIFIED. ) 
 CURVE ( )  GEOMETRIC_REPRESENTATION_ITEM ( )  RATIONAL_B_SPLINE_CURVE ( ( 1.000000000000001998, 0.9238795325112847401, 1.000000000000000000, 0.9238795325112867385, 1.000000000000000000 ) ) 
 REPRESENTATION_ITEM ( '' )  );
#32521=CARTESIAN_POINT ( 'NONE',  ( 6.123233995736766282E-16, -170.0000000000000000, -5.000000000000000000 ) ) ;
#32522=CARTESIAN_POINT ( 'NONE',  ( 9.457646018065525792E-16, -72.31249999863440792, 5.148502694627439702 ) ) ;
#32526=CARTESIAN_POINT ( 'NONE',  ( 3.061616997868383141E-16, -150.8750000027312126, -5.000000000000000000 ) ) ;
#32530=CARTESIAN_POINT ( 'NONE',  ( -4.458734124999999437, 4.687500001365595637, 0.000000000000000000 ) ) ;
#32531=CARTESIAN_POINT ( 'NONE',  ( 3.152801135295366208, -155.5625000013656063, 3.152801135295367985 ) ) ;
#32533=VERTEX_POINT ( 'NONE', #5487 ) ;
#32537=FACE_OUTER_BOUND ( 'NONE', #53620, .T. ) ;
#32546=CARTESIAN_POINT ( 'NONE',  ( -2.229367062499996610, 20.85416666803226349, 3.861377020970582219 ) ) ;
#32548=CARTESIAN_POINT ( 'NONE',  ( -4.458734124999997661, -1.479166665301071992, 2.574251347313722516 ) ) ;
#32550=DIRECTION ( 'NONE',  ( 0.000000000000000000, 0.000000000000000000, 1.000000000000000000 ) ) ;
#32552=CARTESIAN_POINT ( 'NONE',  ( 2.071067811865475505, -142.9375000027312126, -5.000000000000000888 ) ) ;
#32557=AXIS2_PLACEMENT_3D ( 'NONE', #41401, #36908, #7961 ) ;
#32559=CYLINDRICAL_SURFACE ( 'NONE', #19541, 5.000000000000000000 ) ;
#32561=AXIS2_PLACEMENT_3D ( 'NONE', #38473, #19165, #48445 ) ;
#32563=CARTESIAN_POINT ( 'NONE',  ( -3.152801135295367985, -158.0625000013656063, 3.152801135295367096 ) ) ;
#32567=CARTESIAN_POINT ( 'NONE',  ( 2.229367062499998831, 18.10416666803225993, -3.861377020970580887 ) ) ;
#32568=VERTEX_POINT ( 'NONE', #35081 ) ;
#32574=CARTESIAN_POINT ( 'NONE',  ( 5.000000000000000000, 10.49999999999999822, -6.123233995736766282E-16 ) ) ;
#32575=CARTESIAN_POINT ( 'NONE',  ( 2.229367062500001939, -54.97916666530107221, 3.861377020970579999 ) ) ;
#32578=CARTESIAN_POINT ( 'NONE',  ( -4.458734124999998549, -30.22916666530106866, 2.574251347313722516 ) ) ;
#32581=CARTESIAN_POINT ( 'NONE',  ( 0.000000000000000000, -170.0000000000000000, 0.000000000000000000 ) ) ;
#32582=CARTESIAN_POINT ( 'NONE',  ( -5.000000000000000000, -38.99999999999999289, 0.000000000000000000 ) ) ;
#32584=CARTESIAN_POINT ( 'NONE',  ( -5.000000000000000000, 15.00000000000000000, 0.000000000000000000 ) ) ;
#32587=CARTESIAN_POINT ( 'NONE',  ( -4.458734124999999437, -67.31249999863440792, 0.000000000000000000 ) ) ;
#32588=CARTESIAN_POINT ( 'NONE',  ( 3.152801135295367541, -148.5625000013655779, -3.152801135295367541 ) ) ;
#32589=CARTESIAN_POINT ( 'NONE',  ( 2.229367062499998831, -73.64583333196773651, -3.861377020970580887 ) ) ;
#32591=CARTESIAN_POINT ( 'NONE',  ( -2.229367062499996610, -25.39583333196773651, 3.861377020970582219 ) ) ;
#32592=CARTESIAN_POINT ( 'NONE',  ( -2.500000000000000444, -63.04166666393547303, -4.330127018922193649 ) ) ;
#32594=ORIENTED_EDGE ( 'NONE', *, *, #19414, .T. ) ;
#32597=FACE_OUTER_BOUND ( 'NONE', #49493, .T. ) ;
#32602=CARTESIAN_POINT ( 'NONE',  ( 9.457646018065525792E-16, -56.31249999863440081, 5.148502694627439702 ) ) ;
#32605=ORIENTED_EDGE ( 'NONE', *, *, #52399, .T. ) ;
#32606=AXIS2_PLACEMENT_3D ( 'NONE', #50737, #37452, #42895 ) ;
#32608=CARTESIAN_POINT ( 'NONE',  ( -3.152548672688508926E-16, 17.43750000136559564, -5.148502694627439702 ) ) ;
#32610=CARTESIAN_POINT ( 'NONE',  ( 2.500000000000002220, 20.45833333606451987, 4.330127018922192761 ) ) ;
#32613=EDGE_CURVE ( 'NONE', #9714, #53941, #49857, .T. ) ;
#32616=DIRECTION ( 'NONE',  ( -0.000000000000000000, 1.000000000000000000, -0.000000000000000000 ) ) ;
#32621=CARTESIAN_POINT ( 'NONE',  ( 5.000000000000000000, -161.0625000000000000, 2.071067811865478614 ) ) ;
#32623=CYLINDRICAL_SURFACE ( 'NONE', #838, 5.000000000000000000 ) ;
#32626=ORIENTED_EDGE ( 'NONE', *, *, #18460, .F. ) ;
#32627=LINE ( 'NONE', #37774, #50509 ) ;
#32629=CARTESIAN_POINT ( 'NONE',  ( -2.071067811865475061, -152.8125000027311842, -5.000000000000000888 ) ) ;
#32630=ORIENTED_EDGE ( 'NONE', *, *, #39338, .F. ) ;
#32635=CARTESIAN_POINT ( 'NONE',  ( -9.184850993605147944E-16, -145.2500000000000284, 5.000000000000000000 ) ) ;
#32638=CARTESIAN_POINT ( 'NONE',  ( 1.846868145590736310, -168.8750000013656063, 4.458734124999997661 ) ) ;
#32639=CARTESIAN_POINT ( 'NONE',  ( 2.229367062499998831, -22.64583333196773651, -3.861377020970580887 ) ) ;
#32640=CARTESIAN_POINT ( 'NONE',  ( 6.123233995736766282E-16, -170.0000000000000000, -5.000000000000000000 ) ) ;
#32642=CARTESIAN_POINT ( 'NONE',  ( -8.190561711645485556E-16, -147.6875000013656063, 4.458734124999999437 ) ) ;
#32643=ORIENTED_EDGE ( 'NONE', *, *, #41855, .T. ) ;
#32644=CARTESIAN_POINT ( 'NONE',  ( 2.071067811865644703, -149.8125000000000568, -4.999999999999831246 ) ) ;
#32645=CARTESIAN_POINT ( 'NONE',  ( -3.152548672688508926E-16, -51.81249999863440081, -5.148502694627439702 ) ) ;
#32646=AXIS2_PLACEMENT_3D ( 'NONE', #54533, #36189, #40039 ) ;
#32649=CARTESIAN_POINT ( 'NONE',  ( 5.000000000000000000, 25.50000000000000000, -6.123233995736766282E-16 ) ) ;
#32651=( BOUNDED_CURVE ( )  B_SPLINE_CURVE ( 2, ( #3561, #61788, #51503, #3255, #62424, #57285, #18342, #8073, #37964 ),
 .UNSPECIFIED., .F., .F. ) 
 B_SPLINE_CURVE_WITH_KNOTS ( ( 3, 2, 2, 2, 3 ),
 ( 0.8583333333333330595, 0.8624999999999998224, 0.8666666666666664742, 0.8708333333333332371, 0.8749999999999998890 ),
 .UNSPECIFIED. ) 
 CURVE ( )  GEOMETRIC_REPRESENTATION_ITEM ( )  RATIONAL_B_SPLINE_CURVE ( ( 1.000000000000003997, 0.9238795325112826307, 1.000000000000000000, 0.9238795325112867385, 1.000000000000000000, 0.9238795325112867385, 1.000000000000000000, 0.9238795325112887369, 0.9999999999999980016 ) ) 
 REPRESENTATION_ITEM ( '' )  );
#32653=CARTESIAN_POINT ( 'NONE',  ( -4.458734124999999437, -3.395833331967739177, -2.574251347313719407 ) ) ;
#32654=CARTESIAN_POINT ( 'NONE',  ( -6.972266317189433020E-16, -11.25000000000000178, -5.000000000000000000 ) ) ;
#32655=CARTESIAN_POINT ( 'NONE',  ( 5.000000000000000000, -141.0000000000000000, 0.000000000000000000 ) ) ;
#32657=CARTESIAN_POINT ( 'NONE',  ( 9.457646018065525792E-16, 9.687500001365593860, 5.148502694627439702 ) ) ;
#32659=CARTESIAN_POINT ( 'NONE',  ( 5.000000000000000888, -42.58333333333334281, 2.886751345948126879 ) ) ;
#32660=ORIENTED_EDGE ( 'NONE', *, *, #48267, .T. ) ;
#32661=CARTESIAN_POINT ( 'NONE',  ( 1.339745962155615144, -7.580341798530293218, 4.999999999999999112 ) ) ;
#32662=CARTESIAN_POINT ( 'NONE',  ( -2.229367062500000163, -50.47916666530107221, -3.861377020970580443 ) ) ;
#32663=CARTESIAN_POINT ( 'NONE',  ( 1.846868145590735200, -161.5000000013656063, -4.458734125000000326 ) ) ;
#32664=( BOUNDED_CURVE ( )  B_SPLINE_CURVE ( 2, ( #28533, #27903, #48152, #49660, #18877, #34872, #58120, #14052, #9231 ),
 .UNSPECIFIED., .F., .F. ) 
 B_SPLINE_CURVE_WITH_KNOTS ( ( 3, 2, 2, 2, 3 ),
 ( 0.09166666666666674346, 0.09583333333333342308, 0.1000000000000000888, 0.1041666666666667546, 0.1083333333333334203 ),
 .UNSPECIFIED. ) 
 CURVE ( )  GEOMETRIC_REPRESENTATION_ITEM ( )  RATIONAL_B_SPLINE_CURVE ( ( 0.9999999999999984457, 0.9238795325112882928, 1.000000000000000000, 0.9238795325112867385, 1.000000000000000000, 0.9238795325112867385, 1.000000000000000000, 0.9238795325112851842, 1.000000000000001554 ) ) 
 REPRESENTATION_ITEM ( '' )  );
#32665=CARTESIAN_POINT ( 'NONE',  ( -5.000000000000000000, -44.87499999726880873, 0.000000000000000000 ) ) ;
#32666=EDGE_LOOP ( 'NONE', ( #33758, #20962, #33550, #25370 ) ) ;
#32667=CARTESIAN_POINT ( 'NONE',  ( 2.229367062499998831, -21.64583333196774007, -3.861377020970580887 ) ) ;
#32668=ORIENTED_EDGE ( 'NONE', *, *, #23178, .T. ) ;
#32669=CARTESIAN_POINT ( 'NONE',  ( -3.535533905932738641, -142.5000000027311842, 3.535533905932737309 ) ) ;
#32670=CARTESIAN_POINT ( 'NONE',  ( 4.458734124999999437, -160.5000000013656347, 1.846868145590737864 ) ) ;
#32673=CARTESIAN_POINT ( 'NONE',  ( -2.229367062500000163, -38.72916666530107221, -3.861377020970580443 ) ) ;
#32674=CARTESIAN_POINT ( 'NONE',  ( -3.535533905932738641, -147.5000000027311842, 3.535533905932737309 ) ) ;
#32676=EDGE_CURVE ( 'NONE', #39148, #1448, #25128, .T. ) ;
#32677=EDGE_CURVE ( 'NONE', #1040, #6259, #14805, .T. ) ;
#32680=CARTESIAN_POINT ( 'NONE',  ( 1.975475456537005874E-15, -59.74999999999999289, 5.000000000000000000 ) ) ;
#32683=CARTESIAN_POINT ( 'NONE',  ( -6.972266317189433020E-16, -60.12499999726880873, -5.000000000000000000 ) ) ;
#32685=CARTESIAN_POINT ( 'NONE',  ( 9.457646018065525792E-16, -88.31249999863439371, 5.148502694627439702 ) ) ;
#32688=CARTESIAN_POINT ( 'NONE',  ( 2.071067811865392461, -145.3125000027312126, 5.000000000000084377 ) ) ;
#32693=ADVANCED_FACE ( 'NONE', ( #19954 ), #25748, .T. ) ;
#32695=CARTESIAN_POINT ( 'NONE',  ( -6.972266317189433020E-16, -63.12499999726880873, -5.000000000000000000 ) ) ;
#32698=CARTESIAN_POINT ( 'NONE',  ( -6.972266317189433020E-16, 16.87500000273118417, -5.000000000000000000 ) ) ;
#32700=CARTESIAN_POINT ( 'NONE',  ( -4.458734124999999437, -83.56249999863439371, 0.000000000000000000 ) ) ;
#32708=CARTESIAN_POINT ( 'NONE',  ( 3.535533905932738197, -166.0000000027312126, -3.535533905932738197 ) ) ;
#32710=CARTESIAN_POINT ( 'NONE',  ( 4.458734124999999437, 9.937500001365593860, -5.460374474430324690E-16 ) ) ;
#32711=VECTOR ( 'NONE', #49934, 1000.000000000000000 ) ;
#32716=CARTESIAN_POINT ( 'NONE',  ( 4.458734124999999437, -169.6875000013656063, 0.000000000000000000 ) ) ;
#32717=CARTESIAN_POINT ( 'NONE',  ( -4.458734124999999437, -10.31249999863440792, 0.000000000000000000 ) ) ;
#32719=ORIENTED_EDGE ( 'NONE', *, *, #32424, .F. ) ;
#32720=CARTESIAN_POINT ( 'NONE',  ( -2.229367062500000163, -33.72916666530107221, -3.861377020970580443 ) ) ;
#32724=LINE ( 'NONE', #2290, #53216 ) ;
#32727=CARTESIAN_POINT ( 'NONE',  ( 9.457646018065525792E-16, 12.93750000136559386, 5.148502694627439702 ) ) ;
#32728=LINE ( 'NONE', #18868, #31818 ) ;
#32729=CARTESIAN_POINT ( 'NONE',  ( 2.500000000000002220, -55.66666666666667140, 4.330127018922192761 ) ) ;
#32730=CARTESIAN_POINT ( 'NONE',  ( -4.458734124999997661, -81.47916666530106511, 2.574251347313722516 ) ) ;
#32733=CARTESIAN_POINT ( 'NONE',  ( -4.999999999999999112, 19.20833333606451632, 2.886751345948131764 ) ) ;
#32735=CARTESIAN_POINT ( 'NONE',  ( -9.184850993605147944E-16, -147.3750000027312126, 5.000000000000000000 ) ) ;
#32737=CARTESIAN_POINT ( 'NONE',  ( 1.162044386198238837E-16, 28.37500000273118417, 5.000000000000000000 ) ) ;
#32738=CARTESIAN_POINT ( 'NONE',  ( -5.000000000000000000, -30.08333333333333215, -2.886751345948128211 ) ) ;
#32739=CARTESIAN_POINT ( 'NONE',  ( 2.229367062500001939, -34.97916666530107221, 3.861377020970579999 ) ) ;
#32742=CARTESIAN_POINT ( 'NONE',  ( -5.000000000000000000, -29.95833333060214088, -2.886751345948128211 ) ) ;
#32743=CARTESIAN_POINT ( 'NONE',  ( 9.457646018065525792E-16, -62.06249999863440792, 5.148502694627439702 ) ) ;
#32746=CARTESIAN_POINT ( 'NONE',  ( -4.458734124999999437, -11.64583333196773829, -2.574251347313719407 ) ) ;
#32747=ORIENTED_EDGE ( 'NONE', *, *, #14147, .F. ) ;
#32749=CARTESIAN_POINT ( 'NONE',  ( 2.500000000000002220, -79.66666666666665719, 4.330127018922192761 ) ) ;
#32753=CARTESIAN_POINT ( 'NONE',  ( 1.060575238724906964E-15, -77.62499999726881583, 5.773502691896257311 ) ) ;
#32757=CARTESIAN_POINT ( 'NONE',  ( 4.458734124999998549, -21.97916666530107221, -2.574251347313721627 ) ) ;
#32758=CARTESIAN_POINT ( 'NONE',  ( -4.458734124999999437, -58.56249999863440081, 0.000000000000000000 ) ) ;
#32759=ORIENTED_EDGE ( 'NONE', *, *, #34361, .F. ) ;
#32761=CARTESIAN_POINT ( 'NONE',  ( -4.458734124999999437, -140.9375000013656063, -5.460374474430324690E-16 ) ) ;
#32764=ORIENTED_EDGE ( 'NONE', *, *, #18629, .F. ) ;
#32770=CARTESIAN_POINT ( 'NONE',  ( -1.846868145590737420, -148.0000000013655779, 4.458734124999999437 ) ) ;
#32774=CARTESIAN_POINT ( 'NONE',  ( 2.229367062499998831, -67.89583333196773651, -3.861377020970580887 ) ) ;
#32777=CYLINDRICAL_SURFACE ( 'NONE', #58309, 5.000000000000000000 ) ;
#32778=CARTESIAN_POINT ( 'NONE',  ( -4.458734124999999437, -142.9375000013656063, -5.460374474430324690E-16 ) ) ;
#32782=CARTESIAN_POINT ( 'NONE',  ( -1.339745962155610925, -49.66965819600732601, 5.000000000000000000 ) ) ;
#32783=EDGE_CURVE ( 'NONE', #33720, #57628, #49739, .T. ) ;
#32784=CARTESIAN_POINT ( 'NONE',  ( 2.499999999999998668, 16.66666666666666785, -4.330127018922193649 ) ) ;
#32790=CARTESIAN_POINT ( 'NONE',  ( -2.229367062499996610, 28.60416666803226349, 3.861377020970582219 ) ) ;
#32797=CARTESIAN_POINT ( 'NONE',  ( -4.458734124999997661, 6.770833334698928674, 2.574251347313722516 ) ) ;
#32799=CARTESIAN_POINT ( 'NONE',  ( -2.229367062500000163, -21.72916666530107221, -3.861377020970580443 ) ) ;
#32801=CARTESIAN_POINT ( 'NONE',  ( 1.846868145590735200, -158.2500000013656063, -4.458734125000000326 ) ) ;
#32806=CARTESIAN_POINT ( 'NONE',  ( -2.229367062500000163, -39.47916666530107221, -3.861377020970580443 ) ) ;
#32809=CARTESIAN_POINT ( 'NONE',  ( 2.229367062500001939, -70.22916666530107932, 3.861377020970579999 ) ) ;
#32811=CARTESIAN_POINT ( 'NONE',  ( 2.626220312808019583E-14, 14.87500000273118239, -5.000000000000000000 ) ) ;
#32812=LINE ( 'NONE', #37319, #60257 ) ;
#32815=CARTESIAN_POINT ( 'NONE',  ( 2.499999999999998668, -89.20833333060214443, -4.330127018922193649 ) ) ;
#32816=CARTESIAN_POINT ( 'NONE',  ( -3.535250795749689387E-16, -11.25000000000000355, -5.773502691896257311 ) ) ;
#32817=CARTESIAN_POINT ( 'NONE',  ( -4.458734124999999437, -15.31249999863440436, 0.000000000000000000 ) ) ;
#32818=CARTESIAN_POINT ( 'NONE',  ( -4.458734124999997661, -77.22916666530106511, 2.574251347313722516 ) ) ;
#32819=CARTESIAN_POINT ( 'NONE',  ( 5.000000000000000000, -59.37499999726880873, -6.123233995736766282E-16 ) ) ;
#32820=CARTESIAN_POINT ( 'NONE',  ( 2.499999999999998668, -12.20833333060214798, -4.330127018922193649 ) ) ;
#32821=CARTESIAN_POINT ( 'NONE',  ( 4.458734125000001214, -45.89583333196774362, 2.574251347313718519 ) ) ;
#32822=EDGE_LOOP ( 'NONE', ( #48149, #3518, #8852, #41467 ) ) ;
#32824=CARTESIAN_POINT ( 'NONE',  ( -2.229367062500000163, 9.270833334698927786, -3.861377020970580443 ) ) ;
#32826=CARTESIAN_POINT ( 'NONE',  ( 1.975475456537005874E-15, -71.62499999726878741, 5.000000000000000000 ) ) ;
#32827=CARTESIAN_POINT ( 'NONE',  ( 1.060575238724906964E-15, -62.75000000000000000, 5.773502691896257311 ) ) ;
#32828=CARTESIAN_POINT ( 'NONE',  ( -3.152801135295367985, -160.0625000013656063, 3.152801135295367096 ) ) ;
#32830=CARTESIAN_POINT ( 'NONE',  ( 1.975475456537005874E-15, -55.74999999999999289, 5.000000000000000000 ) ) ;
#32831=CARTESIAN_POINT ( 'NONE',  ( -4.458734124999999437, -78.31249999863440792, 0.000000000000000000 ) ) ;
#32832=CARTESIAN_POINT ( 'NONE',  ( -5.000000000000000888, -164.5625000000000000, -2.071067811865475949 ) ) ;
#32833=CARTESIAN_POINT ( 'NONE',  ( 1.975475456537005874E-15, -11.74999999999999645, 5.000000000000000000 ) ) ;
#32835=CARTESIAN_POINT ( 'NONE',  ( -2.229367062499996610, -5.395833331967740953, 3.861377020970582219 ) ) ;
#32836=CARTESIAN_POINT ( 'NONE',  ( -4.458734124999999437, -43.56249999863440081, 0.000000000000000000 ) ) ;
#32843=DIRECTION ( 'NONE',  ( 0.000000000000000000, 0.000000000000000000, 1.000000000000000000 ) ) ;
#32844=CARTESIAN_POINT ( 'NONE',  ( 4.458734125000001214, -69.14583333196773651, 2.574251347313718519 ) ) ;
#32845=CARTESIAN_POINT ( 'NONE',  ( -3.152801135295367985, -145.0625000013655779, 3.152801135295367096 ) ) ;
#32847=CARTESIAN_POINT ( 'NONE',  ( -5.000000000000000888, -150.5625000027311842, 2.071067811865474617 ) ) ;
#32852=CARTESIAN_POINT ( 'NONE',  ( -2.229367062499996610, 0.8541666680322613781, 3.861377020970582219 ) ) ;
#32853=CARTESIAN_POINT ( 'NONE',  ( 5.000000000000000000, -30.29166666393547658, -2.886751345948130876 ) ) ;
#32854=CARTESIAN_POINT ( 'NONE',  ( 4.458734124999997661, -157.5000000013656063, 1.846868145590737864 ) ) ;
#32863=FACE_OUTER_BOUND ( 'NONE', #4447, .T. ) ;
#32868=CARTESIAN_POINT ( 'NONE',  ( -3.152548672688508926E-16, 20.43750000136559208, -5.148502694627439702 ) ) ;
#32870=CARTESIAN_POINT ( 'NONE',  ( 2.229367062500001939, -5.229166665301071326, 3.861377020970579999 ) ) ;
#32871=CARTESIAN_POINT ( 'NONE',  ( 1.975475456537005874E-15, -33.62499999726880873, 5.000000000000000000 ) ) ;
#32873=CARTESIAN_POINT ( 'NONE',  ( -5.000000000000000888, -142.5625000027312694, 2.071067811865474617 ) ) ;
#32875=AXIS2_PLACEMENT_3D ( 'NONE', #2303, #20643, #30265 ) ;
#32882=CARTESIAN_POINT ( 'NONE',  ( -8.190561711645485556E-16, -157.9375000013655779, 4.458734124999999437 ) ) ;
#32886=CARTESIAN_POINT ( 'NONE',  ( -3.152548672688508926E-16, 17.18750000136559919, -5.148502694627439702 ) ) ;
#32892=CARTESIAN_POINT ( 'NONE',  ( -3.535250795749689387E-16, 1.750000000000001554, -5.773502691896257311 ) ) ;
#32894=AXIS2_PLACEMENT_3D ( 'NONE', #9969, #48886, #63073 ) ;
#32895=CARTESIAN_POINT ( 'NONE',  ( -4.458734124999999437, -60.31249999863440081, 0.000000000000000000 ) ) ;
#32896=CYLINDRICAL_SURFACE ( 'NONE', #61635, 5.000000000000000000 ) ;
#32898=CARTESIAN_POINT ( 'NONE',  ( -2.229367062500000163, -30.47916666530107221, -3.861377020970580443 ) ) ;
#32899=CARTESIAN_POINT ( 'NONE',  ( -1.339745962155610925, -37.66965819600733312, 5.000000000000000000 ) ) ;
#32900=CARTESIAN_POINT ( 'NONE',  ( -2.500000000000000444, 25.95833333606451632, -4.330127018922193649 ) ) ;
#32901=( BOUNDED_CURVE ( )  B_SPLINE_CURVE ( 2, ( #32830, #18349, #53386, #18966, #14456, #9010, #47921, #43722, #19283 ),
 .UNSPECIFIED., .F., .F. ) 
 B_SPLINE_CURVE_WITH_KNOTS ( ( 3, 2, 2, 2, 3 ),
 ( 0.7145833333333333481, 0.7152777777777777901, 0.7166666666666666741, 0.7180555555555555580, 0.7187500000000000000 ),
 .UNSPECIFIED. ) 
 CURVE ( )  GEOMETRIC_REPRESENTATION_ITEM ( )  RATIONAL_B_SPLINE_CURVE ( ( 0.9330127018922194093, 0.9330127018922194093, 1.000000000000000000, 0.8660254037844387076, 1.000000000000000000, 0.8660254037844387076, 1.000000000000000000, 0.9330127018922194093, 0.9330127018922194093 ) ) 
 REPRESENTATION_ITEM ( '' )  );
#32903=CARTESIAN_POINT ( 'NONE',  ( -4.999999999999999112, -39.91666666666667140, 2.886751345948131764 ) ) ;
#32904=CARTESIAN_POINT ( 'NONE',  ( 0.000000000000000000, -170.0000000000000000, 5.000000000000000000 ) ) ;
#32909=CARTESIAN_POINT ( 'NONE',  ( 4.458734124999999437, -62.81249999863440792, -5.460374474430324690E-16 ) ) ;
#32910=CARTESIAN_POINT ( 'NONE',  ( -1.846868145590737420, -149.0000000013656063, 4.458734124999999437 ) ) ;
#32911=CARTESIAN_POINT ( 'NONE',  ( 4.458734124999999437, -74.81249999863440792, -5.460374474430324690E-16 ) ) ;
#32913=CARTESIAN_POINT ( 'NONE',  ( 2.229367062499998831, -26.89583333196774007, -3.861377020970580887 ) ) ;
#32914=CARTESIAN_POINT ( 'NONE',  ( 2.500000000000002220, -64.54166666393547303, 4.330127018922192761 ) ) ;
#32915=ORIENTED_EDGE ( 'NONE', *, *, #55941, .T. ) ;
#32917=VERTEX_POINT ( 'NONE', #54587 ) ;
#32920=ORIENTED_EDGE ( 'NONE', *, *, #34552, .T. ) ;
#32921=LINE ( 'NONE', #14782, #5653 ) ;
#32922=CARTESIAN_POINT ( 'NONE',  ( -4.999999999999998224, -77.79166666393547303, 2.886751345948131764 ) ) ;
#32924=CARTESIAN_POINT ( 'NONE',  ( -3.152548672688508926E-16, -54.81249999863440081, -5.148502694627439702 ) ) ;
#32926=EDGE_LOOP ( 'NONE', ( #52451, #52600, #20164, #24733 ) ) ;
#32929=CARTESIAN_POINT ( 'NONE',  ( 2.229367062500001939, 18.02083333469892779, 3.861377020970579999 ) ) ;
#32932=CARTESIAN_POINT ( 'NONE',  ( 3.152801135295367541, -168.3125000013656063, -3.152801135295367541 ) ) ;
#32937=FACE_OUTER_BOUND ( 'NONE', #37793, .T. ) ;
#32940=DIRECTION ( 'NONE',  ( 0.000000000000000000, -1.000000000000000000, 0.000000000000000000 ) ) ;
#32947=CARTESIAN_POINT ( 'NONE',  ( 0.000000000000000000, -170.0000000000000000, 5.000000000000000000 ) ) ;
#32949=CARTESIAN_POINT ( 'NONE',  ( -9.184850993605147944E-16, -152.3750000027311842, 5.000000000000000000 ) ) ;
#32950=ORIENTED_EDGE ( 'NONE', *, *, #31015, .T. ) ;
#32955=CARTESIAN_POINT ( 'NONE',  ( 5.000000000000000888, -148.9375000000000000, -2.071067811865475505 ) ) ;
#32958=CARTESIAN_POINT ( 'NONE',  ( 2.730187237215162345E-16, -169.4375000013656063, -4.458734124999999437 ) ) ;
#32959=CARTESIAN_POINT ( 'NONE',  ( -3.152548672688508926E-16, -30.56249999863440436, -5.148502694627439702 ) ) ;
#32963=CARTESIAN_POINT ( 'NONE',  ( -3.152801135295367096, -147.0625000013655779, -3.152801135295367541 ) ) ;
#32966=CARTESIAN_POINT ( 'NONE',  ( 5.000000000000000000, -150.0625000000000284, 2.071067811865478614 ) ) ;
#32967=CARTESIAN_POINT ( 'NONE',  ( -4.458734124999997661, -54.47916666530107932, 2.574251347313722516 ) ) ;
#32970=CARTESIAN_POINT ( 'NONE',  ( 2.499999999999998668, 17.66666666666666430, -4.330127018922193649 ) ) ;
#32971=AXIS2_PLACEMENT_3D ( 'NONE', #47294, #22223, #46023 ) ;
#32973=CARTESIAN_POINT ( 'NONE',  ( -4.999999999999998224, -88.91666666666667140, 2.886751345948131764 ) ) ;
#32974=CARTESIAN_POINT ( 'NONE',  ( -4.458734124999999437, 1.687500001365593194, 0.000000000000000000 ) ) ;
#32975=DIRECTION ( 'NONE',  ( -0.000000000000000000, 1.000000000000000000, -0.000000000000000000 ) ) ;
#32976=CARTESIAN_POINT ( 'NONE',  ( -3.535533905932738641, -164.3750000000000284, 3.535533905932737309 ) ) ;
#32977=CARTESIAN_POINT ( 'NONE',  ( -4.458734124999998549, 9.520833334698927786, 2.574251347313722516 ) ) ;
#32981=CARTESIAN_POINT ( 'NONE',  ( 1.339745962155612702, -7.169658196007335782, -5.000000000000000000 ) ) ;
#32982=CARTESIAN_POINT ( 'NONE',  ( 4.458734124999998549, -49.72916666530106511, -2.574251347313721627 ) ) ;
#32983=CARTESIAN_POINT ( 'NONE',  ( -3.152801135295367985, -161.0625000013656063, 3.152801135295367096 ) ) ;
#32984=EDGE_CURVE ( 'NONE', #44449, #41004, #51824, .T. ) ;
#32985=CARTESIAN_POINT ( 'NONE',  ( 5.000000000000000000, -49.29166666393547303, -2.886751345948129988 ) ) ;
#32987=CARTESIAN_POINT ( 'NONE',  ( 4.458734124999999437, -21.81249999863440436, -5.460374474430324690E-16 ) ) ;
#32992=CARTESIAN_POINT ( 'NONE',  ( 4.458734125000000326, -161.3750000013656063, -1.846868145590734978 ) ) ;
#32993=CYLINDRICAL_SURFACE ( 'NONE', #3647, 5.000000000000000000 ) ;
#32995=CARTESIAN_POINT ( 'NONE',  ( 4.458734124999999437, -36.06249999863440792, -5.460374474430324690E-16 ) ) ;
#33000=CARTESIAN_POINT ( 'NONE',  ( 0.000000000000000000, -170.0000000000000000, 0.000000000000000000 ) ) ;
#33003=CARTESIAN_POINT ( 'NONE',  ( 2.229367062500001939, -83.22916666530106511, 3.861377020970579999 ) ) ;
#33006=CARTESIAN_POINT ( 'NONE',  ( -8.190561711645485556E-16, -139.9375000013656063, 4.458734124999999437 ) ) ;
#33010=VECTOR ( 'NONE', #41698, 1000.000000000000000 ) ;
#33013=CARTESIAN_POINT ( 'NONE',  ( -5.000000000000000000, -82.08333333333332860, -2.886751345948128211 ) ) ;
#33015=EDGE_CURVE ( 'NONE', #43823, #53443, #3361, .T. ) ;
#33017=DIRECTION ( 'NONE',  ( 0.000000000000000000, 0.000000000000000000, 1.000000000000000000 ) ) ;
#33019=CARTESIAN_POINT ( 'NONE',  ( -4.458734124999999437, -82.64583333196772230, -2.574251347313719407 ) ) ;
#33022=ORIENTED_EDGE ( 'NONE', *, *, #32783, .F. ) ;
#33023=CARTESIAN_POINT ( 'NONE',  ( -5.000000000000000000, -16.95833333060214443, -2.886751345948128211 ) ) ;
#33025=CARTESIAN_POINT ( 'NONE',  ( 2.071067811865476394, -167.3125000027312126, 5.000000000000000000 ) ) ;
#33028=CARTESIAN_POINT ( 'NONE',  ( -1.339745962155610925, -29.79465819873851729, 5.000000000000000000 ) ) ;
#33029=( BOUNDED_CURVE ( )  B_SPLINE_CURVE ( 2, ( #54192, #29099, #38755, #495, #10445, #49369, #20099, #30060, #49687 ),
 .UNSPECIFIED., .F., .F. ) 
 B_SPLINE_CURVE_WITH_KNOTS ( ( 3, 2, 2, 2, 3 ),
 ( 0.04791666666666666990, 0.04861111111111111188, 0.05000000000000000278, 0.05138888888888888673, 0.05208333333333333565 ),
 .UNSPECIFIED. ) 
 CURVE ( )  GEOMETRIC_REPRESENTATION_ITEM ( )  RATIONAL_B_SPLINE_CURVE ( ( 0.9330127018922192983, 0.9330127018922196314, 1.000000000000000000, 0.8660254037844387076, 1.000000000000000000, 0.8660254037844387076, 1.000000000000000000, 0.9330127018922189652, 0.9330127018922192983 ) ) 
 REPRESENTATION_ITEM ( '' )  );
#33034=CARTESIAN_POINT ( 'NONE',  ( 2.500000000000002220, -86.54166666393547303, 4.330127018922192761 ) ) ;
#33035=CARTESIAN_POINT ( 'NONE',  ( -5.000000000000000000, -152.5000000000000284, -6.123233995736766282E-16 ) ) ;
#33036=CARTESIAN_POINT ( 'NONE',  ( -4.458734124999999437, -11.39583333196774007, -2.574251347313719407 ) ) ;
#33038=VERTEX_POINT ( 'NONE', #29803 ) ;
#33039=CARTESIAN_POINT ( 'NONE',  ( 4.458734124999999437, -39.06249999863440081, -5.460374474430324690E-16 ) ) ;
#33047=CARTESIAN_POINT ( 'NONE',  ( 9.457646018065525792E-16, 16.93750000136559564, 5.148502694627439702 ) ) ;
#33048=EDGE_CURVE ( 'NONE', #28941, #36379, #1313, .T. ) ;
#33050=FACE_OUTER_BOUND ( 'NONE', #10368, .T. ) ;
#33052=CARTESIAN_POINT ( 'NONE',  ( 2.229367062499998831, -83.89583333196773651, -3.861377020970580887 ) ) ;
#33054=CARTESIAN_POINT ( 'NONE',  ( -4.999999999999999112, 16.20833333606451987, 2.886751345948131764 ) ) ;
#33055=ORIENTED_EDGE ( 'NONE', *, *, #42218, .F. ) ;
#33059=CARTESIAN_POINT ( 'NONE',  ( 5.000000000000000888, -31.58333333333333215, 2.886751345948126879 ) ) ;
#33060=CARTESIAN_POINT ( 'NONE',  ( 9.457646018065525792E-16, -35.06249999863440792, 5.148502694627439702 ) ) ;
#33063=CARTESIAN_POINT ( 'NONE',  ( 5.000000000000000888, -30.45833333060214443, 2.886751345948126879 ) ) ;
#33064=CARTESIAN_POINT ( 'NONE',  ( 4.458734125000001214, -60.89583333196774362, 2.574251347313718519 ) ) ;
#33065=EDGE_LOOP ( 'NONE', ( #32594, #30867, #52573, #30802 ) ) ;
#33068=CARTESIAN_POINT ( 'NONE',  ( -4.458734124999999437, -6.645833331967741842, -2.574251347313719407 ) ) ;
#33070=CARTESIAN_POINT ( 'NONE',  ( 1.060575238724906964E-15, -76.74999999999998579, 5.773502691896257311 ) ) ;
#33071=CARTESIAN_POINT ( 'NONE',  ( 1.162044386198238837E-16, 28.37500000273118417, 5.000000000000000000 ) ) ;
#33073=CARTESIAN_POINT ( 'NONE',  ( -4.999999999999999112, -75.79166666393545881, 2.886751345948131764 ) ) ;
#33074=DIRECTION ( 'NONE',  ( -0.000000000000000000, 1.000000000000000000, -0.000000000000000000 ) ) ;
#33077=CARTESIAN_POINT ( 'NONE',  ( 2.229367062499998831, -21.89583333196774007, -3.861377020970580887 ) ) ;
#33078=CARTESIAN_POINT ( 'NONE',  ( -4.458734124999999437, -54.64583333196774362, -2.574251347313719407 ) ) ;
#33079=VERTEX_POINT ( 'NONE', #37196 ) ;
#33080=CARTESIAN_POINT ( 'NONE',  ( 4.458734124999999437, -167.7500000013655779, 1.846868145590737864 ) ) ;
#33082=CARTESIAN_POINT ( 'NONE',  ( 1.975475456537005874E-15, -8.624999997268812280, 5.000000000000000000 ) ) ;
#33089=CARTESIAN_POINT ( 'NONE',  ( 3.152801135295366208, -144.8125000013655779, 3.152801135295367985 ) ) ;
#33091=DIRECTION ( 'NONE',  ( 0.000000000000000000, 0.000000000000000000, 1.000000000000000000 ) ) ;
#33093=CARTESIAN_POINT ( 'NONE',  ( 4.458734124999998549, -69.97916666530107932, -2.574251347313721627 ) ) ;
#33096=CARTESIAN_POINT ( 'NONE',  ( -6.972266317189433020E-16, -68.24999999999998579, -5.000000000000000000 ) ) ;
#33098=( BOUNDED_CURVE ( )  B_SPLINE_CURVE ( 2, ( #21383, #40026, #30380, #41300, #36178, #40669, #11716, #31333, #31020 ),
 .UNSPECIFIED., .F., .F. ) 
 B_SPLINE_CURVE_WITH_KNOTS ( ( 3, 2, 2, 2, 3 ),
 ( 0.7520833333333333259, 0.7527777777777777679, 0.7541666666666666519, 0.7555555555555555358, 0.7562499999999999778 ),
 .UNSPECIFIED. ) 
 CURVE ( )  GEOMETRIC_REPRESENTATION_ITEM ( )  RATIONAL_B_SPLINE_CURVE ( ( 0.9330127018922194093, 0.9330127018922194093, 1.000000000000000000, 0.8660254037844387076, 1.000000000000000000, 0.8660254037844387076, 1.000000000000000000, 0.9330127018922194093, 0.9330127018922194093 ) ) 
 REPRESENTATION_ITEM ( '' )  );
#33099=ORIENTED_EDGE ( 'NONE', *, *, #36121, .F. ) ;
#33101=CARTESIAN_POINT ( 'NONE',  ( 5.000000000000000000, -160.0625000000000568, 2.071067811865478614 ) ) ;
#33106=CARTESIAN_POINT ( 'NONE',  ( 2.229367062499998831, 23.10416666803225993, -3.861377020970580887 ) ) ;
#33107=CARTESIAN_POINT ( 'NONE',  ( 0.000000000000000000, -170.0000000000000000, 0.000000000000000000 ) ) ;
#33112=CARTESIAN_POINT ( 'NONE',  ( 1.339745962155612702, -43.16965819600731891, -5.000000000000000000 ) ) ;
#33113=CARTESIAN_POINT ( 'NONE',  ( -4.458734124999999437, 4.604166668032261711, -2.574251347313719407 ) ) ;
#33115=CARTESIAN_POINT ( 'NONE',  ( 4.458734124999999437, -17.06249999863440792, -5.460374474430324690E-16 ) ) ;
#33117=CARTESIAN_POINT ( 'NONE',  ( 3.152801135295366208, -157.5625000013656063, 3.152801135295367985 ) ) ;
#33118=FACE_OUTER_BOUND ( 'NONE', #35878, .T. ) ;
#33122=CARTESIAN_POINT ( 'NONE',  ( 9.457646018065525792E-16, 28.93750000136559564, 5.148502694627439702 ) ) ;
#33123=CARTESIAN_POINT ( 'NONE',  ( 9.457646018065525792E-16, -41.06249999863440081, 5.148502694627439702 ) ) ;
#33127=CARTESIAN_POINT ( 'NONE',  ( -4.458734124999999437, -67.64583333196773651, -2.574251347313719407 ) ) ;
#33130=CARTESIAN_POINT ( 'NONE',  ( 2.500000000000002220, 28.45833333606451987, 4.330127018922192761 ) ) ;
#33131=ORIENTED_EDGE ( 'NONE', *, *, #54313, .T. ) ;
#33133=( BOUNDED_CURVE ( )  B_SPLINE_CURVE ( 2, ( #25690, #40786, #60433, #35979, #55608, #11524, #50766, #6709, #7666 ),
 .UNSPECIFIED., .F., .F. ) 
 B_SPLINE_CURVE_WITH_KNOTS ( ( 3, 2, 2, 2, 3 ),
 ( 0.4854166666666666630, 0.4861111111111111049, 0.4874999999999999889, 0.4888888888888888729, 0.4895833333333333148 ),
 .UNSPECIFIED. ) 
 CURVE ( )  GEOMETRIC_REPRESENTATION_ITEM ( )  RATIONAL_B_SPLINE_CURVE ( ( 0.9330127018922194093, 0.9330127018922194093, 1.000000000000000000, 0.8660254037844387076, 1.000000000000000000, 0.8660254037844387076, 1.000000000000000000, 0.9330127018922194093, 0.9330127018922194093 ) ) 
 REPRESENTATION_ITEM ( '' )  );
#33134=ADVANCED_FACE ( 'NONE', ( #22406 ), #36237, .T. ) ;
#33135=CARTESIAN_POINT ( 'NONE',  ( -6.972266317189433020E-16, -87.12499999726880162, -5.000000000000000000 ) ) ;
#33136=CARTESIAN_POINT ( 'NONE',  ( 2.499999999999998668, -15.33333333333333037, -4.330127018922193649 ) ) ;
#33137=CARTESIAN_POINT ( 'NONE',  ( 4.458734124999998549, -15.72916666530107399, -2.574251347313721627 ) ) ;
#33138=EDGE_CURVE ( 'NONE', #14909, #26438, #34505, .T. ) ;
#33139=CARTESIAN_POINT ( 'NONE',  ( -2.229367062499996610, -78.14583333196773651, 3.861377020970582219 ) ) ;
#33141=CARTESIAN_POINT ( 'NONE',  ( -5.000000000000000000, -12.95833333060214976, -2.886751345948128211 ) ) ;
#33142=CARTESIAN_POINT ( 'NONE',  ( 2.229367062500001939, -45.97916666530106511, 3.861377020970579999 ) ) ;
#33144=CARTESIAN_POINT ( 'NONE',  ( 2.500000000000002220, -41.66666666666667140, 4.330127018922192761 ) ) ;
#33145=CARTESIAN_POINT ( 'NONE',  ( -4.458734124999999437, 7.437500001365594748, 0.000000000000000000 ) ) ;
#33148=CARTESIAN_POINT ( 'NONE',  ( -2.500000000000000444, -59.16666666666665719, -4.330127018922193649 ) ) ;
#33149=EDGE_CURVE ( 'NONE', #47469, #27835, #51452, .T. ) ;
#33150=CARTESIAN_POINT ( 'NONE',  ( -4.458734125000001214, -157.1250000013656063, 1.846868145590734089 ) ) ;
#33152=CARTESIAN_POINT ( 'NONE',  ( -6.972266317189433020E-16, -14.24999999999999822, -5.000000000000000000 ) ) ;
#33153=CARTESIAN_POINT ( 'NONE',  ( -5.000000000000000000, -167.5000000000000000, -6.123233995736766282E-16 ) ) ;
#33154=ADVANCED_FACE ( 'NONE', ( #56821 ), #6978, .T. ) ;
#33156=CARTESIAN_POINT ( 'NONE',  ( 9.457646018065525792E-16, -3.312499998634407472, 5.148502694627439702 ) ) ;
#33157=CARTESIAN_POINT ( 'NONE',  ( 4.458734124999999437, -40.06249999863440081, -5.460374474430324690E-16 ) ) ;
#33158=EDGE_CURVE ( 'NONE', #58699, #47465, #9909, .T. ) ;
#33160=CARTESIAN_POINT ( 'NONE',  ( -8.190561711645485556E-16, -150.6875000013656063, 4.458734124999999437 ) ) ;
#33163=EDGE_LOOP ( 'NONE', ( #43877, #40977, #17956, #54852 ) ) ;
#33166=CARTESIAN_POINT ( 'NONE',  ( -3.152548672688508926E-16, -69.81249999863439371, -5.148502694627439702 ) ) ;
#33167=CARTESIAN_POINT ( 'NONE',  ( 4.458734124999999437, -146.6250000013655779, -1.846868145590734978 ) ) ;
#33171=CARTESIAN_POINT ( 'NONE',  ( -9.184850993605147944E-16, -141.2500000000000284, 5.000000000000000000 ) ) ;
#33172=CARTESIAN_POINT ( 'NONE',  ( -4.458734124999999437, 2.687500001365593860, 0.000000000000000000 ) ) ;
#33173=CARTESIAN_POINT ( 'NONE',  ( 1.846868145590736310, -151.6250000013655779, 4.458734124999997661 ) ) ;
#33175=ORIENTED_EDGE ( 'NONE', *, *, #42212, .F. ) ;
#33182=DIRECTION ( 'NONE',  ( -0.000000000000000000, 1.000000000000000000, -0.000000000000000000 ) ) ;
#33186=CARTESIAN_POINT ( 'NONE',  ( -6.972266317189433020E-16, -44.25000000000000000, -5.000000000000000000 ) ) ;
#33187=CARTESIAN_POINT ( 'NONE',  ( -3.152548672688508926E-16, 22.43750000136559564, -5.148502694627439702 ) ) ;
#33189=CARTESIAN_POINT ( 'NONE',  ( -4.458734124999999437, -5.562499998634402587, 0.000000000000000000 ) ) ;
#33190=CARTESIAN_POINT ( 'NONE',  ( -6.972266317189433020E-16, -83.24999999999998579, -5.000000000000000000 ) ) ;
#33192=CARTESIAN_POINT ( 'NONE',  ( -3.535533905932737309, -142.7500000027311842, -3.535533905932738197 ) ) ;
#33193=CARTESIAN_POINT ( 'NONE',  ( 5.000000000000000888, -75.45833333060214443, 2.886751345948126879 ) ) ;
#33200=CARTESIAN_POINT ( 'NONE',  ( 1.846868145590735200, -158.5000000013656347, -4.458734124999999437 ) ) ;
#33204=CARTESIAN_POINT ( 'NONE',  ( -4.458734124999999437, 18.35416666803225993, -2.574251347313719407 ) ) ;
#33209=CARTESIAN_POINT ( 'NONE',  ( 5.000000000000000888, 5.416666666666666963, 2.886751345948126879 ) ) ;
#33210=( BOUNDED_CURVE ( )  B_SPLINE_CURVE ( 2, ( #14960, #25252, #49376, #10451, #5321, #15610, #502, #20109, #35228 ),
 .UNSPECIFIED., .F., .F. ) 
 B_SPLINE_CURVE_WITH_KNOTS ( ( 3, 2, 2, 2, 3 ),
 ( 0.2062499999999999889, 0.2069444444444444309, 0.2083333333333333426, 0.2097222222222222265, 0.2104166666666666685 ),
 .UNSPECIFIED. ) 
 CURVE ( )  GEOMETRIC_REPRESENTATION_ITEM ( )  RATIONAL_B_SPLINE_CURVE ( ( 0.9330127018922194093, 0.9330127018922194093, 1.000000000000000000, 0.8660254037844387076, 1.000000000000000000, 0.8660254037844387076, 1.000000000000000000, 0.9330127018922194093, 0.9330127018922194093 ) ) 
 REPRESENTATION_ITEM ( '' )  );
#33211=CARTESIAN_POINT ( 'NONE',  ( 2.229367062499998831, -60.64583333196774362, -3.861377020970580887 ) ) ;
#33213=CARTESIAN_POINT ( 'NONE',  ( -3.535250795749689387E-16, 2.875000002731185944, -5.773502691896257311 ) ) ;
#33214=CARTESIAN_POINT ( 'NONE',  ( -3.152548672688508926E-16, -28.56249999863440436, -5.148502694627439702 ) ) ;
#33215=CARTESIAN_POINT ( 'NONE',  ( -5.000000000000000000, -41.99999999999999289, 0.000000000000000000 ) ) ;
#33216=CYLINDRICAL_SURFACE ( 'NONE', #475, 5.000000000000000000 ) ;
#33218=CARTESIAN_POINT ( 'NONE',  ( 5.000000000000000888, -42.58333333333334281, 2.886751345948126879 ) ) ;
#33219=CARTESIAN_POINT ( 'NONE',  ( 5.000000000000000888, -26.45833333060214798, 2.886751345948126879 ) ) ;
#33221=CARTESIAN_POINT ( 'NONE',  ( -4.458734124999999437, -66.31249999863440792, 0.000000000000000000 ) ) ;
#33222=CARTESIAN_POINT ( 'NONE',  ( 3.152801135295366208, -147.8125000013655779, 3.152801135295367985 ) ) ;
#33223=CARTESIAN_POINT ( 'NONE',  ( -4.458734124999999437, -76.31249999863440792, 0.000000000000000000 ) ) ;
#33225=CARTESIAN_POINT ( 'NONE',  ( 9.457646018065525792E-16, -25.31249999863440792, 5.148502694627439702 ) ) ;
#33226=( BOUNDED_CURVE ( )  B_SPLINE_CURVE ( 2, ( #21957, #36752, #56382, #7484, #31603, #46713, #2985, #31921, #60258 ),
 .UNSPECIFIED., .F., .F. ) 
 B_SPLINE_CURVE_WITH_KNOTS ( ( 3, 2, 2, 2, 3 ),
 ( 0.2437499999999999944, 0.2444444444444444364, 0.2458333333333333204, 0.2472222222222222321, 0.2479166666666666741 ),
 .UNSPECIFIED. ) 
 CURVE ( )  GEOMETRIC_REPRESENTATION_ITEM ( )  RATIONAL_B_SPLINE_CURVE ( ( 0.9330127018922194093, 0.9330127018922194093, 1.000000000000000000, 0.8660254037844387076, 1.000000000000000000, 0.8660254037844387076, 1.000000000000000000, 0.9330127018922194093, 0.9330127018922194093 ) ) 
 REPRESENTATION_ITEM ( '' )  );
#33227=CARTESIAN_POINT ( 'NONE',  ( 2.499999999999998668, -66.20833333060213022, -4.330127018922193649 ) ) ;
#33229=CARTESIAN_POINT ( 'NONE',  ( 1.975475456537005874E-15, -21.75000000000000000, 5.000000000000000000 ) ) ;
#33234=EDGE_LOOP ( 'NONE', ( #54252, #23438, #48262, #31711 ) ) ;
#33235=FACE_OUTER_BOUND ( 'NONE', #20315, .T. ) ;
#33236=CARTESIAN_POINT ( 'NONE',  ( 9.457646018065525792E-16, -51.31249999863440792, 5.148502694627439702 ) ) ;
#33241=CARTESIAN_POINT ( 'NONE',  ( -3.152548672688508926E-16, 18.43750000136559564, -5.148502694627439702 ) ) ;
#33243=CARTESIAN_POINT ( 'NONE',  ( 5.000000000000000000, 20.70833333606451987, -2.886751345948130876 ) ) ;
#33244=CARTESIAN_POINT ( 'NONE',  ( -8.190561711645485556E-16, -164.6875000013655779, 4.458734124999999437 ) ) ;
#33247=CARTESIAN_POINT ( 'NONE',  ( -2.499999999999996447, -39.83333333333332860, 4.330127018922195425 ) ) ;
#33249=VECTOR ( 'NONE', #38990, 1000.000000000000000 ) ;
#33250=CARTESIAN_POINT ( 'NONE',  ( 0.000000000000000000, -170.0000000000000000, 0.000000000000000000 ) ) ;
#33255=CARTESIAN_POINT ( 'NONE',  ( 0.000000000000000000, -170.0000000000000000, 0.000000000000000000 ) ) ;
#33261=LINE ( 'NONE', #32947, #1069 ) ;
#33263=CARTESIAN_POINT ( 'NONE',  ( -2.071067811865475061, -151.8125000027311842, -5.000000000000000888 ) ) ;
#33269=CARTESIAN_POINT ( 'NONE',  ( 3.535533905932736864, -141.1250000000000000, 3.535533905932738641 ) ) ;
#33272=CARTESIAN_POINT ( 'NONE',  ( -6.972266317189433020E-16, -55.24999999999999289, -5.000000000000000000 ) ) ;
#33273=CARTESIAN_POINT ( 'NONE',  ( -2.229367062499996610, -29.14583333196774007, 3.861377020970582219 ) ) ;
#33277=CARTESIAN_POINT ( 'NONE',  ( 2.730187237215162345E-16, -147.1875000013656063, -4.458734124999999437 ) ) ;
#33279=CARTESIAN_POINT ( 'NONE',  ( -2.229367062500000163, -54.72916666530107221, -3.861377020970580443 ) ) ;
#33283=CARTESIAN_POINT ( 'NONE',  ( 5.000000000000000000, 19.50000000000000000, -6.123233995736766282E-16 ) ) ;
#33284=CARTESIAN_POINT ( 'NONE',  ( -6.972266317189433020E-16, -89.24999999999998579, -5.000000000000000000 ) ) ;
#33285=CARTESIAN_POINT ( 'NONE',  ( 4.458734124999999437, -1.812499998634406584, -5.460374474430324690E-16 ) ) ;
#33286=CARTESIAN_POINT ( 'NONE',  ( -2.071067811865644259, -154.6875000000000000, -4.999999999999831246 ) ) ;
#33288=CARTESIAN_POINT ( 'NONE',  ( -3.152548672688508926E-16, 8.187500001365595637, -5.148502694627439702 ) ) ;
#33290=CARTESIAN_POINT ( 'NONE',  ( 0.000000000000000000, 30.00000000000000000, 0.000000000000000000 ) ) ;
#33291=CARTESIAN_POINT ( 'NONE',  ( 9.457646018065525792E-16, -49.06249999863440792, 5.148502694627439702 ) ) ;
#33292=CARTESIAN_POINT ( 'NONE',  ( -4.458734125000000326, -160.2500000013656063, -1.846868145590735644 ) ) ;
#33294=CARTESIAN_POINT ( 'NONE',  ( 2.499999999999998668, -52.20833333060213732, -4.330127018922193649 ) ) ;
#33296=CARTESIAN_POINT ( 'NONE',  ( -2.229367062499996610, -23.14583333196773651, 3.861377020970582219 ) ) ;
#33297=VERTEX_POINT ( 'NONE', #10040 ) ;
#33298=DIRECTION ( 'NONE',  ( -0.000000000000000000, 1.000000000000000000, -0.000000000000000000 ) ) ;
#33300=CARTESIAN_POINT ( 'NONE',  ( -3.152801135295367096, -160.0625000013656063, -3.152801135295367541 ) ) ;
#33301=ORIENTED_EDGE ( 'NONE', *, *, #35011, .T. ) ;
#33304=CARTESIAN_POINT ( 'NONE',  ( -2.229367062499996610, -39.39583333196773651, 3.861377020970582219 ) ) ;
#33305=ORIENTED_EDGE ( 'NONE', *, *, #44784, .T. ) ;
#33308=DIRECTION ( 'NONE',  ( 0.000000000000000000, 0.000000000000000000, 1.000000000000000000 ) ) ;
#33309=ORIENTED_EDGE ( 'NONE', *, *, #45607, .F. ) ;
#33311=CARTESIAN_POINT ( 'NONE',  ( 4.458734124999999437, -84.06249999863439371, -5.460374474430324690E-16 ) ) ;
#33314=CARTESIAN_POINT ( 'NONE',  ( 2.500000000000002220, -9.666666666666664298, 4.330127018922192761 ) ) ;
#33315=( BOUNDED_CURVE ( )  B_SPLINE_CURVE ( 2, ( #42930, #43547, #53529, #9457, #28452, #63191, #58360, #52593, #14286 ),
 .UNSPECIFIED., .F., .F. ) 
 B_SPLINE_CURVE_WITH_KNOTS ( ( 3, 2, 2, 2, 3 ),
 ( 0.5479166666666667185, 0.5486111111111111605, 0.5500000000000000444, 0.5513888888888889284, 0.5520833333333333703 ),
 .UNSPECIFIED. ) 
 CURVE ( )  GEOMETRIC_REPRESENTATION_ITEM ( )  RATIONAL_B_SPLINE_CURVE ( ( 0.9330127018922194093, 0.9330127018922194093, 1.000000000000000000, 0.8660254037844387076, 1.000000000000000000, 0.8660254037844387076, 1.000000000000000000, 0.9330127018922194093, 0.9330127018922194093 ) ) 
 REPRESENTATION_ITEM ( '' )  );
#33316=CARTESIAN_POINT ( 'NONE',  ( 5.000000000000000000, -145.1250000027312126, 0.000000000000000000 ) ) ;
#33326=CARTESIAN_POINT ( 'NONE',  ( -5.000000000000000000, -61.00000000000000000, 0.000000000000000000 ) ) ;
#33327=CARTESIAN_POINT ( 'NONE',  ( 9.457646018065525792E-16, -82.31249999863440792, 5.148502694627439702 ) ) ;
#33331=CARTESIAN_POINT ( 'NONE',  ( -9.184850993605147944E-16, -155.3750000027311842, 5.000000000000000000 ) ) ;
#33333=CARTESIAN_POINT ( 'NONE',  ( -2.071067811865478170, -165.4375000027312126, 5.000000000000000000 ) ) ;
#33339=EDGE_CURVE ( 'NONE', #37665, #1132, #58009, .T. ) ;
#33347=CARTESIAN_POINT ( 'NONE',  ( 4.458734124999998549, -16.72916666530107577, -2.574251347313721627 ) ) ;
#33348=LINE ( 'NONE', #38784, #25755 ) ;
#33350=CARTESIAN_POINT ( 'NONE',  ( 4.458734124999998549, -42.97916666530107932, -2.574251347313721627 ) ) ;
#33356=CARTESIAN_POINT ( 'NONE',  ( -2.229367062499996610, 13.85416666803226171, 3.861377020970582219 ) ) ;
#33359=CARTESIAN_POINT ( 'NONE',  ( -4.458734124999997661, -90.47916666530106511, 2.574251347313722516 ) ) ;
#33361=CARTESIAN_POINT ( 'NONE',  ( 1.060575238724906964E-15, 16.37500000273118417, 5.773502691896257311 ) ) ;
#33362=ORIENTED_EDGE ( 'NONE', *, *, #50875, .T. ) ;
#33363=CARTESIAN_POINT ( 'NONE',  ( -1.339745962155610925, -6.669658196007334894, 5.000000000000000000 ) ) ;
#33365=DIRECTION ( 'NONE',  ( 0.000000000000000000, 0.000000000000000000, 1.000000000000000000 ) ) ;
#33366=CARTESIAN_POINT ( 'NONE',  ( -5.000000000000000000, -29.08333333333332860, -2.886751345948128211 ) ) ;
#33367=CARTESIAN_POINT ( 'NONE',  ( 4.458734124999998549, -31.72916666530107577, -2.574251347313721627 ) ) ;
#33368=CARTESIAN_POINT ( 'NONE',  ( -4.999999999999999112, -35.79166666393548013, 2.886751345948131764 ) ) ;
#33370=CARTESIAN_POINT ( 'NONE',  ( -4.458734124999999437, -62.31249999863440792, 0.000000000000000000 ) ) ;
#33371=VERTEX_POINT ( 'NONE', #9405 ) ;
#33373=CARTESIAN_POINT ( 'NONE',  ( 2.229367062499998831, -13.89583333196774184, -3.861377020970580887 ) ) ;
#33374=ORIENTED_EDGE ( 'NONE', *, *, #13465, .F. ) ;
#33375=CARTESIAN_POINT ( 'NONE',  ( -5.000000000000000000, -79.00000000000000000, 0.000000000000000000 ) ) ;
#33376=CARTESIAN_POINT ( 'NONE',  ( 1.339745962155614034, 28.41965820146970501, 5.000000000000000000 ) ) ;
#33378=CARTESIAN_POINT ( 'NONE',  ( -3.535250795749689387E-16, -80.12499999726880162, -5.773502691896257311 ) ) ;
#33379=DIRECTION ( 'NONE',  ( 0.000000000000000000, 0.000000000000000000, 1.000000000000000000 ) ) ;
#33380=ORIENTED_EDGE ( 'NONE', *, *, #16531, .T. ) ;
#33382=CARTESIAN_POINT ( 'NONE',  ( 9.457646018065525792E-16, -20.31249999863440081, 5.148502694627439702 ) ) ;
#33383=CARTESIAN_POINT ( 'NONE',  ( 4.458734124999999437, -55.06249999863440081, -5.460374474430324690E-16 ) ) ;
#33386=CARTESIAN_POINT ( 'NONE',  ( 4.458734125000000326, -165.6250000013656063, -1.846868145590734978 ) ) ;
#33388=CARTESIAN_POINT ( 'NONE',  ( 1.975475456537005874E-15, -50.62499999726881583, 5.000000000000000000 ) ) ;
#33394=EDGE_CURVE ( 'NONE', #15666, #18516, #14419, .T. ) ;
#33398=CARTESIAN_POINT ( 'NONE',  ( -4.458734125000001214, -146.1250000013655779, 1.846868145590734089 ) ) ;
#33402=CARTESIAN_POINT ( 'NONE',  ( -4.458734124999998549, -66.47916666530106511, 2.574251347313722516 ) ) ;
#33404=DIRECTION ( 'NONE',  ( -0.000000000000000000, 1.000000000000000000, -0.000000000000000000 ) ) ;
#33405=CARTESIAN_POINT ( 'NONE',  ( -1.846868145590737420, -142.7500000013655779, 4.458734124999997661 ) ) ;
#33409=CARTESIAN_POINT ( 'NONE',  ( 2.071067811865370256, -159.8125000000000000, -5.000000000000105693 ) ) ;
#33414=CARTESIAN_POINT ( 'NONE',  ( -4.458734124999999437, 25.43750000136559208, 0.000000000000000000 ) ) ;
#33415=CARTESIAN_POINT ( 'NONE',  ( -4.999999999999998224, 23.20833333606451632, 2.886751345948131764 ) ) ;
#33421=CARTESIAN_POINT ( 'NONE',  ( 5.000000000000000000, -80.41666666666665719, -2.886751345948130876 ) ) ;
#33422=CARTESIAN_POINT ( 'NONE',  ( 2.229367062500001939, 3.020833334698928674, 3.861377020970579999 ) ) ;
#33423=CARTESIAN_POINT ( 'NONE',  ( -4.458734124999999437, -25.64583333196773651, -2.574251347313719407 ) ) ;
#33424=CARTESIAN_POINT ( 'NONE',  ( -8.190561711645485556E-16, -156.6875000013655779, 4.458734124999999437 ) ) ;
#33428=CARTESIAN_POINT ( 'NONE',  ( 2.229367062500001939, 29.02083333469892779, 3.861377020970579999 ) ) ;
#33431=CARTESIAN_POINT ( 'NONE',  ( 2.229367062499998831, -72.89583333196773651, -3.861377020970580887 ) ) ;
#33434=CARTESIAN_POINT ( 'NONE',  ( 2.071067811865327624, -155.9375000027312126, -5.000000000000148326 ) ) ;
#33436=CYLINDRICAL_SURFACE ( 'NONE', #29355, 5.000000000000000000 ) ;
#33437=CARTESIAN_POINT ( 'NONE',  ( -2.500000000000000444, 11.95833333606451809, -4.330127018922193649 ) ) ;
#33438=CARTESIAN_POINT ( 'NONE',  ( 5.000000000000000000, -10.41666666666666430, -2.886751345948129988 ) ) ;
#33439=CARTESIAN_POINT ( 'NONE',  ( 9.457646018065525792E-16, -17.06249999863440792, 5.148502694627439702 ) ) ;
#33441=CARTESIAN_POINT ( 'NONE',  ( -4.458734124999999437, -77.39583333196772230, -2.574251347313719407 ) ) ;
#33442=CARTESIAN_POINT ( 'NONE',  ( 4.458734124999999437, -168.7500000013656063, 1.846868145590737864 ) ) ;
#33443=CARTESIAN_POINT ( 'NONE',  ( -2.500000000000000444, -20.04166666393548013, -4.330127018922193649 ) ) ;
#33444=CARTESIAN_POINT ( 'NONE',  ( -4.458734124999999437, -43.31249999863440081, 0.000000000000000000 ) ) ;
#33445=ORIENTED_EDGE ( 'NONE', *, *, #29530, .T. ) ;
#33446=CARTESIAN_POINT ( 'NONE',  ( 2.499999999999998668, -15.20833333060214443, -4.330127018922193649 ) ) ;
#33447=CARTESIAN_POINT ( 'NONE',  ( 9.457646018065525792E-16, 5.687500001365592972, 5.148502694627439702 ) ) ;
#33449=CARTESIAN_POINT ( 'NONE',  ( 1.339745962155615144, -34.58034179853028434, 4.999999999999999112 ) ) ;
#33450=CARTESIAN_POINT ( 'NONE',  ( -3.535250795749689387E-16, -62.25000000000000000, -5.773502691896257311 ) ) ;
#33451=CARTESIAN_POINT ( 'NONE',  ( 2.730187237215162345E-16, -156.4375000013655779, -4.458734124999999437 ) ) ;
#33453=CARTESIAN_POINT ( 'NONE',  ( 1.975475456537005874E-15, -78.74999999999998579, 5.000000000000000000 ) ) ;
#33454=CARTESIAN_POINT ( 'NONE',  ( -3.535533905932738641, -165.3750000000000284, 3.535533905932737309 ) ) ;
#33455=CARTESIAN_POINT ( 'NONE',  ( 2.499999999999998668, 5.791666669397853795, -4.330127018922193649 ) ) ;
#33457=CARTESIAN_POINT ( 'NONE',  ( 2.229367062500001939, -6.229166665301072214, 3.861377020970579999 ) ) ;
#33458=CARTESIAN_POINT ( 'NONE',  ( 2.229367062499998831, -39.89583333196773651, -3.861377020970580887 ) ) ;
#33460=CARTESIAN_POINT ( 'NONE',  ( -8.190561711645485556E-16, -147.6875000013656063, 4.458734124999999437 ) ) ;
#33462=ORIENTED_EDGE ( 'NONE', *, *, #29997, .F. ) ;
#33465=( BOUNDED_CURVE ( )  B_SPLINE_CURVE ( 2, ( #6772, #36997, #1966, #26384, #3223, #51786, #7728, #46001, #21567 ),
 .UNSPECIFIED., .F., .F. ) 
 B_SPLINE_CURVE_WITH_KNOTS ( ( 3, 2, 2, 2, 3 ),
 ( 0.3729166666666666741, 0.3736111111111111160, 0.3750000000000000000, 0.3763888888888888840, 0.3770833333333333259 ),
 .UNSPECIFIED. ) 
 CURVE ( )  GEOMETRIC_REPRESENTATION_ITEM ( )  RATIONAL_B_SPLINE_CURVE ( ( 0.9330127018922194093, 0.9330127018922194093, 1.000000000000000000, 0.8660254037844387076, 1.000000000000000000, 0.8660254037844387076, 1.000000000000000000, 0.9330127018922194093, 0.9330127018922194093 ) ) 
 REPRESENTATION_ITEM ( '' )  );
#33467=CARTESIAN_POINT ( 'NONE',  ( -4.458734124999999437, -74.56249999863440792, 0.000000000000000000 ) ) ;
#33468=EDGE_LOOP ( 'NONE', ( #41316, #61539, #29393, #29954 ) ) ;
#33469=EDGE_CURVE ( 'NONE', #8855, #39123, #21389, .T. ) ;
#33473=EDGE_CURVE ( 'NONE', #22889, #32917, #15826, .T. ) ;
#33475=CARTESIAN_POINT ( 'NONE',  ( 4.458734124999998549, 3.270833334698929118, -2.574251347313721627 ) ) ;
#33476=CARTESIAN_POINT ( 'NONE',  ( -9.184850993605147944E-16, -164.2500000000000000, 5.000000000000000000 ) ) ;
#33477=CARTESIAN_POINT ( 'NONE',  ( 2.730187237215162345E-16, -154.1875000013656063, -4.458734124999999437 ) ) ;
#33487=EDGE_CURVE ( 'NONE', #26202, #49021, #53779, .T. ) ;
#33488=CARTESIAN_POINT ( 'NONE',  ( -4.999999999999998224, -12.91666666666666607, 2.886751345948131764 ) ) ;
#33491=DIRECTION ( 'NONE',  ( 0.000000000000000000, 0.000000000000000000, 1.000000000000000000 ) ) ;
#33493=CARTESIAN_POINT ( 'NONE',  ( 2.500000000000002220, -44.66666666666665719, 4.330127018922192761 ) ) ;
#33495=CARTESIAN_POINT ( 'NONE',  ( 4.458734124999998549, 18.27083333469893134, -2.574251347313721627 ) ) ;
#33496=EDGE_CURVE ( 'NONE', #39254, #21932, #45090, .T. ) ;
#33498=CARTESIAN_POINT ( 'NONE',  ( -2.229367062499996610, -8.395833331967736513, 3.861377020970582219 ) ) ;
#33499=( BOUNDED_CURVE ( )  B_SPLINE_CURVE ( 2, ( #57625, #28333, #58236, #13853, #37363, #8719, #22899, #18049, #13553 ),
 .UNSPECIFIED., .F., .F. ) 
 B_SPLINE_CURVE_WITH_KNOTS ( ( 3, 2, 2, 2, 3 ),
 ( 0.9145833333333333037, 0.9152777777777777457, 0.9166666666666666297, 0.9180555555555555136, 0.9187499999999999556 ),
 .UNSPECIFIED. ) 
 CURVE ( )  GEOMETRIC_REPRESENTATION_ITEM ( )  RATIONAL_B_SPLINE_CURVE ( ( 0.9330127018922194093, 0.9330127018922194093, 1.000000000000000000, 0.8660254037844387076, 1.000000000000000000, 0.8660254037844387076, 1.000000000000000000, 0.9330127018922194093, 0.9330127018922194093 ) ) 
 REPRESENTATION_ITEM ( '' )  );
#33503=CARTESIAN_POINT ( 'NONE',  ( 4.458734124999999437, -168.5000000013656063, 1.846868145590737864 ) ) ;
#33505=ADVANCED_FACE ( 'NONE', ( #20661 ), #44121, .T. ) ;
#33512=CARTESIAN_POINT ( 'NONE',  ( -1.846868145590737420, -156.0000000013656063, 4.458734124999997661 ) ) ;
#33514=CARTESIAN_POINT ( 'NONE',  ( -5.147856630858197489E-14, 2.375000002731183724, 5.000000000000000000 ) ) ;
#33521=CARTESIAN_POINT ( 'NONE',  ( -5.000000000000000000, 4.000000000000000000, 0.000000000000000000 ) ) ;
#33522=AXIS2_PLACEMENT_3D ( 'NONE', #44336, #18946, #53683 ) ;
#33523=CARTESIAN_POINT ( 'NONE',  ( -2.229367062499996610, -64.14583333196773651, 3.861377020970582219 ) ) ;
#33526=CARTESIAN_POINT ( 'NONE',  ( -5.000000000000000000, -1.958333330602145761, -2.886751345948128211 ) ) ;
#33527=CARTESIAN_POINT ( 'NONE',  ( 4.458734125000001214, -26.89583333196774007, 2.574251347313718519 ) ) ;
#33528=DIRECTION ( 'NONE',  ( 0.000000000000000000, 0.000000000000000000, 1.000000000000000000 ) ) ;
#33531=CARTESIAN_POINT ( 'NONE',  ( 2.500000000000002220, -46.66666666666666430, 4.330127018922192761 ) ) ;
#33534=CARTESIAN_POINT ( 'NONE',  ( -1.339745962155623360, 14.33034180399266155, 4.999999999999991118 ) ) ;
#33535=CARTESIAN_POINT ( 'NONE',  ( -2.229367062499996610, -68.14583333196773651, 3.861377020970582219 ) ) ;
#33536=CARTESIAN_POINT ( 'NONE',  ( 4.458734124999999437, -148.6875000013656063, 0.000000000000000000 ) ) ;
#33537=CARTESIAN_POINT ( 'NONE',  ( 2.229367062500001939, -77.97916666530106511, 3.861377020970579999 ) ) ;
#33539=CARTESIAN_POINT ( 'NONE',  ( -4.458734124999999437, -23.56249999863440436, 0.000000000000000000 ) ) ;
#33540=CARTESIAN_POINT ( 'NONE',  ( -5.000000000000000000, -63.95833333060213732, -2.886751345948128211 ) ) ;
#33545=CARTESIAN_POINT ( 'NONE',  ( -1.339745962155613812, 7.919658201469706782, -5.000000000000000000 ) ) ;
#33548=CARTESIAN_POINT ( 'NONE',  ( -4.458734124999999437, -52.64583333196773651, -2.574251347313719407 ) ) ;
#33550=ORIENTED_EDGE ( 'NONE', *, *, #46056, .T. ) ;
#33551=CARTESIAN_POINT ( 'NONE',  ( 1.975475456537005874E-15, 9.250000000000000000, 5.000000000000000000 ) ) ;
#33552=CARTESIAN_POINT ( 'NONE',  ( 4.458734124999999437, 18.18750000136559564, -5.460374474430324690E-16 ) ) ;
#33555=CARTESIAN_POINT ( 'NONE',  ( 4.458734124999999437, -163.3750000013656347, -1.846868145590734978 ) ) ;
#33558=CARTESIAN_POINT ( 'NONE',  ( 1.339745962155615144, -39.70534180126147561, 4.999999999999999112 ) ) ;
#33561=AXIS2_PLACEMENT_3D ( 'NONE', #28818, #48438, #63244 ) ;
#33562=CARTESIAN_POINT ( 'NONE',  ( -2.499999999999996447, 2.166666666666667407, 4.330127018922195425 ) ) ;
#33566=CARTESIAN_POINT ( 'NONE',  ( 2.499999999999998668, -45.33333333333333570, -4.330127018922193649 ) ) ;
#33568=CARTESIAN_POINT ( 'NONE',  ( -3.535533905932737309, -156.6250000000000000, -3.535533905932738197 ) ) ;
#33569=CARTESIAN_POINT ( 'NONE',  ( 0.000000000000000000, -170.0000000000000000, 0.000000000000000000 ) ) ;
#33570=EDGE_CURVE ( 'NONE', #58699, #46845, #58925, .T. ) ;
#33574=CARTESIAN_POINT ( 'NONE',  ( 5.000000000000000888, -148.0625000027312126, -2.071067811865475505 ) ) ;
#33578=( BOUNDED_CURVE ( )  B_SPLINE_CURVE ( 2, ( #35900, #35260, #55208, #55841, #44581, #45224, #49411, #538, #6008 ),
 .UNSPECIFIED., .F., .F. ) 
 B_SPLINE_CURVE_WITH_KNOTS ( ( 3, 2, 2, 2, 3 ),
 ( 0.9354166666666666741, 0.9361111111111111160, 0.9375000000000000000, 0.9388888888888888840, 0.9395833333333333259 ),
 .UNSPECIFIED. ) 
 CURVE ( )  GEOMETRIC_REPRESENTATION_ITEM ( )  RATIONAL_B_SPLINE_CURVE ( ( 0.9330127018922194093, 0.9330127018922194093, 1.000000000000000000, 0.8660254037844387076, 1.000000000000000000, 0.8660254037844387076, 1.000000000000000000, 0.9330127018922194093, 0.9330127018922194093 ) ) 
 REPRESENTATION_ITEM ( '' )  );
#33580=CARTESIAN_POINT ( 'NONE',  ( -3.535533905932738641, -143.3750000000000000, 3.535533905932737309 ) ) ;
#33581=EDGE_CURVE ( 'NONE', #11760, #5864, #16501, .T. ) ;
#33584=CARTESIAN_POINT ( 'NONE',  ( -4.458734124999999437, -32.31249999863440792, 0.000000000000000000 ) ) ;
#33588=CARTESIAN_POINT ( 'NONE',  ( -1.846868145590737420, -146.7500000013656063, 4.458734124999999437 ) ) ;
#33589=ORIENTED_EDGE ( 'NONE', *, *, #27592, .F. ) ;
#33590=CARTESIAN_POINT ( 'NONE',  ( 4.458734125000001214, 26.85416666803225993, 2.574251347313718519 ) ) ;
#33592=CARTESIAN_POINT ( 'NONE',  ( 2.229367062500001939, -55.22916666530107221, 3.861377020970579999 ) ) ;
#33595=CARTESIAN_POINT ( 'NONE',  ( -3.535250795749689387E-16, 16.75000000000000355, -5.773502691896257311 ) ) ;
#33596=CARTESIAN_POINT ( 'NONE',  ( -1.339745962155613812, -89.20534180126146850, -5.000000000000000000 ) ) ;
#33597=CARTESIAN_POINT ( 'NONE',  ( -4.458734124999999437, -7.312499998634404363, 0.000000000000000000 ) ) ;
#33599=CARTESIAN_POINT ( 'NONE',  ( 2.499999999999998668, -48.33333333333332860, -4.330127018922193649 ) ) ;
#33601=CARTESIAN_POINT ( 'NONE',  ( 4.458734124999999437, 9.937500001365593860, -5.460374474430324690E-16 ) ) ;
#33602=CARTESIAN_POINT ( 'NONE',  ( 2.500000000000002220, -53.54166666393548013, 4.330127018922192761 ) ) ;
#33606=CARTESIAN_POINT ( 'NONE',  ( 4.458734125000001214, -54.89583333196773651, 2.574251347313718519 ) ) ;
#33607=CARTESIAN_POINT ( 'NONE',  ( -4.458734124999999437, -159.1875000013655779, -5.460374474430324690E-16 ) ) ;
#33608=MECHANICAL_DESIGN_GEOMETRIC_PRESENTATION_REPRESENTATION('',(#2819),#31546);
#33609=CARTESIAN_POINT ( 'NONE',  ( 2.499999999999998668, -49.20833333060213732, -4.330127018922193649 ) ) ;
#33612=CARTESIAN_POINT ( 'NONE',  ( -3.152548672688508926E-16, 7.187500001365594748, -5.148502694627439702 ) ) ;
#33613=VERTEX_POINT ( 'NONE', #50556 ) ;
#33616=CARTESIAN_POINT ( 'NONE',  ( 2.730187237215162345E-16, -161.1875000013655779, -4.458734124999999437 ) ) ;
#33618=DIRECTION ( 'NONE',  ( -0.000000000000000000, 1.000000000000000000, -0.000000000000000000 ) ) ;
#33621=CARTESIAN_POINT ( 'NONE',  ( -2.229367062500000163, -35.72916666530107221, -3.861377020970580443 ) ) ;
#33623=EDGE_CURVE ( 'NONE', #44350, #51351, #34139, .T. ) ;
#33627=CARTESIAN_POINT ( 'NONE',  ( -3.152548672688508926E-16, -87.81249999863439371, -5.148502694627439702 ) ) ;
#33629=CARTESIAN_POINT ( 'NONE',  ( -4.764381983412779477E-15, 25.37500000273118062, 5.000000000000000000 ) ) ;
#33631=CARTESIAN_POINT ( 'NONE',  ( -1.339745962155613812, -45.08034179853028434, -5.000000000000000000 ) ) ;
#33639=DIRECTION ( 'NONE',  ( -0.000000000000000000, 1.000000000000000000, -0.000000000000000000 ) ) ;
#33640=CARTESIAN_POINT ( 'NONE',  ( -6.972266317189433020E-16, -69.24999999999998579, -5.000000000000000000 ) ) ;
#33641=CARTESIAN_POINT ( 'NONE',  ( -4.458734124999998549, -84.47916666530107932, 2.574251347313722516 ) ) ;
#33644=( BOUNDED_SURFACE ( )  B_SPLINE_SURFACE ( 1, 2, ( 
 ( #16338, #56535, #46236, #61049, #55585, #56213, #12456, #21803, #31121, #41398, #50743, #1558, #12135, #17281, #31757, #6687, #45917, #51390, #36905, #27248, #1247, #1879, #21484, #7332, #20847, #26943, #46559, #47191, #3133, #33025, #33648, #13710, #17909, #42666, #8270, #37854, #4073, #57487, #9202, #52641, #57791, #62305, #48121, #62624, #18547, #8575, #13087, #22753, #37224, #28186, #32708, #38168, #3759, #13404, #52952, #32390, #14020, #53267, #27558, #33333, #61675, #23693, #47802, #42351, #23382, #61989, #38461, #37530, #8889, #42981, #12767, #17608, #56850, #57171, #62928, #47493, #28502, #46875, #2817, #52336, #18227, #52015, #43293, #27873, #22438, #18843, #3446, #7958, #42033, #23061, #58089, #48434, #34577, #510, #14338, #39090, #9815, #33959, #29426, #53580, #9508, #54209, #44554, #20120, #4376, #39403, #19154, #44879, #10146, #25260, #842, #197, #35236, #48738, #29117, #4682, #29753, #39722, #59359, #23993, #59039, #38772, #20445, #49386, #40044, #59686, #19795, #54855, #24304, #14969, #10459, #58410, #34263, #63558, #15619, #5331, #28814, #43597, #24948, #15294, #43909, #58720, #14646, #19476, #63240, #34916, #54538, #53891, #30073, #49058, #49703, #5006, #5647, #24626, #44232, #1800, #7253, #31347, #21081, #45197, #21403, #12055, #31679, #51315, #40686, #25584, #41319, #17202, #41627, #26865, #11101, #30725, #60649, #61281, #60967, #45517, #6604, #35877, #41007, #46478, #16572, #36830, #36194, #21724, #26218, #2424, #26540, #46161, #55815, #60331, #50348, #1164, #11731, #16258, #2123, #50990, #6929, #16887, #60010, #10788, #30398, #55180, #36503, #20763, #22036, #56133, #6295, #50021, #25900, #5975, #1478, #40369, #15933, #35556, #55506, #11420, #31039, #50664, #45838, #47732, #56460, #12382, #32309, #27798, #22358, #52257, #51938, #31995, #18148, #22678, #7563, #62856, #18769, #43216, #51629, #62230, #28115, #41956, #3060, #37460, #61599, #57090, #27175, #46792, #7880, #8816, #13009, #3688, #2738, #17534, #27483, #47423, #37152, #8196, #47112, #56777, #37776, #42277, #12696, #61917, #17837, #32629, #3375, #57408, #23302, #22992, #42593, #13328, #32949, #52572, #8505, #42902, #62551, #18471, #38091, #57717, #13642, #33263, #28432, #52881, #48045, #3997, #23619, #44800, #58337, #4934, #20043, #48361, #43838, #9435, #10394, #58964, #25185, #38396, #29351, #14891, #4305, #48669, #4609, #33885, #30004, #48985, #34498, #29044, #54132, #49634, #19722, #14265, #24554, #53505, #43525, #44159, #34844, #10070, #24232, #9128, #128, #39648, #59286, #15217, #63484, #53195, #5256, #763, #5571, #54467, #38700, #19407, #39331, #58020, #24877, #39022, #34193, #58650, #29684, #13948, #49313, #33574, #44478, #437, #53816, #28735, #23924, #63169, #19080, #14571, #9746, #10715, #26146, #50270, #55740, #40927, #50592, #26467, #5899, #51240, #7175, #1089, #50910, #35169, #60886, #6532, #59940, #11344, #40302, #11976, #15863, #46083, #45765, #49944, #55101, #16495, #31605, #1721, #35484, #30967, #11026, #25505, #21327, #16810, #60573, #30648, #54785, #36117, #21647, #41239, #36431, #6217, #30322, #6852, #26783, #46402, #56060, #20697, #25829, #11656, #20371, #2042, #45445, #16178, #1409, #31276, #39971, #59616, #15548, #45124, #21009, #35803, #40616, #60260, #55427, #27725, #32230, #2660, #56384, #8122, #51861, #37692, #22923, #32552, #8436, #51551, #33192, #52807, #46715, #32873, #17130, #42830, #52177, #41880, #57014, #22280, #57646, #61526, #28040, #47352, #31923, #36754, #12310, #17457, #18394, #2987, #57334, #2351, #21959, #37080, #37381, #7486, #61845, #56701, #41555, #3301, #7804, #27099, #8744, #28351, #61206, #12618, #42515, #13250, #27406, #47038, #22604, #42201, #17764, #12929, #62152, #18070, #52502, #47659, #3612, #23219, #62474, #38014, #13574, #44403, #19965, #19329, #54391, #4236, #14498 ),
 ( #39575, #38943, #44083, #48, #19647, #53119, #9362, #362, #9674, #29608, #58884, #13876, #48912, #3923, #34429, #33503, #10318, #54057, #59214, #18701, #58263, #47968, #14815, #9054, #39258, #28664, #23542, #24163, #43454, #48280, #15144, #49238, #28975, #23851, #48597, #9995, #4858, #24478, #63099, #5180, #63412, #19011, #24798, #43141, #38326, #34119, #34765, #62782, #29282, #58579, #57955, #53742, #38624, #14185, #33812, #53429, #43766, #4537, #40539, #49554, #11269, #55988, #45371, #1337, #5814, #55025, #20935, #25758, #20292, #16741, #1648, #25432, #5496, #45050, #30894, #21247, #60180, #49866, #60816, #35403, #44721, #31209, #30243, #1017, #30567, #25110, #40854, #59863, #40228, #10948, #50838, #16102, #50524, #60497, #39893, #50191, #45691, #10630, #6779, #29929, #36358, #26073, #54710, #16425, #683, #35726, #59539, #20621, #1972, #36044, #15787, #55674, #6143, #55355, #6465, #21572, #11589, #26389, #46007, #41169, #15474, #35091, #46327, #7733, #3537, #51165, #46645, #31848, #62397, #42754, #56308, #41808, #26713, #12234, #2286, #27338, #23146, #7098, #2590, #51480, #18318, #37943, #7418, #27653, #47280, #17059, #37002, #8362, #37309, #57260, #22847, #41485, #12859, #31523, #62080, #61137, #11903, #17993, #21889, #36676, #22210, #27027, #42437, #61453, #8049, #17383, #56629, #51791, #12542, #32155, #27963, #13179, #46969, #2916, #22529, #37619, #32478, #52107, #42125, #32801, #61767, #17695, #3229, #56938, #52430, #47586, #54553, #15310, #20137, #4467, #33117, #28906, #15635, #9289, #59376, #8666, #33737, #52734, #24094, #13501, #39736, #20780, #48527, #43689, #33424, #18935, #63336, #53354, #47892, #45214, #30089, #53043, #28278, #8980, #34932, #49719, #10476, #13804, #25601, #63028, #3848, #59703, #57879, #28591, #58183, #23469, #5664, #23781, #4166, #38551, #35251, #25277, #44899, #858, #43073, #14111, #20461, #38258, #54871, #57576, #1180, #40060, #18636, #10802, #62710, #30414, #48211, #43383, #50038, #5997, #21096, #7267, #1493, #1814, #51004, #12395, #2441, #21418, #41021, #32010, #21739, #16273, #6944, #35892, #45532, #31363, #36844, #60981, #50677, #11115, #26555, #41643, #61295, #17217, #6619, #55195, #26879, #46806, #7578, #56474, #40700, #60345, #46175, #27190, #46493, #11436, #36208, #60664, #2136, #51644, #41334, #2753, #16902, #51329, #55830, #40385, #56148, #12069, #36518, #26232, #55523, #30742, #31694, #45852, #22050, #60026, #15949, #35571, #25914, #50362, #6310, #31054, #16588, #11745, #62870, #8519, #61932, #13343, #42291, #13961, #17851, #48060, #47747, #51955, #37168, #56791, #37473, #38409, #23007, #13657, #22372, #41972, #57108, #57422, #7893, #18165, #13025, #61614, #3703, #52273, #12709, #28750, #48375, #9141, #17548, #28129, #57731, #27498, #32642, #3390, #47127, #42608, #3075, #22692, #23318, #38107, #33277, #32325, #32963, #8210, #58031, #42919, #18782, #33588, #52587, #27813, #47438, #62566, #4013, #62246, #37792, #18485, #53207, #52896, #8832, #28445, #23634, #43229, #14278, #14585, #34205, #63496, #59628, #58978, #453, #39035, #20057, #33897, #29365, #39661, #48681, #44814, #4317, #10727, #59298, #29057, #15230, #54799, #34514, #23937, #4621, #39983, #34858, #24246, #54479, #43850, #48998, #14905, #15561, #30018, #4945, #24568, #53829, #19093, #19421, #38711, #140, #35181, #43538, #58662, #9758, #30334, #63182, #44173, #10406, #49646, #9448, #19734, #776, #29695, #5583, #25200, #53520, #5269, #58350, #20383, #39348, #54145, #10084, #49326, #24890, #44491, #12322, #60899, #15876, #46093, #35496, #25519, #26157, #45457, #50283, #2364, #51252, #11355, #55114, #30978, #16822, #6864, #26479, #11039, #36441, #1735, #30662, #21661, #45137, #40315, #36129, #2053, #41252, #11668, #60588, #1101, #21338, #7187, #40938, #50922, #20710, #45776, #59953, #16508, #5912 ) ),
 .UNSPECIFIED., .F., .F., .F. ) 
 B_SPLINE_SURFACE_WITH_KNOTS ( ( 2, 2 ),
 ( 3, 2, 2, 2, 2, 2, 2, 2, 2, 2, 2, 2, 2, 2, 2, 2, 2, 2, 2, 2, 2, 2, 2, 2, 2, 2, 2, 2, 2, 2, 2, 2, 2, 2, 2, 2, 2, 2, 2, 2, 2, 2, 2, 2, 2, 2, 2, 2, 2, 2, 2, 2, 2, 2, 2, 2, 2, 2, 2, 2, 2, 2, 2, 2, 2, 2, 2, 2, 2, 2, 2, 2, 2, 2, 2, 2, 2, 2, 2, 2, 2, 2, 2, 2, 2, 2, 2, 2, 2, 2, 2, 2, 2, 2, 2, 2, 2, 2, 2, 2, 2, 2, 2, 2, 2, 2, 2, 2, 2, 2, 2, 2, 2, 2, 2, 2, 2, 2, 2, 2, 2, 2, 2, 2, 2, 2, 2, 2, 2, 2, 2, 2, 2, 2, 2, 2, 2, 2, 2, 2, 2, 2, 2, 2, 2, 2, 2, 2, 2, 2, 2, 2, 2, 2, 2, 2, 2, 2, 2, 2, 2, 2, 2, 2, 2, 2, 2, 2, 2, 2, 2, 2, 2, 2, 2, 2, 2, 2, 2, 2, 2, 2, 2, 2, 2, 2, 2, 2, 2, 2, 2, 2, 2, 2, 2, 2, 2, 2, 2, 2, 2, 2, 2, 2, 2, 2, 2, 2, 2, 2, 2, 2, 2, 2, 2, 2, 2, 2, 2, 2, 2, 2, 2, 2, 2, 2, 2, 2, 2, 2, 2, 2, 2, 2, 2, 2, 2, 2, 2, 2, 3 ),
 ( 0.000000000000000000, 1.000000000000000000 ),
 ( 0.000000000000000000, 0.004166666666666666609, 0.008333333333333333218, 0.01250000000000000069, 0.01666666666666666644, 0.02083333333333333218, 0.02500000000000000139, 0.02916666666666666713, 0.03333333333333333287, 0.03749999999999999861, 0.04166666666666666435, 0.04583333333333333010, 0.05000000000000000278, 0.05416666666666666852, 0.05833333333333333426, 0.06250000000000000000, 0.06666666666666666574, 0.07083333333333333148, 0.07499999999999999722, 0.07916666666666666297, 0.08333333333333332871, 0.08749999999999999445, 0.09166666666666666019, 0.09583333333333333981, 0.1000000000000000056, 0.1041666666666666713, 0.1083333333333333370, 0.1125000000000000028, 0.1166666666666666685, 0.1208333333333333343, 0.1250000000000000000, 0.1291666666666666796, 0.1333333333333333315, 0.1375000000000000111, 0.1416666666666666630, 0.1458333333333333426, 0.1499999999999999944, 0.1541666666666666741, 0.1583333333333333259, 0.1625000000000000056, 0.1666666666666666574, 0.1708333333333333370, 0.1749999999999999889, 0.1791666666666666685, 0.1833333333333333204, 0.1875000000000000000, 0.1916666666666666796, 0.1958333333333333315, 0.2000000000000000111, 0.2041666666666666630, 0.2083333333333333426, 0.2124999999999999944, 0.2166666666666666741, 0.2208333333333333259, 0.2250000000000000056, 0.2291666666666666574, 0.2333333333333333370, 0.2374999999999999889, 0.2416666666666666685, 0.2458333333333333204, 0.2500000000000000000, 0.2541666666666666519, 0.2583333333333333592, 0.2625000000000000111, 0.2666666666666666630, 0.2708333333333333148, 0.2750000000000000222, 0.2791666666666666741, 0.2833333333333333259, 0.2874999999999999778, 0.2916666666666666852, 0.2958333333333333370, 0.2999999999999999889, 0.3041666666666666408, 0.3083333333333333481, 0.3125000000000000000, 0.3166666666666666519, 0.3208333333333333592, 0.3250000000000000111, 0.3291666666666666630, 0.3333333333333333148, 0.3375000000000000222, 0.3416666666666666741, 0.3458333333333333259, 0.3499999999999999778, 0.3541666666666666852, 0.3583333333333333370, 0.3624999999999999889, 0.3666666666666666408, 0.3708333333333333481, 0.3750000000000000000, 0.3791666666666666519, 0.3833333333333333592, 0.3875000000000000111, 0.3916666666666666630, 0.3958333333333333148, 0.4000000000000000222, 0.4041666666666666741, 0.4083333333333333259, 0.4124999999999999778, 0.4166666666666666852, 0.4208333333333333370, 0.4249999999999999889, 0.4291666666666666408, 0.4333333333333333481, 0.4375000000000000000, 0.4416666666666666519, 0.4458333333333333592, 0.4500000000000000111, 0.4541666666666666630, 0.4583333333333333148, 0.4625000000000000222, 0.4666666666666666741, 0.4708333333333333259, 0.4749999999999999778, 0.4791666666666666852, 0.4833333333333333370, 0.4874999999999999889, 0.4916666666666666408, 0.4958333333333333481, 0.5000000000000000000, 0.5041666666666666519, 0.5083333333333333037, 0.5124999999999999556, 0.5166666666666667185, 0.5208333333333333703, 0.5250000000000000222, 0.5291666666666666741, 0.5333333333333333259, 0.5374999999999999778, 0.5416666666666666297, 0.5458333333333332815, 0.5500000000000000444, 0.5541666666666666963, 0.5583333333333333481, 0.5625000000000000000, 0.5666666666666666519, 0.5708333333333333037, 0.5749999999999999556, 0.5791666666666667185, 0.5833333333333333703, 0.5875000000000000222, 0.5916666666666666741, 0.5958333333333333259, 0.5999999999999999778, 0.6041666666666666297, 0.6083333333333332815, 0.6125000000000000444, 0.6166666666666666963, 0.6208333333333333481, 0.6250000000000000000, 0.6291666666666666519, 0.6333333333333333037, 0.6374999999999999556, 0.6416666666666667185, 0.6458333333333333703, 0.6500000000000000222, 0.6541666666666666741, 0.6583333333333333259, 0.6624999999999999778, 0.6666666666666666297, 0.6708333333333332815, 0.6750000000000000444, 0.6791666666666666963, 0.6833333333333333481, 0.6875000000000000000, 0.6916666666666666519, 0.6958333333333333037, 0.6999999999999999556, 0.7041666666666667185, 0.7083333333333333703, 0.7125000000000000222, 0.7166666666666666741, 0.7208333333333333259, 0.7249999999999999778, 0.7291666666666666297, 0.7333333333333332815, 0.7375000000000000444, 0.7416666666666666963, 0.7458333333333333481, 0.7500000000000000000, 0.7541666666666666519, 0.7583333333333333037, 0.7624999999999999556, 0.7666666666666667185, 0.7708333333333333703, 0.7750000000000000222, 0.7791666666666666741, 0.7833333333333333259, 0.7874999999999999778, 0.7916666666666666297, 0.7958333333333332815, 0.8000000000000000444, 0.8041666666666666963, 0.8083333333333333481, 0.8125000000000000000, 0.8166666666666666519, 0.8208333333333333037, 0.8249999999999999556, 0.8291666666666667185, 0.8333333333333333703, 0.8375000000000000222, 0.8416666666666666741, 0.8458333333333333259, 0.8499999999999999778, 0.8541666666666666297, 0.8583333333333332815, 0.8625000000000000444, 0.8666666666666666963, 0.8708333333333333481, 0.8750000000000000000, 0.8791666666666666519, 0.8833333333333333037, 0.8874999999999999556, 0.8916666666666667185, 0.8958333333333333703, 0.9000000000000000222, 0.9041666666666666741, 0.9083333333333333259, 0.9124999999999999778, 0.9166666666666666297, 0.9208333333333332815, 0.9250000000000000444, 0.9291666666666666963, 0.9333333333333333481, 0.9375000000000000000, 0.9416666666666666519, 0.9458333333333333037, 0.9499999999999999556, 0.9541666666666667185, 0.9583333333333333703, 0.9625000000000000222, 0.9666666666666666741, 0.9708333333333333259, 0.9749999999999999778, 0.9791666666666666297, 0.9833333333333332815, 0.9875000000000000444, 0.9916666666666666963, 0.9958333333333333481, 1.000000000000000000 ),
 .UNSPECIFIED. ) 
 GEOMETRIC_REPRESENTATION_ITEM ( )  RATIONAL_B_SPLINE_SURFACE ( (
 ( 1.000000000000000000, 0.9238795325112867385, 1.000000000000000000, 0.9238795325112867385, 1.000000000000000000, 0.9238795325112867385, 1.000000000000000000, 0.9238795325112867385, 1.000000000000000000, 0.9238795325112867385, 1.000000000000000000, 0.9238795325112867385, 1.000000000000000000, 0.9238795325112867385, 1.000000000000000000, 0.9238795325112867385, 1.000000000000000000, 0.9238795325112867385, 1.000000000000000000, 0.9238795325112867385, 1.000000000000000000, 0.9238795325112867385, 1.000000000000000000, 0.9238795325112867385, 1.000000000000000000, 0.9238795325112867385, 1.000000000000000000, 0.9238795325112867385, 1.000000000000000000, 0.9238795325112867385, 1.000000000000000000, 0.9238795325112867385, 1.000000000000000000, 0.9238795325112867385, 1.000000000000000000, 0.9238795325112867385, 1.000000000000000000, 0.9238795325112867385, 1.000000000000000000, 0.9238795325112867385, 1.000000000000000000, 0.9238795325112867385, 1.000000000000000000, 0.9238795325112867385, 1.000000000000000000, 0.9238795325112867385, 1.000000000000000000, 0.9238795325112867385, 1.000000000000000000, 0.9238795325112867385, 1.000000000000000000, 0.9238795325112867385, 1.000000000000000000, 0.9238795325112867385, 1.000000000000000000, 0.9238795325112867385, 1.000000000000000000, 0.9238795325112867385, 1.000000000000000000, 0.9238795325112867385, 1.000000000000000000, 0.9238795325112867385, 1.000000000000000000, 0.9238795325112867385, 1.000000000000000000, 0.9238795325112867385, 1.000000000000000000, 0.9238795325112867385, 1.000000000000000000, 0.9238795325112867385, 1.000000000000000000, 0.9238795325112867385, 1.000000000000000000, 0.9238795325112867385, 1.000000000000000000, 0.9238795325112867385, 1.000000000000000000, 0.9238795325112867385, 1.000000000000000000, 0.9238795325112867385, 1.000000000000000000, 0.9238795325112867385, 1.000000000000000000, 0.9238795325112867385, 1.000000000000000000, 0.9238795325112867385, 1.000000000000000000, 0.9238795325112867385, 1.000000000000000000, 0.9238795325112867385, 1.000000000000000000, 0.9238795325112867385, 1.000000000000000000, 0.9238795325112867385, 1.000000000000000000, 0.9238795325112867385, 1.000000000000000000, 0.9238795325112867385, 1.000000000000000000, 0.9238795325112867385, 1.000000000000000000, 0.9238795325112867385, 1.000000000000000000, 0.9238795325112867385, 1.000000000000000000, 0.9238795325112867385, 1.000000000000000000, 0.9238795325112867385, 1.000000000000000000, 0.9238795325112867385, 1.000000000000000000, 0.9238795325112867385, 1.000000000000000000, 0.9238795325112867385, 1.000000000000000000, 0.9238795325112867385, 1.000000000000000000, 0.9238795325112867385, 1.000000000000000000, 0.9238795325112867385, 1.000000000000000000, 0.9238795325112867385, 1.000000000000000000, 0.9238795325112867385, 1.000000000000000000, 0.9238795325112867385, 1.000000000000000000, 0.9238795325112867385, 1.000000000000000000, 0.9238795325112867385, 1.000000000000000000, 0.9238795325112867385, 1.000000000000000000, 0.9238795325112867385, 1.000000000000000000, 0.9238795325112867385, 1.000000000000000000, 0.9238795325112867385, 1.000000000000000000, 0.9238795325112867385, 1.000000000000000000, 0.9238795325112867385, 1.000000000000000000, 0.9238795325112867385, 1.000000000000000000, 0.9238795325112867385, 1.000000000000000000, 0.9238795325112867385, 1.000000000000000000, 0.9238795325112867385, 1.000000000000000000, 0.9238795325112867385, 1.000000000000000000, 0.9238795325112867385, 1.000000000000000000, 0.9238795325112867385, 1.000000000000000000, 0.9238795325112867385, 1.000000000000000000, 0.9238795325112867385, 1.000000000000000000, 0.9238795325112867385, 1.000000000000000000, 0.9238795325112867385, 1.000000000000000000, 0.9238795325112867385, 1.000000000000000000, 0.9238795325112867385, 1.000000000000000000, 0.9238795325112867385, 1.000000000000000000, 0.9238795325112867385, 1.000000000000000000, 0.9238795325112867385, 1.000000000000000000, 0.9238795325112867385, 1.000000000000000000, 0.9238795325112867385, 1.000000000000000000, 0.9238795325112867385, 1.000000000000000000, 0.9238795325112867385, 1.000000000000000000, 0.9238795325112867385, 1.000000000000000000, 0.9238795325112867385, 1.000000000000000000, 0.9238795325112867385, 1.000000000000000000, 0.9238795325112867385, 1.000000000000000000, 0.9238795325112867385, 1.000000000000000000, 0.9238795325112867385, 1.000000000000000000, 0.9238795325112867385, 1.000000000000000000, 0.9238795325112867385, 1.000000000000000000, 0.9238795325112867385, 1.000000000000000000, 0.9238795325112867385, 1.000000000000000000, 0.9238795325112867385, 1.000000000000000000, 0.9238795325112867385, 1.000000000000000000, 0.9238795325112867385, 1.000000000000000000, 0.9238795325112867385, 1.000000000000000000, 0.9238795325112867385, 1.000000000000000000, 0.9238795325112867385, 1.000000000000000000, 0.9238795325112867385, 1.000000000000000000, 0.9238795325112867385, 1.000000000000000000, 0.9238795325112867385, 1.000000000000000000, 0.9238795325112867385, 1.000000000000000000, 0.9238795325112867385, 1.000000000000000000, 0.9238795325112867385, 1.000000000000000000, 0.9238795325112867385, 1.000000000000000000, 0.9238795325112867385, 1.000000000000000000, 0.9238795325112867385, 1.000000000000000000, 0.9238795325112867385, 1.000000000000000000, 0.9238795325112867385, 1.000000000000000000, 0.9238795325112867385, 1.000000000000000000, 0.9238795325112867385, 1.000000000000000000, 0.9238795325112867385, 1.000000000000000000, 0.9238795325112867385, 1.000000000000000000, 0.9238795325112867385, 1.000000000000000000, 0.9238795325112867385, 1.000000000000000000, 0.9238795325112867385, 1.000000000000000000, 0.9238795325112867385, 1.000000000000000000, 0.9238795325112867385, 1.000000000000000000, 0.9238795325112867385, 1.000000000000000000, 0.9238795325112867385, 1.000000000000000000, 0.9238795325112867385, 1.000000000000000000, 0.9238795325112867385, 1.000000000000000000, 0.9238795325112867385, 1.000000000000000000, 0.9238795325112867385, 1.000000000000000000, 0.9238795325112867385, 1.000000000000000000, 0.9238795325112867385, 1.000000000000000000, 0.9238795325112867385, 1.000000000000000000, 0.9238795325112867385, 1.000000000000000000, 0.9238795325112867385, 1.000000000000000000, 0.9238795325112867385, 1.000000000000000000, 0.9238795325112867385, 1.000000000000000000, 0.9238795325112867385, 1.000000000000000000, 0.9238795325112867385, 1.000000000000000000, 0.9238795325112867385, 1.000000000000000000, 0.9238795325112867385, 1.000000000000000000, 0.9238795325112867385, 1.000000000000000000, 0.9238795325112867385, 1.000000000000000000, 0.9238795325112867385, 1.000000000000000000, 0.9238795325112867385, 1.000000000000000000, 0.9238795325112867385, 1.000000000000000000, 0.9238795325112867385, 1.000000000000000000, 0.9238795325112867385, 1.000000000000000000, 0.9238795325112867385, 1.000000000000000000, 0.9238795325112867385, 1.000000000000000000, 0.9238795325112867385, 1.000000000000000000, 0.9238795325112867385, 1.000000000000000000, 0.9238795325112867385, 1.000000000000000000, 0.9238795325112867385, 1.000000000000000000, 0.9238795325112867385, 1.000000000000000000, 0.9238795325112867385, 1.000000000000000000, 0.9238795325112867385, 1.000000000000000000, 0.9238795325112867385, 1.000000000000000000, 0.9238795325112867385, 1.000000000000000000, 0.9238795325112867385, 1.000000000000000000, 0.9238795325112867385, 1.000000000000000000, 0.9238795325112867385, 1.000000000000000000, 0.9238795325112867385, 1.000000000000000000, 0.9238795325112867385, 1.000000000000000000, 0.9238795325112867385, 1.000000000000000000, 0.9238795325112867385, 1.000000000000000000, 0.9238795325112867385, 1.000000000000000000, 0.9238795325112867385, 1.000000000000000000, 0.9238795325112867385, 1.000000000000000000, 0.9238795325112867385, 1.000000000000000000, 0.9238795325112867385, 1.000000000000000000, 0.9238795325112867385, 1.000000000000000000, 0.9238795325112867385, 1.000000000000000000, 0.9238795325112867385, 1.000000000000000000, 0.9238795325112867385, 1.000000000000000000, 0.9238795325112867385, 1.000000000000000000, 0.9238795325112867385, 1.000000000000000000, 0.9238795325112867385, 1.000000000000000000, 0.9238795325112867385, 1.000000000000000000, 0.9238795325112867385, 1.000000000000000000, 0.9238795325112867385, 1.000000000000000000, 0.9238795325112867385, 1.000000000000000000, 0.9238795325112867385, 1.000000000000000000, 0.9238795325112867385, 1.000000000000000000, 0.9238795325112867385, 1.000000000000000000, 0.9238795325112867385, 1.000000000000000000, 0.9238795325112867385, 1.000000000000000000, 0.9238795325112867385, 1.000000000000000000, 0.9238795325112867385, 1.000000000000000000, 0.9238795325112867385, 1.000000000000000000, 0.9238795325112867385, 1.000000000000000000, 0.9238795325112867385, 1.000000000000000000, 0.9238795325112867385, 1.000000000000000000, 0.9238795325112867385, 1.000000000000000000, 0.9238795325112867385, 1.000000000000000000, 0.9238795325112867385, 1.000000000000000000, 0.9238795325112867385, 1.000000000000000000, 0.9238795325112867385, 1.000000000000000000, 0.9238795325112867385, 1.000000000000000000, 0.9238795325112867385, 1.000000000000000000, 0.9238795325112867385, 1.000000000000000000, 0.9238795325112867385, 1.000000000000000000, 0.9238795325112867385, 1.000000000000000000, 0.9238795325112867385, 1.000000000000000000, 0.9238795325112867385, 1.000000000000000000, 0.9238795325112867385, 1.000000000000000000, 0.9238795325112867385, 1.000000000000000000, 0.9238795325112867385, 1.000000000000000000, 0.9238795325112867385, 1.000000000000000000, 0.9238795325112867385, 1.000000000000000000, 0.9238795325112867385, 1.000000000000000000, 0.9238795325112867385, 1.000000000000000000, 0.9238795325112867385, 1.000000000000000000, 0.9238795325112867385, 1.000000000000000000, 0.9238795325112867385, 1.000000000000000000, 0.9238795325112867385, 1.000000000000000000, 0.9238795325112867385, 1.000000000000000000, 0.9238795325112867385, 1.000000000000000000, 0.9238795325112867385, 1.000000000000000000, 0.9238795325112867385, 1.000000000000000000, 0.9238795325112867385, 1.000000000000000000, 0.9238795325112867385, 1.000000000000000000, 0.9238795325112867385, 1.000000000000000000, 0.9238795325112867385, 1.000000000000000000, 0.9238795325112867385, 1.000000000000000000, 0.9238795325112867385, 1.000000000000000000, 0.9238795325112867385, 1.000000000000000000, 0.9238795325112867385, 1.000000000000000000, 0.9238795325112867385, 1.000000000000000000, 0.9238795325112867385, 1.000000000000000000, 0.9238795325112867385, 1.000000000000000000, 0.9238795325112867385, 1.000000000000000000, 0.9238795325112867385, 1.000000000000000000, 0.9238795325112867385, 1.000000000000000000, 0.9238795325112867385, 1.000000000000000000, 0.9238795325112867385, 1.000000000000000000, 0.9238795325112867385, 1.000000000000000000),
 ( 1.000000000000000000, 0.9238795325112867385, 1.000000000000000000, 0.9238795325112867385, 1.000000000000000000, 0.9238795325112867385, 1.000000000000000000, 0.9238795325112867385, 1.000000000000000000, 0.9238795325112867385, 1.000000000000000000, 0.9238795325112867385, 1.000000000000000000, 0.9238795325112867385, 1.000000000000000000, 0.9238795325112867385, 1.000000000000000000, 0.9238795325112867385, 1.000000000000000000, 0.9238795325112867385, 1.000000000000000000, 0.9238795325112867385, 1.000000000000000000, 0.9238795325112867385, 1.000000000000000000, 0.9238795325112867385, 1.000000000000000000, 0.9238795325112867385, 1.000000000000000000, 0.9238795325112867385, 1.000000000000000000, 0.9238795325112867385, 1.000000000000000000, 0.9238795325112867385, 1.000000000000000000, 0.9238795325112867385, 1.000000000000000000, 0.9238795325112867385, 1.000000000000000000, 0.9238795325112867385, 1.000000000000000000, 0.9238795325112867385, 1.000000000000000000, 0.9238795325112867385, 1.000000000000000000, 0.9238795325112867385, 1.000000000000000000, 0.9238795325112867385, 1.000000000000000000, 0.9238795325112867385, 1.000000000000000000, 0.9238795325112867385, 1.000000000000000000, 0.9238795325112867385, 1.000000000000000000, 0.9238795325112867385, 1.000000000000000000, 0.9238795325112867385, 1.000000000000000000, 0.9238795325112867385, 1.000000000000000000, 0.9238795325112867385, 1.000000000000000000, 0.9238795325112867385, 1.000000000000000000, 0.9238795325112867385, 1.000000000000000000, 0.9238795325112867385, 1.000000000000000000, 0.9238795325112867385, 1.000000000000000000, 0.9238795325112867385, 1.000000000000000000, 0.9238795325112867385, 1.000000000000000000, 0.9238795325112867385, 1.000000000000000000, 0.9238795325112867385, 1.000000000000000000, 0.9238795325112867385, 1.000000000000000000, 0.9238795325112867385, 1.000000000000000000, 0.9238795325112867385, 1.000000000000000000, 0.9238795325112867385, 1.000000000000000000, 0.9238795325112867385, 1.000000000000000000, 0.9238795325112867385, 1.000000000000000000, 0.9238795325112867385, 1.000000000000000000, 0.9238795325112867385, 1.000000000000000000, 0.9238795325112867385, 1.000000000000000000, 0.9238795325112867385, 1.000000000000000000, 0.9238795325112867385, 1.000000000000000000, 0.9238795325112867385, 1.000000000000000000, 0.9238795325112867385, 1.000000000000000000, 0.9238795325112867385, 1.000000000000000000, 0.9238795325112867385, 1.000000000000000000, 0.9238795325112867385, 1.000000000000000000, 0.9238795325112867385, 1.000000000000000000, 0.9238795325112867385, 1.000000000000000000, 0.9238795325112867385, 1.000000000000000000, 0.9238795325112867385, 1.000000000000000000, 0.9238795325112867385, 1.000000000000000000, 0.9238795325112867385, 1.000000000000000000, 0.9238795325112867385, 1.000000000000000000, 0.9238795325112867385, 1.000000000000000000, 0.9238795325112867385, 1.000000000000000000, 0.9238795325112867385, 1.000000000000000000, 0.9238795325112867385, 1.000000000000000000, 0.9238795325112867385, 1.000000000000000000, 0.9238795325112867385, 1.000000000000000000, 0.9238795325112867385, 1.000000000000000000, 0.9238795325112867385, 1.000000000000000000, 0.9238795325112867385, 1.000000000000000000, 0.9238795325112867385, 1.000000000000000000, 0.9238795325112867385, 1.000000000000000000, 0.9238795325112867385, 1.000000000000000000, 0.9238795325112867385, 1.000000000000000000, 0.9238795325112867385, 1.000000000000000000, 0.9238795325112867385, 1.000000000000000000, 0.9238795325112867385, 1.000000000000000000, 0.9238795325112867385, 1.000000000000000000, 0.9238795325112867385, 1.000000000000000000, 0.9238795325112867385, 1.000000000000000000, 0.9238795325112867385, 1.000000000000000000, 0.9238795325112867385, 1.000000000000000000, 0.9238795325112867385, 1.000000000000000000, 0.9238795325112867385, 1.000000000000000000, 0.9238795325112867385, 1.000000000000000000, 0.9238795325112867385, 1.000000000000000000, 0.9238795325112867385, 1.000000000000000000, 0.9238795325112867385, 1.000000000000000000, 0.9238795325112867385, 1.000000000000000000, 0.9238795325112867385, 1.000000000000000000, 0.9238795325112867385, 1.000000000000000000, 0.9238795325112867385, 1.000000000000000000, 0.9238795325112867385, 1.000000000000000000, 0.9238795325112867385, 1.000000000000000000, 0.9238795325112867385, 1.000000000000000000, 0.9238795325112867385, 1.000000000000000000, 0.9238795325112867385, 1.000000000000000000, 0.9238795325112867385, 1.000000000000000000, 0.9238795325112867385, 1.000000000000000000, 0.9238795325112867385, 1.000000000000000000, 0.9238795325112867385, 1.000000000000000000, 0.9238795325112867385, 1.000000000000000000, 0.9238795325112867385, 1.000000000000000000, 0.9238795325112867385, 1.000000000000000000, 0.9238795325112867385, 1.000000000000000000, 0.9238795325112867385, 1.000000000000000000, 0.9238795325112867385, 1.000000000000000000, 0.9238795325112867385, 1.000000000000000000, 0.9238795325112867385, 1.000000000000000000, 0.9238795325112867385, 1.000000000000000000, 0.9238795325112867385, 1.000000000000000000, 0.9238795325112867385, 1.000000000000000000, 0.9238795325112867385, 1.000000000000000000, 0.9238795325112867385, 1.000000000000000000, 0.9238795325112867385, 1.000000000000000000, 0.9238795325112867385, 1.000000000000000000, 0.9238795325112867385, 1.000000000000000000, 0.9238795325112867385, 1.000000000000000000, 0.9238795325112867385, 1.000000000000000000, 0.9238795325112867385, 1.000000000000000000, 0.9238795325112867385, 1.000000000000000000, 0.9238795325112867385, 1.000000000000000000, 0.9238795325112867385, 1.000000000000000000, 0.9238795325112867385, 1.000000000000000000, 0.9238795325112867385, 1.000000000000000000, 0.9238795325112867385, 1.000000000000000000, 0.9238795325112867385, 1.000000000000000000, 0.9238795325112867385, 1.000000000000000000, 0.9238795325112867385, 1.000000000000000000, 0.9238795325112867385, 1.000000000000000000, 0.9238795325112867385, 1.000000000000000000, 0.9238795325112867385, 1.000000000000000000, 0.9238795325112867385, 1.000000000000000000, 0.9238795325112867385, 1.000000000000000000, 0.9238795325112867385, 1.000000000000000000, 0.9238795325112867385, 1.000000000000000000, 0.9238795325112867385, 1.000000000000000000, 0.9238795325112867385, 1.000000000000000000, 0.9238795325112867385, 1.000000000000000000, 0.9238795325112867385, 1.000000000000000000, 0.9238795325112867385, 1.000000000000000000, 0.9238795325112867385, 1.000000000000000000, 0.9238795325112867385, 1.000000000000000000, 0.9238795325112867385, 1.000000000000000000, 0.9238795325112867385, 1.000000000000000000, 0.9238795325112867385, 1.000000000000000000, 0.9238795325112867385, 1.000000000000000000, 0.9238795325112867385, 1.000000000000000000, 0.9238795325112867385, 1.000000000000000000, 0.9238795325112867385, 1.000000000000000000, 0.9238795325112867385, 1.000000000000000000, 0.9238795325112867385, 1.000000000000000000, 0.9238795325112867385, 1.000000000000000000, 0.9238795325112867385, 1.000000000000000000, 0.9238795325112867385, 1.000000000000000000, 0.9238795325112867385, 1.000000000000000000, 0.9238795325112867385, 1.000000000000000000, 0.9238795325112867385, 1.000000000000000000, 0.9238795325112867385, 1.000000000000000000, 0.9238795325112867385, 1.000000000000000000, 0.9238795325112867385, 1.000000000000000000, 0.9238795325112867385, 1.000000000000000000, 0.9238795325112867385, 1.000000000000000000, 0.9238795325112867385, 1.000000000000000000, 0.9238795325112867385, 1.000000000000000000, 0.9238795325112867385, 1.000000000000000000, 0.9238795325112867385, 1.000000000000000000, 0.9238795325112867385, 1.000000000000000000, 0.9238795325112867385, 1.000000000000000000, 0.9238795325112867385, 1.000000000000000000, 0.9238795325112867385, 1.000000000000000000, 0.9238795325112867385, 1.000000000000000000, 0.9238795325112867385, 1.000000000000000000, 0.9238795325112867385, 1.000000000000000000, 0.9238795325112867385, 1.000000000000000000, 0.9238795325112867385, 1.000000000000000000, 0.9238795325112867385, 1.000000000000000000, 0.9238795325112867385, 1.000000000000000000, 0.9238795325112867385, 1.000000000000000000, 0.9238795325112867385, 1.000000000000000000, 0.9238795325112867385, 1.000000000000000000, 0.9238795325112867385, 1.000000000000000000, 0.9238795325112867385, 1.000000000000000000, 0.9238795325112867385, 1.000000000000000000, 0.9238795325112867385, 1.000000000000000000, 0.9238795325112867385, 1.000000000000000000, 0.9238795325112867385, 1.000000000000000000, 0.9238795325112867385, 1.000000000000000000, 0.9238795325112867385, 1.000000000000000000, 0.9238795325112867385, 1.000000000000000000, 0.9238795325112867385, 1.000000000000000000, 0.9238795325112867385, 1.000000000000000000, 0.9238795325112867385, 1.000000000000000000, 0.9238795325112867385, 1.000000000000000000, 0.9238795325112867385, 1.000000000000000000, 0.9238795325112867385, 1.000000000000000000, 0.9238795325112867385, 1.000000000000000000, 0.9238795325112867385, 1.000000000000000000, 0.9238795325112867385, 1.000000000000000000, 0.9238795325112867385, 1.000000000000000000, 0.9238795325112867385, 1.000000000000000000, 0.9238795325112867385, 1.000000000000000000, 0.9238795325112867385, 1.000000000000000000, 0.9238795325112867385, 1.000000000000000000, 0.9238795325112867385, 1.000000000000000000, 0.9238795325112867385, 1.000000000000000000, 0.9238795325112867385, 1.000000000000000000, 0.9238795325112867385, 1.000000000000000000, 0.9238795325112867385, 1.000000000000000000, 0.9238795325112867385, 1.000000000000000000, 0.9238795325112867385, 1.000000000000000000, 0.9238795325112867385, 1.000000000000000000, 0.9238795325112867385, 1.000000000000000000, 0.9238795325112867385, 1.000000000000000000, 0.9238795325112867385, 1.000000000000000000, 0.9238795325112867385, 1.000000000000000000, 0.9238795325112867385, 1.000000000000000000, 0.9238795325112867385, 1.000000000000000000, 0.9238795325112867385, 1.000000000000000000, 0.9238795325112867385, 1.000000000000000000, 0.9238795325112867385, 1.000000000000000000, 0.9238795325112867385, 1.000000000000000000, 0.9238795325112867385, 1.000000000000000000, 0.9238795325112867385, 1.000000000000000000, 0.9238795325112867385, 1.000000000000000000, 0.9238795325112867385, 1.000000000000000000, 0.9238795325112867385, 1.000000000000000000, 0.9238795325112867385, 1.000000000000000000, 0.9238795325112867385, 1.000000000000000000, 0.9238795325112867385, 1.000000000000000000, 0.9238795325112867385, 1.000000000000000000, 0.9238795325112867385, 1.000000000000000000, 0.9238795325112867385, 1.000000000000000000, 0.9238795325112867385, 1.000000000000000000, 0.9238795325112867385, 1.000000000000000000, 0.9238795325112867385, 1.000000000000000000, 0.9238795325112867385, 1.000000000000000000, 0.9238795325112867385, 1.000000000000000000, 0.9238795325112867385, 1.000000000000000000) ) ) 
 REPRESENTATION_ITEM ( '' )  SURFACE ( )  );
#33645=ORIENTED_EDGE ( 'NONE', *, *, #2713, .F. ) ;
#33648=CARTESIAN_POINT ( 'NONE',  ( 3.535533905932736864, -167.2500000027312126, 3.535533905932738641 ) ) ;
#33650=AXIS2_PLACEMENT_3D ( 'NONE', #17617, #18556, #3455 ) ;
#33659=CARTESIAN_POINT ( 'NONE',  ( -4.458734124999999437, -15.31249999863440436, 0.000000000000000000 ) ) ;
#33660=CARTESIAN_POINT ( 'NONE',  ( 5.000000000000000000, -71.50000000000000000, -6.123233995736766282E-16 ) ) ;
#33661=ORIENTED_EDGE ( 'NONE', *, *, #30819, .F. ) ;
#33662=CARTESIAN_POINT ( 'NONE',  ( -4.458734124999999437, -43.56249999863440081, 0.000000000000000000 ) ) ;
#33667=CARTESIAN_POINT ( 'NONE',  ( -2.229367062499996610, 10.85416666803225993, 3.861377020970582219 ) ) ;
#33669=CARTESIAN_POINT ( 'NONE',  ( -2.500000000000000444, 11.83333333333333037, -4.330127018922193649 ) ) ;
#33672=CARTESIAN_POINT ( 'NONE',  ( 5.000000000000000000, 14.62500000273118594, -6.123233995736766282E-16 ) ) ;
#33675=ORIENTED_EDGE ( 'NONE', *, *, #4797, .F. ) ;
#33678=CARTESIAN_POINT ( 'NONE',  ( 2.499999999999998668, -28.33333333333333570, -4.330127018922193649 ) ) ;
#33679=CARTESIAN_POINT ( 'NONE',  ( -2.229367062499996610, -31.14583333196773651, 3.861377020970582219 ) ) ;
#33681=CARTESIAN_POINT ( 'NONE',  ( 1.060575238724906964E-15, -33.62499999726880873, 5.773502691896257311 ) ) ;
#33682=CARTESIAN_POINT ( 'NONE',  ( 9.457646018065525792E-16, -66.06249999863440792, 5.148502694627439702 ) ) ;
#33685=CARTESIAN_POINT ( 'NONE',  ( -2.229367062499996610, -14.39583333196774184, 3.861377020970582219 ) ) ;
#33686=VERTEX_POINT ( 'NONE', #11305 ) ;
#33687=CARTESIAN_POINT ( 'NONE',  ( 5.000000000000000000, -75.50000000000000000, -6.123233995736766282E-16 ) ) ;
#33691=( BOUNDED_CURVE ( )  B_SPLINE_CURVE ( 2, ( #58395, #49371, #49044, #4667, #38757, #20430, #497, #14323, #14633 ),
 .UNSPECIFIED., .F., .F. ) 
 B_SPLINE_CURVE_WITH_KNOTS ( ( 3, 2, 2, 2, 3 ),
 ( 0.7562499999999999778, 0.7569444444444444198, 0.7583333333333333037, 0.7597222222222221877, 0.7604166666666666297 ),
 .UNSPECIFIED. ) 
 CURVE ( )  GEOMETRIC_REPRESENTATION_ITEM ( )  RATIONAL_B_SPLINE_CURVE ( ( 0.9330127018922194093, 0.9330127018922194093, 1.000000000000000000, 0.8660254037844387076, 1.000000000000000000, 0.8660254037844387076, 1.000000000000000000, 0.9330127018922194093, 0.9330127018922194093 ) ) 
 REPRESENTATION_ITEM ( '' )  );
#33692=CARTESIAN_POINT ( 'NONE',  ( 2.499999999999998668, -84.20833333060214443, -4.330127018922193649 ) ) ;
#33696=VECTOR ( 'NONE', #53358, 1000.000000000000000 ) ;
#33697=CARTESIAN_POINT ( 'NONE',  ( 4.458734125000001214, -22.14583333196773296, 2.574251347313718519 ) ) ;
#33698=CARTESIAN_POINT ( 'NONE',  ( 4.458734124999998549, -59.97916666530107221, -2.574251347313721627 ) ) ;
#33699=ORIENTED_EDGE ( 'NONE', *, *, #34579, .F. ) ;
#33700=CARTESIAN_POINT ( 'NONE',  ( 1.846868145590736310, -164.8750000013655779, 4.458734124999999437 ) ) ;
#33709=VECTOR ( 'NONE', #38690, 1000.000000000000000 ) ;
#33711=CARTESIAN_POINT ( 'NONE',  ( -8.190561711645485556E-16, -145.9375000013656063, 4.458734124999999437 ) ) ;
#33715=CARTESIAN_POINT ( 'NONE',  ( 4.458734125000001214, -68.14583333196773651, 2.574251347313718519 ) ) ;
#33717=CARTESIAN_POINT ( 'NONE',  ( -6.972266317189433020E-16, -4.249999999999997335, -5.000000000000000000 ) ) ;
#33718=CARTESIAN_POINT ( 'NONE',  ( 3.152801135295367541, -142.3125000013655779, -3.152801135295367541 ) ) ;
#33720=VERTEX_POINT ( 'NONE', #26425 ) ;
#33725=DIRECTION ( 'NONE',  ( -0.000000000000000000, 1.000000000000000000, -0.000000000000000000 ) ) ;
#33727=CARTESIAN_POINT ( 'NONE',  ( -3.152548672688508926E-16, 21.18750000136559208, -5.148502694627439702 ) ) ;
#33728=CYLINDRICAL_SURFACE ( 'NONE', #47929, 5.000000000000000000 ) ;
#33733=CARTESIAN_POINT ( 'NONE',  ( 5.000000000000000888, -80.58333333333332860, 2.886751345948126879 ) ) ;
#33734=CARTESIAN_POINT ( 'NONE',  ( 4.458734125000000326, 3.104166668032260379, 2.574251347313718519 ) ) ;
#33735=CARTESIAN_POINT ( 'NONE',  ( -3.152548672688508926E-16, -23.81249999863440792, -5.148502694627439702 ) ) ;
#33737=CARTESIAN_POINT ( 'NONE',  ( 2.730187237215162345E-16, -157.1875000013655779, -4.458734124999999437 ) ) ;
#33740=AXIS2_PLACEMENT_3D ( 'NONE', #2545, #26664, #42946 ) ;
#33744=CARTESIAN_POINT ( 'NONE',  ( -4.458734124999999437, -74.56249999863440792, 0.000000000000000000 ) ) ;
#33746=CARTESIAN_POINT ( 'NONE',  ( 2.499999999999998668, -73.33333333333332860, -4.330127018922193649 ) ) ;
#33747=CARTESIAN_POINT ( 'NONE',  ( 1.062108568985190270E-13, -11.12499999726881761, -4.999999999999999112 ) ) ;
#33748=ORIENTED_EDGE ( 'NONE', *, *, #21656, .T. ) ;
#33751=CARTESIAN_POINT ( 'NONE',  ( -2.499999999999996447, -10.83333333333333393, 4.330127018922195425 ) ) ;
#33752=CARTESIAN_POINT ( 'NONE',  ( -2.229367062500000163, -19.47916666530106866, -3.861377020970580443 ) ) ;
#33754=CARTESIAN_POINT ( 'NONE',  ( -3.152548672688508926E-16, -75.56249999863440792, -5.148502694627439702 ) ) ;
#33755=CARTESIAN_POINT ( 'NONE',  ( 3.152801135295367541, -168.5625000013656063, -3.152801135295367541 ) ) ;
#33756=CARTESIAN_POINT ( 'NONE',  ( -3.535250795749689387E-16, -19.12499999726881228, -5.773502691896257311 ) ) ;
#33757=CARTESIAN_POINT ( 'NONE',  ( 4.458734124999998549, -43.72916666530106511, -2.574251347313721627 ) ) ;
#33758=ORIENTED_EDGE ( 'NONE', *, *, #5250, .F. ) ;
#33760=CARTESIAN_POINT ( 'NONE',  ( 4.458734124999999437, 2.937500001365594304, -5.460374474430324690E-16 ) ) ;
#33763=CARTESIAN_POINT ( 'NONE',  ( -4.999999999999999112, -62.91666666666667140, 2.886751345948131764 ) ) ;
#33764=CARTESIAN_POINT ( 'NONE',  ( 2.730187237215162345E-16, -154.4375000013655779, -4.458734124999999437 ) ) ;
#33766=CARTESIAN_POINT ( 'NONE',  ( -1.339745962155613812, -79.20534180126146850, -5.000000000000000000 ) ) ;
#33767=CARTESIAN_POINT ( 'NONE',  ( 3.535533905932738197, -160.8750000000000284, -3.535533905932738197 ) ) ;
#33768=EDGE_CURVE ( 'NONE', #7216, #33686, #41100, .T. ) ;
#33769=CARTESIAN_POINT ( 'NONE',  ( -4.458734124999998549, -90.22916666530106511, 2.574251347313722516 ) ) ;
#33771=CARTESIAN_POINT ( 'NONE',  ( -2.229367062499996610, -7.395833331967735624, 3.861377020970582219 ) ) ;
#33772=CARTESIAN_POINT ( 'NONE',  ( -4.458734124999999437, -43.64583333196774362, -2.574251347313719407 ) ) ;
#33774=LINE ( 'NONE', #37345, #55259 ) ;
#33775=CARTESIAN_POINT ( 'NONE',  ( 4.458734124999999437, -147.4375000013656063, 0.000000000000000000 ) ) ;
#33779=ORIENTED_EDGE ( 'NONE', *, *, #31305, .T. ) ;
#33783=AXIS2_PLACEMENT_3D ( 'NONE', #48693, #49658, #24580 ) ;
#33785=VECTOR ( 'NONE', #27616, 1000.000000000000000 ) ;
#33786=VERTEX_POINT ( 'NONE', #6819 ) ;
#33787=FACE_OUTER_BOUND ( 'NONE', #8299, .T. ) ;
#33790=CARTESIAN_POINT ( 'NONE',  ( 4.458734124999999437, -3.812499998634408360, -5.460374474430324690E-16 ) ) ;
#33791=CARTESIAN_POINT ( 'NONE',  ( 2.500000000000002220, -30.54166666393548013, 4.330127018922192761 ) ) ;
#33792=CARTESIAN_POINT ( 'NONE',  ( 4.458734124999999437, -152.3750000013655779, -1.846868145590734978 ) ) ;
#33798=CARTESIAN_POINT ( 'NONE',  ( 0.000000000000000000, -170.0000000000000000, 0.000000000000000000 ) ) ;
#33799=CARTESIAN_POINT ( 'NONE',  ( -1.339745962155613812, -13.20534180126147916, -5.000000000000000000 ) ) ;
#33803=CARTESIAN_POINT ( 'NONE',  ( 0.000000000000000000, -170.0000000000000000, 5.000000000000000000 ) ) ;
#33807=CARTESIAN_POINT ( 'NONE',  ( -4.458734124999999437, 19.68750000136559208, 0.000000000000000000 ) ) ;
#33809=CARTESIAN_POINT ( 'NONE',  ( 9.457646018065525792E-16, -9.312499998634406140, 5.148502694627439702 ) ) ;
#33812=CARTESIAN_POINT ( 'NONE',  ( -3.152801135295367096, -166.0625000013656063, -3.152801135295367541 ) ) ;
#33819=CARTESIAN_POINT ( 'NONE',  ( -8.190561711645485556E-16, -152.9375000013655779, 4.458734124999999437 ) ) ;
#33820=( BOUNDED_CURVE ( )  B_SPLINE_CURVE ( 2, ( #32526, #37047, #27073, #56676, #52154, #32847, #56361, #52475, #51835 ),
 .UNSPECIFIED., .F., .F. ) 
 B_SPLINE_CURVE_WITH_KNOTS ( ( 3, 2, 2, 2, 3 ),
 ( 0.6083333333333329485, 0.6124999999999997113, 0.6166666666666663632, 0.6208333333333330151, 0.6249999999999996669 ),
 .UNSPECIFIED. ) 
 CURVE ( )  GEOMETRIC_REPRESENTATION_ITEM ( )  RATIONAL_B_SPLINE_CURVE ( ( 1.000000000000005995, 0.9238795325112806323, 1.000000000000000000, 0.9238795325112867385, 1.000000000000000000, 0.9238795325112867385, 1.000000000000000000, 0.9238795325112928447, 0.9999999999999938938 ) ) 
 REPRESENTATION_ITEM ( '' )  );
#33828=CARTESIAN_POINT ( 'NONE',  ( 2.071067811865391572, -161.8125000000000568, -5.000000000000086153 ) ) ;
#33829=CARTESIAN_POINT ( 'NONE',  ( -2.500000000000000444, 2.833333333333333481, -4.330127018922193649 ) ) ;
#33831=CARTESIAN_POINT ( 'NONE',  ( -4.458734124999997661, -62.22916666530105090, 2.574251347313722516 ) ) ;
#33835=CARTESIAN_POINT ( 'NONE',  ( -5.000000000000000000, -0.9583333306021485365, -2.886751345948128211 ) ) ;
#33836=CARTESIAN_POINT ( 'NONE',  ( 2.229367062499998831, -28.64583333196774007, -3.861377020970580887 ) ) ;
#33837=CARTESIAN_POINT ( 'NONE',  ( -2.500000000000000444, -48.04166666393547303, -4.330127018922193649 ) ) ;
#33839=CARTESIAN_POINT ( 'NONE',  ( 1.060575238724906964E-15, -45.75000000000000000, 5.773502691896257311 ) ) ;
#33843=CARTESIAN_POINT ( 'NONE',  ( -3.152548672688508926E-16, -69.56249999863439371, -5.148502694627439702 ) ) ;
#33844=CARTESIAN_POINT ( 'NONE',  ( 3.152801135295366208, -143.8125000013655779, 3.152801135295367985 ) ) ;
#33845=CARTESIAN_POINT ( 'NONE',  ( 9.457646018065525792E-16, -74.06249999863440792, 5.148502694627439702 ) ) ;
#33848=CARTESIAN_POINT ( 'NONE',  ( 9.457646018065525792E-16, -23.31249999863440436, 5.148502694627439702 ) ) ;
#33849=CARTESIAN_POINT ( 'NONE',  ( 2.499999999999998668, -67.20833333060214443, -4.330127018922193649 ) ) ;
#33852=EDGE_CURVE ( 'NONE', #19310, #54895, #56350, .T. ) ;
#33853=VERTEX_POINT ( 'NONE', #27691 ) ;
#33855=DIRECTION ( 'NONE',  ( -0.000000000000000000, 1.000000000000000000, -0.000000000000000000 ) ) ;
#33856=ORIENTED_EDGE ( 'NONE', *, *, #44875, .T. ) ;
#33857=CARTESIAN_POINT ( 'NONE',  ( -6.972266317189433020E-16, 16.74999999999999645, -5.000000000000000000 ) ) ;
#33858=CARTESIAN_POINT ( 'NONE',  ( -6.972266317189433020E-16, -83.24999999999998579, -5.000000000000000000 ) ) ;
#33859=CARTESIAN_POINT ( 'NONE',  ( -4.458734124999999437, -61.56249999863440081, 0.000000000000000000 ) ) ;
#33863=CARTESIAN_POINT ( 'NONE',  ( -5.000000000000000000, -22.95833333060214798, -2.886751345948128211 ) ) ;
#33864=CARTESIAN_POINT ( 'NONE',  ( 2.229367062499998831, 12.35416666803226171, -3.861377020970580887 ) ) ;
#33866=CARTESIAN_POINT ( 'NONE',  ( 5.000000000000000888, 20.54166666939784847, 2.886751345948126879 ) ) ;
#33867=CARTESIAN_POINT ( 'NONE',  ( -3.152801135295367985, -164.8125000013656063, 3.152801135295367096 ) ) ;
#33869=ORIENTED_EDGE ( 'NONE', *, *, #25268, .T. ) ;
#33871=CARTESIAN_POINT ( 'NONE',  ( -5.000000000000000000, -69.95833333060214443, -2.886751345948128211 ) ) ;
#33873=CYLINDRICAL_SURFACE ( 'NONE', #56216, 5.000000000000000000 ) ;
#33879=CARTESIAN_POINT ( 'NONE',  ( 3.061616997868383141E-16, -156.7500000000000000, -5.000000000000000000 ) ) ;
#33882=CARTESIAN_POINT ( 'NONE',  ( 4.458734124999999437, 7.937500001365595637, -5.460374474430324690E-16 ) ) ;
#33885=CARTESIAN_POINT ( 'NONE',  ( -2.071067811865478170, -150.4375000027312126, 5.000000000000000000 ) ) ;
#33886=CARTESIAN_POINT ( 'NONE',  ( 1.162044386198238837E-16, 29.25000000000000000, 5.000000000000000000 ) ) ;
#33890=CARTESIAN_POINT ( 'NONE',  ( 5.000000000000000000, -142.0625000000000000, 2.071067811865478614 ) ) ;
#33892=CARTESIAN_POINT ( 'NONE',  ( 1.846868145590735200, -166.5000000013655779, -4.458734124999999437 ) ) ;
#33893=CARTESIAN_POINT ( 'NONE',  ( 2.229367062499998831, -28.64583333196774007, -3.861377020970580887 ) ) ;
#33897=CARTESIAN_POINT ( 'NONE',  ( 1.846868145590735200, -145.2500000013655779, -4.458734125000000326 ) ) ;
#33898=ORIENTED_EDGE ( 'NONE', *, *, #23689, .F. ) ;
#33899=CARTESIAN_POINT ( 'NONE',  ( -4.458734124999998549, 27.52083333469892779, 2.574251347313722516 ) ) ;
#33901=CARTESIAN_POINT ( 'NONE',  ( 9.457646018065525792E-16, -54.31249999863440792, 5.148502694627439702 ) ) ;
#33903=CARTESIAN_POINT ( 'NONE',  ( 3.061616997868383141E-16, -162.7500000000000000, -5.000000000000000000 ) ) ;
#33904=CARTESIAN_POINT ( 'NONE',  ( 2.499999999999998668, 20.66666666666666785, -4.330127018922193649 ) ) ;
#33906=CARTESIAN_POINT ( 'NONE',  ( 9.457646018065525792E-16, -8.062499998634404363, 5.148502694627439702 ) ) ;
#33909=LINE ( 'NONE', #19747, #48151 ) ;
#33914=CARTESIAN_POINT ( 'NONE',  ( -4.458734124999999437, -52.39583333196773651, -2.574251347313719407 ) ) ;
#33915=CARTESIAN_POINT ( 'NONE',  ( -4.458734124999999437, -155.1875000013655779, -5.460374474430324690E-16 ) ) ;
#33917=CARTESIAN_POINT ( 'NONE',  ( -4.999999999999999112, -50.79166666393547303, 2.886751345948131764 ) ) ;
#33918=ORIENTED_EDGE ( 'NONE', *, *, #46424, .T. ) ;
#33919=CARTESIAN_POINT ( 'NONE',  ( 9.457646018065525792E-16, 4.687500001365596525, 5.148502694627439702 ) ) ;
#33920=ORIENTED_EDGE ( 'NONE', *, *, #18499, .T. ) ;
#33923=CARTESIAN_POINT ( 'NONE',  ( -3.152801135295367985, -159.8125000013656063, 3.152801135295367096 ) ) ;
#33925=VERTEX_POINT ( 'NONE', #18973 ) ;
#33927=EDGE_CURVE ( 'NONE', #3130, #13190, #33774, .T. ) ;
#33930=CARTESIAN_POINT ( 'NONE',  ( 1.975475456537005874E-15, -47.62499999726880873, 5.000000000000000000 ) ) ;
#33931=CARTESIAN_POINT ( 'NONE',  ( -4.458734124999998549, -43.47916666530106511, 2.574251347313722516 ) ) ;
#33933=EDGE_CURVE ( 'NONE', #733, #54901, #48562, .T. ) ;
#33938=CARTESIAN_POINT ( 'NONE',  ( -2.229367062500000163, -85.72916666530107932, -3.861377020970580443 ) ) ;
#33940=CARTESIAN_POINT ( 'NONE',  ( 1.339745962155615144, -35.58034179853028434, 4.999999999999999112 ) ) ;
#33942=CARTESIAN_POINT ( 'NONE',  ( 3.535533905932738197, -168.8750000000000284, -3.535533905932738197 ) ) ;
#33944=CARTESIAN_POINT ( 'NONE',  ( 0.000000000000000000, -170.0000000000000000, 0.000000000000000000 ) ) ;
#33948=CARTESIAN_POINT ( 'NONE',  ( -1.339745962155610925, -81.79465819873850307, 5.000000000000000000 ) ) ;
#33951=DIRECTION ( 'NONE',  ( -0.000000000000000000, 1.000000000000000000, -0.000000000000000000 ) ) ;
#33952=CYLINDRICAL_SURFACE ( 'NONE', #21424, 5.000000000000000000 ) ;
#33953=CARTESIAN_POINT ( 'NONE',  ( 4.458734124999999437, -86.06249999863439371, -5.460374474430324690E-16 ) ) ;
#33957=CARTESIAN_POINT ( 'NONE',  ( -5.000000000000000888, -155.5625000027311842, 2.071067811865474617 ) ) ;
#33959=CARTESIAN_POINT ( 'NONE',  ( 5.000000000000000888, -163.0625000027311842, -2.071067811865475505 ) ) ;
#33961=CARTESIAN_POINT ( 'NONE',  ( -5.000000000000000000, 21.91666666666666785, -2.886751345948128211 ) ) ;
#33963=CARTESIAN_POINT ( 'NONE',  ( -5.000000000000000000, -30.08333333333332860, -2.886751345948128211 ) ) ;
#33970=CARTESIAN_POINT ( 'NONE',  ( -2.500000000000000444, -20.16666666666666430, -4.330127018922193649 ) ) ;
#33971=CARTESIAN_POINT ( 'NONE',  ( -4.458734124999999437, -16.31249999863440436, 0.000000000000000000 ) ) ;
#33973=CARTESIAN_POINT ( 'NONE',  ( 3.535533905932738197, -156.8750000000000284, -3.535533905932738197 ) ) ;
#33975=CARTESIAN_POINT ( 'NONE',  ( -2.229367062499996610, -40.39583333196773651, 3.861377020970582219 ) ) ;
#33976=DIRECTION ( 'NONE',  ( -0.000000000000000000, 1.000000000000000000, -0.000000000000000000 ) ) ;
#33981=CARTESIAN_POINT ( 'NONE',  ( 4.458734124999999437, 8.187500001365595637, -5.460374474430324690E-16 ) ) ;
#33982=EDGE_CURVE ( 'NONE', #15736, #41952, #30009, .T. ) ;
#33984=CYLINDRICAL_SURFACE ( 'NONE', #3994, 5.000000000000000000 ) ;
#33986=CARTESIAN_POINT ( 'NONE',  ( -3.152548672688508926E-16, 18.18750000136559564, -5.148502694627439702 ) ) ;
#33988=CARTESIAN_POINT ( 'NONE',  ( -3.535250795749689387E-16, 15.87500000273118417, -5.773502691896257311 ) ) ;
#33992=FACE_OUTER_BOUND ( 'NONE', #10877, .T. ) ;
#33993=CARTESIAN_POINT ( 'NONE',  ( 5.000000000000000888, -32.58333333333333570, 2.886751345948126879 ) ) ;
#33994=CARTESIAN_POINT ( 'NONE',  ( 2.229367062499998831, -37.64583333196773651, -3.861377020970580887 ) ) ;
#33995=CARTESIAN_POINT ( 'NONE',  ( -5.000000000000000000, -36.87499999726881583, 0.000000000000000000 ) ) ;
#33996=CARTESIAN_POINT ( 'NONE',  ( -4.458734124999999437, -64.31249999863440792, 0.000000000000000000 ) ) ;
#33999=CARTESIAN_POINT ( 'NONE',  ( -2.229367062499996610, -13.14583333196774007, 3.861377020970582219 ) ) ;
#34000=CARTESIAN_POINT ( 'NONE',  ( 2.229367062500001939, -16.22916666530107577, 3.861377020970579999 ) ) ;
#34002=CARTESIAN_POINT ( 'NONE',  ( 2.500000000000002220, -76.66666666666665719, 4.330127018922192761 ) ) ;
#34005=CARTESIAN_POINT ( 'NONE',  ( 2.500000000000002220, -84.54166666393547303, 4.330127018922192761 ) ) ;
#34007=ORIENTED_EDGE ( 'NONE', *, *, #28709, .F. ) ;
#34009=CARTESIAN_POINT ( 'NONE',  ( 4.458734125000001214, -27.14583333196774717, 2.574251347313718519 ) ) ;
#34011=CARTESIAN_POINT ( 'NONE',  ( -4.458734124999999437, -167.1875000013655779, -5.460374474430324690E-16 ) ) ;
#34013=CARTESIAN_POINT ( 'NONE',  ( 5.000000000000000888, -50.45833333060213732, 2.886751345948126879 ) ) ;
#34014=VERTEX_POINT ( 'NONE', #39855 ) ;
#34024=CARTESIAN_POINT ( 'NONE',  ( -3.152801135295367096, -142.3125000013655779, -3.152801135295367541 ) ) ;
#34026=CARTESIAN_POINT ( 'NONE',  ( 1.339745962155612702, -70.29465819873850307, -5.000000000000000000 ) ) ;
#34028=CARTESIAN_POINT ( 'NONE',  ( 4.458734125000001214, -66.14583333196772230, 2.574251347313718519 ) ) ;
#34031=CARTESIAN_POINT ( 'NONE',  ( 3.152801135295367541, -140.3125000013655779, -3.152801135295367541 ) ) ;
#34040=CARTESIAN_POINT ( 'NONE',  ( -2.229367062500000163, 23.27083333469892779, -3.861377020970580443 ) ) ;
#34041=CARTESIAN_POINT ( 'NONE',  ( -6.972266317189433020E-16, -56.25000000000000000, -5.000000000000000000 ) ) ;
#34047=CARTESIAN_POINT ( 'NONE',  ( 4.458734124999999437, 3.187500001365594304, -5.460374474430324690E-16 ) ) ;
#34048=CARTESIAN_POINT ( 'NONE',  ( 4.458734125000000326, -23.14583333196772941, 2.574251347313718519 ) ) ;
#34049=( BOUNDED_CURVE ( )  B_SPLINE_CURVE ( 2, ( #19990, #19671, #14522, #28687, #38349, #9697, #43790, #24504, #19352 ),
 .UNSPECIFIED., .F., .F. ) 
 B_SPLINE_CURVE_WITH_KNOTS ( ( 3, 2, 2, 2, 3 ),
 ( 0.09375000000000000000, 0.09444444444444444198, 0.09583333333333333981, 0.09722222222222222376, 0.09791666666666666574 ),
 .UNSPECIFIED. ) 
 CURVE ( )  GEOMETRIC_REPRESENTATION_ITEM ( )  RATIONAL_B_SPLINE_CURVE ( ( 0.9330127018922194093, 0.9330127018922194093, 1.000000000000000000, 0.8660254037844387076, 1.000000000000000000, 0.8660254037844387076, 1.000000000000000000, 0.9330127018922194093, 0.9330127018922194093 ) ) 
 REPRESENTATION_ITEM ( '' )  );
#34053=CARTESIAN_POINT ( 'NONE',  ( 4.458734125000001214, 26.10416666803225993, 2.574251347313718519 ) ) ;
#34056=CARTESIAN_POINT ( 'NONE',  ( 4.458734124999998549, -73.97916666530106511, -2.574251347313721627 ) ) ;
#34059=CARTESIAN_POINT ( 'NONE',  ( -4.999999999999999112, 28.20833333606451632, 2.886751345948131764 ) ) ;
#34062=CARTESIAN_POINT ( 'NONE',  ( 1.975475456537005874E-15, -6.624999997268813168, 5.000000000000000000 ) ) ;
#34063=CARTESIAN_POINT ( 'NONE',  ( -5.000000000000000000, -16.00000000000000000, 0.000000000000000000 ) ) ;
#34064=CARTESIAN_POINT ( 'NONE',  ( 2.229367062499998831, -24.64583333196773651, -3.861377020970580887 ) ) ;
#34065=CARTESIAN_POINT ( 'NONE',  ( 4.458734125000000326, -83.89583333196773651, 2.574251347313718519 ) ) ;
#34066=CARTESIAN_POINT ( 'NONE',  ( -4.458734125000000326, -168.2500000013656063, -1.846868145590735644 ) ) ;
#34067=CARTESIAN_POINT ( 'NONE',  ( 2.499999999999998668, -16.20833333060214443, -4.330127018922193649 ) ) ;
#34068=CARTESIAN_POINT ( 'NONE',  ( -2.229367062500000163, -52.47916666530107221, -3.861377020970580443 ) ) ;
#34071=CARTESIAN_POINT ( 'NONE',  ( 1.975475456537005874E-15, -27.62499999726881228, 5.000000000000000000 ) ) ;
#34072=CARTESIAN_POINT ( 'NONE',  ( 2.229367062499998831, 1.104166668032261711, -3.861377020970580887 ) ) ;
#34075=CARTESIAN_POINT ( 'NONE',  ( 5.000000000000000000, -59.50000000000000000, -6.123233995736766282E-16 ) ) ;
#34076=CARTESIAN_POINT ( 'NONE',  ( 1.846868145590735200, -157.5000000013656063, -4.458734125000000326 ) ) ;
#34079=CARTESIAN_POINT ( 'NONE',  ( -5.000000000000000888, -163.5625000000000284, -2.071067811865475949 ) ) ;
#34082=CARTESIAN_POINT ( 'NONE',  ( 4.458734124999998549, -6.979166665301073103, -2.574251347313721627 ) ) ;
#34083=CARTESIAN_POINT ( 'NONE',  ( 9.457646018065525792E-16, -48.31249999863440081, 5.148502694627439702 ) ) ;
#34085=CARTESIAN_POINT ( 'NONE',  ( -1.846868145590734756, -149.1250000013656063, -4.458734125000000326 ) ) ;
#34087=ORIENTED_EDGE ( 'NONE', *, *, #2066, .T. ) ;
#34089=CARTESIAN_POINT ( 'NONE',  ( 1.975475456537005874E-15, 11.37500000273118239, 5.000000000000000000 ) ) ;
#34093=CYLINDRICAL_SURFACE ( 'NONE', #6179, 5.000000000000000000 ) ;
#34095=CARTESIAN_POINT ( 'NONE',  ( 1.975475456537005874E-15, -50.75000000000000000, 5.000000000000000000 ) ) ;
#34096=CARTESIAN_POINT ( 'NONE',  ( 4.458734124999998549, -2.729166665301069550, -2.574251347313721627 ) ) ;
#34098=CARTESIAN_POINT ( 'NONE',  ( 1.846868145590736310, -153.6250000013655779, 4.458734124999997661 ) ) ;
#34100=ORIENTED_EDGE ( 'NONE', *, *, #6641, .T. ) ;
#34110=CARTESIAN_POINT ( 'NONE',  ( 0.000000000000000000, -170.0000000000000000, 5.000000000000000000 ) ) ;
#34113=VECTOR ( 'NONE', #43923, 1000.000000000000000 ) ;
#34115=CARTESIAN_POINT ( 'NONE',  ( 4.458734124999999437, 18.18750000136559564, -5.460374474430324690E-16 ) ) ;
#34117=CARTESIAN_POINT ( 'NONE',  ( 4.458734124999999437, -7.062499998634404363, -5.460374474430324690E-16 ) ) ;
#34119=CARTESIAN_POINT ( 'NONE',  ( 1.846868145590736310, -166.6250000013656063, 4.458734124999999437 ) ) ;
#34126=CARTESIAN_POINT ( 'NONE',  ( 1.975475456537005874E-15, -69.74999999999998579, 5.000000000000000000 ) ) ;
#34128=CARTESIAN_POINT ( 'NONE',  ( -1.846868145590737420, -152.0000000013656063, 4.458734124999997661 ) ) ;
#34130=CARTESIAN_POINT ( 'NONE',  ( 1.339745962155612702, -46.29465819873851729, -5.000000000000000000 ) ) ;
#34131=CARTESIAN_POINT ( 'NONE',  ( 5.000000000000000888, -162.9375000000000000, -2.071067811865475505 ) ) ;
#34135=FACE_OUTER_BOUND ( 'NONE', #55005, .T. ) ;
#34136=CARTESIAN_POINT ( 'NONE',  ( -3.535250795749689387E-16, 4.750000000000000888, -5.773502691896257311 ) ) ;
#34137=ADVANCED_FACE ( 'NONE', ( #5456 ), #58846, .T. ) ;
#34138=CARTESIAN_POINT ( 'NONE',  ( 4.458734124999998549, -67.72916666530106511, -2.574251347313721627 ) ) ;
#34139=( BOUNDED_CURVE ( )  B_SPLINE_CURVE ( 2, ( #56351, #51518, #47003, #27064, #31242, #12581, #41844, #55709, #7456 ),
 .UNSPECIFIED., .F., .F. ) 
 B_SPLINE_CURVE_WITH_KNOTS ( ( 3, 2, 2, 2, 3 ),
 ( 0.8520833333333333037, 0.8527777777777777457, 0.8541666666666666297, 0.8555555555555555136, 0.8562499999999999556 ),
 .UNSPECIFIED. ) 
 CURVE ( )  GEOMETRIC_REPRESENTATION_ITEM ( )  RATIONAL_B_SPLINE_CURVE ( ( 0.9330127018922194093, 0.9330127018922194093, 1.000000000000000000, 0.8660254037844387076, 1.000000000000000000, 0.8660254037844387076, 1.000000000000000000, 0.9330127018922194093, 0.9330127018922194093 ) ) 
 REPRESENTATION_ITEM ( '' )  );
#34141=CARTESIAN_POINT ( 'NONE',  ( 5.000000000000000000, -3.291666663935477910, -2.886751345948129988 ) ) ;
#34142=CARTESIAN_POINT ( 'NONE',  ( 2.229367062499998831, -33.64583333196772941, -3.861377020970580887 ) ) ;
#34143=ORIENTED_EDGE ( 'NONE', *, *, #13457, .F. ) ;
#34146=CARTESIAN_POINT ( 'NONE',  ( 2.499999999999998668, -47.33333333333333570, -4.330127018922193649 ) ) ;
#34149=CARTESIAN_POINT ( 'NONE',  ( 1.339745962155612702, -4.169658196007335782, -5.000000000000000000 ) ) ;
#34150=CARTESIAN_POINT ( 'NONE',  ( 2.229367062499998831, -69.64583333196773651, -3.861377020970580887 ) ) ;
#34151=CARTESIAN_POINT ( 'NONE',  ( -8.190561711645485556E-16, -145.9375000013656063, 4.458734124999999437 ) ) ;
#34152=CARTESIAN_POINT ( 'NONE',  ( 4.458734125000001214, -76.89583333196775072, 2.574251347313718519 ) ) ;
#34154=CARTESIAN_POINT ( 'NONE',  ( 2.229367062500001939, -31.22916666530107221, 3.861377020970579999 ) ) ;
#34155=CARTESIAN_POINT ( 'NONE',  ( -4.999999999999999112, -68.79166666393547303, 2.886751345948131764 ) ) ;
#34156=VERTEX_POINT ( 'NONE', #9640 ) ;
#34157=EDGE_CURVE ( 'NONE', #50070, #328, #62535, .T. ) ;
#34159=ORIENTED_EDGE ( 'NONE', *, *, #22394, .F. ) ;
#34163=CARTESIAN_POINT ( 'NONE',  ( -1.339745962155613812, 16.79465819873852084, -5.000000000000000000 ) ) ;
#34164=CARTESIAN_POINT ( 'NONE',  ( -5.000000000000000000, -77.95833333060214443, -2.886751345948128211 ) ) ;
#34165=CARTESIAN_POINT ( 'NONE',  ( 9.457646018065525792E-16, -58.31249999863440792, 5.148502694627439702 ) ) ;
#34167=ORIENTED_EDGE ( 'NONE', *, *, #62612, .F. ) ;
#34168=CARTESIAN_POINT ( 'NONE',  ( 1.975475456537005874E-15, -67.74999999999998579, 5.000000000000000000 ) ) ;
#34170=CARTESIAN_POINT ( 'NONE',  ( 4.458734124999999437, 14.18750000136559386, -5.460374474430324690E-16 ) ) ;
#34172=CARTESIAN_POINT ( 'NONE',  ( -6.972266317189433020E-16, -32.24999999999999289, -5.000000000000000000 ) ) ;
#34173=CARTESIAN_POINT ( 'NONE',  ( -4.458734125000000326, -164.8750000013656063, 1.846868145590734089 ) ) ;
#34176=CARTESIAN_POINT ( 'NONE',  ( -2.071067811865686448, -153.6874999999999716, -4.999999999999789502 ) ) ;
#34179=ADVANCED_FACE ( 'NONE', ( #29569 ), #10282, .T. ) ;
#34180=CARTESIAN_POINT ( 'NONE',  ( -5.000000000000000888, -162.5625000027312126, 2.071067811865474617 ) ) ;
#34190=CARTESIAN_POINT ( 'NONE',  ( 9.457646018065525792E-16, 5.687500001365592972, 5.148502694627439702 ) ) ;
#34193=CARTESIAN_POINT ( 'NONE',  ( -9.184850993605147944E-16, -148.3750000027312126, 5.000000000000000000 ) ) ;
#34194=DIRECTION ( 'NONE',  ( -0.000000000000000000, 1.000000000000000000, -0.000000000000000000 ) ) ;
#34198=CARTESIAN_POINT ( 'NONE',  ( 3.061616997868383141E-16, -142.7500000000000284, -5.000000000000000000 ) ) ;
#34201=CARTESIAN_POINT ( 'NONE',  ( 3.152801135295367541, -167.5625000013656063, -3.152801135295367541 ) ) ;
#34202=CARTESIAN_POINT ( 'NONE',  ( 4.458734124999998549, -31.72916666530107577, -2.574251347313721627 ) ) ;
#34205=CARTESIAN_POINT ( 'NONE',  ( -8.190561711645485556E-16, -145.6875000013656063, 4.458734124999999437 ) ) ;
#34207=CARTESIAN_POINT ( 'NONE',  ( -5.000000000000000000, -89.87499999726880162, 0.000000000000000000 ) ) ;
#34208=CARTESIAN_POINT ( 'NONE',  ( -4.458734124999999437, -54.64583333196773651, -2.574251347313719407 ) ) ;
#34210=CARTESIAN_POINT ( 'NONE',  ( -5.000000000000000888, -162.5625000000000000, -2.071067811865475949 ) ) ;
#34211=CARTESIAN_POINT ( 'NONE',  ( 5.000000000000000000, 16.58333333333333215, -2.886751345948129988 ) ) ;
#34212=DIRECTION ( 'NONE',  ( -0.000000000000000000, 1.000000000000000000, -0.000000000000000000 ) ) ;
#34213=CARTESIAN_POINT ( 'NONE',  ( 4.458734124999999437, -3.812499998634408360, -5.460374474430324690E-16 ) ) ;
#34217=CYLINDRICAL_SURFACE ( 'NONE', #22284, 5.000000000000000000 ) ;
#34218=DIRECTION ( 'NONE',  ( -0.000000000000000000, 1.000000000000000000, -0.000000000000000000 ) ) ;
#34221=CARTESIAN_POINT ( 'NONE',  ( -4.458734124999998549, -56.22916666530107221, 2.574251347313722516 ) ) ;
#34222=CARTESIAN_POINT ( 'NONE',  ( -4.458734124999999437, -154.1875000013656063, -5.460374474430324690E-16 ) ) ;
#34223=CARTESIAN_POINT ( 'NONE',  ( 5.000000000000000000, -50.29166666393548013, -2.886751345948129988 ) ) ;
#34225=CARTESIAN_POINT ( 'NONE',  ( -4.458734124999999437, 3.437500001365594748, 0.000000000000000000 ) ) ;
#34226=EDGE_LOOP ( 'NONE', ( #56354, #55816, #16221, #29789 ) ) ;
#34227=CARTESIAN_POINT ( 'NONE',  ( 5.000000000000000000, -56.49999999999999289, -6.123233995736766282E-16 ) ) ;
#34228=CARTESIAN_POINT ( 'NONE',  ( 4.458734124999999437, -157.5000000013656063, 1.846868145590737864 ) ) ;
#34230=( BOUNDED_CURVE ( )  B_SPLINE_CURVE ( 2, ( #45766, #41556, #31924, #2661, #60574, #51552, #59941, #55428, #21328 ),
 .UNSPECIFIED., .F., .F. ) 
 B_SPLINE_CURVE_WITH_KNOTS ( ( 3, 2, 2, 2, 3 ),
 ( 0.3583333333333336146, 0.3625000000000002665, 0.3666666666666669183, 0.3708333333333336257, 0.3750000000000002776 ),
 .UNSPECIFIED. ) 
 CURVE ( )  GEOMETRIC_REPRESENTATION_ITEM ( )  RATIONAL_B_SPLINE_CURVE ( ( 0.9999999999999948930, 0.9238795325112918455, 1.000000000000000000, 0.9238795325112867385, 1.000000000000000000, 0.9238795325112867385, 1.000000000000000000, 0.9238795325112816315, 1.000000000000005107 ) ) 
 REPRESENTATION_ITEM ( '' )  );
#34234=CARTESIAN_POINT ( 'NONE',  ( 2.229367062500001939, -42.22916666530107932, 3.861377020970579999 ) ) ;
#34235=ORIENTED_EDGE ( 'NONE', *, *, #59690, .F. ) ;
#34237=CARTESIAN_POINT ( 'NONE',  ( -6.972266317189433020E-16, -46.24999999999999289, -5.000000000000000000 ) ) ;
#34239=LINE ( 'NONE', #5307, #47159 ) ;
#34241=CARTESIAN_POINT ( 'NONE',  ( -4.458734124999999437, 26.60416666803225993, -2.574251347313719407 ) ) ;
#34244=CARTESIAN_POINT ( 'NONE',  ( -2.500000000000000444, -7.166666666666668739, -4.330127018922193649 ) ) ;
#34249=CARTESIAN_POINT ( 'NONE',  ( -2.499999999999996447, 7.166666666666665186, 4.330127018922195425 ) ) ;
#34250=EDGE_CURVE ( 'NONE', #2012, #16047, #36601, .T. ) ;
#34254=FACE_OUTER_BOUND ( 'NONE', #35497, .T. ) ;
#34255=CARTESIAN_POINT ( 'NONE',  ( -4.999999999999998224, -19.79166666393548013, 2.886751345948131764 ) ) ;
#34261=CARTESIAN_POINT ( 'NONE',  ( -6.972266317189433020E-16, -17.12499999726881583, -5.000000000000000000 ) ) ;
#34263=CARTESIAN_POINT ( 'NONE',  ( 3.061616997868383141E-16, -160.8750000027311842, -5.000000000000000000 ) ) ;
#34276=CARTESIAN_POINT ( 'NONE',  ( 2.229367062500001939, -14.97916666530107399, 3.861377020970579999 ) ) ;
#34277=CARTESIAN_POINT ( 'NONE',  ( 0.000000000000000000, -170.0000000000000000, 0.000000000000000000 ) ) ;
#34278=CARTESIAN_POINT ( 'NONE',  ( -2.071067811865478170, -153.3125000000000000, 5.000000000000000000 ) ) ;
#34281=VERTEX_POINT ( 'NONE', #21535 ) ;
#34282=CARTESIAN_POINT ( 'NONE',  ( 4.458734124999998549, -41.97916666530107932, -2.574251347313721627 ) ) ;
#34284=EDGE_CURVE ( 'NONE', #32107, #41628, #38291, .T. ) ;
#34286=CARTESIAN_POINT ( 'NONE',  ( -5.000000000000000000, -90.87499999726880162, 0.000000000000000000 ) ) ;
#34290=CARTESIAN_POINT ( 'NONE',  ( 2.229367062500001939, 8.020833334698926009, 3.861377020970579999 ) ) ;
#34291=CARTESIAN_POINT ( 'NONE',  ( -2.499999999999996447, -43.83333333333333570, 4.330127018922195425 ) ) ;
#34292=CARTESIAN_POINT ( 'NONE',  ( -6.972266317189433020E-16, -37.12499999726881583, -5.000000000000000000 ) ) ;
#34293=CARTESIAN_POINT ( 'NONE',  ( -2.229367062500000163, -89.72916666530106511, -3.861377020970580443 ) ) ;
#34294=CARTESIAN_POINT ( 'NONE',  ( -4.458734124999999437, 23.43750000136559564, 0.000000000000000000 ) ) ;
#34296=CARTESIAN_POINT ( 'NONE',  ( -4.999999999999999112, 14.20833333606451809, 2.886751345948131764 ) ) ;
#34297=EDGE_LOOP ( 'NONE', ( #63313, #24656, #38440, #62596 ) ) ;
#34298=FACE_OUTER_BOUND ( 'NONE', #11703, .T. ) ;
#34299=ORIENTED_EDGE ( 'NONE', *, *, #44502, .F. ) ;
#34301=CARTESIAN_POINT ( 'NONE',  ( 2.499999999999998668, -35.33333333333332860, -4.330127018922193649 ) ) ;
#34302=CARTESIAN_POINT ( 'NONE',  ( -4.458734124999999437, -39.39583333196773651, -2.574251347313719407 ) ) ;
#34303=CARTESIAN_POINT ( 'NONE',  ( -3.535250795749689387E-16, -32.12499999726880873, -5.773502691896257311 ) ) ;
#34304=CARTESIAN_POINT ( 'NONE',  ( 4.458734124999998549, -63.72916666530107221, -2.574251347313721627 ) ) ;
#34307=CARTESIAN_POINT ( 'NONE',  ( 9.457646018065525792E-16, -15.06249999863440259, 5.148502694627439702 ) ) ;
#34308=CARTESIAN_POINT ( 'NONE',  ( -2.229367062499996610, -16.39583333196773651, 3.861377020970582219 ) ) ;
#34310=CARTESIAN_POINT ( 'NONE',  ( 5.000000000000000888, -80.58333333333332860, 2.886751345948126879 ) ) ;
#34311=CARTESIAN_POINT ( 'NONE',  ( 1.975475456537005874E-15, 1.375000002731185500, 5.000000000000000000 ) ) ;
#34313=CARTESIAN_POINT ( 'NONE',  ( 2.500000000000002220, -81.54166666393547303, 4.330127018922192761 ) ) ;
#34316=CARTESIAN_POINT ( 'NONE',  ( -2.229367062499996610, -26.39583333196774007, 3.861377020970582219 ) ) ;
#34317=VERTEX_POINT ( 'NONE', #58061 ) ;
#34320=CARTESIAN_POINT ( 'NONE',  ( -3.152801135295367985, -167.0625000013656063, 3.152801135295367096 ) ) ;
#34322=CARTESIAN_POINT ( 'NONE',  ( 1.339745962155612702, -55.16965819600732601, -5.000000000000000000 ) ) ;
#34323=ORIENTED_EDGE ( 'NONE', *, *, #48785, .T. ) ;
#34327=CARTESIAN_POINT ( 'NONE',  ( -3.152801135295367096, -147.3125000013655779, -3.152801135295367541 ) ) ;
#34328=CARTESIAN_POINT ( 'NONE',  ( -5.000000000000000000, 0.000000000000000000, 0.000000000000000000 ) ) ;
#34331=VERTEX_POINT ( 'NONE', #53553 ) ;
#34334=CARTESIAN_POINT ( 'NONE',  ( 4.458734125000000326, -143.6250000013656347, -1.846868145590734978 ) ) ;
#34337=LINE ( 'NONE', #8640, #51985 ) ;
#34339=CARTESIAN_POINT ( 'NONE',  ( -3.152548672688508926E-16, -73.81249999863440792, -5.148502694627439702 ) ) ;
#34340=CARTESIAN_POINT ( 'NONE',  ( 3.061616997868383141E-16, -144.8750000027312126, -5.000000000000000000 ) ) ;
#34341=LINE ( 'NONE', #38848, #37744 ) ;
#34342=CARTESIAN_POINT ( 'NONE',  ( 1.339745962155615144, -68.70534180126148271, 4.999999999999999112 ) ) ;
#34344=ORIENTED_EDGE ( 'NONE', *, *, #5515, .T. ) ;
#34349=CARTESIAN_POINT ( 'NONE',  ( 4.458734125000000326, 24.85416666803225993, 2.574251347313718519 ) ) ;
#34350=CARTESIAN_POINT ( 'NONE',  ( -2.499999999999996447, 23.29166666939785202, 4.330127018922195425 ) ) ;
#34355=CARTESIAN_POINT ( 'NONE',  ( 2.229367062500001939, 4.020833334698926009, 3.861377020970579999 ) ) ;
#34356=ORIENTED_EDGE ( 'NONE', *, *, #51074, .F. ) ;
#34357=CARTESIAN_POINT ( 'NONE',  ( -4.458734124999999437, -24.56249999863440436, 0.000000000000000000 ) ) ;
#34360=CARTESIAN_POINT ( 'NONE',  ( -3.152548672688508926E-16, 25.43750000136559208, -5.148502694627439702 ) ) ;
#34361=EDGE_CURVE ( 'NONE', #50557, #60346, #29627, .T. ) ;
#34364=CARTESIAN_POINT ( 'NONE',  ( -4.458734124999997661, -72.47916666530107932, 2.574251347313722516 ) ) ;
#34366=LINE ( 'NONE', #14435, #21313 ) ;
#34367=CARTESIAN_POINT ( 'NONE',  ( 0.000000000000000000, -170.0000000000000000, 0.000000000000000000 ) ) ;
#34369=CYLINDRICAL_SURFACE ( 'NONE', #33522, 5.000000000000000000 ) ;
#34370=CARTESIAN_POINT ( 'NONE',  ( 5.000000000000000000, 2.708333336064520314, -2.886751345948130876 ) ) ;
#34371=CARTESIAN_POINT ( 'NONE',  ( 1.060575238724906964E-15, -19.74999999999999645, 5.773502691896257311 ) ) ;
#34372=CARTESIAN_POINT ( 'NONE',  ( -3.152548672688508926E-16, -20.56249999863440081, -5.148502694627439702 ) ) ;
#34373=CARTESIAN_POINT ( 'NONE',  ( -2.229367062499996610, -82.14583333196773651, 3.861377020970582219 ) ) ;
#34375=CARTESIAN_POINT ( 'NONE',  ( -4.458734124999999437, -166.1875000013655779, -5.460374474430324690E-16 ) ) ;
#34376=CARTESIAN_POINT ( 'NONE',  ( 1.060575238724906964E-15, -16.62499999726881583, 5.773502691896257311 ) ) ;
#34377=CARTESIAN_POINT ( 'NONE',  ( -4.458734124999999437, -48.39583333196772941, -2.574251347313719407 ) ) ;
#34378=ORIENTED_EDGE ( 'NONE', *, *, #56762, .T. ) ;
#34381=CARTESIAN_POINT ( 'NONE',  ( -4.458734124999999437, -0.6458333319677399542, -2.574251347313719407 ) ) ;
#34384=CARTESIAN_POINT ( 'NONE',  ( 5.000000000000000888, -65.58333333333332860, 2.886751345948126879 ) ) ;
#34385=CARTESIAN_POINT ( 'NONE',  ( -3.152801135295367985, -156.0625000013656063, 3.152801135295367096 ) ) ;
#34388=( BOUNDED_CURVE ( )  B_SPLINE_CURVE ( 2, ( #42195, #37071, #27719, #36747, #8430, #23212, #2344, #61837, #17121 ),
 .UNSPECIFIED., .F., .F. ) 
 B_SPLINE_CURVE_WITH_KNOTS ( ( 3, 2, 2, 2, 3 ),
 ( 0.3354166666666666963, 0.3361111111111111382, 0.3375000000000000222, 0.3388888888888889062, 0.3395833333333333481 ),
 .UNSPECIFIED. ) 
 CURVE ( )  GEOMETRIC_REPRESENTATION_ITEM ( )  RATIONAL_B_SPLINE_CURVE ( ( 0.9330127018922194093, 0.9330127018922220739, 1.000000000000000000, 0.8660254037844387076, 1.000000000000000000, 0.8660254037844387076, 1.000000000000000000, 0.9330127018922194093, 0.9330127018922194093 ) ) 
 REPRESENTATION_ITEM ( '' )  );
#34389=CARTESIAN_POINT ( 'NONE',  ( -2.071067811865478170, -164.3125000000000000, 5.000000000000000000 ) ) ;
#34390=CARTESIAN_POINT ( 'NONE',  ( -4.999999999999998224, 7.208333336064517205, 2.886751345948131764 ) ) ;
#34392=CARTESIAN_POINT ( 'NONE',  ( -4.458734124999999437, -8.645833331967736513, -2.574251347313719407 ) ) ;
#34393=CARTESIAN_POINT ( 'NONE',  ( 2.229367062499998831, -43.89583333196774362, -3.861377020970580887 ) ) ;
#34394=CARTESIAN_POINT ( 'NONE',  ( -8.190561711645485556E-16, -146.6875000013656063, 4.458734124999999437 ) ) ;
#34398=CARTESIAN_POINT ( 'NONE',  ( 4.458734125000001214, 28.85416666803225993, 2.574251347313718519 ) ) ;
#34400=ORIENTED_EDGE ( 'NONE', *, *, #56758, .F. ) ;
#34404=CARTESIAN_POINT ( 'NONE',  ( -4.999999999999998224, 2.208333336064519870, 2.886751345948131764 ) ) ;
#34405=CARTESIAN_POINT ( 'NONE',  ( -4.458734124999998549, -3.229166665301069994, 2.574251347313722516 ) ) ;
#34406=CARTESIAN_POINT ( 'NONE',  ( -6.972266317189433020E-16, -73.12499999726878741, -5.000000000000000000 ) ) ;
#34407=CARTESIAN_POINT ( 'NONE',  ( -4.458734124999999437, -153.9375000013655779, -5.460374474430324690E-16 ) ) ;
#34414=CARTESIAN_POINT ( 'NONE',  ( 1.975475456537005874E-15, -49.74999999999999289, 5.000000000000000000 ) ) ;
#34415=CARTESIAN_POINT ( 'NONE',  ( 2.500000000000002220, 29.33333333333333215, 4.330127018922192761 ) ) ;
#34416=AXIS2_PLACEMENT_3D ( 'NONE', #49836, #60148, #45019 ) ;
#34423=CARTESIAN_POINT ( 'NONE',  ( -2.229367062499996610, 15.85416666803226171, 3.861377020970582219 ) ) ;
#34425=ORIENTED_EDGE ( 'NONE', *, *, #29931, .F. ) ;
#34426=CARTESIAN_POINT ( 'NONE',  ( -4.458734124999997661, -10.47916666530106866, 2.574251347313722516 ) ) ;
#34427=LINE ( 'NONE', #11196, #3178 ) ;
#34429=CARTESIAN_POINT ( 'NONE',  ( 3.152801135295366208, -168.5625000013656063, 3.152801135295367985 ) ) ;
#34430=CARTESIAN_POINT ( 'NONE',  ( -1.339745962155613812, -21.08034179853029144, -5.000000000000000000 ) ) ;
#34434=CARTESIAN_POINT ( 'NONE',  ( 1.339745962155612702, -38.29465819873851729, -5.000000000000000000 ) ) ;
#34437=CARTESIAN_POINT ( 'NONE',  ( 4.458734124999999437, -154.6875000013656063, 0.000000000000000000 ) ) ;
#34444=CARTESIAN_POINT ( 'NONE',  ( -4.999999999999998224, -87.79166666393547303, 2.886751345948131764 ) ) ;
#34445=CARTESIAN_POINT ( 'NONE',  ( -2.499999999999996447, 0.1666666666666656582, 4.330127018922195425 ) ) ;
#34446=CARTESIAN_POINT ( 'NONE',  ( -2.229367062500000163, -66.47916666530106511, -3.861377020970580443 ) ) ;
#34447=CARTESIAN_POINT ( 'NONE',  ( -4.729367062499999719, -90.15624999931721106, 0.000000000000000000 ) ) ;
#34448=CARTESIAN_POINT ( 'NONE',  ( -3.535250795749689387E-16, -3.124999997268815832, -5.773502691896257311 ) ) ;
#34449=CARTESIAN_POINT ( 'NONE',  ( 2.229367062500001939, -31.97916666530106866, 3.861377020970579999 ) ) ;
#34454=CARTESIAN_POINT ( 'NONE',  ( -4.999999999999999112, -48.91666666666666430, 2.886751345948131764 ) ) ;
#34457=CARTESIAN_POINT ( 'NONE',  ( 1.339745962155615144, -64.70534180126146850, 4.999999999999999112 ) ) ;
#34458=CARTESIAN_POINT ( 'NONE',  ( 4.458734124999998549, -68.72916666530106511, -2.574251347313721627 ) ) ;
#34459=CARTESIAN_POINT ( 'NONE',  ( -1.846868145590737420, -143.0000000013655779, 4.458734124999999437 ) ) ;
#34460=CARTESIAN_POINT ( 'NONE',  ( -4.458734124999998549, -81.22916666530106511, 2.574251347313722516 ) ) ;
#34463=CARTESIAN_POINT ( 'NONE',  ( -2.229367062500000163, -32.72916666530106511, -3.861377020970580443 ) ) ;
#34464=CARTESIAN_POINT ( 'NONE',  ( -5.000000000000000000, -69.95833333060214443, -2.886751345948128211 ) ) ;
#34465=VERTEX_POINT ( 'NONE', #29085 ) ;
#34466=ORIENTED_EDGE ( 'NONE', *, *, #43719, .F. ) ;
#34468=CARTESIAN_POINT ( 'NONE',  ( -6.972266317189433020E-16, -17.25000000000000000, -5.000000000000000000 ) ) ;
#34469=ORIENTED_EDGE ( 'NONE', *, *, #54759, .T. ) ;
#34472=CARTESIAN_POINT ( 'NONE',  ( -4.458734124999999437, -60.64583333196774362, -2.574251347313719407 ) ) ;
#34475=DIRECTION ( 'NONE',  ( -0.000000000000000000, 1.000000000000000000, -0.000000000000000000 ) ) ;
#34477=CARTESIAN_POINT ( 'NONE',  ( 2.229367062500001939, 15.02083333469892779, 3.861377020970579999 ) ) ;
#34479=CARTESIAN_POINT ( 'NONE',  ( -4.999999999999998224, -0.9166666666666664076, 2.886751345948131764 ) ) ;
#34480=CARTESIAN_POINT ( 'NONE',  ( 4.458734124999997661, -163.5000000013655779, 1.846868145590737864 ) ) ;
#34483=CARTESIAN_POINT ( 'NONE',  ( -6.972266317189433020E-16, -39.25000000000000000, -5.000000000000000000 ) ) ;
#34489=CARTESIAN_POINT ( 'NONE',  ( -4.999999999999998224, -72.79166666393548724, 2.886751345948131764 ) ) ;
#34491=CARTESIAN_POINT ( 'NONE',  ( 2.499999999999998668, -61.33333333333333570, -4.330127018922193649 ) ) ;
#34494=CARTESIAN_POINT ( 'NONE',  ( -4.458734124999999437, 8.437500001365595637, 0.000000000000000000 ) ) ;
#34498=CARTESIAN_POINT ( 'NONE',  ( 3.535533905932736864, -150.2500000027312126, 3.535533905932738641 ) ) ;
#34499=CARTESIAN_POINT ( 'NONE',  ( -5.000000000000000000, 28.99999999999999645, 0.000000000000000000 ) ) ;
#34505=( BOUNDED_CURVE ( )  B_SPLINE_CURVE ( 2, ( #1846, #2167, #41678, #17251, #52307, #36875, #32674, #12427, #7615 ),
 .UNSPECIFIED., .F., .F. ) 
 B_SPLINE_CURVE_WITH_KNOTS ( ( 3, 2, 2, 2, 3 ),
 ( 0.7083333333333329263, 0.7124999999999995781, 0.7166666666666663410, 0.7208333333333329929, 0.7249999999999996447 ),
 .UNSPECIFIED. ) 
 CURVE ( )  GEOMETRIC_REPRESENTATION_ITEM ( )  RATIONAL_B_SPLINE_CURVE ( ( 1.000000000000008216, 0.9238795325112786339, 1.000000000000000000, 0.9238795325112867385, 1.000000000000000000, 0.9238795325112867385, 1.000000000000000000, 0.9238795325112928447, 0.9999999999999938938 ) ) 
 REPRESENTATION_ITEM ( '' )  );
#34506=CARTESIAN_POINT ( 'NONE',  ( 3.535533905932738197, -142.8750000000000000, -3.535533905932738197 ) ) ;
#34509=CARTESIAN_POINT ( 'NONE',  ( 3.152801135295366208, -163.8125000013656063, 3.152801135295367985 ) ) ;
#34510=CARTESIAN_POINT ( 'NONE',  ( -2.229367062500000163, -36.47916666530107221, -3.861377020970580443 ) ) ;
#34511=FACE_OUTER_BOUND ( 'NONE', #33065, .T. ) ;
#34514=CARTESIAN_POINT ( 'NONE',  ( 3.152801135295366208, -144.5625000013655779, 3.152801135295367985 ) ) ;
#34516=CARTESIAN_POINT ( 'NONE',  ( 9.457646018065525792E-16, 28.68750000136559208, 5.148502694627439702 ) ) ;
#34518=CARTESIAN_POINT ( 'NONE',  ( 4.458734124999998549, -63.97916666530106511, -2.574251347313721627 ) ) ;
#34520=CARTESIAN_POINT ( 'NONE',  ( 5.000000000000000000, -90.37499999726880162, -6.123233995736766282E-16 ) ) ;
#34521=CARTESIAN_POINT ( 'NONE',  ( 1.060575238724906964E-15, 13.24999999999999822, 5.773502691896257311 ) ) ;
#34522=CARTESIAN_POINT ( 'NONE',  ( 2.229367062500001939, -51.97916666530107221, 3.861377020970579999 ) ) ;
#34523=CARTESIAN_POINT ( 'NONE',  ( 2.229367062500001939, -4.979166665301071326, 3.861377020970579999 ) ) ;
#34524=CARTESIAN_POINT ( 'NONE',  ( -5.000000000000000000, 4.125000002731186832, 0.000000000000000000 ) ) ;
#34530=CARTESIAN_POINT ( 'NONE',  ( -4.458734124999998549, -53.22916666530107932, 2.574251347313722516 ) ) ;
#34531=CARTESIAN_POINT ( 'NONE',  ( 4.458734124999999437, -157.6875000013655779, 0.000000000000000000 ) ) ;
#34532=ADVANCED_FACE ( 'NONE', ( #19769 ), #19449, .T. ) ;
#34533=CARTESIAN_POINT ( 'NONE',  ( -4.999999999999999112, -55.79166666393548013, 2.886751345948131764 ) ) ;
#34534=ORIENTED_EDGE ( 'NONE', *, *, #11766, .F. ) ;
#34536=CARTESIAN_POINT ( 'NONE',  ( -4.458734124999998549, 6.520833334698930450, 2.574251347313722516 ) ) ;
#34538=DIRECTION ( 'NONE',  ( -0.000000000000000000, 1.000000000000000000, -0.000000000000000000 ) ) ;
#34540=CARTESIAN_POINT ( 'NONE',  ( -3.152801135295367985, -156.8125000013656063, 3.152801135295367096 ) ) ;
#34541=ORIENTED_EDGE ( 'NONE', *, *, #16874, .T. ) ;
#34542=AXIS2_PLACEMENT_3D ( 'NONE', #23556, #63111, #14197 ) ;
#34543=EDGE_CURVE ( 'NONE', #36547, #16762, #32469, .T. ) ;
#34547=CARTESIAN_POINT ( 'NONE',  ( 2.229367062500001939, -41.22916666530107932, 3.861377020970579999 ) ) ;
#34550=AXIS2_PLACEMENT_3D ( 'NONE', #4156, #43064, #49149 ) ;
#34551=CARTESIAN_POINT ( 'NONE',  ( -3.535533905932737309, -145.6250000000000000, -3.535533905932738197 ) ) ;
#34552=EDGE_CURVE ( 'NONE', #44876, #24978, #14308, .T. ) ;
#34555=( BOUNDED_CURVE ( )  B_SPLINE_CURVE ( 2, ( #52147, #60853, #2320, #37348, #47005, #62119, #56667, #47321, #7458 ),
 .UNSPECIFIED., .F., .F. ) 
 B_SPLINE_CURVE_WITH_KNOTS ( ( 3, 2, 2, 2, 3 ),
 ( 0.9687500000000000000, 0.9694444444444444420, 0.9708333333333333259, 0.9722222222222222099, 0.9729166666666666519 ),
 .UNSPECIFIED. ) 
 CURVE ( )  GEOMETRIC_REPRESENTATION_ITEM ( )  RATIONAL_B_SPLINE_CURVE ( ( 0.9330127018922194093, 0.9330127018922194093, 1.000000000000000000, 0.8660254037844387076, 1.000000000000000000, 0.8660254037844387076, 1.000000000000000000, 0.9330127018922194093, 0.9330127018922194093 ) ) 
 REPRESENTATION_ITEM ( '' )  );
#34556=ORIENTED_EDGE ( 'NONE', *, *, #54679, .T. ) ;
#34557=CARTESIAN_POINT ( 'NONE',  ( -4.458734124999998549, 28.77083333469892779, 2.574251347313722516 ) ) ;
#34561=( BOUNDED_CURVE ( )  B_SPLINE_CURVE ( 2, ( #30655, #50278, #6223, #18853, #25835, #37087, #36762, #40933, #26152 ),
 .UNSPECIFIED., .F., .F. ) 
 B_SPLINE_CURVE_WITH_KNOTS ( ( 3, 2, 2, 2, 3 ),
 ( 0.2187500000000000000, 0.2194444444444444420, 0.2208333333333333259, 0.2222222222222222099, 0.2229166666666666796 ),
 .UNSPECIFIED. ) 
 CURVE ( )  GEOMETRIC_REPRESENTATION_ITEM ( )  RATIONAL_B_SPLINE_CURVE ( ( 0.9330127018922194093, 0.9330127018922194093, 1.000000000000000000, 0.8660254037844387076, 1.000000000000000000, 0.8660254037844387076, 1.000000000000000000, 0.9330127018922180770, 0.9330127018922194093 ) ) 
 REPRESENTATION_ITEM ( '' )  );
#34562=CARTESIAN_POINT ( 'NONE',  ( -6.972266317189433020E-16, 1.750000000000000444, -5.000000000000000000 ) ) ;
#34564=FACE_OUTER_BOUND ( 'NONE', #60741, .T. ) ;
#34571=CARTESIAN_POINT ( 'NONE',  ( -4.458734124999999437, -87.56249999863439371, 0.000000000000000000 ) ) ;
#34577=CARTESIAN_POINT ( 'NONE',  ( -9.184850993605147944E-16, -163.3750000027311842, 5.000000000000000000 ) ) ;
#34579=EDGE_CURVE ( 'NONE', #25841, #54515, #23079, .T. ) ;
#34587=( BOUNDED_CURVE ( )  B_SPLINE_CURVE ( 2, ( #41726, #14820, #10001, #50527, #688, #26078, #35410, #1652, #29614 ),
 .UNSPECIFIED., .F., .F. ) 
 B_SPLINE_CURVE_WITH_KNOTS ( ( 3, 2, 2, 2, 3 ),
 ( 0.8895833333333332815, 0.8902777777777777235, 0.8916666666666667185, 0.8930555555555556024, 0.8937500000000000444 ),
 .UNSPECIFIED. ) 
 CURVE ( )  GEOMETRIC_REPRESENTATION_ITEM ( )  RATIONAL_B_SPLINE_CURVE ( ( 0.9330127018922194093, 0.9330127018922194093, 1.000000000000000000, 0.8660254037844387076, 1.000000000000000000, 0.8660254037844387076, 1.000000000000000000, 0.9330127018922194093, 0.9330127018922194093 ) ) 
 REPRESENTATION_ITEM ( '' )  );
#34590=CARTESIAN_POINT ( 'NONE',  ( -3.152548672688508926E-16, -21.56249999863440792, -5.148502694627439702 ) ) ;
#34591=DIRECTION ( 'NONE',  ( 0.000000000000000000, 0.000000000000000000, -1.000000000000000000 ) ) ;
#34592=CARTESIAN_POINT ( 'NONE',  ( 3.061616997868383141E-16, -156.7500000000000000, -5.000000000000000000 ) ) ;
#34594=ORIENTED_EDGE ( 'NONE', *, *, #44166, .F. ) ;
#34595=CARTESIAN_POINT ( 'NONE',  ( 2.229367062499998831, -44.89583333196774362, -3.861377020970580887 ) ) ;
#34597=CARTESIAN_POINT ( 'NONE',  ( -4.999999999999998224, 26.08333333333332860, 2.886751345948131764 ) ) ;
#34599=CARTESIAN_POINT ( 'NONE',  ( -1.510657702057710340E-15, 27.37500000273118417, 5.000000000000000000 ) ) ;
#34602=AXIS2_PLACEMENT_3D ( 'NONE', #43776, #48294, #24489 ) ;
#34604=CARTESIAN_POINT ( 'NONE',  ( 4.458734124999998549, 9.270833334698927786, -2.574251347313721627 ) ) ;
#34606=AXIS2_PLACEMENT_3D ( 'NONE', #50112, #6067, #60100 ) ;
#34607=CARTESIAN_POINT ( 'NONE',  ( -1.339745962155610925, 12.20534180126148094, 5.000000000000000000 ) ) ;
#34608=CARTESIAN_POINT ( 'NONE',  ( -2.229367062499996610, -89.39583333196773651, 3.861377020970582219 ) ) ;
#34609=CARTESIAN_POINT ( 'NONE',  ( -4.458734124999998549, 19.52083333469893134, 2.574251347313722516 ) ) ;
#34611=CARTESIAN_POINT ( 'NONE',  ( -3.535250795749689387E-16, 9.875000002731184168, -5.773502691896257311 ) ) ;
#34612=VERTEX_POINT ( 'NONE', #32440 ) ;
#34614=ORIENTED_EDGE ( 'NONE', *, *, #22892, .T. ) ;
#34616=CARTESIAN_POINT ( 'NONE',  ( 0.000000000000000000, -170.0000000000000000, 0.000000000000000000 ) ) ;
#34617=CARTESIAN_POINT ( 'NONE',  ( -4.999999999999999112, -34.91666666666666430, 2.886751345948131764 ) ) ;
#34618=CARTESIAN_POINT ( 'NONE',  ( -4.458734124999999437, -37.39583333196773651, -2.574251347313719407 ) ) ;
#34620=CARTESIAN_POINT ( 'NONE',  ( -2.500000000000000444, -38.04166666393548013, -4.330127018922193649 ) ) ;
#34622=VERTEX_POINT ( 'NONE', #54513 ) ;
#34624=CARTESIAN_POINT ( 'NONE',  ( -2.229367062500000163, -13.47916666530107221, -3.861377020970580443 ) ) ;
#34625=CARTESIAN_POINT ( 'NONE',  ( -3.152548672688508926E-16, -16.81249999863440436, -5.148502694627439702 ) ) ;
#34627=EDGE_CURVE ( 'NONE', #60995, #45777, #16875, .T. ) ;
#34628=CARTESIAN_POINT ( 'NONE',  ( -3.535250795749689387E-16, -84.24999999999998579, -5.773502691896257311 ) ) ;
#34629=CARTESIAN_POINT ( 'NONE',  ( -1.846868145590737420, -166.7500000013655779, 4.458734124999999437 ) ) ;
#34631=CARTESIAN_POINT ( 'NONE',  ( -2.499999999999996447, -79.70833333060213022, 4.330127018922195425 ) ) ;
#34633=ORIENTED_EDGE ( 'NONE', *, *, #48085, .F. ) ;
#34635=CARTESIAN_POINT ( 'NONE',  ( -4.458734124999999437, -24.56249999863440436, 0.000000000000000000 ) ) ;
#34637=EDGE_CURVE ( 'NONE', #8866, #11945, #12370, .T. ) ;
#34638=ORIENTED_EDGE ( 'NONE', *, *, #4704, .T. ) ;
#34640=CARTESIAN_POINT ( 'NONE',  ( 1.846868145590736310, -163.8750000013655779, 4.458734124999999437 ) ) ;
#34643=CARTESIAN_POINT ( 'NONE',  ( 3.535533905932736864, -148.1250000000000000, 3.535533905932738641 ) ) ;
#34646=CARTESIAN_POINT ( 'NONE',  ( -4.458734124999999437, -73.64583333196773651, -2.574251347313719407 ) ) ;
#34649=CARTESIAN_POINT ( 'NONE',  ( -1.846868145590734756, -144.3750000013656063, -4.458734124999999437 ) ) ;
#34651=EDGE_CURVE ( 'NONE', #25000, #47748, #36226, .T. ) ;
#34653=CARTESIAN_POINT ( 'NONE',  ( -6.972266317189433020E-16, -0.2500000000000001665, -5.000000000000000000 ) ) ;
#34658=ORIENTED_EDGE ( 'NONE', *, *, #19239, .F. ) ;
#34659=CARTESIAN_POINT ( 'NONE',  ( -5.000000000000000888, -167.5625000000000284, -2.071067811865475949 ) ) ;
#34665=CARTESIAN_POINT ( 'NONE',  ( -4.458734124999999437, -71.56249999863439371, 0.000000000000000000 ) ) ;
#34668=CARTESIAN_POINT ( 'NONE',  ( 2.500000000000002220, -68.66666666666667140, 4.330127018922192761 ) ) ;
#34672=CARTESIAN_POINT ( 'NONE',  ( -6.972266317189433020E-16, -15.25000000000000000, -5.000000000000000000 ) ) ;
#34677=CARTESIAN_POINT ( 'NONE',  ( -2.229367062499996610, 18.60416666803225993, 3.861377020970582219 ) ) ;
#34678=CARTESIAN_POINT ( 'NONE',  ( 1.339745962155612702, -18.29465819873851729, -5.000000000000000000 ) ) ;
#34684=CARTESIAN_POINT ( 'NONE',  ( -3.152548672688508926E-16, 2.437500001365593860, -5.148502694627439702 ) ) ;
#34685=CARTESIAN_POINT ( 'NONE',  ( -4.458734124999997661, -26.47916666530107221, 2.574251347313722516 ) ) ;
#34688=CARTESIAN_POINT ( 'NONE',  ( -4.458734124999998549, 26.77083333469893134, 2.574251347313722516 ) ) ;
#34691=CARTESIAN_POINT ( 'NONE',  ( 9.457646018065525792E-16, -75.31249999863440792, 5.148502694627439702 ) ) ;
#34695=CARTESIAN_POINT ( 'NONE',  ( -5.000000000000000000, 26.04166666939784847, -2.886751345948128211 ) ) ;
#34696=VERTEX_POINT ( 'NONE', #10760 ) ;
#34697=CARTESIAN_POINT ( 'NONE',  ( 2.500000000000002220, 6.333333333333333037, 4.330127018922192761 ) ) ;
#34700=CARTESIAN_POINT ( 'NONE',  ( 5.000000000000000000, -19.49999999999999645, -6.123233995736766282E-16 ) ) ;
#34701=CARTESIAN_POINT ( 'NONE',  ( -2.229367062500000163, -24.47916666530106866, -3.861377020970580443 ) ) ;
#34703=CARTESIAN_POINT ( 'NONE',  ( 9.457646018065525792E-16, -82.06249999863440792, 5.148502694627439702 ) ) ;
#34704=( BOUNDED_CURVE ( )  B_SPLINE_CURVE ( 2, ( #5924, #14919, #54157, #29707, #35193, #44504, #54491, #14599, #43551 ),
 .UNSPECIFIED., .F., .F. ) 
 B_SPLINE_CURVE_WITH_KNOTS ( ( 3, 2, 2, 2, 3 ),
 ( 0.3583333333333336146, 0.3625000000000002665, 0.3666666666666669183, 0.3708333333333336257, 0.3750000000000002776 ),
 .UNSPECIFIED. ) 
 CURVE ( )  GEOMETRIC_REPRESENTATION_ITEM ( )  RATIONAL_B_SPLINE_CURVE ( ( 0.9999999999999948930, 0.9238795325112918455, 1.000000000000000000, 0.9238795325112867385, 1.000000000000000000, 0.9238795325112867385, 1.000000000000000000, 0.9238795325112816315, 1.000000000000005107 ) ) 
 REPRESENTATION_ITEM ( '' )  );
#34706=CARTESIAN_POINT ( 'NONE',  ( 5.000000000000000000, -18.37499999726881583, -6.123233995736766282E-16 ) ) ;
#34707=CARTESIAN_POINT ( 'NONE',  ( -4.458734124999999437, -50.31249999863440792, 0.000000000000000000 ) ) ;
#34710=CARTESIAN_POINT ( 'NONE',  ( 1.975475456537005874E-15, -15.62499999726881406, 5.000000000000000000 ) ) ;
#34711=CARTESIAN_POINT ( 'NONE',  ( -2.229367062499996610, 0.6041666680322611560, 3.861377020970582219 ) ) ;
#34714=CARTESIAN_POINT ( 'NONE',  ( -3.535250795749689387E-16, -67.25000000000000000, -5.773502691896257311 ) ) ;
#34715=CARTESIAN_POINT ( 'NONE',  ( 3.152801135295366208, -153.8125000013656063, 3.152801135295367985 ) ) ;
#34718=CARTESIAN_POINT ( 'NONE',  ( -2.071067811865475061, -161.6875000000000000, -5.000000000000000888 ) ) ;
#34721=CARTESIAN_POINT ( 'NONE',  ( -2.229367062500000163, -8.729166665301073991, -3.861377020970580443 ) ) ;
#34722=CARTESIAN_POINT ( 'NONE',  ( 4.458734124999999437, -48.06249999863440792, -5.460374474430324690E-16 ) ) ;
#34723=( BOUNDED_CURVE ( )  B_SPLINE_CURVE ( 2, ( #7432, #7112, #37015, #52443, #37634, #31862, #42143, #21902, #17399 ),
 .UNSPECIFIED., .F., .F. ) 
 B_SPLINE_CURVE_WITH_KNOTS ( ( 3, 2, 2, 2, 3 ),
 ( 0.8249999999999997335, 0.8291666666666664964, 0.8333333333333331483, 0.8374999999999998002, 0.8416666666666664520 ),
 .UNSPECIFIED. ) 
 CURVE ( )  GEOMETRIC_REPRESENTATION_ITEM ( )  RATIONAL_B_SPLINE_CURVE ( ( 1.000000000000003997, 0.9238795325112826307, 1.000000000000000000, 0.9238795325112867385, 1.000000000000000000, 0.9238795325112867385, 1.000000000000000000, 0.9238795325112908463, 0.9999999999999958922 ) ) 
 REPRESENTATION_ITEM ( '' )  );
#34725=CARTESIAN_POINT ( 'NONE',  ( -1.846868145590734756, -148.1250000013655779, -4.458734125000000326 ) ) ;
#34728=ORIENTED_EDGE ( 'NONE', *, *, #1720, .F. ) ;
#34731=CARTESIAN_POINT ( 'NONE',  ( 4.458734124999998549, 29.02083333469893134, -2.574251347313721627 ) ) ;
#34734=CARTESIAN_POINT ( 'NONE',  ( -1.339745962155613812, -62.20534180126146850, -5.000000000000000000 ) ) ;
#34737=EDGE_CURVE ( 'NONE', #26750, #2325, #58754, .T. ) ;
#34741=CARTESIAN_POINT ( 'NONE',  ( -4.458734124999998549, -4.229166665301070438, 2.574251347313722516 ) ) ;
#34743=CARTESIAN_POINT ( 'NONE',  ( 2.730187237215162345E-16, -150.1875000013656063, -4.458734124999999437 ) ) ;
#34746=EDGE_LOOP ( 'NONE', ( #44286, #16573, #12150, #45354 ) ) ;
#34748=CARTESIAN_POINT ( 'NONE',  ( -2.500000000000000444, -75.16666666666665719, -4.330127018922193649 ) ) ;
#34753=DIRECTION ( 'NONE',  ( 0.000000000000000000, 0.000000000000000000, 1.000000000000000000 ) ) ;
#34758=FACE_OUTER_BOUND ( 'NONE', #43804, .T. ) ;
#34759=DIRECTION ( 'NONE',  ( -0.000000000000000000, 1.000000000000000000, -0.000000000000000000 ) ) ;
#34760=CARTESIAN_POINT ( 'NONE',  ( 2.229367062500001939, 18.02083333469892779, 3.861377020970579999 ) ) ;
#34762=VERTEX_POINT ( 'NONE', #26515 ) ;
#34763=CARTESIAN_POINT ( 'NONE',  ( -3.152548672688508926E-16, -7.812499998634405252, -5.148502694627439702 ) ) ;
#34765=CARTESIAN_POINT ( 'NONE',  ( 3.152801135295366208, -166.5625000013656063, 3.152801135295367985 ) ) ;
#34766=CARTESIAN_POINT ( 'NONE',  ( 5.000000000000000000, -63.37499999726880873, -6.123233995736766282E-16 ) ) ;
#34770=CIRCLE ( 'NONE', #48125, 5.000000000000000000 ) ;
#34773=CARTESIAN_POINT ( 'NONE',  ( 0.000000000000000000, 30.00000000000000000, 5.000000000000000000 ) ) ;
#34774=CARTESIAN_POINT ( 'NONE',  ( 3.152801135295367541, -154.5625000013656063, -3.152801135295367541 ) ) ;
#34777=CARTESIAN_POINT ( 'NONE',  ( 0.000000000000000000, -170.0000000000000000, 5.000000000000000000 ) ) ;
#34778=ORIENTED_EDGE ( 'NONE', *, *, #2715, .T. ) ;
#34781=( BOUNDED_CURVE ( )  B_SPLINE_CURVE ( 2, ( #47066, #27433, #2689, #56086, #3331, #41583, #6882, #37412, #36459 ),
 .UNSPECIFIED., .F., .F. ) 
 B_SPLINE_CURVE_WITH_KNOTS ( ( 3, 2, 2, 2, 3 ),
 ( 0.6916666666666663188, 0.6958333333333329707, 0.6999999999999995115, 0.7041666666666662744, 0.7083333333333329263 ),
 .UNSPECIFIED. ) 
 CURVE ( )  GEOMETRIC_REPRESENTATION_ITEM ( )  RATIONAL_B_SPLINE_CURVE ( ( 1.000000000000005995, 0.9238795325112806323, 1.000000000000000000, 0.9238795325112867385, 1.000000000000000000, 0.9238795325112867385, 1.000000000000000000, 0.9238795325112948431, 0.9999999999999918954 ) ) 
 REPRESENTATION_ITEM ( '' )  );
#34782=CARTESIAN_POINT ( 'NONE',  ( 1.975475456537005874E-15, -68.74999999999998579, 5.000000000000000000 ) ) ;
#34783=CARTESIAN_POINT ( 'NONE',  ( 2.499999999999998668, -3.333333333333333925, -4.330127018922193649 ) ) ;
#34784=CARTESIAN_POINT ( 'NONE',  ( 4.458734125000000326, -64.89583333196773651, 2.574251347313718519 ) ) ;
#34786=DIRECTION ( 'NONE',  ( 0.000000000000000000, 0.000000000000000000, 1.000000000000000000 ) ) ;
#34788=CARTESIAN_POINT ( 'NONE',  ( -4.999999999999999112, -0.7916666639354794643, 2.886751345948131764 ) ) ;
#34789=CARTESIAN_POINT ( 'NONE',  ( -2.229367062499996610, -35.14583333196772941, 3.861377020970582219 ) ) ;
#34791=CARTESIAN_POINT ( 'NONE',  ( -6.972266317189433020E-16, 19.75000000000000000, -5.000000000000000000 ) ) ;
#34792=CARTESIAN_POINT ( 'NONE',  ( 2.071067811865327624, -156.8125000000000284, -5.000000000000148326 ) ) ;
#34795=CARTESIAN_POINT ( 'NONE',  ( 2.500000000000002220, -51.66666666666666430, 4.330127018922192761 ) ) ;
#34798=CARTESIAN_POINT ( 'NONE',  ( 5.000000000000000888, -32.45833333060215153, 2.886751345948126879 ) ) ;
#34799=CARTESIAN_POINT ( 'NONE',  ( -2.229367062499996610, -72.14583333196773651, 3.861377020970582219 ) ) ;
#34800=CARTESIAN_POINT ( 'NONE',  ( 3.152801135295367541, -142.5625000013655779, -3.152801135295367541 ) ) ;
#34801=CARTESIAN_POINT ( 'NONE',  ( 9.457646018065525792E-16, -84.06249999863439371, 5.148502694627439702 ) ) ;
#34804=CARTESIAN_POINT ( 'NONE',  ( 4.458734124999998549, -29.97916666530107577, -2.574251347313721627 ) ) ;
#34805=CARTESIAN_POINT ( 'NONE',  ( 5.000000000000000000, -70.29166666393547303, -2.886751345948129988 ) ) ;
#34807=DIRECTION ( 'NONE',  ( -0.000000000000000000, 1.000000000000000000, -0.000000000000000000 ) ) ;
#34811=VERTEX_POINT ( 'NONE', #7851 ) ;
#34813=( BOUNDED_CURVE ( )  B_SPLINE_CURVE ( 2, ( #30829, #31140, #46259, #2218, #26317, #41733, #56238, #21179, #60748 ),
 .UNSPECIFIED., .F., .F. ) 
 B_SPLINE_CURVE_WITH_KNOTS ( ( 3, 2, 2, 2, 3 ),
 ( 0.2354166666666666630, 0.2361111111111111049, 0.2374999999999999889, 0.2388888888888889006, 0.2395833333333333426 ),
 .UNSPECIFIED. ) 
 CURVE ( )  GEOMETRIC_REPRESENTATION_ITEM ( )  RATIONAL_B_SPLINE_CURVE ( ( 0.9330127018922194093, 0.9330127018922194093, 1.000000000000000000, 0.8660254037844387076, 1.000000000000000000, 0.8660254037844387076, 1.000000000000000000, 0.9330127018922194093, 0.9330127018922194093 ) ) 
 REPRESENTATION_ITEM ( '' )  );
#34814=CARTESIAN_POINT ( 'NONE',  ( -9.184850993605147944E-16, -160.2500000000000000, 5.000000000000000000 ) ) ;
#34815=CARTESIAN_POINT ( 'NONE',  ( 4.458734124999998549, -58.97916666530105800, -2.574251347313721627 ) ) ;
#34817=ORIENTED_EDGE ( 'NONE', *, *, #33339, .F. ) ;
#34821=CARTESIAN_POINT ( 'NONE',  ( -4.458734124999999437, 11.60416666803225993, -2.574251347313719407 ) ) ;
#34823=CARTESIAN_POINT ( 'NONE',  ( 1.975475456537005874E-15, -73.75000000000000000, 5.000000000000000000 ) ) ;
#34824=CARTESIAN_POINT ( 'NONE',  ( 2.730187237215162345E-16, -161.1875000013655779, -4.458734124999999437 ) ) ;
#34825=EDGE_LOOP ( 'NONE', ( #47022, #27763, #52820, #20117 ) ) ;
#34827=CARTESIAN_POINT ( 'NONE',  ( -6.972266317189433020E-16, -70.12499999726880162, -5.000000000000000000 ) ) ;
#34835=CARTESIAN_POINT ( 'NONE',  ( 1.339745962155615144, -61.70534180126146850, 4.999999999999999112 ) ) ;
#34840=CARTESIAN_POINT ( 'NONE',  ( -2.229367062499996610, 7.604166668032260823, 3.861377020970582219 ) ) ;
#34841=VECTOR ( 'NONE', #6473, 1000.000000000000000 ) ;
#34842=CARTESIAN_POINT ( 'NONE',  ( 5.000000000000000000, -146.1875000027312126, 2.071067811865478614 ) ) ;
#34844=CARTESIAN_POINT ( 'NONE',  ( -5.000000000000000000, -149.6250000027312126, -6.123233995736766282E-16 ) ) ;
#34845=LINE ( 'NONE', #53817, #22327 ) ;
#34846=EDGE_CURVE ( 'NONE', #50991, #63425, #42796, .T. ) ;
#34851=CARTESIAN_POINT ( 'NONE',  ( 1.975475456537005874E-15, -90.62499999726880162, 5.000000000000000000 ) ) ;
#34854=CARTESIAN_POINT ( 'NONE',  ( -1.846868145590737420, -167.0000000013655779, 4.458734124999997661 ) ) ;
#34855=DIRECTION ( 'NONE',  ( -0.000000000000000000, 1.000000000000000000, -0.000000000000000000 ) ) ;
#34858=CARTESIAN_POINT ( 'NONE',  ( 3.152801135295367541, -144.3125000013655779, -3.152801135295367541 ) ) ;
#34860=CARTESIAN_POINT ( 'NONE',  ( -3.535250795749689387E-16, -90.12499999726881583, -5.773502691896257311 ) ) ;
#34861=ORIENTED_EDGE ( 'NONE', *, *, #63263, .T. ) ;
#34862=CARTESIAN_POINT ( 'NONE',  ( 4.458734125000000326, -60.14583333196774362, 2.574251347313718519 ) ) ;
#34864=CARTESIAN_POINT ( 'NONE',  ( 0.000000000000000000, -170.0000000000000000, 5.000000000000000000 ) ) ;
#34865=CARTESIAN_POINT ( 'NONE',  ( 2.500000000000002220, 14.33333333333333393, 4.330127018922192761 ) ) ;
#34867=CARTESIAN_POINT ( 'NONE',  ( -4.458734124999999437, -53.39583333196773651, -2.574251347313719407 ) ) ;
#34868=CARTESIAN_POINT ( 'NONE',  ( 2.229367062500001939, -3.979166665301070438, 3.861377020970579999 ) ) ;
#34869=CARTESIAN_POINT ( 'NONE',  ( 0.000000000000000000, -170.0000000000000000, 0.000000000000000000 ) ) ;
#34872=CARTESIAN_POINT ( 'NONE',  ( 5.000000000000000888, -166.9375000000000284, -2.071067811865475505 ) ) ;
#34873=CARTESIAN_POINT ( 'NONE',  ( -6.972266317189433020E-16, -21.24999999999999289, -5.000000000000000000 ) ) ;
#34877=CARTESIAN_POINT ( 'NONE',  ( 4.458734124999998549, -51.72916666530107221, -2.574251347313721627 ) ) ;
#34878=CARTESIAN_POINT ( 'NONE',  ( 4.458734125000000326, -154.6250000013655779, -1.846868145590734978 ) ) ;
#34879=CARTESIAN_POINT ( 'NONE',  ( -3.535250795749689387E-16, -54.12499999726880162, -5.773502691896257311 ) ) ;
#34880=ORIENTED_EDGE ( 'NONE', *, *, #24937, .T. ) ;
#34882=CARTESIAN_POINT ( 'NONE',  ( 4.458734124999998549, 5.020833334698926897, -2.574251347313721627 ) ) ;
#34886=CARTESIAN_POINT ( 'NONE',  ( -1.846868145590734756, -155.1250000013655779, -4.458734125000000326 ) ) ;
#34890=CARTESIAN_POINT ( 'NONE',  ( 2.071067811865645591, -153.1875000000000000, 4.999999999999830358 ) ) ;
#34891=AXIS2_PLACEMENT_3D ( 'NONE', #53359, #42761, #58187 ) ;
#34892=CARTESIAN_POINT ( 'NONE',  ( 2.229367062499998831, -43.89583333196774362, -3.861377020970580887 ) ) ;
#34893=EDGE_LOOP ( 'NONE', ( #20795, #10121, #20571, #62979 ) ) ;
#34896=CARTESIAN_POINT ( 'NONE',  ( -4.458734124999998549, -90.47916666530106511, 2.574251347313722516 ) ) ;
#34899=PLANE ( 'NONE',  #10004 ) ;
#34902=CARTESIAN_POINT ( 'NONE',  ( -5.000000000000000000, 10.04166666939785024, -2.886751345948128211 ) ) ;
#34905=CARTESIAN_POINT ( 'NONE',  ( 2.500000000000002220, -33.66666666666666430, 4.330127018922192761 ) ) ;
#34908=CARTESIAN_POINT ( 'NONE',  ( -5.000000000000000000, 24.99999999999999645, 0.000000000000000000 ) ) ;
#34909=DIRECTION ( 'NONE',  ( -0.000000000000000000, 1.000000000000000000, -0.000000000000000000 ) ) ;
#34910=CYLINDRICAL_SURFACE ( 'NONE', #51019, 5.000000000000000000 ) ;
#34913=ORIENTED_EDGE ( 'NONE', *, *, #58518, .T. ) ;
#34916=CARTESIAN_POINT ( 'NONE',  ( 5.000000000000000888, -160.0625000027312126, -2.071067811865475505 ) ) ;
#34927=LINE ( 'NONE', #49397, #6956 ) ;
#34928=CARTESIAN_POINT ( 'NONE',  ( -2.229367062500000163, -18.47916666530106866, -3.861377020970580443 ) ) ;
#34929=CARTESIAN_POINT ( 'NONE',  ( -1.339745962155613812, -80.08034179853028434, -5.000000000000000000 ) ) ;
#34930=CARTESIAN_POINT ( 'NONE',  ( -3.535533905932738641, -154.3750000000000000, 3.535533905932737309 ) ) ;
#34932=CARTESIAN_POINT ( 'NONE',  ( -3.152801135295367096, -156.0625000013656063, -3.152801135295367541 ) ) ;
#34934=CARTESIAN_POINT ( 'NONE',  ( -4.458734124999999437, -45.56249999863440081, 0.000000000000000000 ) ) ;
#34935=CARTESIAN_POINT ( 'NONE',  ( 5.000000000000000000, -44.29166666393546592, -2.886751345948130876 ) ) ;
#34937=CARTESIAN_POINT ( 'NONE',  ( -2.229367062500000163, -88.47916666530106511, -3.861377020970580443 ) ) ;
#34940=CARTESIAN_POINT ( 'NONE',  ( 4.458734125000001214, 7.104166668032259047, 2.574251347313718519 ) ) ;
#34943=EDGE_CURVE ( 'NONE', #33786, #11102, #1684, .T. ) ;
#34944=CARTESIAN_POINT ( 'NONE',  ( -6.972266317189433020E-16, -68.12499999726881583, -5.000000000000000000 ) ) ;
#34946=CARTESIAN_POINT ( 'NONE',  ( 9.457646018065525792E-16, 18.68750000136559208, 5.148502694627439702 ) ) ;
#34948=CARTESIAN_POINT ( 'NONE',  ( -2.500000000000000444, 6.958333336064520758, -4.330127018922193649 ) ) ;
#34949=VERTEX_POINT ( 'NONE', #32283 ) ;
#34950=CARTESIAN_POINT ( 'NONE',  ( 0.000000000000000000, -170.0000000000000000, 0.000000000000000000 ) ) ;
#34953=CARTESIAN_POINT ( 'NONE',  ( 2.229367062500001939, -36.97916666530107221, 3.861377020970579999 ) ) ;
#34955=CARTESIAN_POINT ( 'NONE',  ( -4.999999999999999112, -37.79166666393547303, 2.886751345948131764 ) ) ;
#34958=CARTESIAN_POINT ( 'NONE',  ( 9.457646018065525792E-16, -10.06249999863440792, 5.148502694627439702 ) ) ;
#34959=CARTESIAN_POINT ( 'NONE',  ( 4.458734124999999437, -20.06249999863440081, -5.460374474430324690E-16 ) ) ;
#34961=( BOUNDED_CURVE ( )  B_SPLINE_CURVE ( 2, ( #5940, #41284, #2090, #20410, #11700, #30364, #45806, #25546, #21694 ),
 .UNSPECIFIED., .F., .F. ) 
 B_SPLINE_CURVE_WITH_KNOTS ( ( 3, 2, 2, 2, 3 ),
 ( 0.3750000000000002776, 0.3791666666666669294, 0.3833333333333336368, 0.3875000000000003442, 0.3916666666666669960 ),
 .UNSPECIFIED. ) 
 CURVE ( )  GEOMETRIC_REPRESENTATION_ITEM ( )  RATIONAL_B_SPLINE_CURVE ( ( 0.9999999999999948930, 0.9238795325112918455, 1.000000000000000000, 0.9238795325112867385, 1.000000000000000000, 0.9238795325112867385, 1.000000000000000000, 0.9238795325112806323, 1.000000000000005995 ) ) 
 REPRESENTATION_ITEM ( '' )  );
#34962=CARTESIAN_POINT ( 'NONE',  ( -4.999999999999999112, -83.91666666666667140, 2.886751345948131764 ) ) ;
#34963=DIRECTION ( 'NONE',  ( 0.000000000000000000, 0.000000000000000000, 1.000000000000000000 ) ) ;
#34966=CARTESIAN_POINT ( 'NONE',  ( 2.499999999999998668, -86.20833333060214443, -4.330127018922193649 ) ) ;
#34967=CARTESIAN_POINT ( 'NONE',  ( -5.000000000000000000, -18.00000000000000355, 0.000000000000000000 ) ) ;
#34970=CARTESIAN_POINT ( 'NONE',  ( 2.229367062499998831, -26.89583333196774007, -3.861377020970580887 ) ) ;
#34973=CARTESIAN_POINT ( 'NONE',  ( -4.458734125000001214, -163.1250000013656063, 1.846868145590734089 ) ) ;
#34974=ADVANCED_FACE ( 'NONE', ( #56106 ), #57066, .T. ) ;
#34976=DIRECTION ( 'NONE',  ( -0.000000000000000000, 1.000000000000000000, -0.000000000000000000 ) ) ;
#34977=VERTEX_POINT ( 'NONE', #41291 ) ;
#34980=CARTESIAN_POINT ( 'NONE',  ( -2.229367062500000163, -73.72916666530106511, -3.861377020970580443 ) ) ;
#34983=CARTESIAN_POINT ( 'NONE',  ( 4.458734124999999437, -147.6875000013656063, 0.000000000000000000 ) ) ;
#34984=CARTESIAN_POINT ( 'NONE',  ( 0.000000000000000000, -170.0000000000000000, 5.000000000000000000 ) ) ;
#34989=CARTESIAN_POINT ( 'NONE',  ( -8.190561711645485556E-16, -141.9375000013656063, 4.458734124999999437 ) ) ;
#34992=CARTESIAN_POINT ( 'NONE',  ( -5.000000000000000000, -52.99999999999999289, 0.000000000000000000 ) ) ;
#34994=CARTESIAN_POINT ( 'NONE',  ( 2.229367062500001939, -76.22916666530106511, 3.861377020970579999 ) ) ;
#35000=CARTESIAN_POINT ( 'NONE',  ( 5.000000000000000000, -146.0000000000000284, 0.000000000000000000 ) ) ;
#35006=EDGE_CURVE ( 'NONE', #50566, #14032, #43162, .T. ) ;
#35007=CARTESIAN_POINT ( 'NONE',  ( -4.458734124999997661, 18.52083333469892779, 2.574251347313722516 ) ) ;
#35008=CARTESIAN_POINT ( 'NONE',  ( 0.000000000000000000, -170.0000000000000000, 0.000000000000000000 ) ) ;
#35010=ADVANCED_FACE ( 'NONE', ( #8787 ), #4582, .T. ) ;
#35011=EDGE_CURVE ( 'NONE', #141, #11953, #18927, .T. ) ;
#35016=CARTESIAN_POINT ( 'NONE',  ( 4.458734125000000326, -5.895833331967740953, 2.574251347313718519 ) ) ;
#35017=CARTESIAN_POINT ( 'NONE',  ( 9.457646018065525792E-16, -29.31249999863440436, 5.148502694627439702 ) ) ;
#35022=EDGE_CURVE ( 'NONE', #592, #17293, #24206, .T. ) ;
#35023=CARTESIAN_POINT ( 'NONE',  ( 2.229367062500001939, 25.02083333469892779, 3.861377020970579999 ) ) ;
#35024=DIRECTION ( 'NONE',  ( -0.000000000000000000, 1.000000000000000000, -0.000000000000000000 ) ) ;
#35027=CARTESIAN_POINT ( 'NONE',  ( 4.458734124999998549, -78.97916666530106511, -2.574251347313721627 ) ) ;
#35030=CARTESIAN_POINT ( 'NONE',  ( 1.060575238724906964E-15, 22.37500000273118772, 5.773502691896257311 ) ) ;
#35032=CARTESIAN_POINT ( 'NONE',  ( -6.972266317189433020E-16, -1.124999997268814278, -5.000000000000000000 ) ) ;
#35033=DIRECTION ( 'NONE',  ( -0.000000000000000000, 1.000000000000000000, -0.000000000000000000 ) ) ;
#35034=CARTESIAN_POINT ( 'NONE',  ( 2.499999999999998668, -17.33333333333333215, -4.330127018922193649 ) ) ;
#35035=CARTESIAN_POINT ( 'NONE',  ( -4.458734124999999437, -21.39583333196774007, -2.574251347313719407 ) ) ;
#35037=CARTESIAN_POINT ( 'NONE',  ( 2.229367062499998831, -80.64583333196773651, -3.861377020970580887 ) ) ;
#35038=CARTESIAN_POINT ( 'NONE',  ( -3.535250795749689387E-16, -22.12499999726881228, -5.773502691896257311 ) ) ;
#35039=CARTESIAN_POINT ( 'NONE',  ( 4.458734124999999437, -51.81249999863440792, -5.460374474430324690E-16 ) ) ;
#35043=CARTESIAN_POINT ( 'NONE',  ( 4.458734124999998549, 3.020833334698928674, -2.574251347313721627 ) ) ;
#35046=CARTESIAN_POINT ( 'NONE',  ( -2.500000000000000444, -67.16666666666667140, -4.330127018922193649 ) ) ;
#35047=CARTESIAN_POINT ( 'NONE',  ( -4.458734124999999437, -152.1875000013656063, -5.460374474430324690E-16 ) ) ;
#35049=CARTESIAN_POINT ( 'NONE',  ( -1.339745962155610925, -76.66965819600731891, 5.000000000000000000 ) ) ;
#35050=CARTESIAN_POINT ( 'NONE',  ( -5.000000000000000000, -158.5000000000000000, -6.123233995736766282E-16 ) ) ;
#35053=CARTESIAN_POINT ( 'NONE',  ( 2.229367062500001939, -11.22916666530107044, 3.861377020970579999 ) ) ;
#35054=CARTESIAN_POINT ( 'NONE',  ( -4.458734124999999437, -46.56249999863440792, 0.000000000000000000 ) ) ;
#35056=CARTESIAN_POINT ( 'NONE',  ( -1.846868145590737420, -143.7500000013655779, 4.458734124999999437 ) ) ;
#35059=VERTEX_POINT ( 'NONE', #52546 ) ;
#35063=CARTESIAN_POINT ( 'NONE',  ( -5.000000000000000000, -62.08333333333332860, -2.886751345948128211 ) ) ;
#35066=CARTESIAN_POINT ( 'NONE',  ( -1.049326080737009628E-13, -19.75000000000000000, 5.000000000000000000 ) ) ;
#35068=CARTESIAN_POINT ( 'NONE',  ( 4.458734124999999437, -4.812499998634402587, -5.460374474430324690E-16 ) ) ;
#35069=CARTESIAN_POINT ( 'NONE',  ( 5.000000000000000000, -73.37499999726880162, -6.123233995736766282E-16 ) ) ;
#35070=CARTESIAN_POINT ( 'NONE',  ( 4.458734124999997661, -147.5000000013656063, 1.846868145590737864 ) ) ;
#35072=VERTEX_POINT ( 'NONE', #23272 ) ;
#35079=EDGE_CURVE ( 'NONE', #57060, #31680, #13617, .T. ) ;
#35081=CARTESIAN_POINT ( 'NONE',  ( -6.972266317189433020E-16, 12.87500000273118417, -5.000000000000000000 ) ) ;
#35085=CARTESIAN_POINT ( 'NONE',  ( 9.457646018065525792E-16, 14.93750000136559386, 5.148502694627439702 ) ) ;
#35088=CARTESIAN_POINT ( 'NONE',  ( -4.458734124999997661, -12.47916666530107044, 2.574251347313722516 ) ) ;
#35089=EDGE_CURVE ( 'NONE', #27389, #28458, #8244, .T. ) ;
#35091=CARTESIAN_POINT ( 'NONE',  ( -4.458734125000001214, -161.8750000013656063, 1.846868145590734089 ) ) ;
#35095=ADVANCED_FACE ( 'NONE', ( #18744 ), #62521, .T. ) ;
#35096=ADVANCED_FACE ( 'NONE', ( #33235 ), #13922, .T. ) ;
#35097=( BOUNDED_CURVE ( )  B_SPLINE_CURVE ( 2, ( #58852, #9330, #24765, #28943, #49837, #4508, #4825, #44369, #15 ),
 .UNSPECIFIED., .F., .F. ) 
 B_SPLINE_CURVE_WITH_KNOTS ( ( 3, 2, 2, 2, 3 ),
 ( 0.8145833333333333259, 0.8152777777777777679, 0.8166666666666666519, 0.8180555555555555358, 0.8187499999999999778 ),
 .UNSPECIFIED. ) 
 CURVE ( )  GEOMETRIC_REPRESENTATION_ITEM ( )  RATIONAL_B_SPLINE_CURVE ( ( 0.9330127018922194093, 0.9330127018922194093, 1.000000000000000000, 0.8660254037844387076, 1.000000000000000000, 0.8660254037844387076, 1.000000000000000000, 0.9330127018922194093, 0.9330127018922194093 ) ) 
 REPRESENTATION_ITEM ( '' )  );
#35099=CARTESIAN_POINT ( 'NONE',  ( -5.000000000000000000, -54.95833333060214443, -2.886751345948128211 ) ) ;
#35102=CARTESIAN_POINT ( 'NONE',  ( -3.152801135295367096, -154.3125000013656063, -3.152801135295367541 ) ) ;
#35110=CARTESIAN_POINT ( 'NONE',  ( -5.000000000000000000, -8.958333330602144429, -2.886751345948128211 ) ) ;
#35112=CARTESIAN_POINT ( 'NONE',  ( -5.000000000000000000, -4.999999999999997335, 0.000000000000000000 ) ) ;
#35113=CARTESIAN_POINT ( 'NONE',  ( 4.458734124999998549, -66.72916666530106511, -2.574251347313721627 ) ) ;
#35115=CARTESIAN_POINT ( 'NONE',  ( 1.339745962155615144, -22.58034179853029144, 4.999999999999999112 ) ) ;
#35117=CARTESIAN_POINT ( 'NONE',  ( 5.000000000000000000, -6.291666663935480130, -2.886751345948129988 ) ) ;
#35118=CARTESIAN_POINT ( 'NONE',  ( 4.458734124999999437, -32.81249999863440792, -5.460374474430324690E-16 ) ) ;
#35123=CARTESIAN_POINT ( 'NONE',  ( -5.000000000000000000, -49.08333333333332860, -2.886751345948128211 ) ) ;
#35126=CARTESIAN_POINT ( 'NONE',  ( -2.500000000000000444, 13.95833333606451809, -4.330127018922193649 ) ) ;
#35127=CARTESIAN_POINT ( 'NONE',  ( 2.229367062499998831, -76.64583333196773651, -3.861377020970580887 ) ) ;
#35128=CARTESIAN_POINT ( 'NONE',  ( 1.846868145590735200, -143.5000000013656063, -4.458734125000000326 ) ) ;
#35129=CARTESIAN_POINT ( 'NONE',  ( 4.458734124999999437, -83.81249999863439371, -5.460374474430324690E-16 ) ) ;
#35131=CARTESIAN_POINT ( 'NONE',  ( -3.152548672688508926E-16, -30.81249999863440436, -5.148502694627439702 ) ) ;
#35132=CARTESIAN_POINT ( 'NONE',  ( 2.499999999999998668, -74.20833333060214443, -4.330127018922193649 ) ) ;
#35133=ORIENTED_EDGE ( 'NONE', *, *, #44884, .T. ) ;
#35138=ORIENTED_EDGE ( 'NONE', *, *, #52689, .T. ) ;
#35139=CARTESIAN_POINT ( 'NONE',  ( 5.000000000000000888, 27.41666666666666430, 2.886751345948126879 ) ) ;
#35141=CARTESIAN_POINT ( 'NONE',  ( 4.458734124999998549, -66.97916666530107932, -2.574251347313721627 ) ) ;
#35144=CARTESIAN_POINT ( 'NONE',  ( 0.000000000000000000, -170.0000000000000000, 0.000000000000000000 ) ) ;
#35145=FACE_OUTER_BOUND ( 'NONE', #11007, .T. ) ;
#35146=CARTESIAN_POINT ( 'NONE',  ( 4.458734125000001214, 11.10416666803225993, 2.574251347313718519 ) ) ;
#35148=CARTESIAN_POINT ( 'NONE',  ( 2.500000000000002220, -27.54166666393548013, 4.330127018922192761 ) ) ;
#35149=CARTESIAN_POINT ( 'NONE',  ( 3.152801135295367541, -160.3125000013656063, -3.152801135295367541 ) ) ;
#35151=VERTEX_POINT ( 'NONE', #34814 ) ;
#35153=DIRECTION ( 'NONE',  ( 0.000000000000000000, 0.000000000000000000, 1.000000000000000000 ) ) ;
#35156=DIRECTION ( 'NONE',  ( 0.000000000000000000, 0.000000000000000000, 1.000000000000000000 ) ) ;
#35159=CARTESIAN_POINT ( 'NONE',  ( -5.000000000000000000, -72.87499999726880162, 0.000000000000000000 ) ) ;
#35165=CARTESIAN_POINT ( 'NONE',  ( 4.458734125000000326, 2.854166668032259491, 2.574251347313718519 ) ) ;
#35166=( BOUNDED_CURVE ( )  B_SPLINE_CURVE ( 2, ( #24959, #44564, #522, #20132, #54548, #30084, #49714, #44893, #17543 ),
 .UNSPECIFIED., .F., .F. ) 
 B_SPLINE_CURVE_WITH_KNOTS ( ( 3, 2, 2, 2, 3 ),
 ( 0.9083333333333332149, 0.9124999999999998668, 0.9166666666666665186, 0.9208333333333330595, 0.9249999999999998224 ),
 .UNSPECIFIED. ) 
 CURVE ( )  GEOMETRIC_REPRESENTATION_ITEM ( )  RATIONAL_B_SPLINE_CURVE ( ( 1.000000000000001998, 0.9238795325112847401, 1.000000000000000000, 0.9238795325112867385, 1.000000000000000000, 0.9238795325112867385, 1.000000000000000000, 0.9238795325112908463, 0.9999999999999958922 ) ) 
 REPRESENTATION_ITEM ( '' )  );
#35167=CARTESIAN_POINT ( 'NONE',  ( -3.535533905932737309, -161.7500000027312126, -3.535533905932738197 ) ) ;
#35169=CARTESIAN_POINT ( 'NONE',  ( -5.000000000000000888, -146.6875000027312126, -2.071067811865475949 ) ) ;
#35170=CARTESIAN_POINT ( 'NONE',  ( -2.500000000000000444, 28.83333333333333215, -4.330127018922193649 ) ) ;
#35174=CYLINDRICAL_SURFACE ( 'NONE', #1077, 5.000000000000000000 ) ;
#35175=CARTESIAN_POINT ( 'NONE',  ( -9.184850993605147944E-16, -141.3750000027312126, 5.000000000000000000 ) ) ;
#35177=CARTESIAN_POINT ( 'NONE',  ( 4.458734124999999437, -164.6250000013656063, -1.846868145590734978 ) ) ;
#35181=CARTESIAN_POINT ( 'NONE',  ( 4.458734125000000326, -143.3750000013656063, -1.846868145590734978 ) ) ;
#35182=EDGE_LOOP ( 'NONE', ( #7547, #55910, #2630, #43030 ) ) ;
#35183=CARTESIAN_POINT ( 'NONE',  ( 9.457646018065525792E-16, 22.68750000136559564, 5.148502694627439702 ) ) ;
#35184=VERTEX_POINT ( 'NONE', #45738 ) ;
#35185=CARTESIAN_POINT ( 'NONE',  ( 9.457646018065525792E-16, -62.31249999863440792, 5.148502694627439702 ) ) ;
#35187=CARTESIAN_POINT ( 'NONE',  ( -9.184850993605147944E-16, -139.3750000027312126, 5.000000000000000000 ) ) ;
#35188=CARTESIAN_POINT ( 'NONE',  ( -5.000000000000000000, 12.91666666666666785, -2.886751345948128211 ) ) ;
#35189=CARTESIAN_POINT ( 'NONE',  ( -2.229367062500000163, -51.47916666530107221, -3.861377020970580443 ) ) ;
#35190=CARTESIAN_POINT ( 'NONE',  ( -2.229367062500000163, -13.47916666530107221, -3.861377020970580443 ) ) ;
#35193=CARTESIAN_POINT ( 'NONE',  ( 5.000000000000000000, -158.1250000027311842, 0.000000000000000000 ) ) ;
#35195=CARTESIAN_POINT ( 'NONE',  ( 1.975475456537005874E-15, -9.750000000000000000, 5.000000000000000000 ) ) ;
#35196=( BOUNDED_CURVE ( )  B_SPLINE_CURVE ( 2, ( #24281, #54834, #58696, #43883, #63531, #4979, #53866, #10763, #34237 ),
 .UNSPECIFIED., .F., .F. ) 
 B_SPLINE_CURVE_WITH_KNOTS ( ( 3, 2, 2, 2, 3 ),
 ( 0.6312499999999999778, 0.6319444444444444198, 0.6333333333333333037, 0.6347222222222221877, 0.6354166666666666297 ),
 .UNSPECIFIED. ) 
 CURVE ( )  GEOMETRIC_REPRESENTATION_ITEM ( )  RATIONAL_B_SPLINE_CURVE ( ( 0.9330127018922194093, 0.9330127018922194093, 1.000000000000000000, 0.8660254037844387076, 1.000000000000000000, 0.8660254037844387076, 1.000000000000000000, 0.9330127018922194093, 0.9330127018922194093 ) ) 
 REPRESENTATION_ITEM ( '' )  );
#35200=CARTESIAN_POINT ( 'NONE',  ( 4.458734124999998549, -57.72916666530107221, -2.574251347313721627 ) ) ;
#35201=CARTESIAN_POINT ( 'NONE',  ( -1.846868145590737420, -156.0000000013656063, 4.458734124999999437 ) ) ;
#35202=CARTESIAN_POINT ( 'NONE',  ( 5.000000000000000888, -55.45833333060214443, 2.886751345948126879 ) ) ;
#35204=CARTESIAN_POINT ( 'NONE',  ( 4.458734125000001214, -3.145833331967738733, 2.574251347313718519 ) ) ;
#35207=CARTESIAN_POINT ( 'NONE',  ( -4.458734125000001214, -157.8750000013656063, 1.846868145590734089 ) ) ;
#35209=CARTESIAN_POINT ( 'NONE',  ( 0.000000000000000000, -170.0000000000000000, 0.000000000000000000 ) ) ;
#35211=CARTESIAN_POINT ( 'NONE',  ( 5.000000000000000888, -152.9375000000000000, -2.071067811865475505 ) ) ;
#35212=CARTESIAN_POINT ( 'NONE',  ( -3.152548672688508926E-16, -42.81249999863440081, -5.148502694627439702 ) ) ;
#35214=CARTESIAN_POINT ( 'NONE',  ( 2.071067811865517694, -142.9375000027312126, -4.999999999999958256 ) ) ;
#35216=CARTESIAN_POINT ( 'NONE',  ( -4.458734124999999437, 27.68750000136559208, 0.000000000000000000 ) ) ;
#35218=CARTESIAN_POINT ( 'NONE',  ( 0.000000000000000000, -170.0000000000000000, 5.000000000000000000 ) ) ;
#35219=CARTESIAN_POINT ( 'NONE',  ( -2.499999999999996447, -35.70833333060213732, 4.330127018922195425 ) ) ;
#35224=CARTESIAN_POINT ( 'NONE',  ( 5.000000000000000000, -33.41666666666666430, -2.886751345948130876 ) ) ;
#35225=CARTESIAN_POINT ( 'NONE',  ( -4.999999999999998224, -1.791666663935480353, 2.886751345948131764 ) ) ;
#35228=CARTESIAN_POINT ( 'NONE',  ( -6.972266317189433020E-16, 4.749999999999999112, -5.000000000000000000 ) ) ;
#35230=CARTESIAN_POINT ( 'NONE',  ( -4.458734124999999437, -88.56249999863439371, 0.000000000000000000 ) ) ;
#35233=ORIENTED_EDGE ( 'NONE', *, *, #27971, .T. ) ;
#35236=CARTESIAN_POINT ( 'NONE',  ( 5.000000000000000000, -162.1250000027311842, 0.000000000000000000 ) ) ;
#35239=CARTESIAN_POINT ( 'NONE',  ( 3.535533905932736864, -163.2500000027312126, 3.535533905932738641 ) ) ;
#35247=CARTESIAN_POINT ( 'NONE',  ( 5.000000000000000000, -48.29166666393548724, -2.886751345948130876 ) ) ;
#35248=CARTESIAN_POINT ( 'NONE',  ( -4.458734124999999437, -17.31249999863440792, 0.000000000000000000 ) ) ;
#35249=CARTESIAN_POINT ( 'NONE',  ( 3.061616997868383141E-16, -154.7500000000000000, -5.000000000000000000 ) ) ;
#35251=CARTESIAN_POINT ( 'NONE',  ( -3.152801135295367096, -155.0625000013656063, -3.152801135295367541 ) ) ;
#35253=CARTESIAN_POINT ( 'NONE',  ( -4.458734124999999437, -47.64583333196775072, -2.574251347313719407 ) ) ;
#35256=CARTESIAN_POINT ( 'NONE',  ( 2.499999999999998668, 28.66666666666666785, -4.330127018922193649 ) ) ;
#35257=CARTESIAN_POINT ( 'NONE',  ( -4.458734124999999437, 3.604166668032260379, -2.574251347313719407 ) ) ;
#35260=CARTESIAN_POINT ( 'NONE',  ( 1.339745962155612702, -82.29465819873851729, -5.000000000000000000 ) ) ;
#35261=CARTESIAN_POINT ( 'NONE',  ( 4.458734124999998549, 19.02083333469892779, -2.574251347313721627 ) ) ;
#35263=CARTESIAN_POINT ( 'NONE',  ( -2.499999999999996447, 7.291666669397852019, 4.330127018922195425 ) ) ;
#35268=CARTESIAN_POINT ( 'NONE',  ( 4.458734124999999437, -36.81249999863440792, -5.460374474430324690E-16 ) ) ;
#35270=CARTESIAN_POINT ( 'NONE',  ( 5.000000000000000000, -41.29166666393548013, -2.886751345948129988 ) ) ;
#35272=CARTESIAN_POINT ( 'NONE',  ( 4.458734125000001214, -11.89583333196774007, 2.574251347313718519 ) ) ;
#35274=CARTESIAN_POINT ( 'NONE',  ( -2.500000000000000444, -84.16666666666667140, -4.330127018922193649 ) ) ;
#35275=CARTESIAN_POINT ( 'NONE',  ( -5.000000000000000000, 1.041666669397853351, -2.886751345948128211 ) ) ;
#35277=CARTESIAN_POINT ( 'NONE',  ( 5.000000000000000000, -89.29166666393545881, -2.886751345948129988 ) ) ;
#35278=CARTESIAN_POINT ( 'NONE',  ( -6.972266317189433020E-16, -49.12499999726880162, -5.000000000000000000 ) ) ;
#35279=ORIENTED_EDGE ( 'NONE', *, *, #2009, .T. ) ;
#35281=EDGE_CURVE ( 'NONE', #30690, #42274, #54245, .T. ) ;
#35282=CARTESIAN_POINT ( 'NONE',  ( 4.458734124999998549, -25.97916666530106866, -2.574251347313721627 ) ) ;
#35283=CARTESIAN_POINT ( 'NONE',  ( 1.975475456537005874E-15, -49.74999999999999289, 5.000000000000000000 ) ) ;
#35285=( BOUNDED_CURVE ( )  B_SPLINE_CURVE ( 2, ( #26464, #22278, #46081, #55738, #2040, #12307, #26144, #27404, #61204 ),
 .UNSPECIFIED., .F., .F. ) 
 B_SPLINE_CURVE_WITH_KNOTS ( ( 3, 2, 2, 2, 3 ),
 ( 0.2916666666666669072, 0.2958333333333335591, 0.3000000000000002665, 0.3041666666666669183, 0.3083333333333336257 ),
 .UNSPECIFIED. ) 
 CURVE ( )  GEOMETRIC_REPRESENTATION_ITEM ( )  RATIONAL_B_SPLINE_CURVE ( ( 0.9999999999999958922, 0.9238795325112908463, 1.000000000000000000, 0.9238795325112867385, 1.000000000000000000, 0.9238795325112867385, 1.000000000000000000, 0.9238795325112816315, 1.000000000000005107 ) ) 
 REPRESENTATION_ITEM ( '' )  );
#35286=SHAPE_DEFINITION_REPRESENTATION ( #43011, #25037 ) ;
#35287=CARTESIAN_POINT ( 'NONE',  ( 4.458734124999999437, -164.6875000013655779, 0.000000000000000000 ) ) ;
#35289=CARTESIAN_POINT ( 'NONE',  ( -5.000000000000000000, -38.87499999726880162, 0.000000000000000000 ) ) ;
#35290=ORIENTED_EDGE ( 'NONE', *, *, #49454, .F. ) ;
#35292=CARTESIAN_POINT ( 'NONE',  ( -3.152548672688508926E-16, -74.81249999863439371, -5.148502694627439702 ) ) ;
#35295=CARTESIAN_POINT ( 'NONE',  ( 3.152801135295366208, -142.8125000013655779, 3.152801135295367985 ) ) ;
#35302=CARTESIAN_POINT ( 'NONE',  ( -5.000000000000000000, -167.5000000000000000, -6.123233995736766282E-16 ) ) ;
#35308=CARTESIAN_POINT ( 'NONE',  ( -4.458734124999999437, -71.64583333196773651, -2.574251347313719407 ) ) ;
#35311=CARTESIAN_POINT ( 'NONE',  ( 2.626220312808019583E-14, 14.87500000273118239, -5.000000000000000000 ) ) ;
#35313=ORIENTED_EDGE ( 'NONE', *, *, #59063, .F. ) ;
#35315=CARTESIAN_POINT ( 'NONE',  ( -2.499999999999996447, -59.83333333333333570, 4.330127018922195425 ) ) ;
#35320=CARTESIAN_POINT ( 'NONE',  ( 4.458734125000000326, 15.85416666803226171, 2.574251347313718519 ) ) ;
#35326=CARTESIAN_POINT ( 'NONE',  ( 9.457646018065525792E-16, -84.06249999863439371, 5.148502694627439702 ) ) ;
#35327=CARTESIAN_POINT ( 'NONE',  ( 4.458734124999999437, -3.812499998634408360, -5.460374474430324690E-16 ) ) ;
#35329=CARTESIAN_POINT ( 'NONE',  ( -4.458734124999999437, -31.56249999863440436, 0.000000000000000000 ) ) ;
#35333=CARTESIAN_POINT ( 'NONE',  ( -3.152548672688508926E-16, 24.43750000136559564, -5.148502694627439702 ) ) ;
#35336=CARTESIAN_POINT ( 'NONE',  ( -3.535533905932737309, -145.7500000027311842, -3.535533905932738197 ) ) ;
#35337=CARTESIAN_POINT ( 'NONE',  ( -4.458734124999999437, -76.56249999863440792, 0.000000000000000000 ) ) ;
#35340=CARTESIAN_POINT ( 'NONE',  ( 2.500000000000002220, 26.45833333606451632, 4.330127018922192761 ) ) ;
#35342=CARTESIAN_POINT ( 'NONE',  ( 1.339745962155615144, -1.580341798530293662, 4.999999999999999112 ) ) ;
#35344=LINE ( 'NONE', #49176, #8320 ) ;
#35345=CARTESIAN_POINT ( 'NONE',  ( -4.999999999999999112, -20.91666666666666785, 2.886751345948131764 ) ) ;
#35346=CARTESIAN_POINT ( 'NONE',  ( 4.458734125000001214, -19.89583333196773651, 2.574251347313718519 ) ) ;
#35347=CARTESIAN_POINT ( 'NONE',  ( 4.458734124999998549, -84.72916666530106511, -2.574251347313721627 ) ) ;
#35348=CARTESIAN_POINT ( 'NONE',  ( -5.000000000000000000, -23.95833333060214443, -2.886751345948128211 ) ) ;
#35349=CARTESIAN_POINT ( 'NONE',  ( 2.229367062500001939, -47.97916666530106511, 3.861377020970579999 ) ) ;
#35352=CARTESIAN_POINT ( 'NONE',  ( 4.458734125000001214, -4.145833331967740065, 2.574251347313718519 ) ) ;
#35353=ORIENTED_EDGE ( 'NONE', *, *, #13465, .T. ) ;
#35355=CARTESIAN_POINT ( 'NONE',  ( -3.535250795749689387E-16, -68.25000000000000000, -5.773502691896257311 ) ) ;
#35356=CARTESIAN_POINT ( 'NONE',  ( 4.458734124999999437, -153.7500000013656063, 1.846868145590737864 ) ) ;
#35358=CARTESIAN_POINT ( 'NONE',  ( 5.000000000000000888, -158.9375000000000000, -2.071067811865475505 ) ) ;
#35360=EDGE_CURVE ( 'NONE', #10208, #48999, #19881, .T. ) ;
#35361=CARTESIAN_POINT ( 'NONE',  ( 2.229367062500001939, -13.22916666530107221, 3.861377020970579999 ) ) ;
#35362=CARTESIAN_POINT ( 'NONE',  ( -2.229367062500000163, -49.72916666530107221, -3.861377020970580443 ) ) ;
#35364=DIRECTION ( 'NONE',  ( 0.000000000000000000, 0.000000000000000000, 1.000000000000000000 ) ) ;
#35365=CARTESIAN_POINT ( 'NONE',  ( 3.152801135295366208, -144.5625000013655779, 3.152801135295367985 ) ) ;
#35368=VERTEX_POINT ( 'NONE', #60227 ) ;
#35370=CARTESIAN_POINT ( 'NONE',  ( -3.152548672688508926E-16, 24.18750000136559564, -5.148502694627439702 ) ) ;
#35372=EDGE_CURVE ( 'NONE', #17248, #20760, #3733, .T. ) ;
#35373=CARTESIAN_POINT ( 'NONE',  ( -6.972266317189433020E-16, -65.12499999726880162, -5.000000000000000000 ) ) ;
#35374=ORIENTED_EDGE ( 'NONE', *, *, #58542, .F. ) ;
#35379=CARTESIAN_POINT ( 'NONE',  ( -1.339745962155613812, 1.919658201469706116, -5.000000000000000000 ) ) ;
#35380=CARTESIAN_POINT ( 'NONE',  ( -2.229367062500000163, -6.479166665301072214, -3.861377020970580443 ) ) ;
#35383=CARTESIAN_POINT ( 'NONE',  ( 3.152801135295366208, -147.5625000013655779, 3.152801135295367985 ) ) ;
#35386=ORIENTED_EDGE ( 'NONE', *, *, #10205, .T. ) ;
#35390=DIRECTION ( 'NONE',  ( -0.000000000000000000, 1.000000000000000000, -0.000000000000000000 ) ) ;
#35394=CARTESIAN_POINT ( 'NONE',  ( 2.500000000000002220, -74.66666666666665719, 4.330127018922192761 ) ) ;
#35396=CARTESIAN_POINT ( 'NONE',  ( -5.000000000000000000, -89.87499999726880162, 0.000000000000000000 ) ) ;
#35398=CARTESIAN_POINT ( 'NONE',  ( -2.229367062499996610, 12.85416666803226171, 3.861377020970582219 ) ) ;
#35400=ORIENTED_EDGE ( 'NONE', *, *, #57754, .F. ) ;
#35401=CARTESIAN_POINT ( 'NONE',  ( 4.458734125000000326, -12.14583333196774007, 2.574251347313718519 ) ) ;
#35403=CARTESIAN_POINT ( 'NONE',  ( 4.458734124999999437, -164.5000000013655779, 1.846868145590737864 ) ) ;
#35404=CARTESIAN_POINT ( 'NONE',  ( -2.499999999999996447, -37.83333333333332860, 4.330127018922195425 ) ) ;
#35407=EDGE_CURVE ( 'NONE', #23020, #35439, #36400, .T. ) ;
#35409=AXIS2_PLACEMENT_3D ( 'NONE', #5762, #25707, #45318 ) ;
#35410=CARTESIAN_POINT ( 'NONE',  ( -2.500000000000000444, -77.16666666666665719, -4.330127018922193649 ) ) ;
#35413=CARTESIAN_POINT ( 'NONE',  ( -8.190561711645485556E-16, -148.9375000013656063, 4.458734124999999437 ) ) ;
#35417=ORIENTED_EDGE ( 'NONE', *, *, #8217, .T. ) ;
#35420=CARTESIAN_POINT ( 'NONE',  ( 1.339745962155615144, 12.29465819873851906, 4.999999999999999112 ) ) ;
#35421=CARTESIAN_POINT ( 'NONE',  ( -2.499999999999996447, -1.833333333333332593, 4.330127018922195425 ) ) ;
#35422=CARTESIAN_POINT ( 'NONE',  ( 2.229367062499998831, -64.64583333196773651, -3.861377020970580887 ) ) ;
#35424=CARTESIAN_POINT ( 'NONE',  ( 2.499999999999998668, -6.208333330602149758, -4.330127018922193649 ) ) ;
#35425=CARTESIAN_POINT ( 'NONE',  ( 2.229367062499998831, -35.64583333196772941, -3.861377020970580887 ) ) ;
#35426=ORIENTED_EDGE ( 'NONE', *, *, #24137, .F. ) ;
#35427=CARTESIAN_POINT ( 'NONE',  ( 1.975475456537005874E-15, -77.75000000000000000, 5.000000000000000000 ) ) ;
#35429=CARTESIAN_POINT ( 'NONE',  ( -3.152548672688508926E-16, 12.18750000136559564, -5.148502694627439702 ) ) ;
#35430=ORIENTED_EDGE ( 'NONE', *, *, #16503, .F. ) ;
#35431=CARTESIAN_POINT ( 'NONE',  ( -3.535250795749689387E-16, -48.25000000000000000, -5.773502691896257311 ) ) ;
#35433=CARTESIAN_POINT ( 'NONE',  ( -3.152548672688508926E-16, -73.56249999863440792, -5.148502694627439702 ) ) ;
#35434=CARTESIAN_POINT ( 'NONE',  ( -2.071067811865478170, -169.3125000000000284, 5.000000000000000000 ) ) ;
#35435=CARTESIAN_POINT ( 'NONE',  ( -3.152548672688508926E-16, -80.56249999863440792, -5.148502694627439702 ) ) ;
#35437=CARTESIAN_POINT ( 'NONE',  ( -3.152548672688508926E-16, -27.81249999863440436, -5.148502694627439702 ) ) ;
#35438=EDGE_CURVE ( 'NONE', #43179, #48474, #7771, .T. ) ;
#35439=VERTEX_POINT ( 'NONE', #37352 ) ;
#35445=EDGE_CURVE ( 'NONE', #44005, #25400, #46373, .T. ) ;
#35447=DIRECTION ( 'NONE',  ( 1.000000000000000000, 0.000000000000000000, -0.000000000000000000 ) ) ;
#35448=CARTESIAN_POINT ( 'NONE',  ( 5.000000000000000000, -12.49999999999999645, -6.123233995736766282E-16 ) ) ;
#35449=CARTESIAN_POINT ( 'NONE',  ( -2.229367062499996610, -62.39583333196774362, 3.861377020970582219 ) ) ;
#35452=ORIENTED_EDGE ( 'NONE', *, *, #58150, .T. ) ;
#35453=EDGE_CURVE ( 'NONE', #8541, #20951, #15747, .T. ) ;
#35454=VECTOR ( 'NONE', #15017, 1000.000000000000000 ) ;
#35455=CARTESIAN_POINT ( 'NONE',  ( 1.339745962155612702, -62.29465819873851729, -5.000000000000000000 ) ) ;
#35457=EDGE_CURVE ( 'NONE', #5644, #55393, #51208, .T. ) ;
#35458=EDGE_CURVE ( 'NONE', #51028, #43336, #56357, .T. ) ;
#35459=CARTESIAN_POINT ( 'NONE',  ( 9.457646018065525792E-16, 7.937500001365594748, 5.148502694627439702 ) ) ;
#35461=CARTESIAN_POINT ( 'NONE',  ( 5.000000000000000000, -27.37499999726880873, -6.123233995736766282E-16 ) ) ;
#35462=CARTESIAN_POINT ( 'NONE',  ( -4.458734125000000326, -162.8750000013655779, 1.846868145590734089 ) ) ;
#35464=ORIENTED_EDGE ( 'NONE', *, *, #13866, .T. ) ;
#35465=ADVANCED_FACE ( 'NONE', ( #61497 ), #60544, .T. ) ;
#35467=EDGE_CURVE ( 'NONE', #27870, #51343, #51072, .T. ) ;
#35470=CARTESIAN_POINT ( 'NONE',  ( 0.000000000000000000, -170.0000000000000000, 0.000000000000000000 ) ) ;
#35477=CARTESIAN_POINT ( 'NONE',  ( -2.500000000000000444, -83.04166666393547303, -4.330127018922193649 ) ) ;
#35478=CARTESIAN_POINT ( 'NONE',  ( 4.458734124999999437, 27.18750000136559564, -5.460374474430324690E-16 ) ) ;
#35481=CARTESIAN_POINT ( 'NONE',  ( -2.229367062499996610, 3.604166668032260379, 3.861377020970582219 ) ) ;
#35482=CARTESIAN_POINT ( 'NONE',  ( 6.123233995736766282E-16, -170.0000000000000000, -5.000000000000000000 ) ) ;
#35484=CARTESIAN_POINT ( 'NONE',  ( -3.535533905932737309, -145.7500000027311842, -3.535533905932738197 ) ) ;
#35490=CARTESIAN_POINT ( 'NONE',  ( 5.000000000000000888, -141.0625000027312410, -2.071067811865475505 ) ) ;
#35492=CARTESIAN_POINT ( 'NONE',  ( 1.846868145590735200, -160.5000000013656347, -4.458734124999999437 ) ) ;
#35496=CARTESIAN_POINT ( 'NONE',  ( 3.152801135295366208, -141.5625000013655779, 3.152801135295367985 ) ) ;
#35497=EDGE_LOOP ( 'NONE', ( #6292, #1380, #2939, #57755 ) ) ;
#35498=CARTESIAN_POINT ( 'NONE',  ( -4.458734124999999437, 20.43750000136559208, 0.000000000000000000 ) ) ;
#35499=EDGE_LOOP ( 'NONE', ( #48400, #53376, #61615, #40366 ) ) ;
#35500=CARTESIAN_POINT ( 'NONE',  ( 2.229367062500001939, -60.22916666530106511, 3.861377020970579999 ) ) ;
#35503=CARTESIAN_POINT ( 'NONE',  ( 2.499999999999998668, 11.66666666666666607, -4.330127018922193649 ) ) ;
#35504=CARTESIAN_POINT ( 'NONE',  ( -4.458734124999999437, -51.31249999863440792, 0.000000000000000000 ) ) ;
#35505=CARTESIAN_POINT ( 'NONE',  ( 2.229367062500001939, -12.97916666530107221, 3.861377020970579999 ) ) ;
#35506=LINE ( 'NONE', #50293, #19499 ) ;
#35508=CARTESIAN_POINT ( 'NONE',  ( -1.339745962155613812, -0.08034179853029406460, -5.000000000000000000 ) ) ;
#35509=CARTESIAN_POINT ( 'NONE',  ( 2.499999999999998668, -66.20833333060213022, -4.330127018922193649 ) ) ;
#35510=DIRECTION ( 'NONE',  ( -0.000000000000000000, 1.000000000000000000, -0.000000000000000000 ) ) ;
#35513=CARTESIAN_POINT ( 'NONE',  ( -4.458734124999998549, -58.22916666530105800, 2.574251347313722516 ) ) ;
#35514=CARTESIAN_POINT ( 'NONE',  ( 4.458734124999999437, -151.6875000013656063, 0.000000000000000000 ) ) ;
#35515=CARTESIAN_POINT ( 'NONE',  ( 2.229367062499998831, -65.64583333196773651, -3.861377020970580887 ) ) ;
#35516=CARTESIAN_POINT ( 'NONE',  ( -2.499999999999996447, -53.70833333060213732, 4.330127018922195425 ) ) ;
#35517=EDGE_LOOP ( 'NONE', ( #55524, #16192, #36861, #8833 ) ) ;
#35519=CARTESIAN_POINT ( 'NONE',  ( 4.458734125000001214, 1.854166668032262155, 2.574251347313718519 ) ) ;
#35523=CARTESIAN_POINT ( 'NONE',  ( -8.190561711645485556E-16, -154.6875000013655779, 4.458734124999999437 ) ) ;
#35526=CARTESIAN_POINT ( 'NONE',  ( 2.499999999999998668, -54.33333333333332860, -4.330127018922193649 ) ) ;
#35528=CARTESIAN_POINT ( 'NONE',  ( 1.339745962155615144, -80.58034179853028434, 4.999999999999999112 ) ) ;
#35529=CARTESIAN_POINT ( 'NONE',  ( 4.458734125000001214, -51.14583333196772941, 2.574251347313718519 ) ) ;
#35530=ORIENTED_EDGE ( 'NONE', *, *, #4362, .T. ) ;
#35534=CARTESIAN_POINT ( 'NONE',  ( -2.229367062500000163, 27.52083333469892779, -3.861377020970580443 ) ) ;
#35542=VECTOR ( 'NONE', #12519, 1000.000000000000000 ) ;
#35543=CARTESIAN_POINT ( 'NONE',  ( -2.499999999999996447, -78.70833333060214443, 4.330127018922195425 ) ) ;
#35544=EDGE_CURVE ( 'NONE', #18022, #41008, #6738, .T. ) ;
#35545=CARTESIAN_POINT ( 'NONE',  ( -9.184850993605147944E-16, -157.3750000027311842, 5.000000000000000000 ) ) ;
#35549=FACE_OUTER_BOUND ( 'NONE', #29926, .T. ) ;
#35550=CARTESIAN_POINT ( 'NONE',  ( -2.229367062499996610, -87.39583333196773651, 3.861377020970582219 ) ) ;
#35553=VERTEX_POINT ( 'NONE', #18039 ) ;
#35554=CARTESIAN_POINT ( 'NONE',  ( 1.975475456537005874E-15, -31.75000000000000000, 5.000000000000000000 ) ) ;
#35556=CARTESIAN_POINT ( 'NONE',  ( -2.071067811865475061, -155.8125000027311842, -5.000000000000000888 ) ) ;
#35557=ORIENTED_EDGE ( 'NONE', *, *, #20106, .F. ) ;
#35561=CARTESIAN_POINT ( 'NONE',  ( -1.339745962155613812, -67.20534180126149693, -5.000000000000000000 ) ) ;
#35567=CARTESIAN_POINT ( 'NONE',  ( -4.458734124999997661, -20.22916666530107221, 2.574251347313722516 ) ) ;
#35568=CARTESIAN_POINT ( 'NONE',  ( -6.972266317189433020E-16, -88.25000000000000000, -5.000000000000000000 ) ) ;
#35569=CARTESIAN_POINT ( 'NONE',  ( -5.000000000000000000, -149.5000000000000284, -6.123233995736766282E-16 ) ) ;
#35571=CARTESIAN_POINT ( 'NONE',  ( 1.846868145590735200, -150.2500000013656063, -4.458734125000000326 ) ) ;
#35573=CARTESIAN_POINT ( 'NONE',  ( -3.152548672688508926E-16, -46.81249999863440792, -5.148502694627439702 ) ) ;
#35574=( BOUNDED_CURVE ( )  B_SPLINE_CURVE ( 2, ( #34172, #10051, #59266, #9729, #1070, #107, #58633, #15198, #29332 ),
 .UNSPECIFIED., .F., .F. ) 
 B_SPLINE_CURVE_WITH_KNOTS ( ( 3, 2, 2, 2, 3 ),
 ( 0.5187500000000000444, 0.5194444444444444864, 0.5208333333333333703, 0.5222222222222222543, 0.5229166666666666963 ),
 .UNSPECIFIED. ) 
 CURVE ( )  GEOMETRIC_REPRESENTATION_ITEM ( )  RATIONAL_B_SPLINE_CURVE ( ( 0.9330127018922194093, 0.9330127018922194093, 1.000000000000000000, 0.8660254037844387076, 1.000000000000000000, 0.8660254037844387076, 1.000000000000000000, 0.9330127018922194093, 0.9330127018922194093 ) ) 
 REPRESENTATION_ITEM ( '' )  );
#35577=CARTESIAN_POINT ( 'NONE',  ( 2.499999999999998668, 27.66666666666666430, -4.330127018922193649 ) ) ;
#35578=CARTESIAN_POINT ( 'NONE',  ( -4.458734124999999437, 5.687500001365592972, 0.000000000000000000 ) ) ;
#35580=CARTESIAN_POINT ( 'NONE',  ( 5.000000000000000888, -41.45833333060214443, 2.886751345948126879 ) ) ;
#35582=CARTESIAN_POINT ( 'NONE',  ( -4.458734124999998549, 14.52083333469892779, 2.574251347313722516 ) ) ;
#35584=CARTESIAN_POINT ( 'NONE',  ( 5.000000000000000000, 9.625000002731184168, -6.123233995736766282E-16 ) ) ;
#35587=EDGE_LOOP ( 'NONE', ( #16226, #779, #20333, #18920 ) ) ;
#35590=CARTESIAN_POINT ( 'NONE',  ( -4.458734124999999437, -41.39583333196773651, -2.574251347313719407 ) ) ;
#35591=CARTESIAN_POINT ( 'NONE',  ( -8.190561711645485556E-16, -168.9375000013656063, 4.458734124999999437 ) ) ;
#35592=VECTOR ( 'NONE', #53366, 1000.000000000000000 ) ;
#35593=AXIS2_PLACEMENT_3D ( 'NONE', #5166, #29594, #34753 ) ;
#35594=CARTESIAN_POINT ( 'NONE',  ( -4.999999999999999112, -39.79166666393547303, 2.886751345948131764 ) ) ;
#35595=VERTEX_POINT ( 'NONE', #18361 ) ;
#35596=CARTESIAN_POINT ( 'NONE',  ( -4.458734124999999437, -20.39583333196774362, -2.574251347313719407 ) ) ;
#35598=CARTESIAN_POINT ( 'NONE',  ( 5.000000000000000888, -86.58333333333334281, 2.886751345948126879 ) ) ;
#35599=DIRECTION ( 'NONE',  ( -0.000000000000000000, 1.000000000000000000, -0.000000000000000000 ) ) ;
#35600=CARTESIAN_POINT ( 'NONE',  ( -2.499999999999996447, -88.70833333060214443, 4.330127018922195425 ) ) ;
#35604=CARTESIAN_POINT ( 'NONE',  ( 2.229367062500001939, -32.22916666530106511, 3.861377020970579999 ) ) ;
#35611=CARTESIAN_POINT ( 'NONE',  ( 3.061616997868383141E-16, -166.8750000027312126, -5.000000000000000000 ) ) ;
#35613=CARTESIAN_POINT ( 'NONE',  ( -4.458734124999999437, -76.64583333196775072, -2.574251347313719407 ) ) ;
#35616=CARTESIAN_POINT ( 'NONE',  ( 3.152801135295367541, -142.5625000013655779, -3.152801135295367541 ) ) ;
#35619=CARTESIAN_POINT ( 'NONE',  ( -2.229367062500000163, -44.47916666530106511, -3.861377020970580443 ) ) ;
#35623=CARTESIAN_POINT ( 'NONE',  ( 3.152801135295366208, -140.8125000013655779, 3.152801135295367985 ) ) ;
#35628=CARTESIAN_POINT ( 'NONE',  ( -4.458734124999998549, -76.47916666530105090, 2.574251347313722516 ) ) ;
#35629=CARTESIAN_POINT ( 'NONE',  ( 3.061616997868383141E-16, -166.7500000000000000, -5.000000000000000000 ) ) ;
#35630=CARTESIAN_POINT ( 'NONE',  ( 2.500000000000002220, 14.45833333606451809, 4.330127018922192761 ) ) ;
#35635=CARTESIAN_POINT ( 'NONE',  ( 5.000000000000000000, 23.70833333606451632, -2.886751345948130876 ) ) ;
#35641=CARTESIAN_POINT ( 'NONE',  ( -2.229367062499996610, 15.60416666803225993, 3.861377020970582219 ) ) ;
#35643=VECTOR ( 'NONE', #22421, 1000.000000000000000 ) ;
#35648=CARTESIAN_POINT ( 'NONE',  ( 1.975475456537005874E-15, -50.62499999726881583, 5.000000000000000000 ) ) ;
#35649=CARTESIAN_POINT ( 'NONE',  ( 2.229367062499998831, -83.64583333196773651, -3.861377020970580887 ) ) ;
#35650=CARTESIAN_POINT ( 'NONE',  ( 4.458734124999998549, -3.729166665301070438, -2.574251347313721627 ) ) ;
#35653=CARTESIAN_POINT ( 'NONE',  ( -4.458734124999999437, -29.56249999863440436, 0.000000000000000000 ) ) ;
#35657=EDGE_CURVE ( 'NONE', #55337, #37963, #26843, .T. ) ;
#35659=CARTESIAN_POINT ( 'NONE',  ( -4.458734124999998549, 18.77083333469893134, 2.574251347313722516 ) ) ;
#35661=CARTESIAN_POINT ( 'NONE',  ( 1.339745962155615144, -66.70534180126148271, 4.999999999999999112 ) ) ;
#35662=CARTESIAN_POINT ( 'NONE',  ( -4.458734124999999437, -76.64583333196775072, -2.574251347313719407 ) ) ;
#35665=CARTESIAN_POINT ( 'NONE',  ( 1.060575238724906964E-15, 24.37500000273118417, 5.773502691896257311 ) ) ;
#35666=ORIENTED_EDGE ( 'NONE', *, *, #58695, .F. ) ;
#35670=CARTESIAN_POINT ( 'NONE',  ( 1.060575238724906964E-15, -23.75000000000000000, 5.773502691896257311 ) ) ;
#35671=CARTESIAN_POINT ( 'NONE',  ( -3.152548672688508926E-16, -27.56249999863440081, -5.148502694627439702 ) ) ;
#35672=CARTESIAN_POINT ( 'NONE',  ( 9.457646018065525792E-16, -90.06249999863440792, 5.148502694627439702 ) ) ;
#35674=CARTESIAN_POINT ( 'NONE',  ( 5.000000000000000000, -25.29166666393547658, -2.886751345948129988 ) ) ;
#35675=CARTESIAN_POINT ( 'NONE',  ( 2.229367062499998831, -54.64583333196773651, -3.861377020970580887 ) ) ;
#35678=CARTESIAN_POINT ( 'NONE',  ( -4.458734124999999437, -1.562499998634406140, 0.000000000000000000 ) ) ;
#35681=CARTESIAN_POINT ( 'NONE',  ( 1.060575238724906964E-15, -64.75000000000000000, 5.773502691896257311 ) ) ;
#35682=CARTESIAN_POINT ( 'NONE',  ( 2.730187237215162345E-16, -150.4375000013656063, -4.458734124999999437 ) ) ;
#35684=CARTESIAN_POINT ( 'NONE',  ( -4.999999999999998224, -76.79166666393547303, 2.886751345948131764 ) ) ;
#35686=CARTESIAN_POINT ( 'NONE',  ( -3.535533905932737309, -157.6250000000000284, -3.535533905932738197 ) ) ;
#35689=CARTESIAN_POINT ( 'NONE',  ( -3.152548672688508926E-16, -9.812499998634406140, -5.148502694627439702 ) ) ;
#35690=AXIS2_PLACEMENT_3D ( 'NONE', #58164, #53024, #47874 ) ;
#35691=CARTESIAN_POINT ( 'NONE',  ( 2.229367062500001939, -52.22916666530107221, 3.861377020970579999 ) ) ;
#35693=CARTESIAN_POINT ( 'NONE',  ( -3.152801135295367985, -143.8125000013655779, 3.152801135295367096 ) ) ;
#35696=ORIENTED_EDGE ( 'NONE', *, *, #63342, .T. ) ;
#35698=CARTESIAN_POINT ( 'NONE',  ( -4.458734124999999437, 27.35416666803225993, -2.574251347313719407 ) ) ;
#35702=DIRECTION ( 'NONE',  ( -0.000000000000000000, 1.000000000000000000, -0.000000000000000000 ) ) ;
#35704=CARTESIAN_POINT ( 'NONE',  ( 1.975475456537005874E-15, 9.250000000000000000, 5.000000000000000000 ) ) ;
#35705=CARTESIAN_POINT ( 'NONE',  ( 9.457646018065525792E-16, -7.062499998634404363, 5.148502694627439702 ) ) ;
#35707=CARTESIAN_POINT ( 'NONE',  ( -4.458734124999999437, -149.9375000013656063, -5.460374474430324690E-16 ) ) ;
#35714=CARTESIAN_POINT ( 'NONE',  ( 5.000000000000000888, 1.541666669397853795, 2.886751345948126879 ) ) ;
#35717=CARTESIAN_POINT ( 'NONE',  ( 0.000000000000000000, -170.0000000000000000, 5.000000000000000000 ) ) ;
#35719=DIRECTION ( 'NONE',  ( 0.000000000000000000, 0.000000000000000000, 1.000000000000000000 ) ) ;
#35720=DIRECTION ( 'NONE',  ( 0.000000000000000000, 0.000000000000000000, 1.000000000000000000 ) ) ;
#35721=CARTESIAN_POINT ( 'NONE',  ( 9.457646018065525792E-16, 11.93750000136559564, 5.148502694627439702 ) ) ;
#35723=CARTESIAN_POINT ( 'NONE',  ( -3.152548672688508926E-16, -12.81249999863440259, -5.148502694627439702 ) ) ;
#35724=( BOUNDED_CURVE ( )  B_SPLINE_CURVE ( 2, ( #61217, #40628, #60271, #16189, #17142, #35816, #36766, #55440, #31933 ),
 .UNSPECIFIED., .F., .F. ) 
 B_SPLINE_CURVE_WITH_KNOTS ( ( 3, 2, 2, 2, 3 ),
 ( 0.7229166666666666519, 0.7236111111111110938, 0.7249999999999999778, 0.7263888888888888618, 0.7270833333333333037 ),
 .UNSPECIFIED. ) 
 CURVE ( )  GEOMETRIC_REPRESENTATION_ITEM ( )  RATIONAL_B_SPLINE_CURVE ( ( 0.9330127018922194093, 0.9330127018922194093, 1.000000000000000000, 0.8660254037844387076, 1.000000000000000000, 0.8660254037844387076, 1.000000000000000000, 0.9330127018922194093, 0.9330127018922194093 ) ) 
 REPRESENTATION_ITEM ( '' )  );
#35726=CARTESIAN_POINT ( 'NONE',  ( -4.458734125000001214, -162.8750000013655779, 1.846868145590734089 ) ) ;
#35727=CARTESIAN_POINT ( 'NONE',  ( -2.499999999999996447, -40.70833333060214443, 4.330127018922195425 ) ) ;
#35731=VECTOR ( 'NONE', #11351, 1000.000000000000000 ) ;
#35733=LINE ( 'NONE', #46333, #39836 ) ;
#35735=CARTESIAN_POINT ( 'NONE',  ( 2.229367062499998831, -34.64583333196772941, -3.861377020970580887 ) ) ;
#35736=CARTESIAN_POINT ( 'NONE',  ( 1.339745962155615144, -51.58034179853028434, 4.999999999999999112 ) ) ;
#35743=CARTESIAN_POINT ( 'NONE',  ( 6.123233995736766282E-16, -170.0000000000000000, -5.000000000000000000 ) ) ;
#35744=CARTESIAN_POINT ( 'NONE',  ( 5.000000000000000000, -3.500000000000003109, -6.123233995736766282E-16 ) ) ;
#35746=CARTESIAN_POINT ( 'NONE',  ( 2.229367062499998831, -69.64583333196773651, -3.861377020970580887 ) ) ;
#35747=CARTESIAN_POINT ( 'NONE',  ( -4.999999999999999112, -5.791666663935480130, 2.886751345948131764 ) ) ;
#35748=CARTESIAN_POINT ( 'NONE',  ( 4.458734125000001214, -40.89583333196773651, 2.574251347313718519 ) ) ;
#35752=CARTESIAN_POINT ( 'NONE',  ( 9.457646018065525792E-16, 9.687500001365593860, 5.148502694627439702 ) ) ;
#35753=ORIENTED_EDGE ( 'NONE', *, *, #9074, .F. ) ;
#35755=CARTESIAN_POINT ( 'NONE',  ( -5.000000000000000000, -51.00000000000000711, 0.000000000000000000 ) ) ;
#35757=CARTESIAN_POINT ( 'NONE',  ( -1.339745962155613812, -42.08034179853029144, -5.000000000000000000 ) ) ;
#35758=CARTESIAN_POINT ( 'NONE',  ( 2.229367062500001939, -74.97916666530106511, 3.861377020970579999 ) ) ;
#35759=CARTESIAN_POINT ( 'NONE',  ( -2.071067811865475061, -169.6875000000000284, -5.000000000000000888 ) ) ;
#35760=CARTESIAN_POINT ( 'NONE',  ( 2.229367062500001939, -79.97916666530106511, 3.861377020970579999 ) ) ;
#35762=ADVANCED_FACE ( 'NONE', ( #13221 ), #53400, .T. ) ;
#35763=CARTESIAN_POINT ( 'NONE',  ( -4.458734124999998549, -35.47916666530107221, 2.574251347313722516 ) ) ;
#35764=ORIENTED_EDGE ( 'NONE', *, *, #28667, .F. ) ;
#35765=CARTESIAN_POINT ( 'NONE',  ( -1.339745962155608039, 23.91965820146970501, -5.000000000000004441 ) ) ;
#35766=ORIENTED_EDGE ( 'NONE', *, *, #44364, .F. ) ;
#35768=CARTESIAN_POINT ( 'NONE',  ( -6.972266317189433020E-16, 21.87500000273118417, -5.000000000000000000 ) ) ;
#35773=CARTESIAN_POINT ( 'NONE',  ( 2.229367062500001939, -65.22916666530106511, 3.861377020970579999 ) ) ;
#35774=VECTOR ( 'NONE', #29615, 1000.000000000000000 ) ;
#35776=ORIENTED_EDGE ( 'NONE', *, *, #17576, .F. ) ;
#35777=CARTESIAN_POINT ( 'NONE',  ( 5.000000000000000888, 3.541666669397852019, 2.886751345948126879 ) ) ;
#35779=ORIENTED_EDGE ( 'NONE', *, *, #56962, .T. ) ;
#35782=CARTESIAN_POINT ( 'NONE',  ( 9.457646018065525792E-16, 9.937500001365592084, 5.148502694627439702 ) ) ;
#35783=CARTESIAN_POINT ( 'NONE',  ( 3.061616997868383141E-16, -153.7500000000000000, -5.000000000000000000 ) ) ;
#35784=CARTESIAN_POINT ( 'NONE',  ( -1.846868145590734756, -162.1250000013656347, -4.458734124999999437 ) ) ;
#35786=ORIENTED_EDGE ( 'NONE', *, *, #16092, .F. ) ;
#35788=CARTESIAN_POINT ( 'NONE',  ( 3.535533905932736864, -164.2500000027312126, 3.535533905932738641 ) ) ;
#35790=CYLINDRICAL_SURFACE ( 'NONE', #4669, 5.000000000000000000 ) ;
#35791=CARTESIAN_POINT ( 'NONE',  ( -2.500000000000000444, -68.16666666666667140, -4.330127018922193649 ) ) ;
#35797=CARTESIAN_POINT ( 'NONE',  ( 1.975475456537005874E-15, -82.62499999726878741, 5.000000000000000000 ) ) ;
#35800=CARTESIAN_POINT ( 'NONE',  ( 4.458734124999999437, 3.937500001365595192, -5.460374474430324690E-16 ) ) ;
#35803=CARTESIAN_POINT ( 'NONE',  ( -5.000000000000000888, -143.6875000027312126, -2.071067811865475949 ) ) ;
#35808=CARTESIAN_POINT ( 'NONE',  ( 2.071067811865475505, -140.8125000000000000, -5.000000000000000888 ) ) ;
#35813=CARTESIAN_POINT ( 'NONE',  ( -3.152801135295367096, -162.3125000013656063, -3.152801135295367541 ) ) ;
#35814=CARTESIAN_POINT ( 'NONE',  ( 1.975475456537005874E-15, -59.62499999726880873, 5.000000000000000000 ) ) ;
#35816=CARTESIAN_POINT ( 'NONE',  ( -5.000000000000000000, -57.08333333333333570, -2.886751345948128211 ) ) ;
#35817=ORIENTED_EDGE ( 'NONE', *, *, #38479, .T. ) ;
#35818=CARTESIAN_POINT ( 'NONE',  ( -3.152548672688508926E-16, 24.18750000136559564, -5.148502694627439702 ) ) ;
#35819=ORIENTED_EDGE ( 'NONE', *, *, #37063, .F. ) ;
#35820=VECTOR ( 'NONE', #2025, 1000.000000000000000 ) ;
#35822=DIRECTION ( 'NONE',  ( 0.000000000000000000, 0.000000000000000000, 1.000000000000000000 ) ) ;
#35823=CARTESIAN_POINT ( 'NONE',  ( 5.000000000000000000, 15.50000000000000000, -6.123233995736766282E-16 ) ) ;
#35825=EDGE_CURVE ( 'NONE', #11293, #32107, #44465, .T. ) ;
#35826=CARTESIAN_POINT ( 'NONE',  ( 4.458734125000000326, -50.89583333196772230, 2.574251347313718519 ) ) ;
#35827=CARTESIAN_POINT ( 'NONE',  ( -2.229367062499996610, -10.14583333196773829, 3.861377020970582219 ) ) ;
#35830=CARTESIAN_POINT ( 'NONE',  ( -5.000000000000000000, -37.08333333333332860, -2.886751345948128211 ) ) ;
#35833=CARTESIAN_POINT ( 'NONE',  ( -4.999999999999999112, -31.91666666666666430, 2.886751345948131764 ) ) ;
#35834=FACE_OUTER_BOUND ( 'NONE', #50322, .T. ) ;
#35835=CARTESIAN_POINT ( 'NONE',  ( -4.999999999999998224, -33.91666666666666430, 2.886751345948131764 ) ) ;
#35837=CARTESIAN_POINT ( 'NONE',  ( -3.535533905932737309, -140.7500000027311842, -3.535533905932738197 ) ) ;
#35838=CARTESIAN_POINT ( 'NONE',  ( -4.458734124999998549, -61.22916666530106511, 2.574251347313722516 ) ) ;
#35839=CARTESIAN_POINT ( 'NONE',  ( -1.846868145590737420, -151.0000000013656063, 4.458734124999999437 ) ) ;
#35840=CARTESIAN_POINT ( 'NONE',  ( -3.152548672688508926E-16, -63.56249999863440792, -5.148502694627439702 ) ) ;
#35841=CARTESIAN_POINT ( 'NONE',  ( 5.000000000000000000, -57.37499999726880162, -6.123233995736766282E-16 ) ) ;
#35842=ORIENTED_EDGE ( 'NONE', *, *, #34943, .T. ) ;
#35844=VERTEX_POINT ( 'NONE', #989 ) ;
#35847=CARTESIAN_POINT ( 'NONE',  ( -3.152801135295367096, -153.0625000013656063, -3.152801135295367541 ) ) ;
#35849=CARTESIAN_POINT ( 'NONE',  ( -9.184850993605147944E-16, -169.2500000000000000, 5.000000000000000000 ) ) ;
#35851=CARTESIAN_POINT ( 'NONE',  ( 5.000000000000000888, -161.0625000027312126, -2.071067811865475505 ) ) ;
#35852=CARTESIAN_POINT ( 'NONE',  ( -4.458734124999998549, -47.47916666530106511, 2.574251347313722516 ) ) ;
#35853=EDGE_LOOP ( 'NONE', ( #58573, #11631, #61859, #24679 ) ) ;
#35854=( BOUNDED_CURVE ( )  B_SPLINE_CURVE ( 2, ( #25325, #15359, #30459, #6041, #54599, #10521, #19540, #43973, #63619 ),
 .UNSPECIFIED., .F., .F. ) 
 B_SPLINE_CURVE_WITH_KNOTS ( ( 3, 2, 2, 2, 3 ),
 ( 0.05625000000000000139, 0.05694444444444444337, 0.05833333333333333426, 0.05972222222222222515, 0.06041666666666666713 ),
 .UNSPECIFIED. ) 
 CURVE ( )  GEOMETRIC_REPRESENTATION_ITEM ( )  RATIONAL_B_SPLINE_CURVE ( ( 0.9330127018922192983, 0.9330127018922196314, 1.000000000000000000, 0.8660254037844387076, 1.000000000000000000, 0.8660254037844387076, 1.000000000000000000, 0.9330127018922194093, 0.9330127018922194093 ) ) 
 REPRESENTATION_ITEM ( '' )  );
#35855=CARTESIAN_POINT ( 'NONE',  ( -1.339745962155613812, 16.91965820146970145, -5.000000000000000000 ) ) ;
#35857=CARTESIAN_POINT ( 'NONE',  ( -4.458734124999999437, 22.60416666803225993, -2.574251347313719407 ) ) ;
#35861=AXIS2_PLACEMENT_3D ( 'NONE', #62951, #22460, #51726 ) ;
#35864=CARTESIAN_POINT ( 'NONE',  ( 1.975475456537005874E-15, -28.62499999726881583, 5.000000000000000000 ) ) ;
#35870=DIRECTION ( 'NONE',  ( 0.000000000000000000, 0.000000000000000000, 1.000000000000000000 ) ) ;
#35871=CARTESIAN_POINT ( 'NONE',  ( 2.500000000000002220, -87.66666666666667140, 4.330127018922192761 ) ) ;
#35874=VERTEX_POINT ( 'NONE', #35373 ) ;
#35875=CARTESIAN_POINT ( 'NONE',  ( -3.535533905932738641, -143.5000000027311842, 3.535533905932737309 ) ) ;
#35877=CARTESIAN_POINT ( 'NONE',  ( 5.000000000000000888, -158.0625000027312126, -2.071067811865475505 ) ) ;
#35878=EDGE_LOOP ( 'NONE', ( #28811, #985, #11238, #23594 ) ) ;
#35884=EDGE_CURVE ( 'NONE', #20081, #38026, #22713, .T. ) ;
#35888=CARTESIAN_POINT ( 'NONE',  ( 9.457646018065525792E-16, -21.06249999863440436, 5.148502694627439702 ) ) ;
#35890=CARTESIAN_POINT ( 'NONE',  ( -3.535533905932737309, -151.6250000000000000, -3.535533905932738197 ) ) ;
#35892=CARTESIAN_POINT ( 'NONE',  ( -4.458734125000000326, -153.0000000013656063, -1.846868145590735644 ) ) ;
#35894=CARTESIAN_POINT ( 'NONE',  ( 4.458734124999998549, -44.97916666530107221, -2.574251347313721627 ) ) ;
#35896=CARTESIAN_POINT ( 'NONE',  ( -5.000000000000000000, 27.00000000000000000, 0.000000000000000000 ) ) ;
#35897=CARTESIAN_POINT ( 'NONE',  ( 4.458734125000001214, 6.104166668032262599, 2.574251347313718519 ) ) ;
#35898=CARTESIAN_POINT ( 'NONE',  ( -6.972266317189433020E-16, -74.12499999726878741, -5.000000000000000000 ) ) ;
#35899=CARTESIAN_POINT ( 'NONE',  ( 1.339745962155615144, -37.58034179853029144, 4.999999999999999112 ) ) ;
#35900=CARTESIAN_POINT ( 'NONE',  ( -6.972266317189433020E-16, -82.24999999999998579, -5.000000000000000000 ) ) ;
#35901=CARTESIAN_POINT ( 'NONE',  ( 2.229367062500001939, 13.77083333469892779, 3.861377020970579999 ) ) ;
#35903=( BOUNDED_CURVE ( )  B_SPLINE_CURVE ( 2, ( #51338, #15957, #21102, #56158, #21749, #61304, #55839, #46505, #6628 ),
 .UNSPECIFIED., .F., .F. ) 
 B_SPLINE_CURVE_WITH_KNOTS ( ( 3, 2, 2, 2, 3 ),
 ( 0.9083333333333332149, 0.9124999999999998668, 0.9166666666666665186, 0.9208333333333330595, 0.9249999999999998224 ),
 .UNSPECIFIED. ) 
 CURVE ( )  GEOMETRIC_REPRESENTATION_ITEM ( )  RATIONAL_B_SPLINE_CURVE ( ( 1.000000000000001998, 0.9238795325112847401, 1.000000000000000000, 0.9238795325112867385, 1.000000000000000000, 0.9238795325112867385, 1.000000000000000000, 0.9238795325112908463, 0.9999999999999958922 ) ) 
 REPRESENTATION_ITEM ( '' )  );
#35904=CARTESIAN_POINT ( 'NONE',  ( -5.000000000000000000, 10.12500000273118594, 0.000000000000000000 ) ) ;
#35906=VERTEX_POINT ( 'NONE', #20264 ) ;
#35907=CARTESIAN_POINT ( 'NONE',  ( 2.071067811865550556, -162.3125000027312410, 4.999999999999925393 ) ) ;
#35910=CARTESIAN_POINT ( 'NONE',  ( -2.229367062500000163, -45.47916666530106511, -3.861377020970580443 ) ) ;
#35911=EDGE_CURVE ( 'NONE', #11571, #4948, #31329, .T. ) ;
#35912=CARTESIAN_POINT ( 'NONE',  ( 2.730187237215162345E-16, -165.4375000013655779, -4.458734124999999437 ) ) ;
#35915=CARTESIAN_POINT ( 'NONE',  ( -2.500000000000000444, -42.04166666393548013, -4.330127018922193649 ) ) ;
#35916=ORIENTED_EDGE ( 'NONE', *, *, #15431, .T. ) ;
#35917=CARTESIAN_POINT ( 'NONE',  ( -4.458734124999999437, -16.31249999863440436, 0.000000000000000000 ) ) ;
#35919=CARTESIAN_POINT ( 'NONE',  ( -3.535250795749689387E-16, -87.24999999999998579, -5.773502691896257311 ) ) ;
#35920=CARTESIAN_POINT ( 'NONE',  ( 4.458734124999999437, -167.5000000013655779, 1.846868145590737864 ) ) ;
#35921=CARTESIAN_POINT ( 'NONE',  ( 1.060575238724906964E-15, -86.62499999726881583, 5.773502691896257311 ) ) ;
#35922=CARTESIAN_POINT ( 'NONE',  ( 5.000000000000000000, -20.29166666393548368, -2.886751345948130876 ) ) ;
#35923=ORIENTED_EDGE ( 'NONE', *, *, #61113, .T. ) ;
#35925=CARTESIAN_POINT ( 'NONE',  ( -4.458734124999999437, -30.56249999863440436, 0.000000000000000000 ) ) ;
#35926=CARTESIAN_POINT ( 'NONE',  ( -1.049326080737009628E-13, -5.624999997268816720, 5.000000000000000000 ) ) ;
#35927=ORIENTED_EDGE ( 'NONE', *, *, #24714, .F. ) ;
#35932=ORIENTED_EDGE ( 'NONE', *, *, #7570, .F. ) ;
#35933=CARTESIAN_POINT ( 'NONE',  ( -2.500000000000000444, -26.16666666666666430, -4.330127018922193649 ) ) ;
#35935=CARTESIAN_POINT ( 'NONE',  ( 4.458734124999998549, -81.97916666530106511, -2.574251347313721627 ) ) ;
#35938=CARTESIAN_POINT ( 'NONE',  ( -3.152801135295367985, -143.0625000013655779, 3.152801135295367096 ) ) ;
#35939=CARTESIAN_POINT ( 'NONE',  ( -1.339745962155613812, -58.20534180126147561, -5.000000000000000000 ) ) ;
#35941=CARTESIAN_POINT ( 'NONE',  ( -3.152548672688508926E-16, -43.56249999863439371, -5.148502694627439702 ) ) ;
#35945=CARTESIAN_POINT ( 'NONE',  ( 4.458734124999999437, -140.7500000013655779, 1.846868145590737864 ) ) ;
#35950=CARTESIAN_POINT ( 'NONE',  ( -3.152548672688508926E-16, -77.81249999863440792, -5.148502694627439702 ) ) ;
#35952=CARTESIAN_POINT ( 'NONE',  ( 1.975475456537005874E-15, -76.75000000000000000, 5.000000000000000000 ) ) ;
#35958=CARTESIAN_POINT ( 'NONE',  ( -1.339745962155613812, -60.20534180126147561, -5.000000000000000000 ) ) ;
#35960=CARTESIAN_POINT ( 'NONE',  ( -2.499999999999996447, -4.833333333333335702, 4.330127018922195425 ) ) ;
#35962=CARTESIAN_POINT ( 'NONE',  ( -4.458734124999999437, 18.35416666803225993, -2.574251347313719407 ) ) ;
#35968=CARTESIAN_POINT ( 'NONE',  ( 5.000000000000000000, -38.29166666393548013, -2.886751345948130876 ) ) ;
#35969=CARTESIAN_POINT ( 'NONE',  ( 2.229367062499998831, -86.64583333196773651, -3.861377020970580887 ) ) ;
#35970=CARTESIAN_POINT ( 'NONE',  ( 9.457646018065525792E-16, -5.062499998634402587, 5.148502694627439702 ) ) ;
#35971=CARTESIAN_POINT ( 'NONE',  ( -2.500000000000000444, -31.16666666666666785, -4.330127018922193649 ) ) ;
#35973=CARTESIAN_POINT ( 'NONE',  ( -2.229367062500000163, -31.72916666530107577, -3.861377020970580443 ) ) ;
#35977=CARTESIAN_POINT ( 'NONE',  ( 4.458734124999999437, 22.18750000136559564, -5.460374474430324690E-16 ) ) ;
#35979=CARTESIAN_POINT ( 'NONE',  ( 5.000000000000000000, -28.41666666666666430, -2.886751345948130876 ) ) ;
#35980=CARTESIAN_POINT ( 'NONE',  ( -4.458734124999997661, -79.47916666530106511, 2.574251347313722516 ) ) ;
#35983=CARTESIAN_POINT ( 'NONE',  ( 5.000000000000000888, 22.54166666939784847, 2.886751345948126879 ) ) ;
#35987=CARTESIAN_POINT ( 'NONE',  ( 2.500000000000002220, -22.66666666666666785, 4.330127018922192761 ) ) ;
#35988=CARTESIAN_POINT ( 'NONE',  ( 4.458734125000001214, -26.89583333196774007, 2.574251347313718519 ) ) ;
#35989=CARTESIAN_POINT ( 'NONE',  ( 4.458734124999998549, -87.72916666530107932, -2.574251347313721627 ) ) ;
#35990=CARTESIAN_POINT ( 'NONE',  ( -5.000000000000000000, -22.87499999726881228, 0.000000000000000000 ) ) ;
#35991=CARTESIAN_POINT ( 'NONE',  ( -4.458734124999998549, -54.22916666530107221, 2.574251347313722516 ) ) ;
#35993=CARTESIAN_POINT ( 'NONE',  ( 1.062108568985190270E-13, -27.25000000000000000, -4.999999999999999112 ) ) ;
#35995=CARTESIAN_POINT ( 'NONE',  ( 2.229367062500001939, -2.229166665301068662, 3.861377020970579999 ) ) ;
#35997=CARTESIAN_POINT ( 'NONE',  ( 5.000000000000000000, -71.50000000000000000, -6.123233995736766282E-16 ) ) ;
#35998=CARTESIAN_POINT ( 'NONE',  ( 4.458734124999999437, -152.6875000013656063, 0.000000000000000000 ) ) ;
#36002=CARTESIAN_POINT ( 'NONE',  ( 5.000000000000000000, -158.0000000000000000, 0.000000000000000000 ) ) ;
#36005=CARTESIAN_POINT ( 'NONE',  ( -4.458734124999999437, -16.56249999863440436, 0.000000000000000000 ) ) ;
#36006=CARTESIAN_POINT ( 'NONE',  ( 4.458734125000001214, -49.14583333196772941, 2.574251347313718519 ) ) ;
#36008=CARTESIAN_POINT ( 'NONE',  ( 4.458734125000000326, -143.3750000013656063, -1.846868145590734978 ) ) ;
#36011=ORIENTED_EDGE ( 'NONE', *, *, #56752, .F. ) ;
#36013=CARTESIAN_POINT ( 'NONE',  ( -2.229367062500000163, 27.27083333469892779, -3.861377020970580443 ) ) ;
#36015=DIRECTION ( 'NONE',  ( -0.000000000000000000, 1.000000000000000000, -0.000000000000000000 ) ) ;
#36021=CARTESIAN_POINT ( 'NONE',  ( 4.458734124999998549, -7.729166665301073103, -2.574251347313721627 ) ) ;
#36022=CARTESIAN_POINT ( 'NONE',  ( 1.339745962155615144, 6.419658201469706782, 4.999999999999999112 ) ) ;
#36023=CARTESIAN_POINT ( 'NONE',  ( -1.846868145590737420, -144.7500000013655779, 4.458734124999997661 ) ) ;
#36027=CARTESIAN_POINT ( 'NONE',  ( 3.061616997868383141E-16, -168.8750000027312126, -5.000000000000000000 ) ) ;
#36030=CARTESIAN_POINT ( 'NONE',  ( 2.500000000000002220, -25.54166666393547658, 4.330127018922192761 ) ) ;
#36031=LINE ( 'NONE', #25419, #29356 ) ;
#36035=CARTESIAN_POINT ( 'NONE',  ( 5.000000000000000000, -150.1875000027312126, 2.071067811865478614 ) ) ;
#36038=CARTESIAN_POINT ( 'NONE',  ( 1.339745962155612702, 9.705341801261479162, -5.000000000000000000 ) ) ;
#36039=CARTESIAN_POINT ( 'NONE',  ( 2.229367062499998831, 13.35416666803226171, -3.861377020970580887 ) ) ;
#36041=AXIS2_PLACEMENT_3D ( 'NONE', #34277, #38475, #19807 ) ;
#36042=CARTESIAN_POINT ( 'NONE',  ( 4.458734124999998549, -15.97916666530107221, -2.574251347313721627 ) ) ;
#36044=CARTESIAN_POINT ( 'NONE',  ( 1.846868145590736310, -162.6250000013655779, 4.458734124999999437 ) ) ;
#36046=VECTOR ( 'NONE', #20875, 1000.000000000000000 ) ;
#36051=CARTESIAN_POINT ( 'NONE',  ( -1.339745962155613812, -89.08034179853027013, -5.000000000000000000 ) ) ;
#36052=CARTESIAN_POINT ( 'NONE',  ( 2.229367062499998831, -37.64583333196773651, -3.861377020970580887 ) ) ;
#36053=DIRECTION ( 'NONE',  ( -0.000000000000000000, 1.000000000000000000, -0.000000000000000000 ) ) ;
#36061=CARTESIAN_POINT ( 'NONE',  ( -5.000000000000000000, -9.000000000000001776, 0.000000000000000000 ) ) ;
#36062=CARTESIAN_POINT ( 'NONE',  ( -2.229367062500000163, -72.47916666530107932, -3.861377020970580443 ) ) ;
#36063=CARTESIAN_POINT ( 'NONE',  ( -5.000000000000000000, -17.08333333333333215, -2.886751345948128211 ) ) ;
#36064=CARTESIAN_POINT ( 'NONE',  ( 1.060575238724906964E-15, -6.624999997268813168, 5.773502691896257311 ) ) ;
#36065=CARTESIAN_POINT ( 'NONE',  ( -4.458734124999999437, -39.31249999863440081, 0.000000000000000000 ) ) ;
#36066=ORIENTED_EDGE ( 'NONE', *, *, #47312, .F. ) ;
#36067=DIRECTION ( 'NONE',  ( 0.000000000000000000, 0.000000000000000000, 1.000000000000000000 ) ) ;
#36068=CARTESIAN_POINT ( 'NONE',  ( 4.458734124999998549, 13.02083333469892779, -2.574251347313721627 ) ) ;
#36071=CARTESIAN_POINT ( 'NONE',  ( -2.499999999999996447, -55.83333333333332860, 4.330127018922195425 ) ) ;
#36073=CARTESIAN_POINT ( 'NONE',  ( -6.972266317189433020E-16, -4.249999999999997335, -5.000000000000000000 ) ) ;
#36074=CARTESIAN_POINT ( 'NONE',  ( 2.229367062500001939, -76.97916666530106511, 3.861377020970579999 ) ) ;
#36075=CARTESIAN_POINT ( 'NONE',  ( 1.846868145590736310, -140.8750000013656063, 4.458734124999999437 ) ) ;
#36076=CARTESIAN_POINT ( 'NONE',  ( -3.152548672688508926E-16, -88.56249999863439371, -5.148502694627439702 ) ) ;
#36078=CARTESIAN_POINT ( 'NONE',  ( 4.458734124999999437, -38.06249999863440792, -5.460374474430324690E-16 ) ) ;
#36080=ORIENTED_EDGE ( 'NONE', *, *, #54346, .T. ) ;
#36083=ORIENTED_EDGE ( 'NONE', *, *, #6265, .T. ) ;
#36085=DIRECTION ( 'NONE',  ( 0.000000000000000000, 0.000000000000000000, 1.000000000000000000 ) ) ;
#36087=CARTESIAN_POINT ( 'NONE',  ( -3.152548672688508926E-16, -62.81249999863440792, -5.148502694627439702 ) ) ;
#36088=ADVANCED_FACE ( 'NONE', ( #39863 ), #25730, .T. ) ;
#36095=CARTESIAN_POINT ( 'NONE',  ( -2.229367062500000163, 8.520833334698926009, -3.861377020970580443 ) ) ;
#36096=CARTESIAN_POINT ( 'NONE',  ( -6.972266317189433020E-16, -33.12499999726880873, -5.000000000000000000 ) ) ;
#36097=CARTESIAN_POINT ( 'NONE',  ( -1.846868145590737420, -162.7500000013655779, 4.458734124999997661 ) ) ;
#36098=( BOUNDED_CURVE ( )  B_SPLINE_CURVE ( 2, ( #7968, #62313, #27258, #23392, #46569, #52961, #42674, #7654, #18238 ),
 .UNSPECIFIED., .F., .F. ) 
 B_SPLINE_CURVE_WITH_KNOTS ( ( 3, 2, 2, 2, 3 ),
 ( 0.1020833333333333315, 0.1027777777777777735, 0.1041666666666666713, 0.1055555555555555552, 0.1062499999999999972 ),
 .UNSPECIFIED. ) 
 CURVE ( )  GEOMETRIC_REPRESENTATION_ITEM ( )  RATIONAL_B_SPLINE_CURVE ( ( 0.9330127018922194093, 0.9330127018922194093, 1.000000000000000000, 0.8660254037844387076, 1.000000000000000000, 0.8660254037844387076, 1.000000000000000000, 0.9330127018922194093, 0.9330127018922194093 ) ) 
 REPRESENTATION_ITEM ( '' )  );
#36104=CARTESIAN_POINT ( 'NONE',  ( 0.000000000000000000, -170.0000000000000000, 0.000000000000000000 ) ) ;
#36105=ADVANCED_FACE ( 'NONE', ( #17345 ), #51132, .T. ) ;
#36107=ADVANCED_FACE ( 'NONE', ( #7705 ), #26046, .T. ) ;
#36108=DIRECTION ( 'NONE',  ( -0.000000000000000000, 1.000000000000000000, -0.000000000000000000 ) ) ;
#36110=CARTESIAN_POINT ( 'NONE',  ( -2.499999999999996447, -82.70833333060214443, 4.330127018922195425 ) ) ;
#36111=CARTESIAN_POINT ( 'NONE',  ( 2.229367062499998831, 26.35416666803225993, -3.861377020970580887 ) ) ;
#36114=CARTESIAN_POINT ( 'NONE',  ( 2.229367062499998831, 3.104166668032259935, -3.861377020970580887 ) ) ;
#36115=CARTESIAN_POINT ( 'NONE',  ( -4.764381983412779477E-15, 25.37500000273118062, 5.000000000000000000 ) ) ;
#36117=CARTESIAN_POINT ( 'NONE',  ( 5.000000000000000000, -145.1875000027312126, 2.071067811865478614 ) ) ;
#36118=CARTESIAN_POINT ( 'NONE',  ( 1.975475456537005874E-15, 18.37500000273118062, 5.000000000000000000 ) ) ;
#36121=EDGE_CURVE ( 'NONE', #12871, #8173, #29247, .T. ) ;
#36124=CARTESIAN_POINT ( 'NONE',  ( 1.975475456537005874E-15, -22.74999999999999645, 5.000000000000000000 ) ) ;
#36126=CARTESIAN_POINT ( 'NONE',  ( -1.846868145590734756, -163.3750000013656347, -4.458734124999999437 ) ) ;
#36129=CARTESIAN_POINT ( 'NONE',  ( 3.152801135295367541, -140.3125000013655779, -3.152801135295367541 ) ) ;
#36131=CARTESIAN_POINT ( 'NONE',  ( 4.458734124999999437, 24.93750000136559208, -5.460374474430324690E-16 ) ) ;
#36132=ORIENTED_EDGE ( 'NONE', *, *, #40432, .T. ) ;
#36135=( BOUNDED_CURVE ( )  B_SPLINE_CURVE ( 2, ( #50295, #59965, #6878, #1433, #60602, #20395, #31300, #30347, #39994 ),
 .UNSPECIFIED., .F., .F. ) 
 B_SPLINE_CURVE_WITH_KNOTS ( ( 3, 2, 2, 2, 3 ),
 ( 0.1312500000000000056, 0.1319444444444444475, 0.1333333333333333315, 0.1347222222222222154, 0.1354166666666666574 ),
 .UNSPECIFIED. ) 
 CURVE ( )  GEOMETRIC_REPRESENTATION_ITEM ( )  RATIONAL_B_SPLINE_CURVE ( ( 0.9330127018922194093, 0.9330127018922194093, 1.000000000000000000, 0.8660254037844387076, 1.000000000000000000, 0.8660254037844387076, 1.000000000000000000, 0.9330127018922194093, 0.9330127018922194093 ) ) 
 REPRESENTATION_ITEM ( '' )  );
#36137=FACE_OUTER_BOUND ( 'NONE', #41359, .T. ) ;
#36138=CARTESIAN_POINT ( 'NONE',  ( -2.500000000000000444, 6.833333333333333925, -4.330127018922193649 ) ) ;
#36139=CARTESIAN_POINT ( 'NONE',  ( 2.229367062499998831, -57.64583333196773651, -3.861377020970580887 ) ) ;
#36140=CARTESIAN_POINT ( 'NONE',  ( -3.152548672688508926E-16, -13.56249999863440259, -5.148502694627439702 ) ) ;
#36144=CARTESIAN_POINT ( 'NONE',  ( -5.000000000000000000, -63.95833333060213732, -2.886751345948128211 ) ) ;
#36146=LINE ( 'NONE', #6557, #26868 ) ;
#36147=CARTESIAN_POINT ( 'NONE',  ( -4.999999999999999112, -36.91666666666667140, 2.886751345948131764 ) ) ;
#36149=CARTESIAN_POINT ( 'NONE',  ( -2.499999999999996447, 15.16666666666666607, 4.330127018922195425 ) ) ;
#36152=CARTESIAN_POINT ( 'NONE',  ( 9.457646018065525792E-16, -62.06249999863440792, 5.148502694627439702 ) ) ;
#36153=( BOUNDED_CURVE ( )  B_SPLINE_CURVE ( 2, ( #54214, #30403, #24952, #514, #5982, #25589, #20769, #35561, #1169 ),
 .UNSPECIFIED., .F., .F. ) 
 B_SPLINE_CURVE_WITH_KNOTS ( ( 3, 2, 2, 2, 3 ),
 ( 0.8062500000000000222, 0.8069444444444444642, 0.8083333333333333481, 0.8097222222222222321, 0.8104166666666666741 ),
 .UNSPECIFIED. ) 
 CURVE ( )  GEOMETRIC_REPRESENTATION_ITEM ( )  RATIONAL_B_SPLINE_CURVE ( ( 0.9330127018922194093, 0.9330127018922194093, 1.000000000000000000, 0.8660254037844387076, 1.000000000000000000, 0.8660254037844387076, 1.000000000000000000, 0.9330127018922194093, 0.9330127018922194093 ) ) 
 REPRESENTATION_ITEM ( '' )  );
#36154=CARTESIAN_POINT ( 'NONE',  ( -1.846868145590737420, -154.0000000013655779, 4.458734124999999437 ) ) ;
#36155=CARTESIAN_POINT ( 'NONE',  ( 4.458734125000001214, -72.89583333196775072, 2.574251347313718519 ) ) ;
#36157=CARTESIAN_POINT ( 'NONE',  ( -4.458734124999999437, -21.64583333196774362, -2.574251347313719407 ) ) ;
#36158=CARTESIAN_POINT ( 'NONE',  ( 1.060575238724906964E-15, -58.62499999726880873, 5.773502691896257311 ) ) ;
#36161=ORIENTED_EDGE ( 'NONE', *, *, #62538, .T. ) ;
#36164=CARTESIAN_POINT ( 'NONE',  ( 4.458734124999999437, -152.4375000013655779, 0.000000000000000000 ) ) ;
#36165=ORIENTED_EDGE ( 'NONE', *, *, #53981, .T. ) ;
#36166=CARTESIAN_POINT ( 'NONE',  ( 1.975475456537005874E-15, -54.74999999999999289, 5.000000000000000000 ) ) ;
#36169=CARTESIAN_POINT ( 'NONE',  ( 2.229367062500001939, -46.22916666530106511, 3.861377020970579999 ) ) ;
#36171=ORIENTED_EDGE ( 'NONE', *, *, #11000, .F. ) ;
#36172=EDGE_CURVE ( 'NONE', #53443, #52361, #20641, .T. ) ;
#36175=CARTESIAN_POINT ( 'NONE',  ( -4.458734124999999437, 24.60416666803225993, -2.574251347313719407 ) ) ;
#36178=CARTESIAN_POINT ( 'NONE',  ( 5.000000000000000000, -61.37499999726880873, -6.123233995736766282E-16 ) ) ;
#36184=CARTESIAN_POINT ( 'NONE',  ( -5.000000000000000000, -157.5000000000000000, -6.123233995736766282E-16 ) ) ;
#36187=ADVANCED_FACE ( 'NONE', ( #1618 ), #16396, .T. ) ;
#36188=LINE ( 'NONE', #39715, #25491 ) ;
#36189=DIRECTION ( 'NONE',  ( -0.000000000000000000, 1.000000000000000000, -0.000000000000000000 ) ) ;
#36191=ORIENTED_EDGE ( 'NONE', *, *, #9529, .T. ) ;
#36194=CARTESIAN_POINT ( 'NONE',  ( -3.535533905932737309, -157.7500000027312126, -3.535533905932738197 ) ) ;
#36204=CARTESIAN_POINT ( 'NONE',  ( -4.458734124999997661, -24.22916666530107577, 2.574251347313722516 ) ) ;
#36206=CARTESIAN_POINT ( 'NONE',  ( 3.061616997868383141E-16, -150.7500000000000284, -5.000000000000000000 ) ) ;
#36208=CARTESIAN_POINT ( 'NONE',  ( 3.152801135295366208, -151.5625000013655779, 3.152801135295367985 ) ) ;
#36210=CARTESIAN_POINT ( 'NONE',  ( -2.229367062500000163, -51.72916666530107221, -3.861377020970580443 ) ) ;
#36212=CARTESIAN_POINT ( 'NONE',  ( 5.000000000000000000, 29.58333333333332860, -2.886751345948129988 ) ) ;
#36214=CARTESIAN_POINT ( 'NONE',  ( -4.458734124999998549, 4.770833334698926009, 2.574251347313722516 ) ) ;
#36215=CARTESIAN_POINT ( 'NONE',  ( 1.975475456537005874E-15, -73.62499999726878741, 5.000000000000000000 ) ) ;
#36216=DIRECTION ( 'NONE',  ( -0.000000000000000000, 1.000000000000000000, -0.000000000000000000 ) ) ;
#36217=CARTESIAN_POINT ( 'NONE',  ( 5.000000000000000888, -17.58333333333333215, 2.886751345948126879 ) ) ;
#36218=CARTESIAN_POINT ( 'NONE',  ( 4.458734125000001214, 12.85416666803226171, 2.574251347313718519 ) ) ;
#36219=CARTESIAN_POINT ( 'NONE',  ( -5.000000000000000000, 1.125000002731184390, 0.000000000000000000 ) ) ;
#36222=EDGE_LOOP ( 'NONE', ( #55552, #2468, #27291, #24458 ) ) ;
#36224=CARTESIAN_POINT ( 'NONE',  ( -4.458734124999998549, -46.22916666530106511, 2.574251347313722516 ) ) ;
#36225=CARTESIAN_POINT ( 'NONE',  ( -1.846868145590737420, -163.0000000013655779, 4.458734124999999437 ) ) ;
#36226=( BOUNDED_CURVE ( )  B_SPLINE_CURVE ( 2, ( #20739, #34890, #21055, #55476, #29725, #35211, #54829, #30049, #15908 ),
 .UNSPECIFIED., .F., .F. ) 
 B_SPLINE_CURVE_WITH_KNOTS ( ( 3, 2, 2, 2, 3 ),
 ( 0.5583333333333337922, 0.5625000000000004441, 0.5666666666666670960, 0.5708333333333338588, 0.5750000000000005107 ),
 .UNSPECIFIED. ) 
 CURVE ( )  GEOMETRIC_REPRESENTATION_ITEM ( )  RATIONAL_B_SPLINE_CURVE ( ( 0.9999999999999918954, 0.9238795325112948431, 1.000000000000000000, 0.9238795325112867385, 1.000000000000000000, 0.9238795325112867385, 1.000000000000000000, 0.9238795325112766355, 1.000000000000010214 ) ) 
 REPRESENTATION_ITEM ( '' )  );
#36227=CARTESIAN_POINT ( 'NONE',  ( 5.000000000000000000, -42.37499999726880873, -6.123233995736766282E-16 ) ) ;
#36228=ORIENTED_EDGE ( 'NONE', *, *, #14083, .F. ) ;
#36229=CARTESIAN_POINT ( 'NONE',  ( 2.229367062499998831, -18.64583333196774007, -3.861377020970580887 ) ) ;
#36230=ORIENTED_EDGE ( 'NONE', *, *, #31180, .T. ) ;
#36231=CARTESIAN_POINT ( 'NONE',  ( 2.499999999999998668, -85.33333333333332860, -4.330127018922193649 ) ) ;
#36232=CARTESIAN_POINT ( 'NONE',  ( 1.846868145590735200, -166.2500000013656347, -4.458734125000000326 ) ) ;
#36233=CARTESIAN_POINT ( 'NONE',  ( -1.339745962155610925, -60.66965819600733312, 5.000000000000000000 ) ) ;
#36234=ORIENTED_EDGE ( 'NONE', *, *, #32677, .T. ) ;
#36236=CARTESIAN_POINT ( 'NONE',  ( -2.229367062500000163, -32.72916666530106511, -3.861377020970580443 ) ) ;
#36237=CYLINDRICAL_SURFACE ( 'NONE', #38162, 5.000000000000000000 ) ;
#36244=EDGE_CURVE ( 'NONE', #25625, #9714, #22334, .T. ) ;
#36245=ORIENTED_EDGE ( 'NONE', *, *, #17302, .T. ) ;
#36246=CARTESIAN_POINT ( 'NONE',  ( -2.071067811865446640, -166.4375000027311842, 5.000000000000031086 ) ) ;
#36248=CARTESIAN_POINT ( 'NONE',  ( -4.458734124999998549, -82.47916666530106511, 2.574251347313722516 ) ) ;
#36251=CARTESIAN_POINT ( 'NONE',  ( 1.846868145590735200, -143.5000000013655779, -4.458734124999999437 ) ) ;
#36252=CARTESIAN_POINT ( 'NONE',  ( 1.255007937094098239E-14, 24.75000000000000000, -4.999999999999999112 ) ) ;
#36254=CARTESIAN_POINT ( 'NONE',  ( 2.229367062499998831, -43.64583333196773651, -3.861377020970580887 ) ) ;
#36257=ADVANCED_FACE ( 'NONE', ( #12827 ), #3197, .T. ) ;
#36259=CARTESIAN_POINT ( 'NONE',  ( 1.975475456537005874E-15, -20.74999999999999645, 5.000000000000000000 ) ) ;
#36262=CARTESIAN_POINT ( 'NONE',  ( 2.500000000000002220, 16.45833333606451987, 4.330127018922192761 ) ) ;
#36264=CARTESIAN_POINT ( 'NONE',  ( -3.152548672688508926E-16, -81.81249999863440792, -5.148502694627439702 ) ) ;
#36272=CARTESIAN_POINT ( 'NONE',  ( 1.975475456537005874E-15, -47.74999999999999289, 5.000000000000000000 ) ) ;
#36277=CARTESIAN_POINT ( 'NONE',  ( -4.458734124999997661, 11.52083333469892423, 2.574251347313722516 ) ) ;
#36278=DIRECTION ( 'NONE',  ( 0.000000000000000000, 0.000000000000000000, 1.000000000000000000 ) ) ;
#36283=( BOUNDED_CURVE ( )  B_SPLINE_CURVE ( 2, ( #1908, #55295, #6086, #60442, #55616, #16998, #21514, #60757, #45944 ),
 .UNSPECIFIED., .F., .F. ) 
 B_SPLINE_CURVE_WITH_KNOTS ( ( 3, 2, 2, 2, 3 ),
 ( 0.2520833333333333259, 0.2527777777777777679, 0.2541666666666666519, 0.2555555555555555358, 0.2562499999999999778 ),
 .UNSPECIFIED. ) 
 CURVE ( )  GEOMETRIC_REPRESENTATION_ITEM ( )  RATIONAL_B_SPLINE_CURVE ( ( 0.9330127018922194093, 0.9330127018922194093, 1.000000000000000000, 0.8660254037844387076, 1.000000000000000000, 0.8660254037844387076, 1.000000000000000000, 0.9330127018922194093, 0.9330127018922194093 ) ) 
 REPRESENTATION_ITEM ( '' )  );
#36285=CARTESIAN_POINT ( 'NONE',  ( -4.458734124999999437, -85.31249999863439371, 0.000000000000000000 ) ) ;
#36286=CARTESIAN_POINT ( 'NONE',  ( 9.457646018065525792E-16, -3.062499998634407472, 5.148502694627439702 ) ) ;
#36287=ORIENTED_EDGE ( 'NONE', *, *, #1935, .F. ) ;
#36288=CARTESIAN_POINT ( 'NONE',  ( -3.152548672688508926E-16, -36.81249999863440792, -5.148502694627439702 ) ) ;
#36292=CARTESIAN_POINT ( 'NONE',  ( 9.457646018065525792E-16, 22.93750000136559919, 5.148502694627439702 ) ) ;
#36294=CARTESIAN_POINT ( 'NONE',  ( -6.972266317189433020E-16, -40.12499999726880162, -5.000000000000000000 ) ) ;
#36295=CARTESIAN_POINT ( 'NONE',  ( -2.229367062499996610, -80.39583333196773651, 3.861377020970582219 ) ) ;
#36298=CARTESIAN_POINT ( 'NONE',  ( 5.000000000000000888, 20.54166666939784847, 2.886751345948126879 ) ) ;
#36299=ORIENTED_EDGE ( 'NONE', *, *, #37761, .F. ) ;
#36301=CARTESIAN_POINT ( 'NONE',  ( -5.000000000000000888, -168.5625000027312410, 2.071067811865474617 ) ) ;
#36303=CARTESIAN_POINT ( 'NONE',  ( -5.000000000000000000, -24.08333333333333215, -2.886751345948128211 ) ) ;
#36304=CARTESIAN_POINT ( 'NONE',  ( 4.458734124999999437, -29.81249999863440436, -5.460374474430324690E-16 ) ) ;
#36306=CARTESIAN_POINT ( 'NONE',  ( -2.499999999999996447, -25.70833333060214798, 4.330127018922195425 ) ) ;
#36307=CARTESIAN_POINT ( 'NONE',  ( 4.458734124999998549, -52.72916666530107221, -2.574251347313721627 ) ) ;
#36311=CARTESIAN_POINT ( 'NONE',  ( 4.458734124999999437, -3.062499998634407472, -5.460374474430324690E-16 ) ) ;
#36313=CARTESIAN_POINT ( 'NONE',  ( 1.060575238724906964E-15, -69.75000000000000000, 5.773502691896257311 ) ) ;
#36317=CARTESIAN_POINT ( 'NONE',  ( -2.071067811865478170, -159.3125000000000000, 5.000000000000000000 ) ) ;
#36318=CARTESIAN_POINT ( 'NONE',  ( -2.500000000000000444, -70.04166666393547303, -4.330127018922193649 ) ) ;
#36320=CARTESIAN_POINT ( 'NONE',  ( 2.229367062499998831, -17.89583333196773651, -3.861377020970580887 ) ) ;
#36321=CARTESIAN_POINT ( 'NONE',  ( -4.458734124999999437, -49.56249999863440792, 0.000000000000000000 ) ) ;
#36322=CARTESIAN_POINT ( 'NONE',  ( 1.846868145590736310, -143.6250000013655779, 4.458734124999999437 ) ) ;
#36324=CARTESIAN_POINT ( 'NONE',  ( 2.499999999999998668, -8.208333330602144429, -4.330127018922193649 ) ) ;
#36327=CARTESIAN_POINT ( 'NONE',  ( -4.458734124999999437, 24.35416666803225993, -2.574251347313719407 ) ) ;
#36329=( BOUNDED_CURVE ( )  B_SPLINE_CURVE ( 2, ( #51481, #12860, #42755, #37944, #46646, #2591, #57261, #32479, #13180 ),
 .UNSPECIFIED., .F., .F. ) 
 B_SPLINE_CURVE_WITH_KNOTS ( ( 3, 2, 2, 2, 3 ),
 ( 0.1104166666666666630, 0.1111111111111111049, 0.1125000000000000028, 0.1138888888888888867, 0.1145833333333333426 ),
 .UNSPECIFIED. ) 
 CURVE ( )  GEOMETRIC_REPRESENTATION_ITEM ( )  RATIONAL_B_SPLINE_CURVE ( ( 0.9330127018922194093, 0.9330127018922194093, 1.000000000000000000, 0.8660254037844387076, 1.000000000000000000, 0.8660254037844387076, 1.000000000000000000, 0.9330127018922187432, 0.9330127018922194093 ) ) 
 REPRESENTATION_ITEM ( '' )  );
#36330=DIRECTION ( 'NONE',  ( 0.000000000000000000, 0.000000000000000000, 1.000000000000000000 ) ) ;
#36332=VECTOR ( 'NONE', #42875, 1000.000000000000000 ) ;
#36333=CARTESIAN_POINT ( 'NONE',  ( 1.846868145590736310, -147.8750000013656063, 4.458734124999999437 ) ) ;
#36335=CARTESIAN_POINT ( 'NONE',  ( 4.458734124999998549, -62.97916666530107221, -2.574251347313721627 ) ) ;
#36336=CARTESIAN_POINT ( 'NONE',  ( -4.458734124999999437, -9.312499998634406140, 0.000000000000000000 ) ) ;
#36338=CARTESIAN_POINT ( 'NONE',  ( 3.152801135295367541, -145.3125000013655779, -3.152801135295367541 ) ) ;
#36345=CARTESIAN_POINT ( 'NONE',  ( -4.458734124999999437, 26.35416666803225993, -2.574251347313719407 ) ) ;
#36352=CARTESIAN_POINT ( 'NONE',  ( 5.000000000000000000, -56.29166666393548013, -2.886751345948130876 ) ) ;
#36353=DIRECTION ( 'NONE',  ( -0.000000000000000000, 1.000000000000000000, -0.000000000000000000 ) ) ;
#36354=CARTESIAN_POINT ( 'NONE',  ( -2.229367062499996610, 14.85416666803226171, 3.861377020970582219 ) ) ;
#36356=CARTESIAN_POINT ( 'NONE',  ( -4.458734124999997661, -14.47916666530107221, 2.574251347313722516 ) ) ;
#36358=CARTESIAN_POINT ( 'NONE',  ( 2.730187237215162345E-16, -163.1875000013655779, -4.458734124999999437 ) ) ;
#36359=CARTESIAN_POINT ( 'NONE',  ( 6.123233995736766282E-16, -170.0000000000000000, -5.000000000000000000 ) ) ;
#36363=CARTESIAN_POINT ( 'NONE',  ( 2.071067811865434205, -139.3125000027311842, 5.000000000000041744 ) ) ;
#36364=CARTESIAN_POINT ( 'NONE',  ( -4.458734124999999437, -33.31249999863440792, 0.000000000000000000 ) ) ;
#36365=CARTESIAN_POINT ( 'NONE',  ( 1.975475456537005874E-15, -51.62499999726880873, 5.000000000000000000 ) ) ;
#36372=CARTESIAN_POINT ( 'NONE',  ( 5.000000000000000888, -89.45833333060215864, 2.886751345948126879 ) ) ;
#36373=CARTESIAN_POINT ( 'NONE',  ( 2.500000000000002220, -9.666666666666664298, 4.330127018922192761 ) ) ;
#36374=CARTESIAN_POINT ( 'NONE',  ( -2.229367062499996610, -72.14583333196773651, 3.861377020970582219 ) ) ;
#36376=CYLINDRICAL_SURFACE ( 'NONE', #32875, 5.000000000000000000 ) ;
#36377=CARTESIAN_POINT ( 'NONE',  ( -5.000000000000000000, -6.958333330602150646, -2.886751345948128211 ) ) ;
#36378=CARTESIAN_POINT ( 'NONE',  ( 2.229367062500001939, -36.97916666530107221, 3.861377020970579999 ) ) ;
#36379=VERTEX_POINT ( 'NONE', #22814 ) ;
#36381=CARTESIAN_POINT ( 'NONE',  ( 4.458734124999998549, 14.02083333469892779, -2.574251347313721627 ) ) ;
#36384=CARTESIAN_POINT ( 'NONE',  ( 5.000000000000000888, -53.58333333333333570, 2.886751345948126879 ) ) ;
#36385=CARTESIAN_POINT ( 'NONE',  ( -4.458734125000001214, -159.1250000013656063, 1.846868145590734089 ) ) ;
#36387=DIRECTION ( 'NONE',  ( -0.000000000000000000, 1.000000000000000000, -0.000000000000000000 ) ) ;
#36388=CARTESIAN_POINT ( 'NONE',  ( -4.458734124999998549, -74.22916666530106511, 2.574251347313722516 ) ) ;
#36389=CARTESIAN_POINT ( 'NONE',  ( -5.000000000000000888, -168.5625000000000000, -2.071067811865475949 ) ) ;
#36390=CARTESIAN_POINT ( 'NONE',  ( 2.229367062500001939, -85.97916666530107932, 3.861377020970579999 ) ) ;
#36392=CARTESIAN_POINT ( 'NONE',  ( 2.229367062500001939, -34.22916666530107221, 3.861377020970579999 ) ) ;
#36400=LINE ( 'NONE', #56982, #46617 ) ;
#36401=CARTESIAN_POINT ( 'NONE',  ( -4.458734124999998549, -62.47916666530106511, 2.574251347313722516 ) ) ;
#36403=VERTEX_POINT ( 'NONE', #13772 ) ;
#36404=( BOUNDED_CURVE ( )  B_SPLINE_CURVE ( 2, ( #55225, #50390, #31723, #35922, #6025, #46525, #2467, #15974, #11462 ),
 .UNSPECIFIED., .F., .F. ) 
 B_SPLINE_CURVE_WITH_KNOTS ( ( 3, 2, 2, 2, 3 ),
 ( 0.4104166666666666519, 0.4111111111111110938, 0.4124999999999999778, 0.4138888888888888618, 0.4145833333333333592 ),
 .UNSPECIFIED. ) 
 CURVE ( )  GEOMETRIC_REPRESENTATION_ITEM ( )  RATIONAL_B_SPLINE_CURVE ( ( 0.9330127018922194093, 0.9330127018922194093, 1.000000000000000000, 0.8660254037844387076, 1.000000000000000000, 0.8660254037844387076, 1.000000000000000000, 0.9330127018922167448, 0.9330127018922194093 ) ) 
 REPRESENTATION_ITEM ( '' )  );
#36407=ORIENTED_EDGE ( 'NONE', *, *, #36970, .F. ) ;
#36410=CARTESIAN_POINT ( 'NONE',  ( 4.458734124999999437, 6.187500001365593860, -5.460374474430324690E-16 ) ) ;
#36412=CARTESIAN_POINT ( 'NONE',  ( 4.458734124999997661, -156.5000000013656347, 1.846868145590737864 ) ) ;
#36413=DIRECTION ( 'NONE',  ( -0.000000000000000000, 1.000000000000000000, -0.000000000000000000 ) ) ;
#36414=ORIENTED_EDGE ( 'NONE', *, *, #28405, .F. ) ;
#36418=LINE ( 'NONE', #39954, #12902 ) ;
#36425=CARTESIAN_POINT ( 'NONE',  ( -4.458734124999999437, 28.68750000136559208, 0.000000000000000000 ) ) ;
#36428=CARTESIAN_POINT ( 'NONE',  ( 9.457646018065525792E-16, 0.6875000013655957476, 5.148502694627439702 ) ) ;
#36431=CARTESIAN_POINT ( 'NONE',  ( 3.535533905932738197, -145.0000000027311842, -3.535533905932738197 ) ) ;
#36435=CARTESIAN_POINT ( 'NONE',  ( 6.123233995736766282E-16, -170.0000000000000000, -5.000000000000000000 ) ) ;
#36436=CARTESIAN_POINT ( 'NONE',  ( 2.499999999999998668, -22.33333333333332860, -4.330127018922193649 ) ) ;
#36438=CARTESIAN_POINT ( 'NONE',  ( -1.846868145590737420, -160.0000000013656063, 4.458734124999997661 ) ) ;
#36441=CARTESIAN_POINT ( 'NONE',  ( -8.190561711645485556E-16, -140.6875000013656063, 4.458734124999999437 ) ) ;
#36442=ORIENTED_EDGE ( 'NONE', *, *, #48987, .F. ) ;
#36443=CARTESIAN_POINT ( 'NONE',  ( -2.229367062500000163, 21.27083333469892779, -3.861377020970580443 ) ) ;
#36444=VERTEX_POINT ( 'NONE', #43351 ) ;
#36448=CARTESIAN_POINT ( 'NONE',  ( 1.339745962155615144, -16.70534180126147561, 4.999999999999999112 ) ) ;
#36449=CARTESIAN_POINT ( 'NONE',  ( 5.000000000000000888, 10.41666666666666607, 2.886751345948126879 ) ) ;
#36451=CARTESIAN_POINT ( 'NONE',  ( 2.229367062499998831, -58.64583333196773651, -3.861377020970580887 ) ) ;
#36452=CARTESIAN_POINT ( 'NONE',  ( -2.229367062499996610, -12.14583333196774007, 3.861377020970582219 ) ) ;
#36455=CARTESIAN_POINT ( 'NONE',  ( 0.000000000000000000, -170.0000000000000000, 0.000000000000000000 ) ) ;
#36456=CARTESIAN_POINT ( 'NONE',  ( -2.499999999999996447, 0.2916666693978525737, 4.330127018922195425 ) ) ;
#36458=CARTESIAN_POINT ( 'NONE',  ( 5.000000000000000000, -40.49999999999999289, -6.123233995736766282E-16 ) ) ;
#36459=CARTESIAN_POINT ( 'NONE',  ( 3.061616997868383141E-16, -148.7500000000000284, -5.000000000000000000 ) ) ;
#36463=CARTESIAN_POINT ( 'NONE',  ( 2.229367062500001939, -61.97916666530106511, 3.861377020970579999 ) ) ;
#36464=CARTESIAN_POINT ( 'NONE',  ( -3.152801135295367096, -151.3125000013655779, -3.152801135295367541 ) ) ;
#36465=CARTESIAN_POINT ( 'NONE',  ( 4.458734124999998549, -69.72916666530107932, -2.574251347313721627 ) ) ;
#36467=AXIS2_PLACEMENT_3D ( 'NONE', #6414, #20569, #55934 ) ;
#36468=CARTESIAN_POINT ( 'NONE',  ( 2.229367062499998831, -17.89583333196773651, -3.861377020970580887 ) ) ;
#36469=CARTESIAN_POINT ( 'NONE',  ( 2.499999999999998668, -63.20833333060215153, -4.330127018922193649 ) ) ;
#36470=ORIENTED_EDGE ( 'NONE', *, *, #54778, .T. ) ;
#36471=DIRECTION ( 'NONE',  ( -0.000000000000000000, 1.000000000000000000, -0.000000000000000000 ) ) ;
#36476=CARTESIAN_POINT ( 'NONE',  ( -4.458734125000000326, -153.0000000013656063, -1.846868145590735644 ) ) ;
#36479=CARTESIAN_POINT ( 'NONE',  ( -6.972266317189433020E-16, 25.74999999999999645, -5.000000000000000000 ) ) ;
#36481=CARTESIAN_POINT ( 'NONE',  ( -4.999999999999998224, -74.79166666393547303, 2.886751345948131764 ) ) ;
#36482=CARTESIAN_POINT ( 'NONE',  ( 2.229367062500001939, -47.22916666530106511, 3.861377020970579999 ) ) ;
#36483=ORIENTED_EDGE ( 'NONE', *, *, #15856, .F. ) ;
#36485=CARTESIAN_POINT ( 'NONE',  ( -3.152548672688508926E-16, 22.43750000136559208, -5.148502694627439702 ) ) ;
#36487=CARTESIAN_POINT ( 'NONE',  ( -1.846868145590734756, -169.1250000013656063, -4.458734124999999437 ) ) ;
#36488=ORIENTED_EDGE ( 'NONE', *, *, #25746, .F. ) ;
#36493=CARTESIAN_POINT ( 'NONE',  ( -5.000000000000000000, -27.08333333333333215, -2.886751345948128211 ) ) ;
#36498=( BOUNDED_CURVE ( )  B_SPLINE_CURVE ( 2, ( #16281, #16911, #6318, #59714, #6957, #16598, #30422, #50687, #51012 ),
 .UNSPECIFIED., .F., .F. ) 
 B_SPLINE_CURVE_WITH_KNOTS ( ( 3, 2, 2, 2, 3 ),
 ( 0.1354166666666666574, 0.1361111111111110994, 0.1375000000000000111, 0.1388888888888888951, 0.1395833333333333370 ),
 .UNSPECIFIED. ) 
 CURVE ( )  GEOMETRIC_REPRESENTATION_ITEM ( )  RATIONAL_B_SPLINE_CURVE ( ( 0.9330127018922194093, 0.9330127018922194093, 1.000000000000000000, 0.8660254037844387076, 1.000000000000000000, 0.8660254037844387076, 1.000000000000000000, 0.9330127018922194093, 0.9330127018922194093 ) ) 
 REPRESENTATION_ITEM ( '' )  );
#36503=CARTESIAN_POINT ( 'NONE',  ( -3.535533905932738641, -156.5000000027312126, 3.535533905932737309 ) ) ;
#36510=CARTESIAN_POINT ( 'NONE',  ( 3.535533905932736864, -148.1250000000000000, 3.535533905932738641 ) ) ;
#36514=CARTESIAN_POINT ( 'NONE',  ( -4.458734124999999437, -23.31249999863440436, 0.000000000000000000 ) ) ;
#36516=CARTESIAN_POINT ( 'NONE',  ( -5.000000000000000888, -152.5625000000000284, -2.071067811865475949 ) ) ;
#36518=CARTESIAN_POINT ( 'NONE',  ( -3.152801135295367985, -150.8125000013655779, 3.152801135295367096 ) ) ;
#36519=ORIENTED_EDGE ( 'NONE', *, *, #53455, .T. ) ;
#36520=CARTESIAN_POINT ( 'NONE',  ( 4.458734125000000326, -49.14583333196772941, 2.574251347313718519 ) ) ;
#36521=DIRECTION ( 'NONE',  ( -0.000000000000000000, 1.000000000000000000, -0.000000000000000000 ) ) ;
#36523=CARTESIAN_POINT ( 'NONE',  ( -2.499999999999996447, 23.16666666666666430, 4.330127018922195425 ) ) ;
#36526=CARTESIAN_POINT ( 'NONE',  ( -4.458734124999999437, 6.687500001365593860, 0.000000000000000000 ) ) ;
#36529=FACE_OUTER_BOUND ( 'NONE', #37822, .T. ) ;
#36530=CARTESIAN_POINT ( 'NONE',  ( -4.458734124999998549, 16.52083333469892779, 2.574251347313722516 ) ) ;
#36531=CARTESIAN_POINT ( 'NONE',  ( -2.500000000000000444, 4.958333336064518981, -4.330127018922193649 ) ) ;
#36534=ORIENTED_EDGE ( 'NONE', *, *, #35089, .T. ) ;
#36536=CARTESIAN_POINT ( 'NONE',  ( -4.458734124999999437, -42.31249999863440081, 0.000000000000000000 ) ) ;
#36537=CARTESIAN_POINT ( 'NONE',  ( 3.152801135295366208, -165.8125000013656063, 3.152801135295367985 ) ) ;
#36539=CARTESIAN_POINT ( 'NONE',  ( -2.500000000000000444, -47.04166666393547303, -4.330127018922193649 ) ) ;
#36541=CARTESIAN_POINT ( 'NONE',  ( -4.458734124999999437, -19.39583333196774007, -2.574251347313719407 ) ) ;
#36544=CARTESIAN_POINT ( 'NONE',  ( -5.000000000000000000, -86.00000000000000000, 0.000000000000000000 ) ) ;
#36545=CARTESIAN_POINT ( 'NONE',  ( 4.458734125000000326, -163.3750000013656347, -1.846868145590734978 ) ) ;
#36547=VERTEX_POINT ( 'NONE', #28875 ) ;
#36549=CARTESIAN_POINT ( 'NONE',  ( -4.458734124999999437, -31.64583333196773651, -2.574251347313719407 ) ) ;
#36556=ORIENTED_EDGE ( 'NONE', *, *, #52729, .F. ) ;
#36557=CARTESIAN_POINT ( 'NONE',  ( 3.061616997868383141E-16, -161.7500000000000000, -5.000000000000000000 ) ) ;
#36559=CARTESIAN_POINT ( 'NONE',  ( -4.458734124999999437, -80.56249999863440792, 0.000000000000000000 ) ) ;
#36562=CARTESIAN_POINT ( 'NONE',  ( 4.458734124999997661, -142.7500000013655779, 1.846868145590737864 ) ) ;
#36563=CARTESIAN_POINT ( 'NONE',  ( 5.000000000000000888, 20.41666666666666785, 2.886751345948126879 ) ) ;
#36565=CARTESIAN_POINT ( 'NONE',  ( -4.458734124999997661, -45.22916666530106511, 2.574251347313722516 ) ) ;
#36568=CARTESIAN_POINT ( 'NONE',  ( 2.071067811865645591, -154.3125000027311557, 4.999999999999830358 ) ) ;
#36571=DIRECTION ( 'NONE',  ( 0.000000000000000000, 0.000000000000000000, 1.000000000000000000 ) ) ;
#36572=CARTESIAN_POINT ( 'NONE',  ( -5.000000000000000000, -45.87499999726880873, 0.000000000000000000 ) ) ;
#36573=CARTESIAN_POINT ( 'NONE',  ( 4.458734125000001214, -79.14583333196772230, 2.574251347313718519 ) ) ;
#36579=CARTESIAN_POINT ( 'NONE',  ( 1.339745962155612702, -9.169658196007334894, -5.000000000000000000 ) ) ;
#36581=CARTESIAN_POINT ( 'NONE',  ( -6.972266317189433020E-16, -5.249999999999998224, -5.000000000000000000 ) ) ;
#36583=CARTESIAN_POINT ( 'NONE',  ( -2.229367062499996610, 10.60416666803225993, 3.861377020970582219 ) ) ;
#36590=CARTESIAN_POINT ( 'NONE',  ( -2.229367062499996610, -84.14583333196773651, 3.861377020970582219 ) ) ;
#36591=CARTESIAN_POINT ( 'NONE',  ( -4.458734124999997661, -7.229166665301073103, 2.574251347313722516 ) ) ;
#36594=CARTESIAN_POINT ( 'NONE',  ( -4.458734124999999437, -33.56249999863440792, 0.000000000000000000 ) ) ;
#36595=VECTOR ( 'NONE', #28380, 1000.000000000000000 ) ;
#36601=( BOUNDED_CURVE ( )  B_SPLINE_CURVE ( 2, ( #11234, #2248, #31806, #60779, #16705, #51440, #6739, #16063, #1302 ),
 .UNSPECIFIED., .F., .F. ) 
 B_SPLINE_CURVE_WITH_KNOTS ( ( 3, 2, 2, 2, 3 ),
 ( 0.1604166666666666796, 0.1611111111111111216, 0.1625000000000000056, 0.1638888888888888895, 0.1645833333333333315 ),
 .UNSPECIFIED. ) 
 CURVE ( )  GEOMETRIC_REPRESENTATION_ITEM ( )  RATIONAL_B_SPLINE_CURVE ( ( 0.9330127018922194093, 0.9330127018922207416, 1.000000000000000000, 0.8660254037844387076, 1.000000000000000000, 0.8660254037844387076, 1.000000000000000000, 0.9330127018922194093, 0.9330127018922194093 ) ) 
 REPRESENTATION_ITEM ( '' )  );
#36602=CARTESIAN_POINT ( 'NONE',  ( 4.458734124999999437, -148.6250000013655779, -1.846868145590734978 ) ) ;
#36603=CARTESIAN_POINT ( 'NONE',  ( -2.229367062500000163, 20.52083333469892779, -3.861377020970580443 ) ) ;
#36606=CARTESIAN_POINT ( 'NONE',  ( -5.000000000000000000, -25.95833333060214798, -2.886751345948128211 ) ) ;
#36607=CARTESIAN_POINT ( 'NONE',  ( 4.458734125000000326, -81.14583333196773651, 2.574251347313718519 ) ) ;
#36609=EDGE_CURVE ( 'NONE', #21297, #11671, #29180, .T. ) ;
#36611=CARTESIAN_POINT ( 'NONE',  ( 5.000000000000000000, 18.70833333606451632, -2.886751345948129988 ) ) ;
#36613=CARTESIAN_POINT ( 'NONE',  ( 1.975475456537005874E-15, -75.62499999726880162, 5.000000000000000000 ) ) ;
#36614=CARTESIAN_POINT ( 'NONE',  ( 2.499999999999998668, -26.33333333333333215, -4.330127018922193649 ) ) ;
#36615=CARTESIAN_POINT ( 'NONE',  ( 4.458734125000001214, -29.89583333196773651, 2.574251347313718519 ) ) ;
#36617=EDGE_CURVE ( 'NONE', #141, #37963, #59432, .T. ) ;
#36618=CARTESIAN_POINT ( 'NONE',  ( 1.060575238724906964E-15, -29.62499999726881228, 5.773502691896257311 ) ) ;
#36619=CARTESIAN_POINT ( 'NONE',  ( -3.152548672688508926E-16, -53.56249999863439371, -5.148502694627439702 ) ) ;
#36622=EDGE_CURVE ( 'NONE', #39380, #24136, #19856, .T. ) ;
#36623=CARTESIAN_POINT ( 'NONE',  ( 2.229367062499998831, -4.895833331967740065, -3.861377020970580887 ) ) ;
#36624=ORIENTED_EDGE ( 'NONE', *, *, #59057, .T. ) ;
#36625=CARTESIAN_POINT ( 'NONE',  ( 5.000000000000000888, -70.58333333333332860, 2.886751345948126879 ) ) ;
#36629=EDGE_CURVE ( 'NONE', #29478, #37570, #35854, .T. ) ;
#36630=CARTESIAN_POINT ( 'NONE',  ( 2.500000000000002220, -76.54166666393547303, 4.330127018922192761 ) ) ;
#36633=CARTESIAN_POINT ( 'NONE',  ( -4.458734124999999437, -17.56249999863440792, 0.000000000000000000 ) ) ;
#36634=CARTESIAN_POINT ( 'NONE',  ( -4.458734124999999437, -53.64583333196772941, -2.574251347313719407 ) ) ;
#36637=CARTESIAN_POINT ( 'NONE',  ( -1.846868145590734756, -142.1250000013656063, -4.458734125000000326 ) ) ;
#36639=LINE ( 'NONE', #41135, #2004 ) ;
#36641=CYLINDRICAL_SURFACE ( 'NONE', #52940, 5.000000000000000000 ) ;
#36647=CARTESIAN_POINT ( 'NONE',  ( -4.458734125000001214, -148.1250000013655779, 1.846868145590734089 ) ) ;
#36652=( BOUNDED_CURVE ( )  B_SPLINE_CURVE ( 2, ( #56979, #2953, #13217, #3271, #2629, #61494, #17425, #46370, #51827 ),
 .UNSPECIFIED., .F., .F. ) 
 B_SPLINE_CURVE_WITH_KNOTS ( ( 3, 2, 2, 2, 3 ),
 ( 0.1062499999999999972, 0.1069444444444444392, 0.1083333333333333370, 0.1097222222222222210, 0.1104166666666666630 ),
 .UNSPECIFIED. ) 
 CURVE ( )  GEOMETRIC_REPRESENTATION_ITEM ( )  RATIONAL_B_SPLINE_CURVE ( ( 0.9330127018922194093, 0.9330127018922194093, 1.000000000000000000, 0.8660254037844387076, 1.000000000000000000, 0.8660254037844387076, 1.000000000000000000, 0.9330127018922194093, 0.9330127018922194093 ) ) 
 REPRESENTATION_ITEM ( '' )  );
#36653=CARTESIAN_POINT ( 'NONE',  ( -2.229367062499996610, -61.39583333196774362, 3.861377020970582219 ) ) ;
#36655=LINE ( 'NONE', #7397, #57274 ) ;
#36656=CARTESIAN_POINT ( 'NONE',  ( -4.458734124999999437, -143.9375000013656063, -5.460374474430324690E-16 ) ) ;
#36660=CARTESIAN_POINT ( 'NONE',  ( -3.535533905932738641, -164.5000000027312126, 3.535533905932737309 ) ) ;
#36664=CARTESIAN_POINT ( 'NONE',  ( -4.458734124999999437, 29.43750000136559208, 0.000000000000000000 ) ) ;
#36670=CARTESIAN_POINT ( 'NONE',  ( 1.975475456537005874E-15, -21.62499999726880873, 5.000000000000000000 ) ) ;
#36671=CARTESIAN_POINT ( 'NONE',  ( 2.500000000000002220, 21.33333333333333215, 4.330127018922192761 ) ) ;
#36672=CARTESIAN_POINT ( 'NONE',  ( -4.458734124999999437, 9.604166668032259935, -2.574251347313719407 ) ) ;
#36674=CARTESIAN_POINT ( 'NONE',  ( -4.458734124999997661, -17.47916666530106866, 2.574251347313722516 ) ) ;
#36676=CARTESIAN_POINT ( 'NONE',  ( 4.458734124999999437, -159.5000000013655779, 1.846868145590737864 ) ) ;
#36682=CARTESIAN_POINT ( 'NONE',  ( -2.229367062499996610, -35.14583333196772941, 3.861377020970582219 ) ) ;
#36684=DIRECTION ( 'NONE',  ( 0.000000000000000000, 0.000000000000000000, 1.000000000000000000 ) ) ;
#36685=CARTESIAN_POINT ( 'NONE',  ( 4.458734124999998549, -59.97916666530106511, -2.574251347313721627 ) ) ;
#36689=CARTESIAN_POINT ( 'NONE',  ( 5.000000000000000888, -36.45833333060213732, 2.886751345948126879 ) ) ;
#36694=CARTESIAN_POINT ( 'NONE',  ( 2.500000000000002220, -7.666666666666668739, 4.330127018922192761 ) ) ;
#36695=CARTESIAN_POINT ( 'NONE',  ( -4.458734124999999437, -70.39583333196773651, -2.574251347313719407 ) ) ;
#36698=CARTESIAN_POINT ( 'NONE',  ( -3.535250795749689387E-16, -12.12499999726881761, -5.773502691896257311 ) ) ;
#36699=CARTESIAN_POINT ( 'NONE',  ( -2.229367062500000163, -40.47916666530107221, -3.861377020970580443 ) ) ;
#36700=ORIENTED_EDGE ( 'NONE', *, *, #12488, .T. ) ;
#36703=CARTESIAN_POINT ( 'NONE',  ( -4.458734124999998549, 12.52083333469892779, 2.574251347313722516 ) ) ;
#36705=CARTESIAN_POINT ( 'NONE',  ( 2.500000000000002220, -81.66666666666667140, 4.330127018922192761 ) ) ;
#36706=CARTESIAN_POINT ( 'NONE',  ( -2.499999999999996447, -57.83333333333333570, 4.330127018922195425 ) ) ;
#36707=ADVANCED_FACE ( 'NONE', ( #39154 ), #10214, .T. ) ;
#36708=CARTESIAN_POINT ( 'NONE',  ( -1.846868145590734756, -161.3750000013656063, -4.458734125000000326 ) ) ;
#36711=CARTESIAN_POINT ( 'NONE',  ( -2.229367062499996610, -80.14583333196773651, 3.861377020970582219 ) ) ;
#36713=CARTESIAN_POINT ( 'NONE',  ( 3.152801135295366208, -139.8125000013655779, 3.152801135295367985 ) ) ;
#36715=CARTESIAN_POINT ( 'NONE',  ( -2.229367062499996610, -87.14583333196773651, 3.861377020970582219 ) ) ;
#36717=CARTESIAN_POINT ( 'NONE',  ( -4.458734124999999437, 1.354166668032261933, -2.574251347313719407 ) ) ;
#36718=CARTESIAN_POINT ( 'NONE',  ( -4.458734124999999437, -33.64583333196772941, -2.574251347313719407 ) ) ;
#36719=EDGE_CURVE ( 'NONE', #38746, #45557, #44296, .T. ) ;
#36722=CARTESIAN_POINT ( 'NONE',  ( 5.000000000000000888, -84.58333333333332860, 2.886751345948126879 ) ) ;
#36725=CARTESIAN_POINT ( 'NONE',  ( -1.339745962155660663, -18.66965819600733667, 4.999999999999972466 ) ) ;
#36726=CARTESIAN_POINT ( 'NONE',  ( -3.152548672688508926E-16, -70.81249999863440792, -5.148502694627439702 ) ) ;
#36728=EDGE_LOOP ( 'NONE', ( #5536, #51110, #5327, #19614 ) ) ;
#36729=CARTESIAN_POINT ( 'NONE',  ( 1.339745962155612702, -3.169658196007334894, -5.000000000000000000 ) ) ;
#36732=CARTESIAN_POINT ( 'NONE',  ( -2.229367062499996610, 8.854166668032261711, 3.861377020970582219 ) ) ;
#36734=CARTESIAN_POINT ( 'NONE',  ( -3.152801135295367096, -159.0625000013656063, -3.152801135295367541 ) ) ;
#36737=ORIENTED_EDGE ( 'NONE', *, *, #41053, .T. ) ;
#36739=CARTESIAN_POINT ( 'NONE',  ( -4.999999999999998224, -24.91666666666666430, 2.886751345948131764 ) ) ;
#36747=CARTESIAN_POINT ( 'NONE',  ( 5.000000000000000000, -10.41666666666666607, -2.886751345948130876 ) ) ;
#36748=CARTESIAN_POINT ( 'NONE',  ( -2.229367062500000163, 28.52083333469892779, -3.861377020970580443 ) ) ;
#36751=CARTESIAN_POINT ( 'NONE',  ( 2.229367062499998831, -1.895833331967737623, -3.861377020970580887 ) ) ;
#36752=CARTESIAN_POINT ( 'NONE',  ( 1.339745962155612702, -0.1696581960073343942, -5.000000000000000000 ) ) ;
#36754=CARTESIAN_POINT ( 'NONE',  ( -2.071067811865475061, -141.8125000027311842, -5.000000000000000888 ) ) ;
#36755=CYLINDRICAL_SURFACE ( 'NONE', #17174, 5.000000000000000000 ) ;
#36758=AXIS2_PLACEMENT_3D ( 'NONE', #26933, #17273, #36897 ) ;
#36760=LINE ( 'NONE', #56389, #22653 ) ;
#36761=EDGE_CURVE ( 'NONE', #19705, #32024, #27210, .T. ) ;
#36762=CARTESIAN_POINT ( 'NONE',  ( 2.500000000000002220, 3.333333333333333925, 4.330127018922192761 ) ) ;
#36764=CARTESIAN_POINT ( 'NONE',  ( 2.730187237215162345E-16, -163.4375000013655779, -4.458734124999999437 ) ) ;
#36766=CARTESIAN_POINT ( 'NONE',  ( -2.500000000000000444, -57.16666666666667140, -4.330127018922193649 ) ) ;
#36767=ORIENTED_EDGE ( 'NONE', *, *, #1539, .T. ) ;
#36768=CARTESIAN_POINT ( 'NONE',  ( 9.457646018065525792E-16, 18.68750000136559208, 5.148502694627439702 ) ) ;
#36769=EDGE_LOOP ( 'NONE', ( #49863, #6140, #53264, #12094 ) ) ;
#36774=CARTESIAN_POINT ( 'NONE',  ( -2.499999999999996447, 9.166666666666666075, 4.330127018922195425 ) ) ;
#36775=CARTESIAN_POINT ( 'NONE',  ( -2.229367062500000163, -55.47916666530107221, -3.861377020970580443 ) ) ;
#36776=CARTESIAN_POINT ( 'NONE',  ( 1.339745962155615144, -6.705341801261480050, 4.999999999999999112 ) ) ;
#36778=CARTESIAN_POINT ( 'NONE',  ( 5.000000000000000000, 7.625000002731186832, -6.123233995736766282E-16 ) ) ;
#36780=CARTESIAN_POINT ( 'NONE',  ( 5.000000000000000888, -39.58333333333333570, 2.886751345948126879 ) ) ;
#36781=DIRECTION ( 'NONE',  ( -0.000000000000000000, 1.000000000000000000, -0.000000000000000000 ) ) ;
#36784=CARTESIAN_POINT ( 'NONE',  ( 1.975475456537005874E-15, 13.24999999999999822, 5.000000000000000000 ) ) ;
#36785=CARTESIAN_POINT ( 'NONE',  ( 2.229367062499998831, -64.64583333196773651, -3.861377020970580887 ) ) ;
#36786=CARTESIAN_POINT ( 'NONE',  ( -1.846868145590737420, -152.0000000013655779, 4.458734124999999437 ) ) ;
#36787=CARTESIAN_POINT ( 'NONE',  ( 4.458734125000001214, -70.89583333196773651, 2.574251347313718519 ) ) ;
#36788=AXIS2_PLACEMENT_3D ( 'NONE', #49352, #5941, #25230 ) ;
#36791=CARTESIAN_POINT ( 'NONE',  ( 4.458734124999999437, -17.06249999863440792, -5.460374474430324690E-16 ) ) ;
#36792=CARTESIAN_POINT ( 'NONE',  ( -5.000000000000000000, -59.95833333060215153, -2.886751345948128211 ) ) ;
#36793=ORIENTED_EDGE ( 'NONE', *, *, #48929, .F. ) ;
#36794=CARTESIAN_POINT ( 'NONE',  ( -2.500000000000000444, -49.16666666666666430, -4.330127018922193649 ) ) ;
#36797=CARTESIAN_POINT ( 'NONE',  ( -9.184850993605147944E-16, -144.2500000000000284, 5.000000000000000000 ) ) ;
#36798=CARTESIAN_POINT ( 'NONE',  ( 1.846868145590735200, -152.2500000013656347, -4.458734125000000326 ) ) ;
#36799=ORIENTED_EDGE ( 'NONE', *, *, #16940, .T. ) ;
#36803=CARTESIAN_POINT ( 'NONE',  ( -4.458734124999998549, -46.47916666530107221, 2.574251347313722516 ) ) ;
#36805=VECTOR ( 'NONE', #41872, 1000.000000000000000 ) ;
#36809=CARTESIAN_POINT ( 'NONE',  ( -4.458734124999999437, 21.68750000136559208, 0.000000000000000000 ) ) ;
#36813=ORIENTED_EDGE ( 'NONE', *, *, #98, .T. ) ;
#36817=EDGE_CURVE ( 'NONE', #25520, #7918, #37913, .T. ) ;
#36821=CARTESIAN_POINT ( 'NONE',  ( 0.000000000000000000, -170.0000000000000000, 0.000000000000000000 ) ) ;
#36822=DIRECTION ( 'NONE',  ( 0.000000000000000000, 0.000000000000000000, 1.000000000000000000 ) ) ;
#36823=CARTESIAN_POINT ( 'NONE',  ( -1.339745962155613812, 18.79465819873852084, -5.000000000000000000 ) ) ;
#36826=EDGE_LOOP ( 'NONE', ( #46143, #23105, #53957, #16943 ) ) ;
#36830=CARTESIAN_POINT ( 'NONE',  ( -2.071067811865475061, -157.8125000027311842, -5.000000000000000888 ) ) ;
#36836=CARTESIAN_POINT ( 'NONE',  ( 3.535533905932738197, -146.8750000000000000, -3.535533905932738197 ) ) ;
#36840=CARTESIAN_POINT ( 'NONE',  ( -4.458734124999999437, -25.31249999863440792, 0.000000000000000000 ) ) ;
#36842=CARTESIAN_POINT ( 'NONE',  ( 2.071067811865475505, -151.8125000000000284, -5.000000000000000888 ) ) ;
#36844=CARTESIAN_POINT ( 'NONE',  ( -3.152801135295367985, -152.8125000013656063, 3.152801135295367096 ) ) ;
#36845=ORIENTED_EDGE ( 'NONE', *, *, #31305, .F. ) ;
#36847=CARTESIAN_POINT ( 'NONE',  ( -2.229367062500000163, -52.72916666530107221, -3.861377020970580443 ) ) ;
#36850=CARTESIAN_POINT ( 'NONE',  ( -2.500000000000000444, 22.83333333333333215, -4.330127018922193649 ) ) ;
#36852=LINE ( 'NONE', #31369, #8857 ) ;
#36853=CARTESIAN_POINT ( 'NONE',  ( 4.458734124999998549, -1.729166665301068440, -2.574251347313721627 ) ) ;
#36856=CARTESIAN_POINT ( 'NONE',  ( 2.499999999999998668, -7.333333333333330373, -4.330127018922193649 ) ) ;
#36857=CARTESIAN_POINT ( 'NONE',  ( 4.458734125000001214, 15.85416666803226171, 2.574251347313718519 ) ) ;
#36858=CARTESIAN_POINT ( 'NONE',  ( 5.000000000000000000, 0.6250000027311873874, -6.123233995736766282E-16 ) ) ;
#36861=ORIENTED_EDGE ( 'NONE', *, *, #18629, .T. ) ;
#36862=( BOUNDED_CURVE ( )  B_SPLINE_CURVE ( 2, ( #33186, #58252, #4850, #43135, #62775, #57949, #33493, #19003, #53112 ),
 .UNSPECIFIED., .F., .F. ) 
 B_SPLINE_CURVE_WITH_KNOTS ( ( 3, 2, 2, 2, 3 ),
 ( 0.6187500000000000222, 0.6194444444444444642, 0.6208333333333333481, 0.6222222222222222321, 0.6229166666666666741 ),
 .UNSPECIFIED. ) 
 CURVE ( )  GEOMETRIC_REPRESENTATION_ITEM ( )  RATIONAL_B_SPLINE_CURVE ( ( 0.9330127018922194093, 0.9330127018922194093, 1.000000000000000000, 0.8660254037844387076, 1.000000000000000000, 0.8660254037844387076, 1.000000000000000000, 0.9330127018922194093, 0.9330127018922194093 ) ) 
 REPRESENTATION_ITEM ( '' )  );
#36863=CARTESIAN_POINT ( 'NONE',  ( 9.457646018065525792E-16, -45.06249999863440792, 5.148502694627439702 ) ) ;
#36864=CARTESIAN_POINT ( 'NONE',  ( -4.458734124999999437, -165.1875000013655779, -5.460374474430324690E-16 ) ) ;
#36865=CARTESIAN_POINT ( 'NONE',  ( -5.000000000000000000, -44.95833333060215153, -2.886751345948128211 ) ) ;
#36866=ORIENTED_EDGE ( 'NONE', *, *, #12950, .T. ) ;
#36867=CARTESIAN_POINT ( 'NONE',  ( 9.457646018065525792E-16, -20.06249999863440081, 5.148502694627439702 ) ) ;
#36868=ORIENTED_EDGE ( 'NONE', *, *, #41984, .F. ) ;
#36869=CARTESIAN_POINT ( 'NONE',  ( -5.000000000000000000, -89.00000000000000000, 0.000000000000000000 ) ) ;
#36870=CARTESIAN_POINT ( 'NONE',  ( 4.458734124999999437, -163.4375000013655779, 0.000000000000000000 ) ) ;
#36873=VECTOR ( 'NONE', #49520, 1000.000000000000000 ) ;
#36874=CARTESIAN_POINT ( 'NONE',  ( 9.457646018065525792E-16, -31.31249999863440436, 5.148502694627439702 ) ) ;
#36875=CARTESIAN_POINT ( 'NONE',  ( -5.000000000000000888, -147.5625000027311842, 2.071067811865474617 ) ) ;
#36879=CARTESIAN_POINT ( 'NONE',  ( 5.000000000000000888, 24.54166666939784847, 2.886751345948126879 ) ) ;
#36880=ORIENTED_EDGE ( 'NONE', *, *, #33048, .T. ) ;
#36883=CARTESIAN_POINT ( 'NONE',  ( -4.458734124999998549, -78.47916666530107932, 2.574251347313722516 ) ) ;
#36886=CARTESIAN_POINT ( 'NONE',  ( 2.499999999999998668, -9.333333333333332149, -4.330127018922193649 ) ) ;
#36887=( BOUNDED_CURVE ( )  B_SPLINE_CURVE ( 2, ( #54516, #10439, #30052, #9480, #29401, #49361, #44531, #173, #816 ),
 .UNSPECIFIED., .F., .F. ) 
 B_SPLINE_CURVE_WITH_KNOTS ( ( 3, 2, 2, 2, 3 ),
 ( 0.1604166666666666796, 0.1611111111111111216, 0.1625000000000000056, 0.1638888888888888895, 0.1645833333333333315 ),
 .UNSPECIFIED. ) 
 CURVE ( )  GEOMETRIC_REPRESENTATION_ITEM ( )  RATIONAL_B_SPLINE_CURVE ( ( 0.9330127018922194093, 0.9330127018922207416, 1.000000000000000000, 0.8660254037844387076, 1.000000000000000000, 0.8660254037844387076, 1.000000000000000000, 0.9330127018922194093, 0.9330127018922194093 ) ) 
 REPRESENTATION_ITEM ( '' )  );
#36888=CARTESIAN_POINT ( 'NONE',  ( -6.972266317189433020E-16, 5.875000002731184168, -5.000000000000000000 ) ) ;
#36890=CARTESIAN_POINT ( 'NONE',  ( 4.458734124999999437, -47.81249999863440792, -5.460374474430324690E-16 ) ) ;
#36891=CARTESIAN_POINT ( 'NONE',  ( -2.500000000000000444, 20.83333333333333215, -4.330127018922193649 ) ) ;
#36892=EDGE_CURVE ( 'NONE', #52029, #53780, #2992, .T. ) ;
#36896=DIRECTION ( 'NONE',  ( -0.000000000000000000, 1.000000000000000000, -0.000000000000000000 ) ) ;
#36897=DIRECTION ( 'NONE',  ( 0.000000000000000000, 0.000000000000000000, 1.000000000000000000 ) ) ;
#36898=CARTESIAN_POINT ( 'NONE',  ( 4.458734124999998549, -79.97916666530107932, -2.574251347313721627 ) ) ;
#36899=DIRECTION ( 'NONE',  ( -0.000000000000000000, 1.000000000000000000, -0.000000000000000000 ) ) ;
#36902=ORIENTED_EDGE ( 'NONE', *, *, #1200, .T. ) ;
#36903=CYLINDRICAL_SURFACE ( 'NONE', #6340, 5.000000000000000000 ) ;
#36905=CARTESIAN_POINT ( 'NONE',  ( 3.535533905932738197, -168.0000000027312126, -3.535533905932738197 ) ) ;
#36907=CARTESIAN_POINT ( 'NONE',  ( 2.229367062500001939, 10.77083333469892956, 3.861377020970579999 ) ) ;
#36908=DIRECTION ( 'NONE',  ( -0.000000000000000000, 1.000000000000000000, -0.000000000000000000 ) ) ;
#36910=EDGE_CURVE ( 'NONE', #37124, #30399, #30787, .T. ) ;
#36915=CARTESIAN_POINT ( 'NONE',  ( -9.184850993605147944E-16, -146.3750000027312126, 5.000000000000000000 ) ) ;
#36916=CARTESIAN_POINT ( 'NONE',  ( 2.229367062499998831, -6.645833331967741842, -3.861377020970580887 ) ) ;
#36917=CARTESIAN_POINT ( 'NONE',  ( -9.184850993605147944E-16, -142.2500000000000284, 5.000000000000000000 ) ) ;
#36918=ORIENTED_EDGE ( 'NONE', *, *, #51676, .T. ) ;
#36919=CARTESIAN_POINT ( 'NONE',  ( 4.458734125000000326, -35.14583333196772941, 2.574251347313718519 ) ) ;
#36922=CARTESIAN_POINT ( 'NONE',  ( 1.339745962155612702, 0.8303418039926664385, -5.000000000000000000 ) ) ;
#36926=EDGE_CURVE ( 'NONE', #30862, #26215, #26453, .T. ) ;
#36927=CARTESIAN_POINT ( 'NONE',  ( -3.152801135295367096, -149.3125000013655779, -3.152801135295367541 ) ) ;
#36928=CARTESIAN_POINT ( 'NONE',  ( 2.229367062500001939, 21.02083333469892779, 3.861377020970579999 ) ) ;
#36929=CARTESIAN_POINT ( 'NONE',  ( -4.764381983412779477E-15, 27.25000000000000000, 5.000000000000000000 ) ) ;
#36930=DIRECTION ( 'NONE',  ( 0.000000000000000000, 0.000000000000000000, 1.000000000000000000 ) ) ;
#36931=CARTESIAN_POINT ( 'NONE',  ( 4.458734124999999437, -82.06249999863440792, -5.460374474430324690E-16 ) ) ;
#36933=CARTESIAN_POINT ( 'NONE',  ( 1.339745962155615144, -72.58034179853027013, 4.999999999999999112 ) ) ;
#36934=CARTESIAN_POINT ( 'NONE',  ( -3.535250795749689387E-16, 19.87500000273118417, -5.773502691896257311 ) ) ;
#36936=CARTESIAN_POINT ( 'NONE',  ( 5.000000000000000000, -35.41666666666666430, -2.886751345948130876 ) ) ;
#36939=CARTESIAN_POINT ( 'NONE',  ( 5.000000000000000000, -21.50000000000000000, -6.123233995736766282E-16 ) ) ;
#36940=CARTESIAN_POINT ( 'NONE',  ( 4.458734124999998549, -29.72916666530107221, -2.574251347313721627 ) ) ;
#36941=CARTESIAN_POINT ( 'NONE',  ( -4.458734124999997661, -89.22916666530107932, 2.574251347313722516 ) ) ;
#36942=CARTESIAN_POINT ( 'NONE',  ( 5.000000000000000000, -28.29166666393548013, -2.886751345948129988 ) ) ;
#36943=EDGE_CURVE ( 'NONE', #17113, #54593, #62157, .T. ) ;
#36944=CARTESIAN_POINT ( 'NONE',  ( 4.458734124999999437, -56.81249999863440081, -5.460374474430324690E-16 ) ) ;
#36945=EDGE_LOOP ( 'NONE', ( #37169, #37894, #1838, #59159 ) ) ;
#36946=CARTESIAN_POINT ( 'NONE',  ( 4.458734124999999437, -8.062499998634404363, -5.460374474430324690E-16 ) ) ;
#36948=CARTESIAN_POINT ( 'NONE',  ( 5.000000000000000888, -73.58333333333334281, 2.886751345948126879 ) ) ;
#36951=CARTESIAN_POINT ( 'NONE',  ( 5.000000000000000000, -76.29166666393547303, -2.886751345948129988 ) ) ;
#36952=CARTESIAN_POINT ( 'NONE',  ( -4.999999999999998224, -53.79166666393548013, 2.886751345948131764 ) ) ;
#36955=CARTESIAN_POINT ( 'NONE',  ( -2.229367062499996610, -14.39583333196774184, 3.861377020970582219 ) ) ;
#36956=CARTESIAN_POINT ( 'NONE',  ( 4.458734124999998549, -57.97916666530107221, -2.574251347313721627 ) ) ;
#36958=CARTESIAN_POINT ( 'NONE',  ( -1.846868145590737420, -139.7500000013655779, 4.458734124999999437 ) ) ;
#36962=DIRECTION ( 'NONE',  ( -0.000000000000000000, 1.000000000000000000, -0.000000000000000000 ) ) ;
#36964=CARTESIAN_POINT ( 'NONE',  ( -3.152548672688508926E-16, -0.8124999986344055847, -5.148502694627439702 ) ) ;
#36965=CARTESIAN_POINT ( 'NONE',  ( 1.975475456537005874E-15, -12.62499999726881050, 5.000000000000000000 ) ) ;
#36967=EDGE_CURVE ( 'NONE', #56591, #47541, #45897, .T. ) ;
#36970=EDGE_CURVE ( 'NONE', #41833, #42072, #46563, .T. ) ;
#36971=EDGE_CURVE ( 'NONE', #17887, #50557, #13301, .T. ) ;
#36972=CARTESIAN_POINT ( 'NONE',  ( 1.846868145590735200, -147.5000000013656063, -4.458734125000000326 ) ) ;
#36974=CARTESIAN_POINT ( 'NONE',  ( 0.000000000000000000, -170.0000000000000000, 5.000000000000000000 ) ) ;
#36976=CARTESIAN_POINT ( 'NONE',  ( 4.458734124999998549, -60.97916666530106511, -2.574251347313721627 ) ) ;
#36977=CARTESIAN_POINT ( 'NONE',  ( -6.972266317189433020E-16, -84.12499999726880162, -5.000000000000000000 ) ) ;
#36979=CARTESIAN_POINT ( 'NONE',  ( 2.730187237215162345E-16, -143.1875000013656063, -4.458734124999999437 ) ) ;
#36981=EDGE_LOOP ( 'NONE', ( #60863, #25796, #16602, #63214 ) ) ;
#36983=FACE_OUTER_BOUND ( 'NONE', #15418, .T. ) ;
#36988=CARTESIAN_POINT ( 'NONE',  ( 0.000000000000000000, -170.0000000000000000, 0.000000000000000000 ) ) ;
#36989=DIRECTION ( 'NONE',  ( -0.000000000000000000, 1.000000000000000000, -0.000000000000000000 ) ) ;
#36990=( BOUNDED_CURVE ( )  B_SPLINE_CURVE ( 2, ( #42974, #57784, #9499, #13704, #33326, #8881, #9809, #4066, #23685 ),
 .UNSPECIFIED., .F., .F. ) 
 B_SPLINE_CURVE_WITH_KNOTS ( ( 3, 2, 2, 2, 3 ),
 ( 0.7562499999999999778, 0.7569444444444444198, 0.7583333333333333037, 0.7597222222222221877, 0.7604166666666666297 ),
 .UNSPECIFIED. ) 
 CURVE ( )  GEOMETRIC_REPRESENTATION_ITEM ( )  RATIONAL_B_SPLINE_CURVE ( ( 0.9330127018922194093, 0.9330127018922194093, 1.000000000000000000, 0.8660254037844387076, 1.000000000000000000, 0.8660254037844387076, 1.000000000000000000, 0.9330127018922194093, 0.9330127018922194093 ) ) 
 REPRESENTATION_ITEM ( '' )  );
#36993=CARTESIAN_POINT ( 'NONE',  ( -9.184850993605147944E-16, -150.3750000027312126, 5.000000000000000000 ) ) ;
#36995=CARTESIAN_POINT ( 'NONE',  ( 0.000000000000000000, -170.0000000000000000, 5.000000000000000000 ) ) ;
#36997=CARTESIAN_POINT ( 'NONE',  ( -1.339745962155610925, -14.79465819873851729, 5.000000000000000000 ) ) ;
#36998=CARTESIAN_POINT ( 'NONE',  ( 4.458734124999998549, 5.270833334698926897, -2.574251347313721627 ) ) ;
#37000=CARTESIAN_POINT ( 'NONE',  ( -4.458734124999999437, -17.56249999863440792, 0.000000000000000000 ) ) ;
#37002=CARTESIAN_POINT ( 'NONE',  ( 3.152801135295367541, -160.3125000013656063, -3.152801135295367541 ) ) ;
#37006=CARTESIAN_POINT ( 'NONE',  ( -4.458734124999999437, -41.39583333196773651, -2.574251347313719407 ) ) ;
#37007=LINE ( 'NONE', #56636, #52349 ) ;
#37008=CARTESIAN_POINT ( 'NONE',  ( -3.152548672688508926E-16, -68.81249999863439371, -5.148502694627439702 ) ) ;
#37010=CARTESIAN_POINT ( 'NONE',  ( -6.972266317189433020E-16, 9.750000000000000000, -5.000000000000000000 ) ) ;
#37011=CARTESIAN_POINT ( 'NONE',  ( 5.000000000000000888, -152.0625000027312410, -2.071067811865475505 ) ) ;
#37013=CARTESIAN_POINT ( 'NONE',  ( -6.972266317189433020E-16, -85.25000000000000000, -5.000000000000000000 ) ) ;
#37014=AXIS2_PLACEMENT_3D ( 'NONE', #44220, #19785, #39393 ) ;
#37015=CARTESIAN_POINT ( 'NONE',  ( 3.535533905932736864, -144.2500000027311842, 3.535533905932738641 ) ) ;
#37016=CARTESIAN_POINT ( 'NONE',  ( -5.000000000000000000, -8.000000000000000000, 0.000000000000000000 ) ) ;
#37018=CARTESIAN_POINT ( 'NONE',  ( 4.458734125000000326, -69.89583333196773651, 2.574251347313718519 ) ) ;
#37020=CARTESIAN_POINT ( 'NONE',  ( 2.500000000000002220, -15.54166666393548191, 4.330127018922192761 ) ) ;
#37021=CARTESIAN_POINT ( 'NONE',  ( 4.458734124999998549, -38.72916666530106511, -2.574251347313721627 ) ) ;
#37022=EDGE_LOOP ( 'NONE', ( #48644, #17661, #32920, #21024 ) ) ;
#37023=CARTESIAN_POINT ( 'NONE',  ( 0.000000000000000000, -170.0000000000000000, 0.000000000000000000 ) ) ;
#37024=CARTESIAN_POINT ( 'NONE',  ( -4.458734124999999437, 5.437500001365592972, 0.000000000000000000 ) ) ;
#37026=CARTESIAN_POINT ( 'NONE',  ( -9.184850993605147944E-16, -151.2500000000000284, 5.000000000000000000 ) ) ;
#37027=CARTESIAN_POINT ( 'NONE',  ( 2.500000000000002220, -57.66666666666667140, 4.330127018922192761 ) ) ;
#37028=CARTESIAN_POINT ( 'NONE',  ( -1.846868145590734756, -160.3750000013656063, -4.458734125000000326 ) ) ;
#37031=CARTESIAN_POINT ( 'NONE',  ( 9.457646018065525792E-16, -82.06249999863442213, 5.148502694627439702 ) ) ;
#37032=CARTESIAN_POINT ( 'NONE',  ( 2.071067811865475505, -164.8124999999999716, -5.000000000000000888 ) ) ;
#37033=CARTESIAN_POINT ( 'NONE',  ( -2.229367062500000163, -87.47916666530107932, -3.861377020970580443 ) ) ;
#37035=CARTESIAN_POINT ( 'NONE',  ( 9.457646018065525792E-16, 1.687500001365593194, 5.148502694627439702 ) ) ;
#37036=CARTESIAN_POINT ( 'NONE',  ( 2.229367062499998831, -35.89583333196773651, -3.861377020970580887 ) ) ;
#37043=( BOUNDED_CURVE ( )  B_SPLINE_CURVE ( 2, ( #27904, #56880, #52050, #47525, #62336, #18257, #2532, #23089, #7988 ),
 .UNSPECIFIED., .F., .F. ) 
 B_SPLINE_CURVE_WITH_KNOTS ( ( 3, 2, 2, 2, 3 ),
 ( 0.6854166666666666741, 0.6861111111111111160, 0.6875000000000000000, 0.6888888888888888840, 0.6895833333333333259 ),
 .UNSPECIFIED. ) 
 CURVE ( )  GEOMETRIC_REPRESENTATION_ITEM ( )  RATIONAL_B_SPLINE_CURVE ( ( 0.9330127018922194093, 0.9330127018922194093, 1.000000000000000000, 0.8660254037844387076, 1.000000000000000000, 0.8660254037844387076, 1.000000000000000000, 0.9330127018922194093, 0.9330127018922194093 ) ) 
 REPRESENTATION_ITEM ( '' )  );
#37044=CARTESIAN_POINT ( 'NONE',  ( -4.458734124999999437, -71.56249999863439371, 0.000000000000000000 ) ) ;
#37046=ORIENTED_EDGE ( 'NONE', *, *, #57810, .F. ) ;
#37047=CARTESIAN_POINT ( 'NONE',  ( -2.071067811865348496, -150.8125000027311842, -5.000000000000127898 ) ) ;
#37049=CARTESIAN_POINT ( 'NONE',  ( -6.972266317189433020E-16, -3.124999997268813612, -5.000000000000000000 ) ) ;
#37051=CARTESIAN_POINT ( 'NONE',  ( -5.147856630858197489E-14, 3.249999999999997335, 5.000000000000000000 ) ) ;
#37052=CARTESIAN_POINT ( 'NONE',  ( 2.229367062500001939, 3.020833334698928674, 3.861377020970579999 ) ) ;
#37054=CARTESIAN_POINT ( 'NONE',  ( -4.999999999999998224, -32.79166666393547303, 2.886751345948131764 ) ) ;
#37055=CARTESIAN_POINT ( 'NONE',  ( 1.846868145590735200, -158.2500000013656063, -4.458734124999999437 ) ) ;
#37056=EDGE_CURVE ( 'NONE', #9299, #17113, #37534, .T. ) ;
#37062=AXIS2_PLACEMENT_3D ( 'NONE', #30261, #49883, #50853 ) ;
#37063=EDGE_CURVE ( 'NONE', #35844, #41033, #44089, .T. ) ;
#37064=CARTESIAN_POINT ( 'NONE',  ( 0.000000000000000000, -170.0000000000000000, 0.000000000000000000 ) ) ;
#37065=EDGE_CURVE ( 'NONE', #14611, #34762, #42017, .T. ) ;
#37069=CARTESIAN_POINT ( 'NONE',  ( 0.000000000000000000, -170.0000000000000000, 0.000000000000000000 ) ) ;
#37071=CARTESIAN_POINT ( 'NONE',  ( 1.339745962155661996, -10.29465819873852261, -4.999999999999970690 ) ) ;
#37073=CARTESIAN_POINT ( 'NONE',  ( -4.458734124999999437, 23.60416666803225993, -2.574251347313719407 ) ) ;
#37074=EDGE_CURVE ( 'NONE', #21757, #16025, #57280, .T. ) ;
#37076=CARTESIAN_POINT ( 'NONE',  ( 4.458734124999999437, -2.062499998634406584, -5.460374474430324690E-16 ) ) ;
#37077=CARTESIAN_POINT ( 'NONE',  ( -9.184850993605147944E-16, -161.3750000027311842, 5.000000000000000000 ) ) ;
#37080=CARTESIAN_POINT ( 'NONE',  ( 2.071067811865476394, -141.3125000027312126, 5.000000000000000000 ) ) ;
#37081=CARTESIAN_POINT ( 'NONE',  ( -4.999999999999998224, -51.91666666666666430, 2.886751345948131764 ) ) ;
#37085=DIRECTION ( 'NONE',  ( -0.000000000000000000, 1.000000000000000000, -0.000000000000000000 ) ) ;
#37086=EDGE_CURVE ( 'NONE', #10357, #26556, #44539, .T. ) ;
#37087=CARTESIAN_POINT ( 'NONE',  ( 5.000000000000000888, 3.416666666666665186, 2.886751345948126879 ) ) ;
#37089=CARTESIAN_POINT ( 'NONE',  ( 2.730187237215162345E-16, -159.4375000013655779, -4.458734124999999437 ) ) ;
#37091=ORIENTED_EDGE ( 'NONE', *, *, #44530, .F. ) ;
#37092=CARTESIAN_POINT ( 'NONE',  ( -2.229367062500000163, 15.27083333469892779, -3.861377020970580443 ) ) ;
#37093=ORIENTED_EDGE ( 'NONE', *, *, #61227, .T. ) ;
#37097=( BOUNDED_CURVE ( )  B_SPLINE_CURVE ( 2, ( #36557, #45573, #60704, #6661, #56188, #51365, #16624, #26268, #30781 ),
 .UNSPECIFIED., .F., .T. ) 
 B_SPLINE_CURVE_WITH_KNOTS ( ( 3, 2, 2, 2, 3 ),
 ( 0.2750000000000002442, 0.2791666666666668961, 0.2833333333333335480, 0.2875000000000001998, 0.2916666666666669072 ),
 .UNSPECIFIED. ) 
 CURVE ( )  GEOMETRIC_REPRESENTATION_ITEM ( )  RATIONAL_B_SPLINE_CURVE ( ( 0.9999999999999958922, 0.9238795325112908463, 1.000000000000000000, 0.9238795325112867385, 1.000000000000000000, 0.9238795325112867385, 1.000000000000000000, 0.9238795325112826307, 1.000000000000003997 ) ) 
 REPRESENTATION_ITEM ( '' )  );
#37098=CARTESIAN_POINT ( 'NONE',  ( 1.975475456537005874E-15, -16.74999999999999645, 5.000000000000000000 ) ) ;
#37099=CARTESIAN_POINT ( 'NONE',  ( -5.000000000000000000, 5.999999999999998224, 0.000000000000000000 ) ) ;
#37100=CARTESIAN_POINT ( 'NONE',  ( 4.458734125000000326, -55.89583333196773651, 2.574251347313718519 ) ) ;
#37101=CARTESIAN_POINT ( 'NONE',  ( -1.339745962155613812, -53.08034179853029144, -5.000000000000000000 ) ) ;
#37103=CYLINDRICAL_SURFACE ( 'NONE', #7777, 5.000000000000000000 ) ;
#37107=CARTESIAN_POINT ( 'NONE',  ( -5.000000000000000000, -37.99999999999999289, 0.000000000000000000 ) ) ;
#37111=CARTESIAN_POINT ( 'NONE',  ( -1.339745962155610925, 13.20534180126147916, 5.000000000000000000 ) ) ;
#37112=CARTESIAN_POINT ( 'NONE',  ( 2.229367062499998831, -65.64583333196773651, -3.861377020970580887 ) ) ;
#37113=CARTESIAN_POINT ( 'NONE',  ( 4.458734124999999437, -149.6875000013656063, 0.000000000000000000 ) ) ;
#37114=AXIS2_PLACEMENT_3D ( 'NONE', #7319, #50729, #6673 ) ;
#37115=CARTESIAN_POINT ( 'NONE',  ( -4.458734124999999437, -70.31249999863439371, 0.000000000000000000 ) ) ;
#37117=CARTESIAN_POINT ( 'NONE',  ( 2.229367062499998831, -19.89583333196774007, -3.861377020970580887 ) ) ;
#37118=CARTESIAN_POINT ( 'NONE',  ( -5.000000000000000000, -59.87499999726880873, 0.000000000000000000 ) ) ;
#37119=ORIENTED_EDGE ( 'NONE', *, *, #4672, .T. ) ;
#37121=ORIENTED_EDGE ( 'NONE', *, *, #11984, .F. ) ;
#37123=CARTESIAN_POINT ( 'NONE',  ( 0.000000000000000000, -170.0000000000000000, 0.000000000000000000 ) ) ;
#37124=VERTEX_POINT ( 'NONE', #48725 ) ;
#37126=LINE ( 'NONE', #17176, #60074 ) ;
#37128=CARTESIAN_POINT ( 'NONE',  ( 2.229367062500001939, -55.22916666530107221, 3.861377020970579999 ) ) ;
#37130=ORIENTED_EDGE ( 'NONE', *, *, #51074, .T. ) ;
#37131=LINE ( 'NONE', #56750, #39833 ) ;
#37133=CARTESIAN_POINT ( 'NONE',  ( 2.229367062500001939, 16.02083333469892779, 3.861377020970579999 ) ) ;
#37136=CARTESIAN_POINT ( 'NONE',  ( 4.458734124999999437, -167.4375000013655779, 0.000000000000000000 ) ) ;
#37139=CARTESIAN_POINT ( 'NONE',  ( -5.000000000000000000, -85.87499999726880162, 0.000000000000000000 ) ) ;
#37145=CARTESIAN_POINT ( 'NONE',  ( 3.535533905932736864, -161.1250000000000284, 3.535533905932738641 ) ) ;
#37149=ORIENTED_EDGE ( 'NONE', *, *, #57099, .T. ) ;
#37152=CARTESIAN_POINT ( 'NONE',  ( -9.184850993605147944E-16, -153.3750000027311842, 5.000000000000000000 ) ) ;
#37155=VECTOR ( 'NONE', #11809, 1000.000000000000000 ) ;
#37159=CARTESIAN_POINT ( 'NONE',  ( -2.071067811865475061, -145.6875000000000000, -5.000000000000000888 ) ) ;
#37160=EDGE_CURVE ( 'NONE', #42868, #871, #20255, .T. ) ;
#37164=CARTESIAN_POINT ( 'NONE',  ( -4.458734124999999437, -25.39583333196773651, -2.574251347313719407 ) ) ;
#37166=CARTESIAN_POINT ( 'NONE',  ( -2.499999999999996447, 9.291666669397853795, 4.330127018922195425 ) ) ;
#37168=CARTESIAN_POINT ( 'NONE',  ( 2.730187237215162345E-16, -149.1875000013656063, -4.458734124999999437 ) ) ;
#37169=ORIENTED_EDGE ( 'NONE', *, *, #42774, .F. ) ;
#37171=CARTESIAN_POINT ( 'NONE',  ( 2.229367062499998831, -53.89583333196773651, -3.861377020970580887 ) ) ;
#37172=VECTOR ( 'NONE', #34807, 1000.000000000000000 ) ;
#37174=CARTESIAN_POINT ( 'NONE',  ( -3.535250795749689387E-16, 25.74999999999999645, -5.773502691896257311 ) ) ;
#37175=( BOUNDED_CURVE ( )  B_SPLINE_CURVE ( 2, ( #46108, #15888, #36456, #51267, #25533, #45791, #1750, #35508, #7200 ),
 .UNSPECIFIED., .F., .F. ) 
 B_SPLINE_CURVE_WITH_KNOTS ( ( 3, 2, 2, 2, 3 ),
 ( 0.2395833333333333426, 0.2402777777777777846, 0.2416666666666666685, 0.2430555555555555525, 0.2437499999999999944 ),
 .UNSPECIFIED. ) 
 CURVE ( )  GEOMETRIC_REPRESENTATION_ITEM ( )  RATIONAL_B_SPLINE_CURVE ( ( 0.9330127018922194093, 0.9330127018922194093, 1.000000000000000000, 0.8660254037844387076, 1.000000000000000000, 0.8660254037844387076, 1.000000000000000000, 0.9330127018922194093, 0.9330127018922194093 ) ) 
 REPRESENTATION_ITEM ( '' )  );
#37176=CARTESIAN_POINT ( 'NONE',  ( -3.152548672688508926E-16, -1.562499998634406140, -5.148502694627439702 ) ) ;
#37179=CARTESIAN_POINT ( 'NONE',  ( -4.458734124999999437, 11.35416666803225993, -2.574251347313719407 ) ) ;
#37182=VERTEX_POINT ( 'NONE', #19461 ) ;
#37183=CARTESIAN_POINT ( 'NONE',  ( 2.071067811865484387, -168.3125000027312126, 4.999999999999991118 ) ) ;
#37184=CARTESIAN_POINT ( 'NONE',  ( -3.152548672688508926E-16, -47.56249999863440792, -5.148502694627439702 ) ) ;
#37185=CARTESIAN_POINT ( 'NONE',  ( 4.458734124999999437, -163.7500000013655779, 1.846868145590737864 ) ) ;
#37187=CARTESIAN_POINT ( 'NONE',  ( -4.999999999999999112, -43.79166666393546592, 2.886751345948131764 ) ) ;
#37189=CARTESIAN_POINT ( 'NONE',  ( -3.152548672688508926E-16, -25.56249999863440436, -5.148502694627439702 ) ) ;
#37192=CARTESIAN_POINT ( 'NONE',  ( -4.458734125000000326, -165.0000000013655779, -1.846868145590735644 ) ) ;
#37195=CARTESIAN_POINT ( 'NONE',  ( 2.229367062500001939, -39.22916666530107221, 3.861377020970579999 ) ) ;
#37196=CARTESIAN_POINT ( 'NONE',  ( 3.061616997868383141E-16, -163.7500000000000000, -5.000000000000000000 ) ) ;
#37197=ORIENTED_EDGE ( 'NONE', *, *, #40175, .F. ) ;
#37200=CARTESIAN_POINT ( 'NONE',  ( 2.500000000000002220, 24.45833333606451987, 4.330127018922192761 ) ) ;
#37204=CARTESIAN_POINT ( 'NONE',  ( -4.458734124999999437, -80.64583333196773651, -2.574251347313719407 ) ) ;
#37206=CARTESIAN_POINT ( 'NONE',  ( 2.071067811865392461, -143.1875000000000568, 5.000000000000084377 ) ) ;
#37208=CARTESIAN_POINT ( 'NONE',  ( -5.000000000000000000, -44.95833333060214443, -2.886751345948128211 ) ) ;
#37213=LINE ( 'NONE', #51053, #33010 ) ;
#37216=CARTESIAN_POINT ( 'NONE',  ( 1.975475456537005874E-15, -72.75000000000000000, 5.000000000000000000 ) ) ;
#37218=CARTESIAN_POINT ( 'NONE',  ( -4.458734124999999437, -80.56249999863440792, 0.000000000000000000 ) ) ;
#37224=CARTESIAN_POINT ( 'NONE',  ( 5.000000000000000000, -166.1250000027312126, 0.000000000000000000 ) ) ;
#37226=CARTESIAN_POINT ( 'NONE',  ( 2.229367062499998831, 14.10416666803226171, -3.861377020970580887 ) ) ;
#37227=LINE ( 'NONE', #61362, #60306 ) ;
#37233=CARTESIAN_POINT ( 'NONE',  ( -5.000000000000000000, -21.95833333060214798, -2.886751345948128211 ) ) ;
#37234=CARTESIAN_POINT ( 'NONE',  ( -4.458734124999999437, -8.312499998634406140, 0.000000000000000000 ) ) ;
#37237=CARTESIAN_POINT ( 'NONE',  ( 4.458734125000000326, -36.14583333196773651, 2.574251347313718519 ) ) ;
#37243=CARTESIAN_POINT ( 'NONE',  ( 4.458734124999997661, -149.7500000013656063, 1.846868145590737864 ) ) ;
#37244=CARTESIAN_POINT ( 'NONE',  ( 9.457646018065525792E-16, 14.93750000136559564, 5.148502694627439702 ) ) ;
#37246=CARTESIAN_POINT ( 'NONE',  ( 2.229367062500001939, -83.22916666530106511, 3.861377020970579999 ) ) ;
#37248=CARTESIAN_POINT ( 'NONE',  ( 1.975475456537005874E-15, -1.624999997268813834, 5.000000000000000000 ) ) ;
#37249=CARTESIAN_POINT ( 'NONE',  ( 2.500000000000002220, 21.45833333606451987, 4.330127018922192761 ) ) ;
#37250=ORIENTED_EDGE ( 'NONE', *, *, #25920, .T. ) ;
#37251=CARTESIAN_POINT ( 'NONE',  ( 0.000000000000000000, -170.0000000000000000, 0.000000000000000000 ) ) ;
#37252=CARTESIAN_POINT ( 'NONE',  ( -3.535250795749689387E-16, -28.24999999999999645, -5.773502691896257311 ) ) ;
#37253=CARTESIAN_POINT ( 'NONE',  ( -4.458734124999999437, -34.39583333196772941, -2.574251347313719407 ) ) ;
#37256=CARTESIAN_POINT ( 'NONE',  ( -2.499999999999996447, -27.70833333060214798, 4.330127018922195425 ) ) ;
#37257=CARTESIAN_POINT ( 'NONE',  ( 4.458734124999999437, -59.81249999863440081, -5.460374474430324690E-16 ) ) ;
#37258=ORIENTED_EDGE ( 'NONE', *, *, #49603, .F. ) ;
#37259=CARTESIAN_POINT ( 'NONE',  ( 6.123233995736766282E-16, -170.0000000000000000, -5.000000000000000000 ) ) ;
#37260=CARTESIAN_POINT ( 'NONE',  ( 4.458734124999999437, -11.06249999863440792, -5.460374474430324690E-16 ) ) ;
#37262=CARTESIAN_POINT ( 'NONE',  ( 1.060575238724906964E-15, -71.75000000000000000, 5.773502691896257311 ) ) ;
#37265=( BOUNDED_CURVE ( )  B_SPLINE_CURVE ( 2, ( #29817, #49450, #5392, #25009, #1538, #12441, #11486, #21143, #27234 ),
 .UNSPECIFIED., .F., .F. ) 
 B_SPLINE_CURVE_WITH_KNOTS ( ( 3, 2, 2, 2, 3 ),
 ( 0.01458333333333333356, 0.01527777777777777728, 0.01666666666666666644, 0.01805555555555555386, 0.01874999999999999931 ),
 .UNSPECIFIED. ) 
 CURVE ( )  GEOMETRIC_REPRESENTATION_ITEM ( )  RATIONAL_B_SPLINE_CURVE ( ( 0.9330127018922192983, 0.9330127018922194093, 1.000000000000000000, 0.8660254037844387076, 1.000000000000000000, 0.8660254037844387076, 1.000000000000000000, 0.9330127018922194093, 0.9330127018922194093 ) ) 
 REPRESENTATION_ITEM ( '' )  );
#37266=CARTESIAN_POINT ( 'NONE',  ( 2.500000000000002220, -78.54166666393547303, 4.330127018922192761 ) ) ;
#37267=CARTESIAN_POINT ( 'NONE',  ( 2.499999999999998668, -13.33333333333333570, -4.330127018922193649 ) ) ;
#37268=ORIENTED_EDGE ( 'NONE', *, *, #3313, .T. ) ;
#37270=CARTESIAN_POINT ( 'NONE',  ( 2.229367062499998831, -18.89583333196774007, -3.861377020970580887 ) ) ;
#37271=CARTESIAN_POINT ( 'NONE',  ( -3.152548672688508926E-16, -56.81249999863439371, -5.148502694627439702 ) ) ;
#37273=CARTESIAN_POINT ( 'NONE',  ( -2.500000000000000444, -24.16666666666666430, -4.330127018922193649 ) ) ;
#37274=CARTESIAN_POINT ( 'NONE',  ( -4.458734124999999437, -141.9375000013656063, -5.460374474430324690E-16 ) ) ;
#37280=CARTESIAN_POINT ( 'NONE',  ( -1.339745962155564296, -13.08034179853029499, -5.000000000000028422 ) ) ;
#37283=CARTESIAN_POINT ( 'NONE',  ( -8.190561711645485556E-16, -149.9375000013656063, 4.458734124999999437 ) ) ;
#37287=CARTESIAN_POINT ( 'NONE',  ( 2.229367062500001939, -64.22916666530106511, 3.861377020970579999 ) ) ;
#37290=CARTESIAN_POINT ( 'NONE',  ( 2.730187237215162345E-16, -146.1875000013656063, -4.458734124999999437 ) ) ;
#37299=CARTESIAN_POINT ( 'NONE',  ( 9.457646018065525792E-16, 26.68750000136559564, 5.148502694627439702 ) ) ;
#37303=CARTESIAN_POINT ( 'NONE',  ( 1.339745962155612702, -56.16965819600733312, -5.000000000000000000 ) ) ;
#37304=LINE ( 'NONE', #22524, #45922 ) ;
#37305=CARTESIAN_POINT ( 'NONE',  ( 9.457646018065525792E-16, 5.937500001365593860, 5.148502694627439702 ) ) ;
#37307=CARTESIAN_POINT ( 'NONE',  ( -4.458734124999997661, -20.47916666530107577, 2.574251347313722516 ) ) ;
#37309=CARTESIAN_POINT ( 'NONE',  ( 2.730187237215162345E-16, -160.1875000013655779, -4.458734124999999437 ) ) ;
#37310=CARTESIAN_POINT ( 'NONE',  ( 6.972266317189433020E-16, 28.87500000273118417, -5.000000000000000000 ) ) ;
#37314=CARTESIAN_POINT ( 'NONE',  ( -2.229367062499996610, -42.14583333196773651, 3.861377020970582219 ) ) ;
#37316=CARTESIAN_POINT ( 'NONE',  ( 4.458734124999999437, -69.06249999863439371, -5.460374474430324690E-16 ) ) ;
#37318=CARTESIAN_POINT ( 'NONE',  ( 5.000000000000000000, -57.29166666393548013, -2.886751345948130876 ) ) ;
#37319=CARTESIAN_POINT ( 'NONE',  ( 6.123233995736766282E-16, -170.0000000000000000, -5.000000000000000000 ) ) ;
#37320=ORIENTED_EDGE ( 'NONE', *, *, #18155, .F. ) ;
#37322=CARTESIAN_POINT ( 'NONE',  ( 1.339745962155612702, -89.16965819600733312, -5.000000000000000000 ) ) ;
#37323=CARTESIAN_POINT ( 'NONE',  ( -2.500000000000000444, -6.166666666666667851, -4.330127018922193649 ) ) ;
#37325=CARTESIAN_POINT ( 'NONE',  ( -2.229367062499996610, -79.14583333196773651, 3.861377020970582219 ) ) ;
#37327=CARTESIAN_POINT ( 'NONE',  ( 5.000000000000000888, -12.45833333060214976, 2.886751345948126879 ) ) ;
#37328=CARTESIAN_POINT ( 'NONE',  ( -3.152548672688508926E-16, -42.56249999863440792, -5.148502694627439702 ) ) ;
#37330=CARTESIAN_POINT ( 'NONE',  ( 9.457646018065525792E-16, 4.687500001365596525, 5.148502694627439702 ) ) ;
#37331=VERTEX_POINT ( 'NONE', #34562 ) ;
#37333=CARTESIAN_POINT ( 'NONE',  ( 2.499999999999998668, -58.33333333333333570, -4.330127018922193649 ) ) ;
#37334=CARTESIAN_POINT ( 'NONE',  ( 4.458734124999999437, -158.7500000013656063, 1.846868145590737864 ) ) ;
#37336=CARTESIAN_POINT ( 'NONE',  ( -5.000000000000000000, -35.08333333333332860, -2.886751345948128211 ) ) ;
#37337=CARTESIAN_POINT ( 'NONE',  ( 4.458734124999998549, -80.72916666530106511, -2.574251347313721627 ) ) ;
#37338=CARTESIAN_POINT ( 'NONE',  ( -2.071067811865478170, -168.3125000000000000, 5.000000000000000000 ) ) ;
#37339=EDGE_CURVE ( 'NONE', #26215, #9342, #33029, .T. ) ;
#37340=CARTESIAN_POINT ( 'NONE',  ( 2.229367062500001939, -89.97916666530106511, 3.861377020970579999 ) ) ;
#37342=CARTESIAN_POINT ( 'NONE',  ( 2.229367062500001939, -2.229166665301068662, 3.861377020970579999 ) ) ;
#37343=CARTESIAN_POINT ( 'NONE',  ( -4.458734124999999437, -40.56249999863440081, 0.000000000000000000 ) ) ;
#37345=CARTESIAN_POINT ( 'NONE',  ( 6.123233995736766282E-16, -170.0000000000000000, -5.000000000000000000 ) ) ;
#37348=CARTESIAN_POINT ( 'NONE',  ( 5.000000000000000000, -86.41666666666667140, -2.886751345948130876 ) ) ;
#37352=CARTESIAN_POINT ( 'NONE',  ( 1.975475456537005874E-15, -68.62499999726881583, 5.000000000000000000 ) ) ;
#37353=CARTESIAN_POINT ( 'NONE',  ( -4.458734124999998549, -72.47916666530107932, 2.574251347313722516 ) ) ;
#37357=CYLINDRICAL_SURFACE ( 'NONE', #16397, 5.000000000000000000 ) ;
#37362=CARTESIAN_POINT ( 'NONE',  ( 4.458734125000001214, 5.104166668032261711, 2.574251347313718519 ) ) ;
#37363=CARTESIAN_POINT ( 'NONE',  ( -5.000000000000000000, -80.00000000000000000, 0.000000000000000000 ) ) ;
#37364=CARTESIAN_POINT ( 'NONE',  ( 2.730187237215162345E-16, -157.1875000013655779, -4.458734124999999437 ) ) ;
#37366=VERTEX_POINT ( 'NONE', #54840 ) ;
#37376=CARTESIAN_POINT ( 'NONE',  ( 2.229367062500001939, 21.02083333469892779, 3.861377020970579999 ) ) ;
#37378=CARTESIAN_POINT ( 'NONE',  ( 4.458734125000000326, -1.145833331967740287, 2.574251347313718519 ) ) ;
#37379=CARTESIAN_POINT ( 'NONE',  ( -2.499999999999996447, -33.70833333060213732, 4.330127018922195425 ) ) ;
#37381=CARTESIAN_POINT ( 'NONE',  ( 3.535533905932736864, -141.2500000027311842, 3.535533905932738641 ) ) ;
#37386=AXIS2_PLACEMENT_3D ( 'NONE', #44837, #30040, #54820 ) ;
#37387=DIRECTION ( 'NONE',  ( -0.000000000000000000, 1.000000000000000000, -0.000000000000000000 ) ) ;
#37388=CARTESIAN_POINT ( 'NONE',  ( 0.000000000000000000, -170.0000000000000000, 5.000000000000000000 ) ) ;
#37390=CARTESIAN_POINT ( 'NONE',  ( 4.458734124999999437, -156.6875000013655779, 0.000000000000000000 ) ) ;
#37394=CARTESIAN_POINT ( 'NONE',  ( 4.458734125000001214, 18.85416666803226349, 2.574251347313718519 ) ) ;
#37400=CARTESIAN_POINT ( 'NONE',  ( 1.060575238724906964E-15, 8.250000000000000000, 5.773502691896257311 ) ) ;
#37401=CARTESIAN_POINT ( 'NONE',  ( 4.458734124999999437, -55.81249999863440081, -5.460374474430324690E-16 ) ) ;
#37402=CARTESIAN_POINT ( 'NONE',  ( -4.999999999999998224, -7.916666666666668739, 2.886751345948131764 ) ) ;
#37404=EDGE_CURVE ( 'NONE', #24529, #7439, #13674, .T. ) ;
#37406=CARTESIAN_POINT ( 'NONE',  ( 4.458734124999999437, -28.81249999863440436, -5.460374474430324690E-16 ) ) ;
#37407=CARTESIAN_POINT ( 'NONE',  ( 2.071067811865645591, -153.3125000027311557, 4.999999999999830358 ) ) ;
#37411=CARTESIAN_POINT ( 'NONE',  ( 2.499999999999998668, -41.33333333333333570, -4.330127018922193649 ) ) ;
#37412=CARTESIAN_POINT ( 'NONE',  ( 2.071067811865644703, -148.8125000000000000, -4.999999999999831246 ) ) ;
#37417=CARTESIAN_POINT ( 'NONE',  ( 2.229367062500001939, -65.97916666530106511, 3.861377020970579999 ) ) ;
#37418=CARTESIAN_POINT ( 'NONE',  ( -4.458734125000001214, -149.1250000013656063, 1.846868145590734089 ) ) ;
#37419=CARTESIAN_POINT ( 'NONE',  ( -3.152548672688508926E-16, -72.56249999863439371, -5.148502694627439702 ) ) ;
#37421=EDGE_CURVE ( 'NONE', #40520, #51921, #12596, .T. ) ;
#37422=CARTESIAN_POINT ( 'NONE',  ( -4.458734124999999437, -25.56249999863440792, 0.000000000000000000 ) ) ;
#37423=CARTESIAN_POINT ( 'NONE',  ( -2.500000000000000444, -59.04166666393546592, -4.330127018922193649 ) ) ;
#37424=ORIENTED_EDGE ( 'NONE', *, *, #60243, .F. ) ;
#37429=CARTESIAN_POINT ( 'NONE',  ( 2.071067811865644703, -148.9375000027312410, -4.999999999999831246 ) ) ;
#37430=ADVANCED_FACE ( 'NONE', ( #50004 ), #56680, .F. ) ;
#37431=ORIENTED_EDGE ( 'NONE', *, *, #15862, .T. ) ;
#37435=CARTESIAN_POINT ( 'NONE',  ( 4.458734124999998549, -53.97916666530107221, -2.574251347313721627 ) ) ;
#37436=EDGE_LOOP ( 'NONE', ( #27829, #1904, #51975, #53101 ) ) ;
#37437=VECTOR ( 'NONE', #18098, 1000.000000000000000 ) ;
#37440=CARTESIAN_POINT ( 'NONE',  ( -2.229367062500000163, 20.52083333469892779, -3.861377020970580443 ) ) ;
#37446=CARTESIAN_POINT ( 'NONE',  ( -5.000000000000000000, -85.95833333060214443, -2.886751345948128211 ) ) ;
#37448=CARTESIAN_POINT ( 'NONE',  ( 5.000000000000000000, -69.37499999726880162, -6.123233995736766282E-16 ) ) ;
#37452=DIRECTION ( 'NONE',  ( -0.000000000000000000, 1.000000000000000000, -0.000000000000000000 ) ) ;
#37457=( BOUNDED_CURVE ( )  B_SPLINE_CURVE ( 2, ( #27391, #47024, #2973, #27711, #3288, #4522, #48581, #18686, #9978 ),
 .UNSPECIFIED., .F., .F. ) 
 B_SPLINE_CURVE_WITH_KNOTS ( ( 3, 2, 2, 2, 3 ),
 ( 0.6395833333333332815, 0.6402777777777777235, 0.6416666666666667185, 0.6430555555555556024, 0.6437500000000000444 ),
 .UNSPECIFIED. ) 
 CURVE ( )  GEOMETRIC_REPRESENTATION_ITEM ( )  RATIONAL_B_SPLINE_CURVE ( ( 0.9330127018922194093, 0.9330127018922194093, 1.000000000000000000, 0.8660254037844387076, 1.000000000000000000, 0.8660254037844387076, 1.000000000000000000, 0.9330127018922194093, 0.9330127018922194093 ) ) 
 REPRESENTATION_ITEM ( '' )  );
#37460=CARTESIAN_POINT ( 'NONE',  ( 5.000000000000000000, -154.1875000027312126, 2.071067811865478614 ) ) ;
#37466=CARTESIAN_POINT ( 'NONE',  ( -5.000000000000000888, -145.5625000000000568, -2.071067811865475949 ) ) ;
#37469=CARTESIAN_POINT ( 'NONE',  ( -3.152801135295367985, -169.0625000013656063, 3.152801135295367096 ) ) ;
#37470=CARTESIAN_POINT ( 'NONE',  ( -2.229367062500000163, -26.47916666530106866, -3.861377020970580443 ) ) ;
#37471=CARTESIAN_POINT ( 'NONE',  ( 2.499999999999998668, 14.66666666666666607, -4.330127018922193649 ) ) ;
#37473=CARTESIAN_POINT ( 'NONE',  ( -3.152801135295367096, -149.0625000013655779, -3.152801135295367541 ) ) ;
#37476=CARTESIAN_POINT ( 'NONE',  ( -4.458734124999997661, -50.47916666530107221, 2.574251347313722516 ) ) ;
#37477=FACE_OUTER_BOUND ( 'NONE', #15181, .T. ) ;
#37478=CARTESIAN_POINT ( 'NONE',  ( 5.000000000000000000, 24.50000000000000000, -6.123233995736766282E-16 ) ) ;
#37481=CARTESIAN_POINT ( 'NONE',  ( 2.229367062500001939, -2.979166665301069550, 3.861377020970579999 ) ) ;
#37482=CARTESIAN_POINT ( 'NONE',  ( 1.975475456537005874E-15, 19.25000000000000000, 5.000000000000000000 ) ) ;
#37484=CARTESIAN_POINT ( 'NONE',  ( -2.229367062499996610, 8.604166668032261711, 3.861377020970582219 ) ) ;
#37488=CARTESIAN_POINT ( 'NONE',  ( -6.972266317189433020E-16, -71.25000000000000000, -5.000000000000000000 ) ) ;
#37489=CARTESIAN_POINT ( 'NONE',  ( 2.229367062500001939, -49.97916666530107221, 3.861377020970579999 ) ) ;
#37490=CARTESIAN_POINT ( 'NONE',  ( -1.846868145590734756, -158.3750000013655779, -4.458734125000000326 ) ) ;
#37491=CARTESIAN_POINT ( 'NONE',  ( 2.500000000000002220, -46.54166666393547303, 4.330127018922192761 ) ) ;
#37492=ORIENTED_EDGE ( 'NONE', *, *, #41340, .F. ) ;
#37493=CARTESIAN_POINT ( 'NONE',  ( 4.458734125000001214, -23.89583333196774007, 2.574251347313718519 ) ) ;
#37494=ORIENTED_EDGE ( 'NONE', *, *, #32321, .F. ) ;
#37496=CARTESIAN_POINT ( 'NONE',  ( 4.458734124999999437, -159.5000000013655779, 1.846868145590737864 ) ) ;
#37501=CARTESIAN_POINT ( 'NONE',  ( -3.152548672688508926E-16, -39.81249999863440081, -5.148502694627439702 ) ) ;
#37502=DIRECTION ( 'NONE',  ( 0.000000000000000000, 0.000000000000000000, 1.000000000000000000 ) ) ;
#37503=ORIENTED_EDGE ( 'NONE', *, *, #34846, .T. ) ;
#37507=CARTESIAN_POINT ( 'NONE',  ( 2.500000000000002220, -24.54166666393548368, 4.330127018922192761 ) ) ;
#37508=ORIENTED_EDGE ( 'NONE', *, *, #35089, .F. ) ;
#37510=CARTESIAN_POINT ( 'NONE',  ( 9.457646018065525792E-16, -87.31249999863440792, 5.148502694627439702 ) ) ;
#37513=CARTESIAN_POINT ( 'NONE',  ( -3.535533905932738641, -158.5000000027312126, 3.535533905932737309 ) ) ;
#37516=CARTESIAN_POINT ( 'NONE',  ( -5.000000000000000000, -84.87499999726880162, 0.000000000000000000 ) ) ;
#37519=CARTESIAN_POINT ( 'NONE',  ( -6.972266317189433020E-16, -22.24999999999999645, -5.000000000000000000 ) ) ;
#37522=DIRECTION ( 'NONE',  ( 0.000000000000000000, 0.000000000000000000, 1.000000000000000000 ) ) ;
#37523=CARTESIAN_POINT ( 'NONE',  ( 6.123233995736766282E-16, -170.0000000000000000, -5.000000000000000000 ) ) ;
#37524=CARTESIAN_POINT ( 'NONE',  ( 2.229367062500001939, -84.22916666530107932, 3.861377020970579999 ) ) ;
#37527=ORIENTED_EDGE ( 'NONE', *, *, #6767, .T. ) ;
#37530=CARTESIAN_POINT ( 'NONE',  ( 2.071067811865475505, -164.9375000027312126, -5.000000000000000888 ) ) ;
#37532=CARTESIAN_POINT ( 'NONE',  ( 2.229367062500001939, 12.77083333469892779, 3.861377020970579999 ) ) ;
#37534=( BOUNDED_CURVE ( )  B_SPLINE_CURVE ( 2, ( #57467, #62290, #27542, #28170, #52625, #8558, #3743, #23365, #8255 ),
 .UNSPECIFIED., .F., .F. ) 
 B_SPLINE_CURVE_WITH_KNOTS ( ( 3, 2, 2, 2, 3 ),
 ( 0.7270833333333333037, 0.7277777777777777457, 0.7291666666666666297, 0.7305555555555555136, 0.7312499999999999556 ),
 .UNSPECIFIED. ) 
 CURVE ( )  GEOMETRIC_REPRESENTATION_ITEM ( )  RATIONAL_B_SPLINE_CURVE ( ( 0.9330127018922194093, 0.9330127018922194093, 1.000000000000000000, 0.8660254037844387076, 1.000000000000000000, 0.8660254037844387076, 1.000000000000000000, 0.9330127018922194093, 0.9330127018922194093 ) ) 
 REPRESENTATION_ITEM ( '' )  );
#37540=CARTESIAN_POINT ( 'NONE',  ( -2.500000000000000444, -22.04166666393548013, -4.330127018922193649 ) ) ;
#37541=CARTESIAN_POINT ( 'NONE',  ( 2.229367062499998831, -9.645833331967738289, -3.861377020970580887 ) ) ;
#37543=ORIENTED_EDGE ( 'NONE', *, *, #54329, .F. ) ;
#37544=CARTESIAN_POINT ( 'NONE',  ( -4.458734124999999437, -33.64583333196772941, -2.574251347313719407 ) ) ;
#37549=CARTESIAN_POINT ( 'NONE',  ( -3.152548672688508926E-16, 13.43750000136559386, -5.148502694627439702 ) ) ;
#37553=CARTESIAN_POINT ( 'NONE',  ( 4.458734124999998549, -80.97916666530106511, -2.574251347313721627 ) ) ;
#37555=CARTESIAN_POINT ( 'NONE',  ( 6.123233995736766282E-16, -170.0000000000000000, -5.000000000000000000 ) ) ;
#37556=CARTESIAN_POINT ( 'NONE',  ( 2.499999999999998668, 19.79166666939785202, -4.330127018922193649 ) ) ;
#37557=VERTEX_POINT ( 'NONE', #33171 ) ;
#37558=CARTESIAN_POINT ( 'NONE',  ( -1.339745962155613812, -66.20534180126148271, -5.000000000000000000 ) ) ;
#37561=CARTESIAN_POINT ( 'NONE',  ( -3.535250795749689387E-16, -27.24999999999999645, -5.773502691896257311 ) ) ;
#37562=CARTESIAN_POINT ( 'NONE',  ( -2.229367062499996610, -34.14583333196772941, 3.861377020970582219 ) ) ;
#37564=AXIS2_PLACEMENT_3D ( 'NONE', #39479, #53332, #33091 ) ;
#37565=CARTESIAN_POINT ( 'NONE',  ( 2.499999999999998668, -29.20833333060214798, -4.330127018922193649 ) ) ;
#37566=CARTESIAN_POINT ( 'NONE',  ( 2.229367062499998831, -61.64583333196774362, -3.861377020970580887 ) ) ;
#37567=ORIENTED_EDGE ( 'NONE', *, *, #8025, .F. ) ;
#37568=CARTESIAN_POINT ( 'NONE',  ( 1.975475456537005874E-15, -62.62499999726880873, 5.000000000000000000 ) ) ;
#37569=CARTESIAN_POINT ( 'NONE',  ( -2.229367062499996610, -11.39583333196773829, 3.861377020970582219 ) ) ;
#37570=VERTEX_POINT ( 'NONE', #48574 ) ;
#37571=CARTESIAN_POINT ( 'NONE',  ( -5.000000000000000000, -77.00000000000000000, 0.000000000000000000 ) ) ;
#37574=CARTESIAN_POINT ( 'NONE',  ( 5.000000000000000000, -78.29166666393547303, -2.886751345948129988 ) ) ;
#37575=CARTESIAN_POINT ( 'NONE',  ( 1.339745962155612702, -65.16965819600733312, -5.000000000000000000 ) ) ;
#37576=ORIENTED_EDGE ( 'NONE', *, *, #13377, .F. ) ;
#37578=CARTESIAN_POINT ( 'NONE',  ( 2.229367062500001939, -21.22916666530107221, 3.861377020970579999 ) ) ;
#37579=CARTESIAN_POINT ( 'NONE',  ( 4.458734125000001214, -56.14583333196774362, 2.574251347313718519 ) ) ;
#37580=ORIENTED_EDGE ( 'NONE', *, *, #53528, .F. ) ;
#37581=CARTESIAN_POINT ( 'NONE',  ( 1.846868145590735200, -141.2500000013656063, -4.458734125000000326 ) ) ;
#37587=CARTESIAN_POINT ( 'NONE',  ( 1.975475456537005874E-15, 18.24999999999999645, 5.000000000000000000 ) ) ;
#37590=CARTESIAN_POINT ( 'NONE',  ( 3.152801135295366208, -148.8125000013655779, 3.152801135295367985 ) ) ;
#37594=CARTESIAN_POINT ( 'NONE',  ( 4.458734124999999437, -64.06249999863440792, -5.460374474430324690E-16 ) ) ;
#37597=CARTESIAN_POINT ( 'NONE',  ( 2.730187237215162345E-16, -142.1875000013656063, -4.458734124999999437 ) ) ;
#37599=( BOUNDED_CURVE ( )  B_SPLINE_CURVE ( 2, ( #207, #25596, #19805, #35247, #39102, #10797, #30409, #50033, #5991 ),
 .UNSPECIFIED., .F., .F. ) 
 B_SPLINE_CURVE_WITH_KNOTS ( ( 3, 2, 2, 2, 3 ),
 ( 0.6437500000000000444, 0.6444444444444444864, 0.6458333333333333703, 0.6472222222222222543, 0.6479166666666666963 ),
 .UNSPECIFIED. ) 
 CURVE ( )  GEOMETRIC_REPRESENTATION_ITEM ( )  RATIONAL_B_SPLINE_CURVE ( ( 0.9330127018922194093, 0.9330127018922194093, 1.000000000000000000, 0.8660254037844387076, 1.000000000000000000, 0.8660254037844387076, 1.000000000000000000, 0.9330127018922194093, 0.9330127018922194093 ) ) 
 REPRESENTATION_ITEM ( '' )  );
#37605=CARTESIAN_POINT ( 'NONE',  ( 2.500000000000002220, -14.54166666393548191, 4.330127018922192761 ) ) ;
#37609=CARTESIAN_POINT ( 'NONE',  ( -2.229367062499996610, 26.60416666803225993, 3.861377020970582219 ) ) ;
#37610=CARTESIAN_POINT ( 'NONE',  ( -2.499999999999996447, -17.70833333060214443, 4.330127018922195425 ) ) ;
#37615=CARTESIAN_POINT ( 'NONE',  ( 2.229367062500001939, 7.020833334698928674, 3.861377020970579999 ) ) ;
#37617=CARTESIAN_POINT ( 'NONE',  ( -4.458734124999999437, -21.64583333196774007, -2.574251347313719407 ) ) ;
#37619=CARTESIAN_POINT ( 'NONE',  ( 4.458734124999999437, -158.5000000013656631, 1.846868145590737864 ) ) ;
#37620=LINE ( 'NONE', #61768, #9946 ) ;
#37623=CARTESIAN_POINT ( 'NONE',  ( 5.000000000000000888, 15.41666666666666607, 2.886751345948126879 ) ) ;
#37624=CARTESIAN_POINT ( 'NONE',  ( -4.458734124999999437, -40.31249999863440081, 0.000000000000000000 ) ) ;
#37625=CARTESIAN_POINT ( 'NONE',  ( -1.339745962155613812, -84.20534180126149693, -5.000000000000000000 ) ) ;
#37627=CARTESIAN_POINT ( 'NONE',  ( 4.458734124999999437, -67.06249999863440792, -5.460374474430324690E-16 ) ) ;
#37629=CARTESIAN_POINT ( 'NONE',  ( 1.339745962155615144, -57.58034179853029144, 4.999999999999999112 ) ) ;
#37632=CARTESIAN_POINT ( 'NONE',  ( -5.000000000000000000, -85.08333333333332860, -2.886751345948128211 ) ) ;
#37634=CARTESIAN_POINT ( 'NONE',  ( 5.000000000000000000, -144.1250000027312126, 0.000000000000000000 ) ) ;
#37635=CARTESIAN_POINT ( 'NONE',  ( 2.499999999999998668, -13.33333333333333570, -4.330127018922193649 ) ) ;
#37636=CARTESIAN_POINT ( 'NONE',  ( 4.458734124999999437, -15.81249999863440436, -5.460374474430324690E-16 ) ) ;
#37637=CARTESIAN_POINT ( 'NONE',  ( -2.229367062500000163, -79.47916666530106511, -3.861377020970580443 ) ) ;
#37639=CARTESIAN_POINT ( 'NONE',  ( 5.000000000000000888, -11.45833333060214798, 2.886751345948126879 ) ) ;
#37640=CARTESIAN_POINT ( 'NONE',  ( 2.229367062499998831, -44.64583333196774362, -3.861377020970580887 ) ) ;
#37642=CARTESIAN_POINT ( 'NONE',  ( -2.500000000000000444, 29.83333333333333215, -4.330127018922193649 ) ) ;
#37643=CARTESIAN_POINT ( 'NONE',  ( -4.458734124999998549, 9.520833334698927786, 2.574251347313722516 ) ) ;
#37645=CYLINDRICAL_SURFACE ( 'NONE', #16575, 5.000000000000000000 ) ;
#37646=CARTESIAN_POINT ( 'NONE',  ( 5.000000000000000000, -62.41666666666666430, -2.886751345948129988 ) ) ;
#37647=CARTESIAN_POINT ( 'NONE',  ( -3.152801135295367985, -162.0625000013656063, 3.152801135295367096 ) ) ;
#37650=CARTESIAN_POINT ( 'NONE',  ( -4.458734124999999437, -81.39583333196773651, -2.574251347313719407 ) ) ;
#37651=CARTESIAN_POINT ( 'NONE',  ( 5.000000000000000000, -165.0625000000000000, 2.071067811865478614 ) ) ;
#37655=CARTESIAN_POINT ( 'NONE',  ( 9.457646018065525792E-16, -7.312499998634405252, 5.148502694627439702 ) ) ;
#37657=CARTESIAN_POINT ( 'NONE',  ( 4.458734124999999437, -43.06249999863440081, -5.460374474430324690E-16 ) ) ;
#37660=CARTESIAN_POINT ( 'NONE',  ( 0.000000000000000000, -170.0000000000000000, 0.000000000000000000 ) ) ;
#37661=ORIENTED_EDGE ( 'NONE', *, *, #50764, .F. ) ;
#37663=CARTESIAN_POINT ( 'NONE',  ( -3.152548672688508926E-16, -68.81249999863439371, -5.148502694627439702 ) ) ;
#37664=CARTESIAN_POINT ( 'NONE',  ( -8.190561711645485556E-16, -145.9375000013656063, 4.458734124999999437 ) ) ;
#37665=VERTEX_POINT ( 'NONE', #8717 ) ;
#37666=CARTESIAN_POINT ( 'NONE',  ( -9.184850993605147944E-16, -164.2500000000000000, 5.000000000000000000 ) ) ;
#37667=CARTESIAN_POINT ( 'NONE',  ( 1.339745962155565406, -3.580341798530294550, 5.000000000000028422 ) ) ;
#37670=CARTESIAN_POINT ( 'NONE',  ( 4.458734124999999437, 2.187500001365593416, -5.460374474430324690E-16 ) ) ;
#37672=CARTESIAN_POINT ( 'NONE',  ( 4.458734124999999437, -156.4375000013655779, 0.000000000000000000 ) ) ;
#37674=ORIENTED_EDGE ( 'NONE', *, *, #42116, .F. ) ;
#37679=EDGE_CURVE ( 'NONE', #13190, #43260, #14041, .T. ) ;
#37681=CARTESIAN_POINT ( 'NONE',  ( 1.339745962155612702, -23.16965819600733312, -5.000000000000000000 ) ) ;
#37682=CARTESIAN_POINT ( 'NONE',  ( 2.499999999999998668, -67.33333333333332860, -4.330127018922193649 ) ) ;
#37687=CARTESIAN_POINT ( 'NONE',  ( -2.229367062499996610, 24.85416666803225993, 3.861377020970582219 ) ) ;
#37689=CARTESIAN_POINT ( 'NONE',  ( 2.229367062500001939, -4.229166665301070438, 3.861377020970579999 ) ) ;
#37690=CARTESIAN_POINT ( 'NONE',  ( -2.500000000000000444, -34.04166666393547303, -4.330127018922193649 ) ) ;
#37692=CARTESIAN_POINT ( 'NONE',  ( 5.000000000000000888, -143.0625000027312126, -2.071067811865475505 ) ) ;
#37696=VECTOR ( 'NONE', #28457, 1000.000000000000000 ) ;
#37698=CARTESIAN_POINT ( 'NONE',  ( 6.123233995736766282E-16, -170.0000000000000000, -5.000000000000000000 ) ) ;
#37700=LINE ( 'NONE', #4242, #62416 ) ;
#37701=VECTOR ( 'NONE', #19886, 1000.000000000000000 ) ;
#37704=CARTESIAN_POINT ( 'NONE',  ( -4.458734125000000326, -156.1250000013655779, 1.846868145590734089 ) ) ;
#37706=DIRECTION ( 'NONE',  ( 0.000000000000000000, 0.000000000000000000, 1.000000000000000000 ) ) ;
#37708=CARTESIAN_POINT ( 'NONE',  ( -2.229367062500000163, 17.27083333469892779, -3.861377020970580443 ) ) ;
#37709=ORIENTED_EDGE ( 'NONE', *, *, #40979, .F. ) ;
#37714=CARTESIAN_POINT ( 'NONE',  ( -5.000000000000000000, 1.999999999999998224, 0.000000000000000000 ) ) ;
#37715=( BOUNDED_CURVE ( )  B_SPLINE_CURVE ( 2, ( #11889, #25744, #49854, #26377, #11258, #35714, #1960, #10936, #46317 ),
 .UNSPECIFIED., .F., .F. ) 
 B_SPLINE_CURVE_WITH_KNOTS ( ( 3, 2, 2, 2, 3 ),
 ( 0.2270833333333333315, 0.2277777777777777735, 0.2291666666666666574, 0.2305555555555555691, 0.2312500000000000111 ),
 .UNSPECIFIED. ) 
 CURVE ( )  GEOMETRIC_REPRESENTATION_ITEM ( )  RATIONAL_B_SPLINE_CURVE ( ( 0.9330127018922194093, 0.9330127018922194093, 1.000000000000000000, 0.8660254037844387076, 1.000000000000000000, 0.8660254037844387076, 1.000000000000000000, 0.9330127018922194093, 0.9330127018922194093 ) ) 
 REPRESENTATION_ITEM ( '' )  );
#37716=EDGE_CURVE ( 'NONE', #52361, #8855, #9534, .T. ) ;
#37717=CARTESIAN_POINT ( 'NONE',  ( -2.229367062499996610, -61.14583333196774362, 3.861377020970582219 ) ) ;
#37718=CARTESIAN_POINT ( 'NONE',  ( -5.000000000000000000, -52.95833333060214443, -2.886751345948128211 ) ) ;
#37720=CARTESIAN_POINT ( 'NONE',  ( 4.458734124999999437, -27.81249999863440081, -5.460374474430324690E-16 ) ) ;
#37723=FACE_OUTER_BOUND ( 'NONE', #4318, .T. ) ;
#37724=CARTESIAN_POINT ( 'NONE',  ( -2.499999999999996447, -39.83333333333332860, 4.330127018922195425 ) ) ;
#37726=CARTESIAN_POINT ( 'NONE',  ( 1.062108568985190270E-13, -26.12499999726881583, -4.999999999999999112 ) ) ;
#37729=CARTESIAN_POINT ( 'NONE',  ( 4.458734125000001214, -64.89583333196773651, 2.574251347313718519 ) ) ;
#37730=CARTESIAN_POINT ( 'NONE',  ( -3.152801135295367985, -148.0625000013655779, 3.152801135295367096 ) ) ;
#37731=CARTESIAN_POINT ( 'NONE',  ( -4.458734124999999437, -75.39583333196773651, -2.574251347313719407 ) ) ;
#37733=CARTESIAN_POINT ( 'NONE',  ( -4.458734124999999437, -26.64583333196773651, -2.574251347313719407 ) ) ;
#37734=( BOUNDED_CURVE ( )  B_SPLINE_CURVE ( 2, ( #49373, #5318, #24936, #35224, #499, #59349, #34905, #15282, #5959 ),
 .UNSPECIFIED., .F., .F. ) 
 B_SPLINE_CURVE_WITH_KNOTS ( ( 3, 2, 2, 2, 3 ),
 ( 0.5270833333333333481, 0.5277777777777777901, 0.5291666666666666741, 0.5305555555555555580, 0.5312500000000000000 ),
 .UNSPECIFIED. ) 
 CURVE ( )  GEOMETRIC_REPRESENTATION_ITEM ( )  RATIONAL_B_SPLINE_CURVE ( ( 0.9330127018922194093, 0.9330127018922194093, 1.000000000000000000, 0.8660254037844387076, 1.000000000000000000, 0.8660254037844387076, 1.000000000000000000, 0.9330127018922194093, 0.9330127018922194093 ) ) 
 REPRESENTATION_ITEM ( '' )  );
#37735=CARTESIAN_POINT ( 'NONE',  ( 5.000000000000000888, -68.45833333060214443, 2.886751345948126879 ) ) ;
#37737=EDGE_CURVE ( 'NONE', #7641, #45160, #39955, .T. ) ;
#37738=CARTESIAN_POINT ( 'NONE',  ( 5.000000000000000000, -1.500000000000001332, -6.123233995736766282E-16 ) ) ;
#37744=VECTOR ( 'NONE', #24703, 1000.000000000000000 ) ;
#37746=DIRECTION ( 'NONE',  ( -0.000000000000000000, 1.000000000000000000, -0.000000000000000000 ) ) ;
#37747=CARTESIAN_POINT ( 'NONE',  ( 4.458734125000001214, -54.14583333196773651, 2.574251347313718519 ) ) ;
#37753=CARTESIAN_POINT ( 'NONE',  ( 9.457646018065525792E-16, 17.93750000136559208, 5.148502694627439702 ) ) ;
#37755=CARTESIAN_POINT ( 'NONE',  ( -5.000000000000000000, -2.000000000000001776, 0.000000000000000000 ) ) ;
#37756=CARTESIAN_POINT ( 'NONE',  ( 3.152801135295366208, -168.5625000013656063, 3.152801135295367985 ) ) ;
#37759=CARTESIAN_POINT ( 'NONE',  ( -6.972266317189433020E-16, -40.24999999999999289, -5.000000000000000000 ) ) ;
#37761=EDGE_CURVE ( 'NONE', #54515, #42874, #54368, .T. ) ;
#37763=CARTESIAN_POINT ( 'NONE',  ( 2.071067811865392461, -140.3125000027312694, 5.000000000000084377 ) ) ;
#37764=EDGE_CURVE ( 'NONE', #59122, #41205, #11233, .T. ) ;
#37774=CARTESIAN_POINT ( 'NONE',  ( 0.000000000000000000, -170.0000000000000000, 5.000000000000000000 ) ) ;
#37776=CARTESIAN_POINT ( 'NONE',  ( 5.000000000000000000, -153.1250000027312126, 0.000000000000000000 ) ) ;
#37777=ORIENTED_EDGE ( 'NONE', *, *, #1935, .T. ) ;
#37783=CARTESIAN_POINT ( 'NONE',  ( -3.535533905932738641, -146.3750000000000000, 3.535533905932737309 ) ) ;
#37787=CARTESIAN_POINT ( 'NONE',  ( -3.152801135295367985, -168.0625000013656063, 3.152801135295367096 ) ) ;
#37788=CARTESIAN_POINT ( 'NONE',  ( 4.458734125000000326, -29.89583333196773651, 2.574251347313718519 ) ) ;
#37792=CARTESIAN_POINT ( 'NONE',  ( 3.152801135295367541, -146.3125000013655779, -3.152801135295367541 ) ) ;
#37793=EDGE_LOOP ( 'NONE', ( #13292, #24811, #14872, #56149 ) ) ;
#37795=CARTESIAN_POINT ( 'NONE',  ( -4.458734124999999437, -56.56249999863440081, 0.000000000000000000 ) ) ;
#37800=CARTESIAN_POINT ( 'NONE',  ( 2.500000000000002220, 24.33333333333333215, 4.330127018922192761 ) ) ;
#37801=VECTOR ( 'NONE', #28670, 1000.000000000000000 ) ;
#37802=DIRECTION ( 'NONE',  ( -0.000000000000000000, 1.000000000000000000, -0.000000000000000000 ) ) ;
#37803=CARTESIAN_POINT ( 'NONE',  ( -3.152548672688508926E-16, -0.5624999986344053626, -5.148502694627439702 ) ) ;
#37805=CARTESIAN_POINT ( 'NONE',  ( -2.071067811865415109, -164.3125000000000000, 5.000000000000062172 ) ) ;
#37806=CARTESIAN_POINT ( 'NONE',  ( -2.229367062499996610, 9.604166668032261711, 3.861377020970582219 ) ) ;
#37809=ORIENTED_EDGE ( 'NONE', *, *, #13455, .T. ) ;
#37811=CARTESIAN_POINT ( 'NONE',  ( 4.458734125000001214, -48.89583333196772941, 2.574251347313718519 ) ) ;
#37812=CARTESIAN_POINT ( 'NONE',  ( 4.458734125000000326, -158.6250000013655779, -1.846868145590734978 ) ) ;
#37813=CARTESIAN_POINT ( 'NONE',  ( 2.500000000000002220, -51.54166666393547303, 4.330127018922192761 ) ) ;
#37815=CARTESIAN_POINT ( 'NONE',  ( 2.229367062499998831, -24.64583333196773651, -3.861377020970580887 ) ) ;
#37818=CARTESIAN_POINT ( 'NONE',  ( -1.846868145590737420, -161.7500000013655495, 4.458734124999999437 ) ) ;
#37819=DIRECTION ( 'NONE',  ( -0.000000000000000000, 1.000000000000000000, -0.000000000000000000 ) ) ;
#37821=CARTESIAN_POINT ( 'NONE',  ( -3.152548672688508926E-16, -38.81249999863440081, -5.148502694627439702 ) ) ;
#37822=EDGE_LOOP ( 'NONE', ( #25782, #30270, #30907, #36171 ) ) ;
#37827=CARTESIAN_POINT ( 'NONE',  ( -5.000000000000000000, -59.87499999726880873, 0.000000000000000000 ) ) ;
#37829=CARTESIAN_POINT ( 'NONE',  ( 4.458734124999999437, -85.06249999863439371, -5.460374474430324690E-16 ) ) ;
#37835=CARTESIAN_POINT ( 'NONE',  ( -2.500000000000000444, -45.04166666393547303, -4.330127018922193649 ) ) ;
#37842=EDGE_CURVE ( 'NONE', #59664, #37124, #40345, .T. ) ;
#37845=CARTESIAN_POINT ( 'NONE',  ( 0.000000000000000000, -170.0000000000000000, 0.000000000000000000 ) ) ;
#37847=CARTESIAN_POINT ( 'NONE',  ( 2.229367062500001939, -86.22916666530107932, 3.861377020970579999 ) ) ;
#37850=ORIENTED_EDGE ( 'NONE', *, *, #15258, .T. ) ;
#37851=EDGE_CURVE ( 'NONE', #31664, #54505, #17811, .T. ) ;
#37852=CARTESIAN_POINT ( 'NONE',  ( -2.071067811865622943, -155.8125000027310989, -4.999999999999850786 ) ) ;
#37854=CARTESIAN_POINT ( 'NONE',  ( 2.071067811865475505, -166.9375000027312126, -5.000000000000000888 ) ) ;
#37861=CARTESIAN_POINT ( 'NONE',  ( 5.000000000000000000, -86.29166666393547303, -2.886751345948130876 ) ) ;
#37862=DIRECTION ( 'NONE',  ( -0.000000000000000000, 1.000000000000000000, -0.000000000000000000 ) ) ;
#37863=CARTESIAN_POINT ( 'NONE',  ( -2.229367062499996610, -11.14583333196773829, 3.861377020970582219 ) ) ;
#37865=ADVANCED_FACE ( 'NONE', ( #60477 ), #27003, .T. ) ;
#37867=CARTESIAN_POINT ( 'NONE',  ( -4.458734124999999437, -38.56249999863440081, 0.000000000000000000 ) ) ;
#37870=CARTESIAN_POINT ( 'NONE',  ( -6.972266317189433020E-16, 0.8750000027311866102, -5.000000000000000000 ) ) ;
#37874=CARTESIAN_POINT ( 'NONE',  ( -3.152548672688508926E-16, 15.43750000136559564, -5.148502694627439702 ) ) ;
#37878=CARTESIAN_POINT ( 'NONE',  ( 2.229367062499998831, -82.89583333196773651, -3.861377020970580887 ) ) ;
#37880=CARTESIAN_POINT ( 'NONE',  ( 5.000000000000000000, 15.62500000273118417, -6.123233995736766282E-16 ) ) ;
#37882=CARTESIAN_POINT ( 'NONE',  ( 1.339745962155615144, -35.70534180126148271, 4.999999999999999112 ) ) ;
#37883=CARTESIAN_POINT ( 'NONE',  ( -2.500000000000000444, 15.83333333333333037, -4.330127018922193649 ) ) ;
#37885=CARTESIAN_POINT ( 'NONE',  ( 2.499999999999998668, -27.33333333333333570, -4.330127018922193649 ) ) ;
#37886=CARTESIAN_POINT ( 'NONE',  ( 4.458734124999999437, -31.81249999863440436, -5.460374474430324690E-16 ) ) ;
#37887=AXIS2_PLACEMENT_3D ( 'NONE', #28780, #34538, #10113 ) ;
#37889=CARTESIAN_POINT ( 'NONE',  ( -5.000000000000000000, -28.87499999726881228, 0.000000000000000000 ) ) ;
#37890=CARTESIAN_POINT ( 'NONE',  ( -4.458734124999999437, -59.31249999863440081, 0.000000000000000000 ) ) ;
#37893=CARTESIAN_POINT ( 'NONE',  ( 9.457646018065525792E-16, -8.312499998634406140, 5.148502694627439702 ) ) ;
#37894=ORIENTED_EDGE ( 'NONE', *, *, #42064, .T. ) ;
#37895=CARTESIAN_POINT ( 'NONE',  ( -5.000000000000000000, -76.08333333333332860, -2.886751345948128211 ) ) ;
#37898=CARTESIAN_POINT ( 'NONE',  ( -2.499999999999996447, -78.70833333060214443, 4.330127018922195425 ) ) ;
#37902=CARTESIAN_POINT ( 'NONE',  ( -4.458734124999999437, -21.56249999863440436, 0.000000000000000000 ) ) ;
#37903=CARTESIAN_POINT ( 'NONE',  ( -4.458734124999999437, -54.56249999863440081, 0.000000000000000000 ) ) ;
#37906=CARTESIAN_POINT ( 'NONE',  ( 4.458734124999999437, -142.5000000013656347, 1.846868145590737864 ) ) ;
#37913=( BOUNDED_CURVE ( )  B_SPLINE_CURVE ( 2, ( #46218, #11483, #51686, #7627, #41379, #36563, #32050, #12115, #16318 ),
 .UNSPECIFIED., .F., .F. ) 
 B_SPLINE_CURVE_WITH_KNOTS ( ( 3, 2, 2, 2, 3 ),
 ( 0.07708333333333333703, 0.07777777777777777901, 0.07916666666666666297, 0.08055555555555556080, 0.08125000000000000278 ),
 .UNSPECIFIED. ) 
 CURVE ( )  GEOMETRIC_REPRESENTATION_ITEM ( )  RATIONAL_B_SPLINE_CURVE ( ( 0.9330127018922194093, 0.9330127018922194093, 1.000000000000000000, 0.8660254037844387076, 1.000000000000000000, 0.8660254037844387076, 1.000000000000000000, 0.9330127018922194093, 0.9330127018922194093 ) ) 
 REPRESENTATION_ITEM ( '' )  );
#37915=CARTESIAN_POINT ( 'NONE',  ( 1.846868145590735200, -144.5000000013656063, -4.458734125000000326 ) ) ;
#37917=DIRECTION ( 'NONE',  ( -0.000000000000000000, 1.000000000000000000, -0.000000000000000000 ) ) ;
#37919=CARTESIAN_POINT ( 'NONE',  ( 4.458734124999998549, -66.97916666530107932, -2.574251347313721627 ) ) ;
#37922=CARTESIAN_POINT ( 'NONE',  ( -4.458734124999999437, -140.9375000013656063, -5.460374474430324690E-16 ) ) ;
#37926=CARTESIAN_POINT ( 'NONE',  ( -2.071067811865562991, -144.3124999999999716, 4.999999999999913847 ) ) ;
#37929=CARTESIAN_POINT ( 'NONE',  ( 1.975475456537005874E-15, -35.75000000000000711, 5.000000000000000000 ) ) ;
#37931=AXIS2_PLACEMENT_3D ( 'NONE', #32516, #8089, #27693 ) ;
#37932=CARTESIAN_POINT ( 'NONE',  ( -2.229367062499996610, 22.60416666803225993, 3.861377020970582219 ) ) ;
#37938=DIRECTION ( 'NONE',  ( -0.000000000000000000, 1.000000000000000000, -0.000000000000000000 ) ) ;
#37939=CARTESIAN_POINT ( 'NONE',  ( -2.229367062499996610, 4.854166668032261711, 3.861377020970582219 ) ) ;
#37941=CARTESIAN_POINT ( 'NONE',  ( -2.229367062500000163, -17.72916666530106866, -3.861377020970580443 ) ) ;
#37943=CARTESIAN_POINT ( 'NONE',  ( 1.846868145590736310, -160.6250000013655779, 4.458734124999999437 ) ) ;
#37944=CARTESIAN_POINT ( 'NONE',  ( 5.000000000000000000, 15.70833333606451809, -2.886751345948130876 ) ) ;
#37947=CARTESIAN_POINT ( 'NONE',  ( 4.458734124999999437, 29.18750000136559208, -5.460374474430324690E-16 ) ) ;
#37948=CARTESIAN_POINT ( 'NONE',  ( 4.458734124999998549, -40.72916666530107221, -2.574251347313721627 ) ) ;
#37949=CARTESIAN_POINT ( 'NONE',  ( -5.000000000000000000, -83.99999999999998579, 0.000000000000000000 ) ) ;
#37951=CARTESIAN_POINT ( 'NONE',  ( 2.229367062499998831, -68.89583333196773651, -3.861377020970580887 ) ) ;
#37954=CARTESIAN_POINT ( 'NONE',  ( 2.071067811865264563, -151.9375000027311842, -5.000000000000211386 ) ) ;
#37957=CARTESIAN_POINT ( 'NONE',  ( 5.000000000000000000, -14.41666666666666963, -2.886751345948129988 ) ) ;
#37958=CARTESIAN_POINT ( 'NONE',  ( -4.458734124999999437, -17.31249999863440792, 0.000000000000000000 ) ) ;
#37959=CARTESIAN_POINT ( 'NONE',  ( 2.229367062499998831, -75.64583333196773651, -3.861377020970580887 ) ) ;
#37961=CARTESIAN_POINT ( 'NONE',  ( 5.000000000000000000, -12.37499999726881050, -6.123233995736766282E-16 ) ) ;
#37962=CARTESIAN_POINT ( 'NONE',  ( 4.458734125000001214, -42.89583333196773651, 2.574251347313718519 ) ) ;
#37963=VERTEX_POINT ( 'NONE', #26364 ) ;
#37964=CARTESIAN_POINT ( 'NONE',  ( 3.061616997868383141E-16, -143.7500000000000284, -5.000000000000000000 ) ) ;
#37965=CARTESIAN_POINT ( 'NONE',  ( 4.458734124999998549, 7.020833334698929562, -2.574251347313721627 ) ) ;
#37967=( BOUNDED_CURVE ( )  B_SPLINE_CURVE ( 2, ( #6955, #12081, #31704, #7277, #41653, #38118, #17860, #3085, #37482 ),
 .UNSPECIFIED., .F., .F. ) 
 B_SPLINE_CURVE_WITH_KNOTS ( ( 3, 2, 2, 2, 3 ),
 ( 0.08541666666666666852, 0.08611111111111111049, 0.08749999999999999445, 0.08888888888888889228, 0.08958333333333333426 ),
 .UNSPECIFIED. ) 
 CURVE ( )  GEOMETRIC_REPRESENTATION_ITEM ( )  RATIONAL_B_SPLINE_CURVE ( ( 0.9330127018922194093, 0.9330127018922194093, 1.000000000000000000, 0.8660254037844387076, 1.000000000000000000, 0.8660254037844387076, 1.000000000000000000, 0.9330127018922194093, 0.9330127018922194093 ) ) 
 REPRESENTATION_ITEM ( '' )  );
#37969=CARTESIAN_POINT ( 'NONE',  ( -2.500000000000000444, -61.16666666666666430, -4.330127018922193649 ) ) ;
#37970=CARTESIAN_POINT ( 'NONE',  ( 4.458734124999999437, -156.6875000013655779, 0.000000000000000000 ) ) ;
#37974=CARTESIAN_POINT ( 'NONE',  ( 3.535533905932738197, -166.8750000000000284, -3.535533905932738197 ) ) ;
#37975=CARTESIAN_POINT ( 'NONE',  ( 0.000000000000000000, -170.0000000000000000, 5.000000000000000000 ) ) ;
#37976=AXIS2_PLACEMENT_3D ( 'NONE', #29363, #13959, #5267 ) ;
#37978=CARTESIAN_POINT ( 'NONE',  ( -4.458734124999999437, -5.562499998634402587, 0.000000000000000000 ) ) ;
#37979=CARTESIAN_POINT ( 'NONE',  ( -3.152548672688508926E-16, -39.81249999863440081, -5.148502694627439702 ) ) ;
#37980=CARTESIAN_POINT ( 'NONE',  ( 5.000000000000000888, -67.45833333060214443, 2.886751345948126879 ) ) ;
#37981=CARTESIAN_POINT ( 'NONE',  ( 4.458734125000000326, -154.3750000013655779, -1.846868145590734978 ) ) ;
#37983=ORIENTED_EDGE ( 'NONE', *, *, #30741, .F. ) ;
#37985=CARTESIAN_POINT ( 'NONE',  ( 5.000000000000000888, -2.458333330602146205, 2.886751345948126879 ) ) ;
#37986=CARTESIAN_POINT ( 'NONE',  ( -4.458734124999998549, -69.47916666530107932, 2.574251347313722516 ) ) ;
#37987=CARTESIAN_POINT ( 'NONE',  ( 1.846868145590735200, -147.5000000013656063, -4.458734124999999437 ) ) ;
#37988=ORIENTED_EDGE ( 'NONE', *, *, #38985, .F. ) ;
#37992=CARTESIAN_POINT ( 'NONE',  ( 2.229367062500001939, 1.020833334698927120, 3.861377020970579999 ) ) ;
#37994=CARTESIAN_POINT ( 'NONE',  ( -1.846868145590737420, -151.7500000013656063, 4.458734124999997661 ) ) ;
#37998=FACE_OUTER_BOUND ( 'NONE', #17167, .T. ) ;
#38002=DIRECTION ( 'NONE',  ( -0.000000000000000000, 1.000000000000000000, -0.000000000000000000 ) ) ;
#38003=CARTESIAN_POINT ( 'NONE',  ( 5.000000000000000000, -87.50000000000000000, -6.123233995736766282E-16 ) ) ;
#38005=LINE ( 'NONE', #33803, #16445 ) ;
#38007=LINE ( 'NONE', #48905, #25297 ) ;
#38008=CARTESIAN_POINT ( 'NONE',  ( 2.229367062500001939, 23.02083333469892423, 3.861377020970579999 ) ) ;
#38010=CARTESIAN_POINT ( 'NONE',  ( -4.458734124999999437, -4.645833331967739177, -2.574251347313719407 ) ) ;
#38014=CARTESIAN_POINT ( 'NONE',  ( -5.000000000000000888, -139.5625000027311842, 2.071067811865474617 ) ) ;
#38015=CARTESIAN_POINT ( 'NONE',  ( 5.000000000000000000, -75.29166666393548724, -2.886751345948130876 ) ) ;
#38023=CARTESIAN_POINT ( 'NONE',  ( -4.458734125000000326, -159.1250000013656063, 1.846868145590734089 ) ) ;
#38026=VERTEX_POINT ( 'NONE', #52087 ) ;
#38027=CARTESIAN_POINT ( 'NONE',  ( 2.229367062499998831, 19.10416666803225993, -3.861377020970580887 ) ) ;
#38028=ORIENTED_EDGE ( 'NONE', *, *, #35453, .T. ) ;
#38032=CARTESIAN_POINT ( 'NONE',  ( 6.123233995736766282E-16, -170.0000000000000000, -5.000000000000000000 ) ) ;
#38033=CARTESIAN_POINT ( 'NONE',  ( 5.000000000000000000, 5.500000000000001776, -6.123233995736766282E-16 ) ) ;
#38034=CARTESIAN_POINT ( 'NONE',  ( -3.152548672688508926E-16, -61.56249999863440081, -5.148502694627439702 ) ) ;
#38035=CARTESIAN_POINT ( 'NONE',  ( -1.339745962155610925, -52.66965819600733312, 5.000000000000000000 ) ) ;
#38036=CARTESIAN_POINT ( 'NONE',  ( 5.000000000000000888, 5.541666669397854683, 2.886751345948126879 ) ) ;
#38037=CARTESIAN_POINT ( 'NONE',  ( 4.458734125000001214, -29.89583333196773651, 2.574251347313718519 ) ) ;
#38040=CARTESIAN_POINT ( 'NONE',  ( 1.975475456537005874E-15, -24.62499999726881583, 5.000000000000000000 ) ) ;
#38041=CARTESIAN_POINT ( 'NONE',  ( 2.499999999999998668, -43.33333333333333570, -4.330127018922193649 ) ) ;
#38044=CARTESIAN_POINT ( 'NONE',  ( 1.339745962155615144, -4.580341798530294994, 4.999999999999999112 ) ) ;
#38045=CARTESIAN_POINT ( 'NONE',  ( -3.152548672688508926E-16, -65.56249999863440792, -5.148502694627439702 ) ) ;
#38046=CARTESIAN_POINT ( 'NONE',  ( -1.846868145590737420, -150.0000000013655779, 4.458734124999999437 ) ) ;
#38047=CARTESIAN_POINT ( 'NONE',  ( 4.458734125000001214, -75.89583333196775072, 2.574251347313718519 ) ) ;
#38048=EDGE_CURVE ( 'NONE', #12482, #52029, #53491, .T. ) ;
#38050=CARTESIAN_POINT ( 'NONE',  ( 9.457646018065525792E-16, -24.31249999863440792, 5.148502694627439702 ) ) ;
#38051=CARTESIAN_POINT ( 'NONE',  ( -3.535250795749689387E-16, -65.12499999726881583, -5.773502691896257311 ) ) ;
#38052=ORIENTED_EDGE ( 'NONE', *, *, #38998, .F. ) ;
#38053=CARTESIAN_POINT ( 'NONE',  ( -3.535533905932738641, -152.5000000027312126, 3.535533905932737309 ) ) ;
#38054=ORIENTED_EDGE ( 'NONE', *, *, #19301, .T. ) ;
#38059=AXIS2_PLACEMENT_3D ( 'NONE', #19558, #48196, #58488 ) ;
#38062=CARTESIAN_POINT ( 'NONE',  ( -2.229367062500000163, -52.72916666530107221, -3.861377020970580443 ) ) ;
#38064=VERTEX_POINT ( 'NONE', #56605 ) ;
#38065=ADVANCED_FACE ( 'NONE', ( #31496 ), #47260, .F. ) ;
#38069=CARTESIAN_POINT ( 'NONE',  ( 4.458734125000001214, 21.10416666803226349, 2.574251347313718519 ) ) ;
#38072=CARTESIAN_POINT ( 'NONE',  ( 3.152801135295367541, -165.3125000013656063, -3.152801135295367541 ) ) ;
#38076=CARTESIAN_POINT ( 'NONE',  ( 0.000000000000000000, -170.0000000000000000, 0.000000000000000000 ) ) ;
#38079=CARTESIAN_POINT ( 'NONE',  ( 1.339745962155612702, -69.16965819600731891, -5.000000000000000000 ) ) ;
#38082=CARTESIAN_POINT ( 'NONE',  ( 1.339745962155612702, -20.29465819873851729, -5.000000000000000000 ) ) ;
#38086=CARTESIAN_POINT ( 'NONE',  ( -5.000000000000000000, -159.5000000000000000, -6.123233995736766282E-16 ) ) ;
#38089=DIRECTION ( 'NONE',  ( -0.000000000000000000, 1.000000000000000000, -0.000000000000000000 ) ) ;
#38091=CARTESIAN_POINT ( 'NONE',  ( 3.535533905932738197, -152.0000000027312126, -3.535533905932738197 ) ) ;
#38096=( BOUNDED_CURVE ( )  B_SPLINE_CURVE ( 2, ( #61252, #3032, #56432, #28942, #31967, #9329, #46763, #4507, #18979 ),
 .UNSPECIFIED., .F., .F. ) 
 B_SPLINE_CURVE_WITH_KNOTS ( ( 3, 2, 2, 2, 3 ),
 ( 0.4583333333333337589, 0.4625000000000004663, 0.4666666666666671182, 0.4708333333333337700, 0.4750000000000004219 ),
 .UNSPECIFIED. ) 
 CURVE ( )  GEOMETRIC_REPRESENTATION_ITEM ( )  RATIONAL_B_SPLINE_CURVE ( ( 0.9999999999999918954, 0.9238795325112948431, 1.000000000000000000, 0.9238795325112867385, 1.000000000000000000, 0.9238795325112867385, 1.000000000000000000, 0.9238795325112786339, 1.000000000000008216 ) ) 
 REPRESENTATION_ITEM ( '' )  );
#38098=CARTESIAN_POINT ( 'NONE',  ( -9.184850993605147944E-16, -143.2500000000000284, 5.000000000000000000 ) ) ;
#38099=EDGE_CURVE ( 'NONE', #34811, #30019, #60095, .T. ) ;
#38102=CARTESIAN_POINT ( 'NONE',  ( -5.000000000000000000, -55.08333333333332860, -2.886751345948128211 ) ) ;
#38103=CARTESIAN_POINT ( 'NONE',  ( -4.458734124999997661, -30.22916666530106866, 2.574251347313722516 ) ) ;
#38104=CARTESIAN_POINT ( 'NONE',  ( 0.000000000000000000, -170.0000000000000000, 0.000000000000000000 ) ) ;
#38105=CARTESIAN_POINT ( 'NONE',  ( 5.000000000000000000, 18.70833333606451632, -2.886751345948130876 ) ) ;
#38107=CARTESIAN_POINT ( 'NONE',  ( 1.846868145590735200, -147.2500000013656063, -4.458734125000000326 ) ) ;
#38108=ORIENTED_EDGE ( 'NONE', *, *, #60430, .F. ) ;
#38109=VECTOR ( 'NONE', #10392, 1000.000000000000000 ) ;
#38110=CARTESIAN_POINT ( 'NONE',  ( 6.123233995736766282E-16, -170.0000000000000000, -5.000000000000000000 ) ) ;
#38111=CARTESIAN_POINT ( 'NONE',  ( 4.458734125000000326, -59.14583333196772230, 2.574251347313718519 ) ) ;
#38114=CARTESIAN_POINT ( 'NONE',  ( 5.000000000000000000, 20.49999999999999645, -6.123233995736766282E-16 ) ) ;
#38115=FACE_OUTER_BOUND ( 'NONE', #21721, .T. ) ;
#38116=CARTESIAN_POINT ( 'NONE',  ( -2.229367062499996610, -2.145833331967737845, 3.861377020970582219 ) ) ;
#38118=CARTESIAN_POINT ( 'NONE',  ( 5.000000000000000888, 19.41666666666666785, 2.886751345948126879 ) ) ;
#38120=CARTESIAN_POINT ( 'NONE',  ( -3.152548672688508926E-16, 12.18750000136559564, -5.148502694627439702 ) ) ;
#38124=CARTESIAN_POINT ( 'NONE',  ( -4.458734124999999437, -51.31249999863440792, 0.000000000000000000 ) ) ;
#38125=CARTESIAN_POINT ( 'NONE',  ( -3.152801135295367985, -158.0625000013656063, 3.152801135295367096 ) ) ;
#38127=CARTESIAN_POINT ( 'NONE',  ( -2.500000000000000444, -52.04166666393547303, -4.330127018922193649 ) ) ;
#38129=CARTESIAN_POINT ( 'NONE',  ( 2.229367062500001939, -22.97916666530107221, 3.861377020970579999 ) ) ;
#38132=CARTESIAN_POINT ( 'NONE',  ( -9.184850993605147944E-16, -142.3750000027312126, 5.000000000000000000 ) ) ;
#38133=CARTESIAN_POINT ( 'NONE',  ( 4.458734125000000326, -160.3750000013656063, -1.846868145590734978 ) ) ;
#38134=ORIENTED_EDGE ( 'NONE', *, *, #48929, .T. ) ;
#38137=CARTESIAN_POINT ( 'NONE',  ( -3.152548672688508926E-16, -36.81249999863440792, -5.148502694627439702 ) ) ;
#38142=CARTESIAN_POINT ( 'NONE',  ( 0.000000000000000000, -170.0000000000000000, 5.000000000000000000 ) ) ;
#38145=CARTESIAN_POINT ( 'NONE',  ( -4.458734124999999437, -86.56249999863439371, 0.000000000000000000 ) ) ;
#38148=CARTESIAN_POINT ( 'NONE',  ( 5.000000000000000000, -9.500000000000001776, -6.123233995736766282E-16 ) ) ;
#38149=CARTESIAN_POINT ( 'NONE',  ( -5.000000000000000000, -46.87499999726880873, 0.000000000000000000 ) ) ;
#38159=CARTESIAN_POINT ( 'NONE',  ( -2.500000000000000444, -67.04166666393547303, -4.330127018922193649 ) ) ;
#38160=CARTESIAN_POINT ( 'NONE',  ( -2.229367062500000163, -86.72916666530107932, -3.861377020970580443 ) ) ;
#38162=AXIS2_PLACEMENT_3D ( 'NONE', #55865, #41366, #37502 ) ;
#38165=ORIENTED_EDGE ( 'NONE', *, *, #19048, .F. ) ;
#38166=CARTESIAN_POINT ( 'NONE',  ( -2.499999999999996447, -80.83333333333332860, 4.330127018922195425 ) ) ;
#38168=CARTESIAN_POINT ( 'NONE',  ( 2.071067811865475505, -165.9375000027311842, -5.000000000000000888 ) ) ;
#38178=LINE ( 'NONE', #13413, #16215 ) ;
#38179=CARTESIAN_POINT ( 'NONE',  ( 4.458734124999999437, -15.81249999863440436, -5.460374474430324690E-16 ) ) ;
#38182=CARTESIAN_POINT ( 'NONE',  ( 2.229367062500001939, -39.22916666530107221, 3.861377020970579999 ) ) ;
#38183=UNCERTAINTY_MEASURE_WITH_UNIT (LENGTH_MEASURE( 1.000000000000000082E-05 ), #22932, 'distance_accuracy_value', 'NONE');
#38185=CARTESIAN_POINT ( 'NONE',  ( 1.975475456537005874E-15, 0.3750000027311862216, 5.000000000000000000 ) ) ;
#38186=CARTESIAN_POINT ( 'NONE',  ( -6.972266317189433020E-16, 26.87500000273118417, -5.000000000000000000 ) ) ;
#38189=CARTESIAN_POINT ( 'NONE',  ( 2.229367062500001939, 15.02083333469892779, 3.861377020970579999 ) ) ;
#38190=CARTESIAN_POINT ( 'NONE',  ( -4.999999999999998224, -64.79166666393547303, 2.886751345948131764 ) ) ;
#38191=CARTESIAN_POINT ( 'NONE',  ( 4.458734125000000326, -87.14583333196773651, 2.574251347313718519 ) ) ;
#38193=CARTESIAN_POINT ( 'NONE',  ( -4.999999999999999112, 11.20833333606451632, 2.886751345948131764 ) ) ;
#38194=EDGE_LOOP ( 'NONE', ( #25695, #6184, #5704, #26827 ) ) ;
#38195=CARTESIAN_POINT ( 'NONE',  ( 2.500000000000002220, -79.66666666666665719, 4.330127018922192761 ) ) ;
#38198=CARTESIAN_POINT ( 'NONE',  ( -5.000000000000000000, -27.08333333333333215, -2.886751345948128211 ) ) ;
#38199=CARTESIAN_POINT ( 'NONE',  ( -4.458734124999998549, -34.22916666530107221, 2.574251347313722516 ) ) ;
#38201=CARTESIAN_POINT ( 'NONE',  ( 2.500000000000002220, -33.54166666393547303, 4.330127018922192761 ) ) ;
#38203=CARTESIAN_POINT ( 'NONE',  ( -4.458734124999998549, -62.22916666530106511, 2.574251347313722516 ) ) ;
#38204=VERTEX_POINT ( 'NONE', #13781 ) ;
#38206=CARTESIAN_POINT ( 'NONE',  ( 4.458734124999998549, -8.979166665301073991, -2.574251347313721627 ) ) ;
#38207=EDGE_LOOP ( 'NONE', ( #18042, #9845, #33362, #10246 ) ) ;
#38209=CARTESIAN_POINT ( 'NONE',  ( -5.000000000000000000, -77.08333333333334281, -2.886751345948128211 ) ) ;
#38214=CARTESIAN_POINT ( 'NONE',  ( -5.000000000000000000, -81.95833333060213022, -2.886751345948128211 ) ) ;
#38215=FACE_OUTER_BOUND ( 'NONE', #27795, .T. ) ;
#38219=CARTESIAN_POINT ( 'NONE',  ( -3.152548672688508926E-16, -20.81249999863440081, -5.148502694627439702 ) ) ;
#38221=CARTESIAN_POINT ( 'NONE',  ( 2.229367062499998831, -57.89583333196773651, -3.861377020970580887 ) ) ;
#38224=CARTESIAN_POINT ( 'NONE',  ( -4.458734125000001214, -165.1250000013656063, 1.846868145590734089 ) ) ;
#38227=EDGE_CURVE ( 'NONE', #43422, #43716, #59709, .T. ) ;
#38231=EDGE_CURVE ( 'NONE', #62831, #27835, #29829, .T. ) ;
#38235=CARTESIAN_POINT ( 'NONE',  ( -3.152801135295367096, -143.3125000013655779, -3.152801135295367541 ) ) ;
#38239=CARTESIAN_POINT ( 'NONE',  ( 4.458734124999999437, -66.06249999863440792, -5.460374474430324690E-16 ) ) ;
#38240=CARTESIAN_POINT ( 'NONE',  ( 1.339745962155615144, -43.70534180126147561, 4.999999999999999112 ) ) ;
#38242=CARTESIAN_POINT ( 'NONE',  ( 5.000000000000000000, -68.41666666666667140, -2.886751345948130876 ) ) ;
#38249=CARTESIAN_POINT ( 'NONE',  ( 9.457646018065525792E-16, 25.68750000136559208, 5.148502694627439702 ) ) ;
#38255=FACE_OUTER_BOUND ( 'NONE', #20384, .T. ) ;
#38256=CARTESIAN_POINT ( 'NONE',  ( 4.458734125000000326, 0.1041666680322607674, 2.574251347313718519 ) ) ;
#38257=CARTESIAN_POINT ( 'NONE',  ( 2.229367062500001939, -25.22916666530106866, 3.861377020970579999 ) ) ;
#38258=CARTESIAN_POINT ( 'NONE',  ( 1.846868145590736310, -154.6250000013655779, 4.458734124999999437 ) ) ;
#38261=CARTESIAN_POINT ( 'NONE',  ( -2.229367062499996610, 28.85416666803226349, 3.861377020970582219 ) ) ;
#38264=CARTESIAN_POINT ( 'NONE',  ( 4.458734124999999437, -72.06249999863439371, -5.460374474430324690E-16 ) ) ;
#38268=ORIENTED_EDGE ( 'NONE', *, *, #2434, .T. ) ;
#38269=CARTESIAN_POINT ( 'NONE',  ( 0.000000000000000000, -170.0000000000000000, 0.000000000000000000 ) ) ;
#38270=CARTESIAN_POINT ( 'NONE',  ( -2.499999999999996447, 12.29166666939785202, 4.330127018922195425 ) ) ;
#38271=CARTESIAN_POINT ( 'NONE',  ( 5.000000000000000000, -11.41666666666666607, -2.886751345948129988 ) ) ;
#38272=CARTESIAN_POINT ( 'NONE',  ( 2.229367062500001939, -15.97916666530107399, 3.861377020970579999 ) ) ;
#38273=CARTESIAN_POINT ( 'NONE',  ( 2.229367062500001939, -78.97916666530106511, 3.861377020970579999 ) ) ;
#38274=FACE_OUTER_BOUND ( 'NONE', #61218, .T. ) ;
#38275=CARTESIAN_POINT ( 'NONE',  ( 5.000000000000000888, -18.45833333060214798, 2.886751345948126879 ) ) ;
#38276=CARTESIAN_POINT ( 'NONE',  ( 9.457646018065525792E-16, -44.06249999863439371, 5.148502694627439702 ) ) ;
#38277=ORIENTED_EDGE ( 'NONE', *, *, #19414, .F. ) ;
#38279=CARTESIAN_POINT ( 'NONE',  ( 4.458734124999999437, 5.937500001365593860, -5.460374474430324690E-16 ) ) ;
#38281=CARTESIAN_POINT ( 'NONE',  ( 1.975475456537005874E-15, -86.62499999726880162, 5.000000000000000000 ) ) ;
#38282=CARTESIAN_POINT ( 'NONE',  ( -2.499999999999996447, -62.83333333333333570, 4.330127018922195425 ) ) ;
#38283=CARTESIAN_POINT ( 'NONE',  ( 4.458734125000000326, -155.6250000013656063, -1.846868145590734978 ) ) ;
#38285=CARTESIAN_POINT ( 'NONE',  ( 1.975475456537005874E-15, -64.74999999999998579, 5.000000000000000000 ) ) ;
#38286=CARTESIAN_POINT ( 'NONE',  ( -9.184850993605147944E-16, -168.2500000000000000, 5.000000000000000000 ) ) ;
#38287=DIRECTION ( 'NONE',  ( 0.000000000000000000, 0.000000000000000000, 1.000000000000000000 ) ) ;
#38289=CARTESIAN_POINT ( 'NONE',  ( 4.458734124999998549, -4.979166665301072214, -2.574251347313721627 ) ) ;
#38290=CARTESIAN_POINT ( 'NONE',  ( -4.458734124999999437, -40.64583333196773651, -2.574251347313719407 ) ) ;
#38291=( BOUNDED_CURVE ( )  B_SPLINE_CURVE ( 2, ( #61096, #26988, #46607, #56586, #32117, #7697, #47243, #63528, #49032 ),
 .UNSPECIFIED., .F., .F. ) 
 B_SPLINE_CURVE_WITH_KNOTS ( ( 3, 2, 2, 2, 3 ),
 ( 0.4895833333333333148, 0.4902777777777777568, 0.4916666666666666408, 0.4930555555555555802, 0.4937500000000000222 ),
 .UNSPECIFIED. ) 
 CURVE ( )  GEOMETRIC_REPRESENTATION_ITEM ( )  RATIONAL_B_SPLINE_CURVE ( ( 0.9330127018922194093, 0.9330127018922194093, 1.000000000000000000, 0.8660254037844387076, 1.000000000000000000, 0.8660254037844387076, 1.000000000000000000, 0.9330127018922194093, 0.9330127018922194093 ) ) 
 REPRESENTATION_ITEM ( '' )  );
#38293=CARTESIAN_POINT ( 'NONE',  ( 2.730187237215162345E-16, -148.1875000013656063, -4.458734124999999437 ) ) ;
#38297=ADVANCED_FACE ( 'NONE', ( #15372 ), #1239, .T. ) ;
#38298=CARTESIAN_POINT ( 'NONE',  ( -5.000000000000000888, -148.6875000027312126, -2.071067811865475949 ) ) ;
#38300=CARTESIAN_POINT ( 'NONE',  ( 4.458734124999998549, -73.97916666530106511, -2.574251347313721627 ) ) ;
#38303=CARTESIAN_POINT ( 'NONE',  ( -6.972266317189433020E-16, 3.749999999999999556, -5.000000000000000000 ) ) ;
#38306=CARTESIAN_POINT ( 'NONE',  ( -3.152548672688508926E-16, 1.437500001365596525, -5.148502694627439702 ) ) ;
#38308=CARTESIAN_POINT ( 'NONE',  ( 1.846868145590735200, -151.2500000013656063, -4.458734124999999437 ) ) ;
#38312=CARTESIAN_POINT ( 'NONE',  ( 1.975475456537005874E-15, -57.62499999726880873, 5.000000000000000000 ) ) ;
#38315=CARTESIAN_POINT ( 'NONE',  ( -5.000000000000000000, 28.04166666939785202, -2.886751345948128211 ) ) ;
#38316=CARTESIAN_POINT ( 'NONE',  ( 6.123233995736766282E-16, -170.0000000000000000, -5.000000000000000000 ) ) ;
#38319=CARTESIAN_POINT ( 'NONE',  ( 0.000000000000000000, -170.0000000000000000, 0.000000000000000000 ) ) ;
#38321=CARTESIAN_POINT ( 'NONE',  ( 4.458734124999999437, 22.18750000136559564, -5.460374474430324690E-16 ) ) ;
#38323=CARTESIAN_POINT ( 'NONE',  ( -2.229367062499996610, -11.39583333196773829, 3.861377020970582219 ) ) ;
#38324=CARTESIAN_POINT ( 'NONE',  ( -4.999999999999998224, -62.91666666666665719, 2.886751345948131764 ) ) ;
#38326=CARTESIAN_POINT ( 'NONE',  ( -8.190561711645485556E-16, -166.6875000013655779, 4.458734124999999437 ) ) ;
#38327=LINE ( 'NONE', #8123, #40761 ) ;
#38334=CARTESIAN_POINT ( 'NONE',  ( -1.846868145590734756, -157.3750000013655779, -4.458734124999999437 ) ) ;
#38335=( BOUNDED_CURVE ( )  B_SPLINE_CURVE ( 2, ( #52041, #58112, #62950, #52355, #4096, #57191, #48460, #52972, #7980 ),
 .UNSPECIFIED., .F., .F. ) 
 B_SPLINE_CURVE_WITH_KNOTS ( ( 3, 2, 2, 2, 3 ),
 ( 0.9229166666666667185, 0.9236111111111111605, 0.9250000000000000444, 0.9263888888888889284, 0.9270833333333333703 ),
 .UNSPECIFIED. ) 
 CURVE ( )  GEOMETRIC_REPRESENTATION_ITEM ( )  RATIONAL_B_SPLINE_CURVE ( ( 0.9330127018922194093, 0.9330127018922194093, 1.000000000000000000, 0.8660254037844387076, 1.000000000000000000, 0.8660254037844387076, 1.000000000000000000, 0.9330127018922194093, 0.9330127018922194093 ) ) 
 REPRESENTATION_ITEM ( '' )  );
#38338=CARTESIAN_POINT ( 'NONE',  ( 5.000000000000000000, -163.0625000000000000, 2.071067811865478614 ) ) ;
#38344=CARTESIAN_POINT ( 'NONE',  ( 5.000000000000000000, 3.499999999999999556, -6.123233995736766282E-16 ) ) ;
#38345=CARTESIAN_POINT ( 'NONE',  ( 2.229367062500001939, -58.97916666530106511, 3.861377020970579999 ) ) ;
#38347=CARTESIAN_POINT ( 'NONE',  ( 1.060575238724906964E-15, 1.375000002731184834, 5.773502691896257311 ) ) ;
#38348=CARTESIAN_POINT ( 'NONE',  ( 2.229367062500001939, -29.97916666530107221, 3.861377020970579999 ) ) ;
#38349=CARTESIAN_POINT ( 'NONE',  ( 5.000000000000000000, 17.62500000273118417, -6.123233995736766282E-16 ) ) ;
#38351=CARTESIAN_POINT ( 'NONE',  ( 6.123233995736766282E-16, -170.0000000000000000, -5.000000000000000000 ) ) ;
#38352=CARTESIAN_POINT ( 'NONE',  ( -3.535250795749689387E-16, -45.25000000000000000, -5.773502691896257311 ) ) ;
#38353=CARTESIAN_POINT ( 'NONE',  ( 1.975475456537005874E-15, -72.75000000000000000, 5.000000000000000000 ) ) ;
#38355=CARTESIAN_POINT ( 'NONE',  ( 3.535533905932736864, -155.1250000000000000, 3.535533905932738641 ) ) ;
#38356=CARTESIAN_POINT ( 'NONE',  ( 2.229367062499998831, -71.64583333196773651, -3.861377020970580887 ) ) ;
#38357=CARTESIAN_POINT ( 'NONE',  ( 1.846868145590735200, -149.5000000013655779, -4.458734125000000326 ) ) ;
#38358=CARTESIAN_POINT ( 'NONE',  ( 9.457646018065525792E-16, -76.06249999863440792, 5.148502694627439702 ) ) ;
#38360=CARTESIAN_POINT ( 'NONE',  ( 4.458734125000001214, -24.14583333196773651, 2.574251347313718519 ) ) ;
#38361=CARTESIAN_POINT ( 'NONE',  ( 1.060575238724906964E-15, -66.62499999726881583, 5.773502691896257311 ) ) ;
#38362=VERTEX_POINT ( 'NONE', #4755 ) ;
#38364=ORIENTED_EDGE ( 'NONE', *, *, #10634, .F. ) ;
#38366=CARTESIAN_POINT ( 'NONE',  ( -5.000000000000000000, 8.041666669397852019, -2.886751345948128211 ) ) ;
#38367=DIRECTION ( 'NONE',  ( 0.000000000000000000, 0.000000000000000000, 1.000000000000000000 ) ) ;
#38369=CARTESIAN_POINT ( 'NONE',  ( -1.339745962155610925, -82.79465819873851729, 5.000000000000000000 ) ) ;
#38370=CARTESIAN_POINT ( 'NONE',  ( -4.458734124999999437, -55.64583333196773651, -2.574251347313719407 ) ) ;
#38374=CARTESIAN_POINT ( 'NONE',  ( 2.229367062499998831, 18.35416666803225993, -3.861377020970580887 ) ) ;
#38376=CARTESIAN_POINT ( 'NONE',  ( -6.972266317189433020E-16, -2.250000000000000000, -5.000000000000000000 ) ) ;
#38377=CARTESIAN_POINT ( 'NONE',  ( 1.846868145590735200, -164.2500000013656063, -4.458734124999999437 ) ) ;
#38383=CARTESIAN_POINT ( 'NONE',  ( -2.071067811865538566, -162.8125000027311842, -4.999999999999937828 ) ) ;
#38387=CARTESIAN_POINT ( 'NONE',  ( 1.975475456537005874E-15, -45.74999999999999289, 5.000000000000000000 ) ) ;
#38388=CARTESIAN_POINT ( 'NONE',  ( 5.000000000000000000, -61.41666666666665719, -2.886751345948130876 ) ) ;
#38396=CARTESIAN_POINT ( 'NONE',  ( -2.071067811865475061, -150.8125000027311842, -5.000000000000000888 ) ) ;
#38402=CARTESIAN_POINT ( 'NONE',  ( -5.000000000000000888, -143.4375000000000284, 2.071067811865474617 ) ) ;
#38404=DIRECTION ( 'NONE',  ( -0.000000000000000000, 1.000000000000000000, -0.000000000000000000 ) ) ;
#38405=CARTESIAN_POINT ( 'NONE',  ( -2.229367062500000163, -29.47916666530107221, -3.861377020970580443 ) ) ;
#38407=CARTESIAN_POINT ( 'NONE',  ( 1.339745962155612702, -45.16965819600733312, -5.000000000000000000 ) ) ;
#38409=CARTESIAN_POINT ( 'NONE',  ( -4.458734125000000326, -149.0000000013656063, -1.846868145590735644 ) ) ;
#38411=CARTESIAN_POINT ( 'NONE',  ( -3.152548672688508926E-16, -55.81249999863440081, -5.148502694627439702 ) ) ;
#38413=CARTESIAN_POINT ( 'NONE',  ( 1.339745962155615144, -90.58034179853029855, 4.999999999999999112 ) ) ;
#38414=CARTESIAN_POINT ( 'NONE',  ( -5.000000000000000000, 20.99999999999999645, 0.000000000000000000 ) ) ;
#38415=DIRECTION ( 'NONE',  ( -0.000000000000000000, 1.000000000000000000, -0.000000000000000000 ) ) ;
#38416=CARTESIAN_POINT ( 'NONE',  ( 4.458734124999999437, -4.812499998634402587, -5.460374474430324690E-16 ) ) ;
#38417=CARTESIAN_POINT ( 'NONE',  ( -5.000000000000000000, -11.00000000000000355, 0.000000000000000000 ) ) ;
#38418=CARTESIAN_POINT ( 'NONE',  ( -4.458734124999999437, 12.35416666803225993, -2.574251347313719407 ) ) ;
#38419=CARTESIAN_POINT ( 'NONE',  ( 6.972266317189433020E-16, 28.87500000273118417, -5.000000000000000000 ) ) ;
#38420=ORIENTED_EDGE ( 'NONE', *, *, #19666, .T. ) ;
#38422=CARTESIAN_POINT ( 'NONE',  ( -3.152548672688508926E-16, -49.56249999863440792, -5.148502694627439702 ) ) ;
#38423=CARTESIAN_POINT ( 'NONE',  ( 2.730187237215162345E-16, -159.4375000013655779, -4.458734124999999437 ) ) ;
#38424=CARTESIAN_POINT ( 'NONE',  ( 2.499999999999998668, -48.20833333060215153, -4.330127018922193649 ) ) ;
#38426=CARTESIAN_POINT ( 'NONE',  ( 4.458734124999999437, -23.81249999863440436, -5.460374474430324690E-16 ) ) ;
#38427=ORIENTED_EDGE ( 'NONE', *, *, #13364, .F. ) ;
#38428=CARTESIAN_POINT ( 'NONE',  ( 1.339745962155612702, -56.29465819873852439, -5.000000000000000000 ) ) ;
#38430=CARTESIAN_POINT ( 'NONE',  ( -4.458734125000000326, -159.0000000013656063, -1.846868145590735644 ) ) ;
#38431=VERTEX_POINT ( 'NONE', #54929 ) ;
#38434=CARTESIAN_POINT ( 'NONE',  ( -4.999999999999998224, -23.91666666666666785, 2.886751345948131764 ) ) ;
#38435=CARTESIAN_POINT ( 'NONE',  ( -3.152548672688508926E-16, -37.81249999863440792, -5.148502694627439702 ) ) ;
#38439=CARTESIAN_POINT ( 'NONE',  ( 5.000000000000000888, -59.58333333333335702, 2.886751345948126879 ) ) ;
#38440=ORIENTED_EDGE ( 'NONE', *, *, #32984, .T. ) ;
#38441=CARTESIAN_POINT ( 'NONE',  ( -3.152548672688508926E-16, -85.81249999863440792, -5.148502694627439702 ) ) ;
#38443=CARTESIAN_POINT ( 'NONE',  ( 5.000000000000000888, -35.45833333060213732, 2.886751345948126879 ) ) ;
#38445=CARTESIAN_POINT ( 'NONE',  ( 5.000000000000000888, -145.0625000027311842, -2.071067811865475505 ) ) ;
#38447=CARTESIAN_POINT ( 'NONE',  ( 6.123233995736766282E-16, -170.0000000000000000, -5.000000000000000000 ) ) ;
#38453=FACE_OUTER_BOUND ( 'NONE', #161, .T. ) ;
#38455=CARTESIAN_POINT ( 'NONE',  ( -3.152548672688508926E-16, -83.81249999863439371, -5.148502694627439702 ) ) ;
#38458=ORIENTED_EDGE ( 'NONE', *, *, #45601, .F. ) ;
#38459=CARTESIAN_POINT ( 'NONE',  ( -2.071067811865538566, -163.8125000027312126, -4.999999999999937828 ) ) ;
#38461=CARTESIAN_POINT ( 'NONE',  ( 3.535533905932738197, -165.0000000027312126, -3.535533905932738197 ) ) ;
#38463=EDGE_CURVE ( 'NONE', #42072, #26895, #28877, .T. ) ;
#38468=( BOUNDED_CURVE ( )  B_SPLINE_CURVE ( 2, ( #41396, #36579, #57484, #58718, #4680, #14644, #28500, #3444, #48119 ),
 .UNSPECIFIED., .F., .F. ) 
 B_SPLINE_CURVE_WITH_KNOTS ( ( 3, 2, 2, 2, 3 ),
 ( 0.3187499999999999778, 0.3194444444444444198, 0.3208333333333333592, 0.3222222222222222432, 0.3229166666666666852 ),
 .UNSPECIFIED. ) 
 CURVE ( )  GEOMETRIC_REPRESENTATION_ITEM ( )  RATIONAL_B_SPLINE_CURVE ( ( 0.9330127018922194093, 0.9330127018922194093, 1.000000000000000000, 0.8660254037844387076, 1.000000000000000000, 0.8660254037844387076, 1.000000000000000000, 0.9330127018922194093, 0.9330127018922194093 ) ) 
 REPRESENTATION_ITEM ( '' )  );
#38473=CARTESIAN_POINT ( 'NONE',  ( 0.000000000000000000, -170.0000000000000000, 0.000000000000000000 ) ) ;
#38474=CARTESIAN_POINT ( 'NONE',  ( -4.458734124999999437, -14.39583333196773474, -2.574251347313719407 ) ) ;
#38475=DIRECTION ( 'NONE',  ( -0.000000000000000000, 1.000000000000000000, -0.000000000000000000 ) ) ;
#38477=CARTESIAN_POINT ( 'NONE',  ( -2.229367062499996610, -43.39583333196773651, 3.861377020970582219 ) ) ;
#38478=CARTESIAN_POINT ( 'NONE',  ( -5.000000000000000000, -11.99999999999999645, 0.000000000000000000 ) ) ;
#38479=EDGE_CURVE ( 'NONE', #43626, #46822, #24757, .T. ) ;
#38480=CARTESIAN_POINT ( 'NONE',  ( -6.972266317189433020E-16, -30.25000000000000000, -5.000000000000000000 ) ) ;
#38483=CARTESIAN_POINT ( 'NONE',  ( -4.458734124999998549, 14.77083333469892779, 2.574251347313722516 ) ) ;
#38487=CARTESIAN_POINT ( 'NONE',  ( -3.152548672688508926E-16, -89.81249999863440792, -5.148502694627439702 ) ) ;
#38489=CARTESIAN_POINT ( 'NONE',  ( 1.060575238724906964E-15, 13.37500000273118594, 5.773502691896257311 ) ) ;
#38494=CARTESIAN_POINT ( 'NONE',  ( -6.972266317189433020E-16, -85.25000000000000000, -5.000000000000000000 ) ) ;
#38495=CARTESIAN_POINT ( 'NONE',  ( 5.000000000000000000, -26.49999999999999645, -6.123233995736766282E-16 ) ) ;
#38496=CARTESIAN_POINT ( 'NONE',  ( 4.458734124999999437, -32.81249999863440792, -5.460374474430324690E-16 ) ) ;
#38497=CARTESIAN_POINT ( 'NONE',  ( 5.000000000000000000, -36.37499999726881583, -6.123233995736766282E-16 ) ) ;
#38498=CARTESIAN_POINT ( 'NONE',  ( -4.458734124999999437, -68.31249999863439371, 0.000000000000000000 ) ) ;
#38501=CARTESIAN_POINT ( 'NONE',  ( 9.457646018065525792E-16, -15.31249999863440436, 5.148502694627439702 ) ) ;
#38502=ORIENTED_EDGE ( 'NONE', *, *, #33570, .F. ) ;
#38503=CARTESIAN_POINT ( 'NONE',  ( 2.500000000000002220, -77.66666666666665719, 4.330127018922192761 ) ) ;
#38504=CARTESIAN_POINT ( 'NONE',  ( 2.499999999999998668, 28.79166666939784847, -4.330127018922193649 ) ) ;
#38506=CARTESIAN_POINT ( 'NONE',  ( -2.500000000000000444, -84.04166666393547303, -4.330127018922193649 ) ) ;
#38507=DIRECTION ( 'NONE',  ( 0.000000000000000000, 0.000000000000000000, 1.000000000000000000 ) ) ;
#38510=CARTESIAN_POINT ( 'NONE',  ( -4.458734124999998549, -23.47916666530107577, 2.574251347313722516 ) ) ;
#38511=CARTESIAN_POINT ( 'NONE',  ( 4.458734125000001214, -60.14583333196774362, 2.574251347313718519 ) ) ;
#38514=CARTESIAN_POINT ( 'NONE',  ( -3.152801135295367096, -168.3125000013656063, -3.152801135295367541 ) ) ;
#38525=CARTESIAN_POINT ( 'NONE',  ( -4.458734125000001214, -145.1250000013655779, 1.846868145590734089 ) ) ;
#38529=CARTESIAN_POINT ( 'NONE',  ( 2.229367062499998831, -70.89583333196773651, -3.861377020970580887 ) ) ;
#38532=CARTESIAN_POINT ( 'NONE',  ( 1.846868145590735200, -141.2500000013656063, -4.458734124999999437 ) ) ;
#38534=EDGE_LOOP ( 'NONE', ( #36161, #15008, #8405, #21438 ) ) ;
#38540=CARTESIAN_POINT ( 'NONE',  ( -2.229367062499996610, 24.60416666803225993, 3.861377020970582219 ) ) ;
#38549=CARTESIAN_POINT ( 'NONE',  ( -3.152548672688508926E-16, -0.5624999986344053626, -5.148502694627439702 ) ) ;
#38550=CARTESIAN_POINT ( 'NONE',  ( 4.458734124999998549, -22.97916666530107221, -2.574251347313721627 ) ) ;
#38551=CARTESIAN_POINT ( 'NONE',  ( -1.846868145590734756, -155.1250000013655779, -4.458734125000000326 ) ) ;
#38554=ADVANCED_FACE ( 'NONE', ( #61352 ), #41704, .T. ) ;
#38557=CARTESIAN_POINT ( 'NONE',  ( -2.499999999999996447, -83.83333333333332860, 4.330127018922195425 ) ) ;
#38560=CARTESIAN_POINT ( 'NONE',  ( 9.457646018065525792E-16, -71.31249999863439371, 5.148502694627439702 ) ) ;
#38563=CARTESIAN_POINT ( 'NONE',  ( -3.535250795749689387E-16, 27.87500000273118417, -5.773502691896257311 ) ) ;
#38564=ORIENTED_EDGE ( 'NONE', *, *, #32329, .F. ) ;
#38567=CARTESIAN_POINT ( 'NONE',  ( -2.499999999999996447, -11.83333333333333393, 4.330127018922195425 ) ) ;
#38568=CARTESIAN_POINT ( 'NONE',  ( 2.229367062500001939, -18.97916666530106866, 3.861377020970579999 ) ) ;
#38569=CARTESIAN_POINT ( 'NONE',  ( -3.152548672688508926E-16, -77.56249999863440792, -5.148502694627439702 ) ) ;
#38570=CARTESIAN_POINT ( 'NONE',  ( 4.458734125000000326, -169.6250000013656063, -1.846868145590734978 ) ) ;
#38571=CARTESIAN_POINT ( 'NONE',  ( 5.000000000000000888, -19.45833333060214798, 2.886751345948126879 ) ) ;
#38572=CARTESIAN_POINT ( 'NONE',  ( -2.229367062499996610, -44.14583333196774362, 3.861377020970582219 ) ) ;
#38574=CARTESIAN_POINT ( 'NONE',  ( 5.000000000000000888, -15.45833333060214443, 2.886751345948126879 ) ) ;
#38575=CARTESIAN_POINT ( 'NONE',  ( -2.229367062500000163, 1.270833334698927342, -3.861377020970580443 ) ) ;
#38576=ORIENTED_EDGE ( 'NONE', *, *, #56679, .T. ) ;
#38577=CARTESIAN_POINT ( 'NONE',  ( -4.999999999999998224, -86.79166666393547303, 2.886751345948131764 ) ) ;
#38578=CARTESIAN_POINT ( 'NONE',  ( -3.535250795749689387E-16, -63.25000000000000000, -5.773502691896257311 ) ) ;
#38579=CARTESIAN_POINT ( 'NONE',  ( 4.458734125000000326, -154.6250000013655779, -1.846868145590734978 ) ) ;
#38581=CARTESIAN_POINT ( 'NONE',  ( -2.500000000000000444, -79.16666666666665719, -4.330127018922193649 ) ) ;
#38582=CARTESIAN_POINT ( 'NONE',  ( -5.000000000000000888, -161.5625000000000568, -2.071067811865475949 ) ) ;
#38583=CARTESIAN_POINT ( 'NONE',  ( -9.184850993605147944E-16, -168.2500000000000000, 5.000000000000000000 ) ) ;
#38585=CARTESIAN_POINT ( 'NONE',  ( -4.458734124999999437, -4.562499998634401699, 0.000000000000000000 ) ) ;
#38586=CARTESIAN_POINT ( 'NONE',  ( -4.458734124999998549, -38.47916666530107221, 2.574251347313722516 ) ) ;
#38588=CARTESIAN_POINT ( 'NONE',  ( 4.458734124999999437, -148.5000000013656347, 1.846868145590737864 ) ) ;
#38591=ORIENTED_EDGE ( 'NONE', *, *, #37404, .F. ) ;
#38594=CARTESIAN_POINT ( 'NONE',  ( 2.499999999999998668, -2.208333330602146205, -4.330127018922193649 ) ) ;
#38595=CARTESIAN_POINT ( 'NONE',  ( 9.457646018065525792E-16, -75.31249999863440792, 5.148502694627439702 ) ) ;
#38596=ORIENTED_EDGE ( 'NONE', *, *, #18020, .F. ) ;
#38597=VECTOR ( 'NONE', #26890, 1000.000000000000000 ) ;
#38602=CARTESIAN_POINT ( 'NONE',  ( -4.458734124999998549, -0.2291666653010705768, 2.574251347313722516 ) ) ;
#38603=CARTESIAN_POINT ( 'NONE',  ( 5.000000000000000888, -30.45833333060214443, 2.886751345948126879 ) ) ;
#38604=CARTESIAN_POINT ( 'NONE',  ( 4.458734124999999437, -154.3750000013655779, -1.846868145590734978 ) ) ;
#38615=FACE_OUTER_BOUND ( 'NONE', #11468, .T. ) ;
#38617=CARTESIAN_POINT ( 'NONE',  ( -1.339745962155613812, -72.20534180126148271, -5.000000000000000000 ) ) ;
#38619=CARTESIAN_POINT ( 'NONE',  ( 2.229367062499998831, 19.35416666803225993, -3.861377020970580887 ) ) ;
#38621=CARTESIAN_POINT ( 'NONE',  ( -3.152548672688508926E-16, -8.812499998634406140, -5.148502694627439702 ) ) ;
#38622=CARTESIAN_POINT ( 'NONE',  ( 1.975475456537005874E-15, -15.62499999726881406, 5.000000000000000000 ) ) ;
#38624=CARTESIAN_POINT ( 'NONE',  ( 2.730187237215162345E-16, -166.1875000013655779, -4.458734124999999437 ) ) ;
#38632=CARTESIAN_POINT ( 'NONE',  ( -1.846868145590734756, -155.3750000013656063, -4.458734124999999437 ) ) ;
#38635=EDGE_CURVE ( 'NONE', #1769, #7560, #63088, .T. ) ;
#38641=DIRECTION ( 'NONE',  ( -0.000000000000000000, 1.000000000000000000, -0.000000000000000000 ) ) ;
#38642=ADVANCED_FACE ( 'NONE', ( #55467 ), #25543, .T. ) ;
#38643=CARTESIAN_POINT ( 'NONE',  ( 1.060575238724906964E-15, 4.250000000000000000, 5.773502691896257311 ) ) ;
#38645=CARTESIAN_POINT ( 'NONE',  ( 2.229367062499998831, -61.64583333196774362, -3.861377020970580887 ) ) ;
#38649=CARTESIAN_POINT ( 'NONE',  ( -2.500000000000000444, -2.041666663935480575, -4.330127018922193649 ) ) ;
#38650=CARTESIAN_POINT ( 'NONE',  ( -4.458734124999999437, -26.31249999863440792, 0.000000000000000000 ) ) ;
#38652=CARTESIAN_POINT ( 'NONE',  ( -6.972266317189433020E-16, -48.12499999726880873, -5.000000000000000000 ) ) ;
#38653=DIRECTION ( 'NONE',  ( -0.000000000000000000, 1.000000000000000000, -0.000000000000000000 ) ) ;
#38654=CARTESIAN_POINT ( 'NONE',  ( -4.999999999999999112, -43.91666666666665719, 2.886751345948131764 ) ) ;
#38657=CARTESIAN_POINT ( 'NONE',  ( -2.498395430326213474E-14, 15.37500000273118239, 5.000000000000000000 ) ) ;
#38658=CARTESIAN_POINT ( 'NONE',  ( -4.458734124999999437, -68.39583333196773651, -2.574251347313719407 ) ) ;
#38659=CARTESIAN_POINT ( 'NONE',  ( 4.458734125000000326, -144.6250000013655779, -1.846868145590734978 ) ) ;
#38660=CARTESIAN_POINT ( 'NONE',  ( 2.229367062499998831, -78.64583333196773651, -3.861377020970580887 ) ) ;
#38662=CARTESIAN_POINT ( 'NONE',  ( -4.458734124999999437, -23.64583333196773651, -2.574251347313719407 ) ) ;
#38663=CARTESIAN_POINT ( 'NONE',  ( -5.000000000000000000, -66.87499999726881583, 0.000000000000000000 ) ) ;
#38666=ORIENTED_EDGE ( 'NONE', *, *, #56989, .F. ) ;
#38668=CARTESIAN_POINT ( 'NONE',  ( 5.000000000000000888, -165.9375000000000000, -2.071067811865475505 ) ) ;
#38669=( NAMED_UNIT ( * ) SI_UNIT ( $, .STERADIAN. ) SOLID_ANGLE_UNIT ( ) );
#38670=ORIENTED_EDGE ( 'NONE', *, *, #34651, .T. ) ;
#38673=CARTESIAN_POINT ( 'NONE',  ( 2.229367062500001939, -61.22916666530106511, 3.861377020970579999 ) ) ;
#38675=ORIENTED_EDGE ( 'NONE', *, *, #23973, .F. ) ;
#38677=CARTESIAN_POINT ( 'NONE',  ( 2.229367062499998831, 13.35416666803226171, -3.861377020970580887 ) ) ;
#38679=CARTESIAN_POINT ( 'NONE',  ( -2.500000000000000444, -2.166666666666663854, -4.330127018922193649 ) ) ;
#38680=CARTESIAN_POINT ( 'NONE',  ( -1.846868145590734756, -163.1250000013656347, -4.458734124999999437 ) ) ;
#38683=CARTESIAN_POINT ( 'NONE',  ( -2.071067811865308972, -153.3125000000000284, 5.000000000000169642 ) ) ;
#38685=AXIS2_PLACEMENT_3D ( 'NONE', #55129, #44505, #30350 ) ;
#38686=CARTESIAN_POINT ( 'NONE',  ( 2.500000000000002220, -19.54166666393548013, 4.330127018922192761 ) ) ;
#38690=DIRECTION ( 'NONE',  ( -0.000000000000000000, 1.000000000000000000, -0.000000000000000000 ) ) ;
#38697=CARTESIAN_POINT ( 'NONE',  ( 2.229367062499998831, 6.104166668032262599, -3.861377020970580887 ) ) ;
#38698=FACE_OUTER_BOUND ( 'NONE', #27484, .T. ) ;
#38700=CARTESIAN_POINT ( 'NONE',  ( -3.535533905932737309, -148.7500000027311842, -3.535533905932738197 ) ) ;
#38705=CARTESIAN_POINT ( 'NONE',  ( -5.000000000000000000, -141.5000000000000284, -6.123233995736766282E-16 ) ) ;
#38707=CARTESIAN_POINT ( 'NONE',  ( 9.457646018065525792E-16, -31.06249999863440436, 5.148502694627439702 ) ) ;
#38711=CARTESIAN_POINT ( 'NONE',  ( 4.458734124999999437, -143.5000000013656063, 1.846868145590737864 ) ) ;
#38713=CARTESIAN_POINT ( 'NONE',  ( -4.458734124999999437, 26.43750000136559564, 0.000000000000000000 ) ) ;
#38715=CARTESIAN_POINT ( 'NONE',  ( -4.458734124999997661, -57.47916666530108643, 2.574251347313722516 ) ) ;
#38718=CARTESIAN_POINT ( 'NONE',  ( 2.499999999999998668, 16.66666666666666785, -4.330127018922193649 ) ) ;
#38720=CARTESIAN_POINT ( 'NONE',  ( -4.458734124999998549, -6.229166665301072214, 2.574251347313722516 ) ) ;
#38721=CARTESIAN_POINT ( 'NONE',  ( -2.071067811865459518, -168.3125000000000284, 5.000000000000019540 ) ) ;
#38727=VECTOR ( 'NONE', #61207, 1000.000000000000000 ) ;
#38729=CARTESIAN_POINT ( 'NONE',  ( 2.229367062500001939, -55.97916666530107221, 3.861377020970579999 ) ) ;
#38730=CARTESIAN_POINT ( 'NONE',  ( 1.846868145590735200, -160.5000000013656347, -4.458734125000000326 ) ) ;
#38731=CARTESIAN_POINT ( 'NONE',  ( -3.535250795749689387E-16, -50.12499999726881583, -5.773502691896257311 ) ) ;
#38732=ORIENTED_EDGE ( 'NONE', *, *, #26024, .F. ) ;
#38734=CARTESIAN_POINT ( 'NONE',  ( -4.458734124999999437, 7.437500001365594748, 0.000000000000000000 ) ) ;
#38735=ORIENTED_EDGE ( 'NONE', *, *, #3572, .F. ) ;
#38738=CARTESIAN_POINT ( 'NONE',  ( 4.458734124999999437, -162.4375000013655779, 0.000000000000000000 ) ) ;
#38739=EDGE_LOOP ( 'NONE', ( #58559, #5752, #47153, #19322 ) ) ;
#38740=( BOUNDED_CURVE ( )  B_SPLINE_CURVE ( 2, ( #684, #53430, #48598, #30244, #9363, #39259, #28976, #54058, #29930 ),
 .UNSPECIFIED., .F., .F. ) 
 B_SPLINE_CURVE_WITH_KNOTS ( ( 3, 2, 2, 2, 3 ),
 ( 0.9854166666666667185, 0.9861111111111111605, 0.9875000000000000444, 0.9888888888888889284, 0.9895833333333333703 ),
 .UNSPECIFIED. ) 
 CURVE ( )  GEOMETRIC_REPRESENTATION_ITEM ( )  RATIONAL_B_SPLINE_CURVE ( ( 0.9330127018922194093, 0.9330127018922194093, 1.000000000000000000, 0.8660254037844387076, 1.000000000000000000, 0.8660254037844387076, 1.000000000000000000, 0.9330127018922194093, 0.9330127018922194093 ) ) 
 REPRESENTATION_ITEM ( '' )  );
#38744=CARTESIAN_POINT ( 'NONE',  ( -5.000000000000000000, -58.95833333060213732, -2.886751345948128211 ) ) ;
#38745=CARTESIAN_POINT ( 'NONE',  ( 2.229367062500001939, -43.22916666530107932, 3.861377020970579999 ) ) ;
#38746=VERTEX_POINT ( 'NONE', #24911 ) ;
#38751=CARTESIAN_POINT ( 'NONE',  ( -2.229367062499996610, -85.39583333196773651, 3.861377020970582219 ) ) ;
#38753=CARTESIAN_POINT ( 'NONE',  ( 2.499999999999998668, -35.20833333060213732, -4.330127018922193649 ) ) ;
#38755=CARTESIAN_POINT ( 'NONE',  ( -2.499999999999996447, 24.16666666666666785, 4.330127018922195425 ) ) ;
#38757=CARTESIAN_POINT ( 'NONE',  ( -5.000000000000000000, -61.87499999726880873, 0.000000000000000000 ) ) ;
#38763=CARTESIAN_POINT ( 'NONE',  ( 6.123233995736766282E-16, -170.0000000000000000, -5.000000000000000000 ) ) ;
#38765=CARTESIAN_POINT ( 'NONE',  ( -3.152548672688508926E-16, -85.81249999863440792, -5.148502694627439702 ) ) ;
#38769=AXIS2_PLACEMENT_3D ( 'NONE', #48576, #22584, #9032 ) ;
#38770=CARTESIAN_POINT ( 'NONE',  ( -5.000000000000000000, -81.00000000000000000, 0.000000000000000000 ) ) ;
#38772=CARTESIAN_POINT ( 'NONE',  ( -5.000000000000000888, -161.5625000027311842, 2.071067811865474617 ) ) ;
#38783=CARTESIAN_POINT ( 'NONE',  ( 9.457646018065525792E-16, -16.06249999863440436, 5.148502694627439702 ) ) ;
#38784=CARTESIAN_POINT ( 'NONE',  ( 6.123233995736766282E-16, -170.0000000000000000, -5.000000000000000000 ) ) ;
#38785=CARTESIAN_POINT ( 'NONE',  ( -3.535533905932737309, -153.6250000000000000, -3.535533905932738197 ) ) ;
#38786=ORIENTED_EDGE ( 'NONE', *, *, #39359, .F. ) ;
#38787=CARTESIAN_POINT ( 'NONE',  ( -3.152548672688508926E-16, -42.81249999863440081, -5.148502694627439702 ) ) ;
#38788=CARTESIAN_POINT ( 'NONE',  ( 1.975475456537005874E-15, -83.62499999726878741, 5.000000000000000000 ) ) ;
#38793=CARTESIAN_POINT ( 'NONE',  ( 4.458734124999999437, 11.18750000136559386, -5.460374474430324690E-16 ) ) ;
#38794=CARTESIAN_POINT ( 'NONE',  ( -5.000000000000000000, 30.00000000000000000, 0.000000000000000000 ) ) ;
#38795=CARTESIAN_POINT ( 'NONE',  ( -5.000000000000000000, -165.6250000027312126, -6.123233995736766282E-16 ) ) ;
#38796=CARTESIAN_POINT ( 'NONE',  ( 2.229367062499998831, -88.89583333196773651, -3.861377020970580887 ) ) ;
#38798=CARTESIAN_POINT ( 'NONE',  ( -5.000000000000000000, 15.04166666939785202, -2.886751345948128211 ) ) ;
#38800=CARTESIAN_POINT ( 'NONE',  ( 5.000000000000000888, -79.58333333333332860, 2.886751345948126879 ) ) ;
#38803=FACE_OUTER_BOUND ( 'NONE', #20230, .T. ) ;
#38804=CARTESIAN_POINT ( 'NONE',  ( 5.000000000000000888, -33.58333333333332860, 2.886751345948126879 ) ) ;
#38805=CARTESIAN_POINT ( 'NONE',  ( 4.458734125000001214, -36.89583333196773651, 2.574251347313718519 ) ) ;
#38806=CARTESIAN_POINT ( 'NONE',  ( -4.999999999999999112, -31.79166666393548724, 2.886751345948131764 ) ) ;
#38807=CARTESIAN_POINT ( 'NONE',  ( -2.229367062500000163, -65.47916666530106511, -3.861377020970580443 ) ) ;
#38810=CARTESIAN_POINT ( 'NONE',  ( 4.458734124999999437, -11.81249999863440081, -5.460374474430324690E-16 ) ) ;
#38811=CARTESIAN_POINT ( 'NONE',  ( 4.458734125000001214, -15.14583333196773651, 2.574251347313718519 ) ) ;
#38813=CARTESIAN_POINT ( 'NONE',  ( 5.000000000000000000, -76.41666666666665719, -2.886751345948129988 ) ) ;
#38816=APPLICATION_CONTEXT ( 'automotive_design' ) ;
#38817=CARTESIAN_POINT ( 'NONE',  ( -5.000000000000000000, -79.87499999726881583, 0.000000000000000000 ) ) ;
#38818=LINE ( 'NONE', #39456, #35454 ) ;
#38823=CARTESIAN_POINT ( 'NONE',  ( 9.457646018065525792E-16, -24.31249999863440792, 5.148502694627439702 ) ) ;
#38824=VERTEX_POINT ( 'NONE', #39369 ) ;
#38825=( BOUNDED_CURVE ( )  B_SPLINE_CURVE ( 2, ( #47617, #3265, #47926, #57607, #43413, #3570, #18665, #62433, #32833 ),
 .UNSPECIFIED., .F., .F. ) 
 B_SPLINE_CURVE_WITH_KNOTS ( ( 3, 2, 2, 2, 3 ),
 ( 0.3437500000000000000, 0.3444444444444444420, 0.3458333333333333259, 0.3472222222222222099, 0.3479166666666666519 ),
 .UNSPECIFIED. ) 
 CURVE ( )  GEOMETRIC_REPRESENTATION_ITEM ( )  RATIONAL_B_SPLINE_CURVE ( ( 0.9330127018922194093, 0.9330127018922194093, 1.000000000000000000, 0.8660254037844387076, 1.000000000000000000, 0.8660254037844387076, 1.000000000000000000, 0.9330127018922194093, 0.9330127018922194093 ) ) 
 REPRESENTATION_ITEM ( '' )  );
#38827=CARTESIAN_POINT ( 'NONE',  ( 4.458734125000000326, -168.6250000013655779, -1.846868145590734978 ) ) ;
#38838=VERTEX_POINT ( 'NONE', #49348 ) ;
#38841=CARTESIAN_POINT ( 'NONE',  ( 1.846868145590735200, -142.5000000013656347, -4.458734125000000326 ) ) ;
#38843=EDGE_CURVE ( 'NONE', #49754, #19960, #43709, .T. ) ;
#38846=CARTESIAN_POINT ( 'NONE',  ( 2.229367062499998831, -66.89583333196773651, -3.861377020970580887 ) ) ;
#38848=CARTESIAN_POINT ( 'NONE',  ( 6.123233995736766282E-16, -170.0000000000000000, -5.000000000000000000 ) ) ;
#38849=CARTESIAN_POINT ( 'NONE',  ( -3.152801135295367985, -141.8125000013655779, 3.152801135295367096 ) ) ;
#38851=ORIENTED_EDGE ( 'NONE', *, *, #61048, .F. ) ;
#38857=CARTESIAN_POINT ( 'NONE',  ( -2.229367062500000163, 25.27083333469892779, -3.861377020970580443 ) ) ;
#38858=CARTESIAN_POINT ( 'NONE',  ( -4.764381983412779477E-15, 27.25000000000000000, 5.000000000000000000 ) ) ;
#38864=CARTESIAN_POINT ( 'NONE',  ( -4.458734124999997661, -0.2291666653010705768, 2.574251347313722516 ) ) ;
#38866=CARTESIAN_POINT ( 'NONE',  ( 2.229367062499998831, -26.89583333196774007, -3.861377020970580887 ) ) ;
#38867=AXIS2_PLACEMENT_3D ( 'NONE', #5553, #52629, #25165 ) ;
#38871=CARTESIAN_POINT ( 'NONE',  ( 4.458734124999999437, 27.18750000136559564, -5.460374474430324690E-16 ) ) ;
#38873=EDGE_CURVE ( 'NONE', #30395, #49021, #58936, .T. ) ;
#38874=DIRECTION ( 'NONE',  ( -0.000000000000000000, 1.000000000000000000, -0.000000000000000000 ) ) ;
#38875=CARTESIAN_POINT ( 'NONE',  ( 4.458734124999998549, -70.97916666530107932, -2.574251347313721627 ) ) ;
#38878=CARTESIAN_POINT ( 'NONE',  ( 2.499999999999998668, 28.79166666939784847, -4.330127018922193649 ) ) ;
#38879=ORIENTED_EDGE ( 'NONE', *, *, #48019, .F. ) ;
#38881=CARTESIAN_POINT ( 'NONE',  ( 1.339745962155612702, 2.830341803992664662, -5.000000000000000000 ) ) ;
#38882=CARTESIAN_POINT ( 'NONE',  ( 5.000000000000000000, -14.49999999999999822, -6.123233995736766282E-16 ) ) ;
#38883=CARTESIAN_POINT ( 'NONE',  ( 4.458734124999998549, -14.72916666530107399, -2.574251347313721627 ) ) ;
#38884=CARTESIAN_POINT ( 'NONE',  ( -4.458734124999999437, -83.31249999863439371, 0.000000000000000000 ) ) ;
#38885=VECTOR ( 'NONE', #11036, 1000.000000000000000 ) ;
#38886=CARTESIAN_POINT ( 'NONE',  ( 1.846868145590736310, -166.8750000013655779, 4.458734124999999437 ) ) ;
#38887=CARTESIAN_POINT ( 'NONE',  ( -5.000000000000000000, -15.95833333060214443, -2.886751345948128211 ) ) ;
#38888=CARTESIAN_POINT ( 'NONE',  ( 2.229367062500001939, -50.97916666530107221, 3.861377020970579999 ) ) ;
#38889=EDGE_LOOP ( 'NONE', ( #55472, #34817, #63295, #29386 ) ) ;
#38890=CARTESIAN_POINT ( 'NONE',  ( -2.499999999999996447, -27.70833333060214798, 4.330127018922195425 ) ) ;
#38891=CARTESIAN_POINT ( 'NONE',  ( -3.152548672688508926E-16, 1.187500001365596081, -5.148502694627439702 ) ) ;
#38892=ORIENTED_EDGE ( 'NONE', *, *, #16043, .F. ) ;
#38893=CARTESIAN_POINT ( 'NONE',  ( 1.975475456537005874E-15, -34.62499999726880873, 5.000000000000000000 ) ) ;
#38894=CARTESIAN_POINT ( 'NONE',  ( 5.000000000000000000, -63.41666666666665719, -2.886751345948129988 ) ) ;
#38895=CARTESIAN_POINT ( 'NONE',  ( 4.458734124999999437, -156.7500000013656063, 1.846868145590737864 ) ) ;
#38897=CARTESIAN_POINT ( 'NONE',  ( 2.500000000000002220, -14.66666666666666785, 4.330127018922192761 ) ) ;
#38898=( BOUNDED_CURVE ( )  B_SPLINE_CURVE ( 2, ( #42140, #3244, #62092, #57273, #13191, #47598, #28292, #23481, #39831 ),
 .UNSPECIFIED., .F., .F. ) 
 B_SPLINE_CURVE_WITH_KNOTS ( ( 3, 2, 2, 2, 3 ),
 ( 0.1145833333333333426, 0.1152777777777777846, 0.1166666666666666685, 0.1180555555555555525, 0.1187500000000000083 ),
 .UNSPECIFIED. ) 
 CURVE ( )  GEOMETRIC_REPRESENTATION_ITEM ( )  RATIONAL_B_SPLINE_CURVE ( ( 0.9330127018922194093, 0.9330127018922200755, 1.000000000000000000, 0.8660254037844387076, 1.000000000000000000, 0.8660254037844387076, 1.000000000000000000, 0.9330127018922187432, 0.9330127018922194093 ) ) 
 REPRESENTATION_ITEM ( '' )  );
#38899=CARTESIAN_POINT ( 'NONE',  ( -2.071067811865475061, -160.6875000000000284, -5.000000000000000888 ) ) ;
#38903=CARTESIAN_POINT ( 'NONE',  ( -3.152548672688508926E-16, -4.812499998634402587, -5.148502694627439702 ) ) ;
#38904=CARTESIAN_POINT ( 'NONE',  ( 4.458734124999998549, -47.97916666530107221, -2.574251347313721627 ) ) ;
#38906=ADVANCED_FACE ( 'NONE', ( #41922 ), #61564, .T. ) ;
#38907=CARTESIAN_POINT ( 'NONE',  ( 3.535533905932738197, -151.0000000027312126, -3.535533905932738197 ) ) ;
#38908=CARTESIAN_POINT ( 'NONE',  ( 3.152801135295367541, -147.3125000013655779, -3.152801135295367541 ) ) ;
#38912=CARTESIAN_POINT ( 'NONE',  ( -6.972266317189433020E-16, 2.875000002731185500, -5.000000000000000000 ) ) ;
#38913=CARTESIAN_POINT ( 'NONE',  ( -2.229367062500000163, 28.27083333469892779, -3.861377020970580443 ) ) ;
#38916=ORIENTED_EDGE ( 'NONE', *, *, #28411, .F. ) ;
#38919=EDGE_CURVE ( 'NONE', #2786, #30395, #46445, .T. ) ;
#38920=CARTESIAN_POINT ( 'NONE',  ( -4.458734124999999437, -0.3124999986344051406, 0.000000000000000000 ) ) ;
#38922=CARTESIAN_POINT ( 'NONE',  ( -4.458734125000000326, -154.8750000013655779, 1.846868145590734089 ) ) ;
#38928=CARTESIAN_POINT ( 'NONE',  ( 1.339745962155612702, -40.29465819873851729, -5.000000000000000000 ) ) ;
#38931=CARTESIAN_POINT ( 'NONE',  ( -5.000000000000000000, -12.99999999999999822, 0.000000000000000000 ) ) ;
#38938=CARTESIAN_POINT ( 'NONE',  ( 4.458734124999999437, 19.18750000136559564, -5.460374474430324690E-16 ) ) ;
#38940=CARTESIAN_POINT ( 'NONE',  ( -4.458734124999999437, -8.562499998634406140, 0.000000000000000000 ) ) ;
#38941=CARTESIAN_POINT ( 'NONE',  ( -6.972266317189433020E-16, -31.24999999999999645, -5.000000000000000000 ) ) ;
#38943=CARTESIAN_POINT ( 'NONE',  ( 4.458734125000000326, -169.3750000013656347, -1.846868145590734978 ) ) ;
#38947=CARTESIAN_POINT ( 'NONE',  ( -6.972266317189433020E-16, -38.25000000000000000, -5.000000000000000000 ) ) ;
#38949=DIRECTION ( 'NONE',  ( -0.000000000000000000, 1.000000000000000000, -0.000000000000000000 ) ) ;
#38950=CARTESIAN_POINT ( 'NONE',  ( -4.458734124999999437, -152.1875000013656063, -5.460374474430324690E-16 ) ) ;
#38953=CARTESIAN_POINT ( 'NONE',  ( 0.000000000000000000, -170.0000000000000000, 5.000000000000000000 ) ) ;
#38954=ORIENTED_EDGE ( 'NONE', *, *, #13436, .F. ) ;
#38957=( GEOMETRIC_REPRESENTATION_CONTEXT ( 3 ) GLOBAL_UNCERTAINTY_ASSIGNED_CONTEXT ( ( #19121 ) ) GLOBAL_UNIT_ASSIGNED_CONTEXT ( ( #4901, #5540, #38669 ) ) REPRESENTATION_CONTEXT ( 'NONE', 'WORKASPACE' ) );
#38958=CARTESIAN_POINT ( 'NONE',  ( 3.535533905932738197, -161.8750000000000284, -3.535533905932738197 ) ) ;
#38959=CARTESIAN_POINT ( 'NONE',  ( 1.060575238724906964E-15, 2.249999999999998668, 5.773502691896257311 ) ) ;
#38960=VECTOR ( 'NONE', #57729, 1000.000000000000000 ) ;
#38961=CARTESIAN_POINT ( 'NONE',  ( 4.458734124999999437, -62.81249999863440792, -5.460374474430324690E-16 ) ) ;
#38963=CARTESIAN_POINT ( 'NONE',  ( 2.500000000000002220, -2.541666663935477466, 4.330127018922192761 ) ) ;
#38964=CARTESIAN_POINT ( 'NONE',  ( -4.458734124999999437, -31.39583333196773296, -2.574251347313719407 ) ) ;
#38965=ORIENTED_EDGE ( 'NONE', *, *, #1280, .F. ) ;
#38967=CARTESIAN_POINT ( 'NONE',  ( -1.339745962155613812, -48.08034179853029144, -5.000000000000000000 ) ) ;
#38969=CARTESIAN_POINT ( 'NONE',  ( 2.500000000000002220, -45.66666666666666430, 4.330127018922192761 ) ) ;
#38970=CARTESIAN_POINT ( 'NONE',  ( 0.000000000000000000, -170.0000000000000000, 5.000000000000000000 ) ) ;
#38972=CARTESIAN_POINT ( 'NONE',  ( 2.500000000000002220, -4.541666663935479242, 4.330127018922192761 ) ) ;
#38973=CARTESIAN_POINT ( 'NONE',  ( 9.457646018065525792E-16, -68.06249999863440792, 5.148502694627439702 ) ) ;
#38974=CARTESIAN_POINT ( 'NONE',  ( -3.152801135295367985, -145.0625000013655779, 3.152801135295367096 ) ) ;
#38975=CARTESIAN_POINT ( 'NONE',  ( -3.152548672688508926E-16, -74.56249999863440792, -5.148502694627439702 ) ) ;
#38977=CARTESIAN_POINT ( 'NONE',  ( 2.229367062499998831, -29.89583333196773296, -3.861377020970580887 ) ) ;
#38978=CARTESIAN_POINT ( 'NONE',  ( -3.535250795749689387E-16, -68.12499999726881583, -5.773502691896257311 ) ) ;
#38979=EDGE_CURVE ( 'NONE', #53169, #53313, #6363, .T. ) ;
#38982=ORIENTED_EDGE ( 'NONE', *, *, #48346, .F. ) ;
#38985=EDGE_CURVE ( 'NONE', #12164, #7641, #52219, .T. ) ;
#38989=EDGE_CURVE ( 'NONE', #29232, #25897, #47852, .T. ) ;
#38990=DIRECTION ( 'NONE',  ( -0.000000000000000000, 1.000000000000000000, -0.000000000000000000 ) ) ;
#38991=CARTESIAN_POINT ( 'NONE',  ( -4.458734124999999437, -61.64583333196773651, -2.574251347313719407 ) ) ;
#38996=CARTESIAN_POINT ( 'NONE',  ( 5.000000000000000000, -142.0000000000000284, 0.000000000000000000 ) ) ;
#38998=EDGE_CURVE ( 'NONE', #15810, #50806, #30184, .T. ) ;
#38999=CARTESIAN_POINT ( 'NONE',  ( 4.458734124999998549, 14.27083333469892779, -2.574251347313721627 ) ) ;
#39001=CARTESIAN_POINT ( 'NONE',  ( -1.339745962155610925, -1.794658198738520616, 5.000000000000000000 ) ) ;
#39002=CARTESIAN_POINT ( 'NONE',  ( -8.190561711645485556E-16, -166.6875000013655779, 4.458734124999999437 ) ) ;
#39007=CARTESIAN_POINT ( 'NONE',  ( -4.764381983412779477E-15, 26.25000000000000000, 5.000000000000000000 ) ) ;
#39009=VECTOR ( 'NONE', #29628, 1000.000000000000114 ) ;
#39010=EDGE_CURVE ( 'NONE', #38431, #35874, #52539, .T. ) ;
#39011=CARTESIAN_POINT ( 'NONE',  ( -5.000000000000000000, 1.916666666666667407, -2.886751345948128211 ) ) ;
#39014=CARTESIAN_POINT ( 'NONE',  ( -5.000000000000000000, 5.916666666666666963, -2.886751345948128211 ) ) ;
#39015=CARTESIAN_POINT ( 'NONE',  ( 2.500000000000002220, -45.66666666666666430, 4.330127018922192761 ) ) ;
#39019=CARTESIAN_POINT ( 'NONE',  ( -4.458734124999999437, 5.354166668032261711, -2.574251347313719407 ) ) ;
#39022=CARTESIAN_POINT ( 'NONE',  ( -2.071067811865478170, -148.4375000027312126, 5.000000000000000000 ) ) ;
#39028=CARTESIAN_POINT ( 'NONE',  ( 2.071067811865476394, -143.1875000000000000, 5.000000000000000000 ) ) ;
#39030=CARTESIAN_POINT ( 'NONE',  ( -3.152801135295367096, -167.3125000013656063, -3.152801135295367541 ) ) ;
#39031=CARTESIAN_POINT ( 'NONE',  ( 4.458734124999999437, -31.81249999863440436, -5.460374474430324690E-16 ) ) ;
#39035=CARTESIAN_POINT ( 'NONE',  ( 4.458734125000000326, -145.3750000013656347, -1.846868145590734978 ) ) ;
#39037=CARTESIAN_POINT ( 'NONE',  ( 2.229367062499998831, 26.10416666803225993, -3.861377020970580887 ) ) ;
#39038=CARTESIAN_POINT ( 'NONE',  ( 4.458734124999999437, -56.06249999863440081, -5.460374474430324690E-16 ) ) ;
#39040=CARTESIAN_POINT ( 'NONE',  ( -2.500000000000000444, 18.83333333333333215, -4.330127018922193649 ) ) ;
#39041=CARTESIAN_POINT ( 'NONE',  ( -9.184850993605147944E-16, -168.2500000000000000, 5.000000000000000000 ) ) ;
#39042=CARTESIAN_POINT ( 'NONE',  ( 2.229367062499998831, -5.645833331967740953, -3.861377020970580887 ) ) ;
#39043=DIRECTION ( 'NONE',  ( 0.000000000000000000, 0.000000000000000000, 1.000000000000000000 ) ) ;
#39050=CARTESIAN_POINT ( 'NONE',  ( 4.458734124999998549, -55.72916666530107221, -2.574251347313721627 ) ) ;
#39051=CARTESIAN_POINT ( 'NONE',  ( -3.152801135295367096, -154.3125000013656063, -3.152801135295367541 ) ) ;
#39053=CARTESIAN_POINT ( 'NONE',  ( -5.000000000000000000, -49.95833333060213022, -2.886751345948128211 ) ) ;
#39055=CARTESIAN_POINT ( 'NONE',  ( 2.229367062499998831, 4.104166668032260823, -3.861377020970580887 ) ) ;
#39056=ORIENTED_EDGE ( 'NONE', *, *, #48085, .T. ) ;
#39059=CARTESIAN_POINT ( 'NONE',  ( -3.152801135295367096, -157.0625000013656063, -3.152801135295367541 ) ) ;
#39065=CARTESIAN_POINT ( 'NONE',  ( -4.458734124999998549, -42.47916666530107932, 2.574251347313722516 ) ) ;
#39066=ORIENTED_EDGE ( 'NONE', *, *, #51943, .F. ) ;
#39072=CARTESIAN_POINT ( 'NONE',  ( 9.457646018065525792E-16, 27.93750000136559208, 5.148502694627439702 ) ) ;
#39074=CARTESIAN_POINT ( 'NONE',  ( -5.000000000000000000, 25.04166666939785202, -2.886751345948128211 ) ) ;
#39078=CARTESIAN_POINT ( 'NONE',  ( 1.975475456537005874E-15, 10.37500000273118417, 5.000000000000000000 ) ) ;
#39080=EDGE_CURVE ( 'NONE', #25339, #44494, #21576, .T. ) ;
#39083=CARTESIAN_POINT ( 'NONE',  ( 0.000000000000000000, -170.0000000000000000, 0.000000000000000000 ) ) ;
#39084=CARTESIAN_POINT ( 'NONE',  ( -3.152548672688508926E-16, -87.81249999863439371, -5.148502694627439702 ) ) ;
#39088=CARTESIAN_POINT ( 'NONE',  ( -2.500000000000000444, -17.04166666393548368, -4.330127018922193649 ) ) ;
#39090=CARTESIAN_POINT ( 'NONE',  ( 5.000000000000000000, -163.1875000027312410, 2.071067811865478614 ) ) ;
#39092=VECTOR ( 'NONE', #45783, 1000.000000000000000 ) ;
#39093=CARTESIAN_POINT ( 'NONE',  ( 1.339745962155612702, -49.16965819600731891, -5.000000000000000000 ) ) ;
#39102=CARTESIAN_POINT ( 'NONE',  ( 5.000000000000000000, -48.37499999726880873, -6.123233995736766282E-16 ) ) ;
#39103=CARTESIAN_POINT ( 'NONE',  ( -4.458734124999999437, -12.31249999863440259, 0.000000000000000000 ) ) ;
#39104=CARTESIAN_POINT ( 'NONE',  ( 1.975475456537005874E-15, -21.75000000000000000, 5.000000000000000000 ) ) ;
#39105=CARTESIAN_POINT ( 'NONE',  ( 5.000000000000000888, -156.9375000000000284, -2.071067811865475505 ) ) ;
#39108=CARTESIAN_POINT ( 'NONE',  ( -2.229367062500000163, -41.72916666530107932, -3.861377020970580443 ) ) ;
#39109=LINE ( 'NONE', #18858, #4759 ) ;
#39114=CARTESIAN_POINT ( 'NONE',  ( -2.229367062500000163, 11.52083333469892601, -3.861377020970580443 ) ) ;
#39117=CARTESIAN_POINT ( 'NONE',  ( -4.458734124999999437, -87.64583333196773651, -2.574251347313719407 ) ) ;
#39118=CARTESIAN_POINT ( 'NONE',  ( 4.458734125000001214, 22.85416666803225993, 2.574251347313718519 ) ) ;
#39120=CARTESIAN_POINT ( 'NONE',  ( -5.000000000000000000, 14.04166666939785202, -2.886751345948128211 ) ) ;
#39121=ORIENTED_EDGE ( 'NONE', *, *, #11395, .T. ) ;
#39122=CARTESIAN_POINT ( 'NONE',  ( -6.972266317189433020E-16, -7.124999997268814056, -5.000000000000000000 ) ) ;
#39123=VERTEX_POINT ( 'NONE', #3964 ) ;
#39125=LINE ( 'NONE', #44588, #17267 ) ;
#39126=CARTESIAN_POINT ( 'NONE',  ( -2.500000000000000444, -34.16666666666666430, -4.330127018922193649 ) ) ;
#39127=CARTESIAN_POINT ( 'NONE',  ( 4.458734124999998549, -38.72916666530106511, -2.574251347313721627 ) ) ;
#39128=CARTESIAN_POINT ( 'NONE',  ( -4.999999999999999112, -33.79166666393547303, 2.886751345948131764 ) ) ;
#39129=CARTESIAN_POINT ( 'NONE',  ( 4.458734124999999437, -63.81249999863440792, -5.460374474430324690E-16 ) ) ;
#39130=ORIENTED_EDGE ( 'NONE', *, *, #36172, .T. ) ;
#39132=CARTESIAN_POINT ( 'NONE',  ( 4.458734125000001214, -13.89583333196774007, 2.574251347313718519 ) ) ;
#39133=CARTESIAN_POINT ( 'NONE',  ( 4.458734125000001214, -16.14583333196773651, 2.574251347313718519 ) ) ;
#39134=EDGE_LOOP ( 'NONE', ( #1509, #19757, #54146, #36230 ) ) ;
#39135=CARTESIAN_POINT ( 'NONE',  ( 2.499999999999998668, -80.33333333333332860, -4.330127018922193649 ) ) ;
#39138=CARTESIAN_POINT ( 'NONE',  ( 5.000000000000000000, -81.37499999726881583, -6.123233995736766282E-16 ) ) ;
#39139=CARTESIAN_POINT ( 'NONE',  ( -1.049326080737009628E-13, -17.75000000000000355, 5.000000000000000000 ) ) ;
#39140=ORIENTED_EDGE ( 'NONE', *, *, #2339, .T. ) ;
#39141=VECTOR ( 'NONE', #26739, 1000.000000000000000 ) ;
#39143=CARTESIAN_POINT ( 'NONE',  ( -2.229367062500000163, -25.72916666530106866, -3.861377020970580443 ) ) ;
#39145=CARTESIAN_POINT ( 'NONE',  ( 1.846868145590735200, -165.5000000013655779, -4.458734125000000326 ) ) ;
#39148=VERTEX_POINT ( 'NONE', #43180 ) ;
#39153=CARTESIAN_POINT ( 'NONE',  ( 4.458734124999997661, -144.7500000013655779, 1.846868145590737864 ) ) ;
#39154=FACE_OUTER_BOUND ( 'NONE', #10182, .T. ) ;
#39159=CARTESIAN_POINT ( 'NONE',  ( 3.152801135295366208, -143.8125000013655779, 3.152801135295367985 ) ) ;
#39164=CARTESIAN_POINT ( 'NONE',  ( 2.229367062500001939, -67.22916666530106511, 3.861377020970579999 ) ) ;
#39166=CARTESIAN_POINT ( 'NONE',  ( 5.000000000000000000, -54.29166666393549434, -2.886751345948130876 ) ) ;
#39175=CARTESIAN_POINT ( 'NONE',  ( -4.458734124999997661, 25.52083333469892423, 2.574251347313722516 ) ) ;
#39176=CARTESIAN_POINT ( 'NONE',  ( 2.500000000000002220, -18.66666666666666430, 4.330127018922192761 ) ) ;
#39181=CARTESIAN_POINT ( 'NONE',  ( -1.339745962155613812, -51.08034179853027723, -5.000000000000000000 ) ) ;
#39182=CARTESIAN_POINT ( 'NONE',  ( -2.229367062500000163, 0.5208333346989266754, -3.861377020970580443 ) ) ;
#39184=CARTESIAN_POINT ( 'NONE',  ( -4.458734124999999437, -23.64583333196773651, -2.574251347313719407 ) ) ;
#39185=AXIS2_PLACEMENT_3D ( 'NONE', #44386, #4841, #44066 ) ;
#39189=CARTESIAN_POINT ( 'NONE',  ( 2.229367062499998831, 25.35416666803225993, -3.861377020970580887 ) ) ;
#39191=CARTESIAN_POINT ( 'NONE',  ( 6.123233995736766282E-16, -170.0000000000000000, -5.000000000000000000 ) ) ;
#39192=CARTESIAN_POINT ( 'NONE',  ( -3.152548672688508926E-16, -71.81249999863439371, -5.148502694627439702 ) ) ;
#39195=CARTESIAN_POINT ( 'NONE',  ( -2.499999999999996447, 28.29166666939785202, 4.330127018922195425 ) ) ;
#39198=CARTESIAN_POINT ( 'NONE',  ( 5.000000000000000888, -16.58333333333333215, 2.886751345948126879 ) ) ;
#39199=CARTESIAN_POINT ( 'NONE',  ( -2.229367062499996610, -24.14583333196773651, 3.861377020970582219 ) ) ;
#39200=CARTESIAN_POINT ( 'NONE',  ( -3.152548672688508926E-16, -84.56249999863439371, -5.148502694627439702 ) ) ;
#39202=CARTESIAN_POINT ( 'NONE',  ( -1.846868145590737420, -168.0000000013655779, 4.458734124999999437 ) ) ;
#39204=CARTESIAN_POINT ( 'NONE',  ( 2.500000000000002220, -18.54166666393547658, 4.330127018922192761 ) ) ;
#39205=CARTESIAN_POINT ( 'NONE',  ( -4.458734124999999437, -48.31249999863440792, 0.000000000000000000 ) ) ;
#39206=ORIENTED_EDGE ( 'NONE', *, *, #24500, .T. ) ;
#39209=CARTESIAN_POINT ( 'NONE',  ( -4.458734124999999437, 2.437500001365593860, 0.000000000000000000 ) ) ;
#39210=VERTEX_POINT ( 'NONE', #59310 ) ;
#39212=CARTESIAN_POINT ( 'NONE',  ( -5.000000000000000000, -68.99999999999998579, 0.000000000000000000 ) ) ;
#39213=CARTESIAN_POINT ( 'NONE',  ( 1.846868145590735200, -154.5000000013656347, -4.458734125000000326 ) ) ;
#39215=DIRECTION ( 'NONE',  ( -0.000000000000000000, 1.000000000000000000, -0.000000000000000000 ) ) ;
#39216=CARTESIAN_POINT ( 'NONE',  ( -5.000000000000000888, -160.4375000000000568, 2.071067811865474617 ) ) ;
#39217=CARTESIAN_POINT ( 'NONE',  ( 1.975475456537005874E-15, -51.62499999726880873, 5.000000000000000000 ) ) ;
#39219=CARTESIAN_POINT ( 'NONE',  ( -4.458734124999999437, -10.56249999863440792, 0.000000000000000000 ) ) ;
#39220=CARTESIAN_POINT ( 'NONE',  ( 4.458734124999998549, -48.97916666530107221, -2.574251347313721627 ) ) ;
#39222=DIRECTION ( 'NONE',  ( 0.000000000000000000, 0.000000000000000000, 1.000000000000000000 ) ) ;
#39223=CARTESIAN_POINT ( 'NONE',  ( 4.458734124999999437, -148.4375000013656063, 0.000000000000000000 ) ) ;
#39228=CARTESIAN_POINT ( 'NONE',  ( -5.000000000000000000, -5.874999997268811391, 0.000000000000000000 ) ) ;
#39230=CARTESIAN_POINT ( 'NONE',  ( 5.000000000000000000, -29.37499999726881228, -6.123233995736766282E-16 ) ) ;
#39231=VERTEX_POINT ( 'NONE', #49972 ) ;
#39235=CARTESIAN_POINT ( 'NONE',  ( -2.229367062500000163, -2.479166665301069106, -3.861377020970580443 ) ) ;
#39236=LINE ( 'NONE', #10609, #30565 ) ;
#39237=CARTESIAN_POINT ( 'NONE',  ( -4.458734125000000326, -153.8750000013655779, 1.846868145590734089 ) ) ;
#39239=VERTEX_POINT ( 'NONE', #29071 ) ;
#39242=CARTESIAN_POINT ( 'NONE',  ( 5.000000000000000000, -12.29166666393547835, -2.886751345948130876 ) ) ;
#39245=CARTESIAN_POINT ( 'NONE',  ( 5.000000000000000000, 29.50000000000000000, -6.123233995736766282E-16 ) ) ;
#39252=CARTESIAN_POINT ( 'NONE',  ( 4.458734124999998549, 16.27083333469892779, -2.574251347313721627 ) ) ;
#39254=VERTEX_POINT ( 'NONE', #44186 ) ;
#39255=CARTESIAN_POINT ( 'NONE',  ( -2.229367062500000163, -10.72916666530106866, -3.861377020970580443 ) ) ;
#39258=CARTESIAN_POINT ( 'NONE',  ( -4.458734124999999437, -167.9375000013655779, -5.460374474430324690E-16 ) ) ;
#39259=CARTESIAN_POINT ( 'NONE',  ( 5.000000000000000888, -88.58333333333332860, 2.886751345948126879 ) ) ;
#39262=EDGE_CURVE ( 'NONE', #17113, #49521, #58990, .T. ) ;
#39266=CARTESIAN_POINT ( 'NONE',  ( 3.152801135295366208, -151.8125000013655779, 3.152801135295367985 ) ) ;
#39268=CARTESIAN_POINT ( 'NONE',  ( 2.500000000000002220, -46.66666666666666430, 4.330127018922192761 ) ) ;
#39270=VERTEX_POINT ( 'NONE', #39995 ) ;
#39273=( BOUNDED_CURVE ( )  B_SPLINE_CURVE ( 2, ( #17830, #6681, #26288, #8189, #3681, #23295, #40758, #27791, #35952 ),
 .UNSPECIFIED., .F., .F. ) 
 B_SPLINE_CURVE_WITH_KNOTS ( ( 3, 2, 2, 2, 3 ),
 ( 0.8854166666666666297, 0.8861111111111110716, 0.8874999999999999556, 0.8888888888888888395, 0.8895833333333332815 ),
 .UNSPECIFIED. ) 
 CURVE ( )  GEOMETRIC_REPRESENTATION_ITEM ( )  RATIONAL_B_SPLINE_CURVE ( ( 0.9330127018922194093, 0.9330127018922194093, 1.000000000000000000, 0.8660254037844387076, 1.000000000000000000, 0.8660254037844387076, 1.000000000000000000, 0.9330127018922194093, 0.9330127018922194093 ) ) 
 REPRESENTATION_ITEM ( '' )  );
#39274=DIRECTION ( 'NONE',  ( -0.000000000000000000, 1.000000000000000000, -0.000000000000000000 ) ) ;
#39275=CARTESIAN_POINT ( 'NONE',  ( 5.000000000000000000, -0.5000000000000004441, -6.123233995736766282E-16 ) ) ;
#39276=ADVANCED_FACE ( 'NONE', ( #20070 ), #58364, .T. ) ;
#39277=CARTESIAN_POINT ( 'NONE',  ( 2.229367062500001939, -68.97916666530107932, 3.861377020970579999 ) ) ;
#39278=LINE ( 'NONE', #34447, #39009 ) ;
#39279=CARTESIAN_POINT ( 'NONE',  ( -3.535250795749689387E-16, -0.1249999972688133065, -5.773502691896257311 ) ) ;
#39280=CARTESIAN_POINT ( 'NONE',  ( 2.229367062499998831, -31.64583333196773651, -3.861377020970580887 ) ) ;
#39283=FACE_OUTER_BOUND ( 'NONE', #54819, .T. ) ;
#39285=DIRECTION ( 'NONE',  ( -0.000000000000000000, 1.000000000000000000, -0.000000000000000000 ) ) ;
#39286=CARTESIAN_POINT ( 'NONE',  ( 5.000000000000000000, -43.50000000000000000, -6.123233995736766282E-16 ) ) ;
#39287=DIRECTION ( 'NONE',  ( -0.000000000000000000, 1.000000000000000000, -0.000000000000000000 ) ) ;
#39290=CARTESIAN_POINT ( 'NONE',  ( 2.229367062500001939, -71.97916666530107932, 3.861377020970579999 ) ) ;
#39291=CARTESIAN_POINT ( 'NONE',  ( 2.730187237215162345E-16, -143.4375000013656063, -4.458734124999999437 ) ) ;
#39292=CARTESIAN_POINT ( 'NONE',  ( 4.458734124999998549, -80.72916666530106511, -2.574251347313721627 ) ) ;
#39294=CARTESIAN_POINT ( 'NONE',  ( 2.229367062500001939, -29.22916666530107221, 3.861377020970579999 ) ) ;
#39295=CARTESIAN_POINT ( 'NONE',  ( 1.060575238724906964E-15, -73.62499999726881583, 5.773502691896257311 ) ) ;
#39296=ORIENTED_EDGE ( 'NONE', *, *, #60597, .T. ) ;
#39300=CARTESIAN_POINT ( 'NONE',  ( -1.127183054612291972E-14, 22.37500000273118417, 4.999999999999999112 ) ) ;
#39306=CARTESIAN_POINT ( 'NONE',  ( -2.229367062499996610, -59.39583333196773651, 3.861377020970582219 ) ) ;
#39309=CARTESIAN_POINT ( 'NONE',  ( 3.535533905932736864, -142.1250000000000000, 3.535533905932738641 ) ) ;
#39311=CARTESIAN_POINT ( 'NONE',  ( 4.458734125000001214, 12.10416666803226171, 2.574251347313718519 ) ) ;
#39313=CARTESIAN_POINT ( 'NONE',  ( 3.152801135295366208, -164.5625000013656063, 3.152801135295367985 ) ) ;
#39316=CARTESIAN_POINT ( 'NONE',  ( -1.339745962155613812, -52.08034179853028434, -5.000000000000000000 ) ) ;
#39319=CARTESIAN_POINT ( 'NONE',  ( 0.000000000000000000, -170.0000000000000000, 0.000000000000000000 ) ) ;
#39324=FACE_OUTER_BOUND ( 'NONE', #46494, .T. ) ;
#39325=CARTESIAN_POINT ( 'NONE',  ( 1.339745962155612702, -58.29465819873852439, -5.000000000000000000 ) ) ;
#39328=CARTESIAN_POINT ( 'NONE',  ( -2.229367062499996610, 6.604166668032259935, 3.861377020970582219 ) ) ;
#39329=CARTESIAN_POINT ( 'NONE',  ( -9.184850993605147944E-16, -146.3750000027312126, 5.000000000000000000 ) ) ;
#39331=CARTESIAN_POINT ( 'NONE',  ( -5.000000000000000000, -148.6250000027312126, -6.123233995736766282E-16 ) ) ;
#39332=CARTESIAN_POINT ( 'NONE',  ( 6.123233995736766282E-16, -170.0000000000000000, -5.000000000000000000 ) ) ;
#39336=CARTESIAN_POINT ( 'NONE',  ( 5.000000000000000000, -144.0625000000000284, 2.071067811865478614 ) ) ;
#39338=EDGE_CURVE ( 'NONE', #23654, #29728, #34704, .T. ) ;
#39342=CARTESIAN_POINT ( 'NONE',  ( 1.846868145590735200, -164.5000000013655779, -4.458734124999999437 ) ) ;
#39343=CARTESIAN_POINT ( 'NONE',  ( 9.457646018065525792E-16, -35.06249999863440792, 5.148502694627439702 ) ) ;
#39345=CARTESIAN_POINT ( 'NONE',  ( 3.061616997868383141E-16, -160.7500000000000000, -5.000000000000000000 ) ) ;
#39346=CARTESIAN_POINT ( 'NONE',  ( -6.972266317189433020E-16, 7.750000000000000000, -5.000000000000000000 ) ) ;
#39348=CARTESIAN_POINT ( 'NONE',  ( 2.730187237215162345E-16, -142.1875000013656063, -4.458734124999999437 ) ) ;
#39349=ORIENTED_EDGE ( 'NONE', *, *, #28053, .T. ) ;
#39350=CARTESIAN_POINT ( 'NONE',  ( -4.458734124999999437, 28.43750000136559208, 0.000000000000000000 ) ) ;
#39352=CARTESIAN_POINT ( 'NONE',  ( 4.458734124999998549, -61.97916666530106511, -2.574251347313721627 ) ) ;
#39354=CARTESIAN_POINT ( 'NONE',  ( 5.000000000000000888, 16.41666666666666785, 2.886751345948126879 ) ) ;
#39356=CARTESIAN_POINT ( 'NONE',  ( 4.458734125000000326, -52.89583333196772941, 2.574251347313718519 ) ) ;
#39357=CARTESIAN_POINT ( 'NONE',  ( 4.458734124999998549, -6.729166665301073103, -2.574251347313721627 ) ) ;
#39359=EDGE_CURVE ( 'NONE', #733, #22693, #1483, .T. ) ;
#39361=CARTESIAN_POINT ( 'NONE',  ( 5.000000000000000000, 0.5000000000000004441, -6.123233995736766282E-16 ) ) ;
#39363=DIRECTION ( 'NONE',  ( 0.000000000000000000, 1.000000000000000000, 0.000000000000000000 ) ) ;
#39364=CARTESIAN_POINT ( 'NONE',  ( -4.458734124999999437, -53.39583333196773651, -2.574251347313719407 ) ) ;
#39365=CARTESIAN_POINT ( 'NONE',  ( -1.846868145590734756, -156.3750000013655779, -4.458734125000000326 ) ) ;
#39367=CARTESIAN_POINT ( 'NONE',  ( 5.000000000000000000, -54.29166666393549434, -2.886751345948129988 ) ) ;
#39369=CARTESIAN_POINT ( 'NONE',  ( 3.061616997868383141E-16, -142.7500000000000284, -5.000000000000000000 ) ) ;
#39370=CARTESIAN_POINT ( 'NONE',  ( 4.458734125000001214, 6.854166668032259935, 2.574251347313718519 ) ) ;
#39372=CARTESIAN_POINT ( 'NONE',  ( -6.972266317189433020E-16, -56.25000000000000000, -5.000000000000000000 ) ) ;
#39374=CARTESIAN_POINT ( 'NONE',  ( 3.152801135295367541, -155.3125000013656063, -3.152801135295367541 ) ) ;
#39378=CARTESIAN_POINT ( 'NONE',  ( -2.499999999999996447, -58.70833333060214443, 4.330127018922195425 ) ) ;
#39379=CARTESIAN_POINT ( 'NONE',  ( -4.458734124999999437, -42.56249999863440081, 0.000000000000000000 ) ) ;
#39380=VERTEX_POINT ( 'NONE', #55452 ) ;
#39381=AXIS2_PLACEMENT_3D ( 'NONE', #32125, #26356, #36330 ) ;
#39384=ORIENTED_EDGE ( 'NONE', *, *, #58518, .F. ) ;
#39385=CARTESIAN_POINT ( 'NONE',  ( -4.458734124999999437, -89.64583333196773651, -2.574251347313719407 ) ) ;
#39388=CARTESIAN_POINT ( 'NONE',  ( -5.000000000000000000, -7.083333333333330373, -2.886751345948128211 ) ) ;
#39389=CARTESIAN_POINT ( 'NONE',  ( 5.000000000000000888, -52.45833333060213732, 2.886751345948126879 ) ) ;
#39392=( BOUNDED_CURVE ( )  B_SPLINE_CURVE ( 2, ( #42199, #23540, #28349, #38324, #53117, #8434, #28662, #9360, #47966 ),
 .UNSPECIFIED., .F., .F. ) 
 B_SPLINE_CURVE_WITH_KNOTS ( ( 3, 2, 2, 2, 3 ),
 ( 0.7729166666666666963, 0.7736111111111111382, 0.7750000000000000222, 0.7763888888888889062, 0.7770833333333333481 ),
 .UNSPECIFIED. ) 
 CURVE ( )  GEOMETRIC_REPRESENTATION_ITEM ( )  RATIONAL_B_SPLINE_CURVE ( ( 0.9330127018922194093, 0.9330127018922194093, 1.000000000000000000, 0.8660254037844387076, 1.000000000000000000, 0.8660254037844387076, 1.000000000000000000, 0.9330127018922194093, 0.9330127018922194093 ) ) 
 REPRESENTATION_ITEM ( '' )  );
#39393=DIRECTION ( 'NONE',  ( 0.000000000000000000, 0.000000000000000000, 1.000000000000000000 ) ) ;
#39396=CARTESIAN_POINT ( 'NONE',  ( -1.339745962155610925, -66.66965819600733312, 5.000000000000000000 ) ) ;
#39403=CARTESIAN_POINT ( 'NONE',  ( -5.000000000000000888, -162.5625000027312126, 2.071067811865474617 ) ) ;
#39415=CARTESIAN_POINT ( 'NONE',  ( -3.152548672688508926E-16, -16.56249999863440436, -5.148502694627439702 ) ) ;
#39417=CARTESIAN_POINT ( 'NONE',  ( 5.000000000000000888, -153.9375000000000000, -2.071067811865475505 ) ) ;
#39419=ORIENTED_EDGE ( 'NONE', *, *, #59779, .T. ) ;
#39420=CARTESIAN_POINT ( 'NONE',  ( -2.229367062500000163, -48.72916666530106511, -3.861377020970580443 ) ) ;
#39426=CARTESIAN_POINT ( 'NONE',  ( -2.229367062500000163, 10.52083333469892779, -3.861377020970580443 ) ) ;
#39428=CARTESIAN_POINT ( 'NONE',  ( 5.000000000000000888, -37.45833333060213732, 2.886751345948126879 ) ) ;
#39430=CARTESIAN_POINT ( 'NONE',  ( -3.152548672688508926E-16, 20.18750000136559208, -5.148502694627439702 ) ) ;
#39432=CARTESIAN_POINT ( 'NONE',  ( 2.500000000000002220, 8.458333336064518093, 4.330127018922192761 ) ) ;
#39439=CARTESIAN_POINT ( 'NONE',  ( -3.535250795749689387E-16, -32.25000000000000000, -5.773502691896257311 ) ) ;
#39440=CARTESIAN_POINT ( 'NONE',  ( -4.458734124999999437, -40.31249999863440081, 0.000000000000000000 ) ) ;
#39441=EDGE_CURVE ( 'NONE', #1762, #3107, #37175, .T. ) ;
#39442=EDGE_CURVE ( 'NONE', #28553, #40991, #3912, .T. ) ;
#39443=CARTESIAN_POINT ( 'NONE',  ( 5.000000000000000888, -34.45833333060213732, 2.886751345948126879 ) ) ;
#39444=CARTESIAN_POINT ( 'NONE',  ( -4.458734124999999437, -66.31249999863440792, 0.000000000000000000 ) ) ;
#39447=CARTESIAN_POINT ( 'NONE',  ( -4.458734124999998549, -11.22916666530106866, 2.574251347313722516 ) ) ;
#39448=CARTESIAN_POINT ( 'NONE',  ( -3.152548672688508926E-16, -12.81249999863440259, -5.148502694627439702 ) ) ;
#39450=( BOUNDED_CURVE ( )  B_SPLINE_CURVE ( 2, ( #17960, #61100, #55951, #2878, #56590, #22809, #32443, #31810, #51445 ),
 .UNSPECIFIED., .F., .F. ) 
 B_SPLINE_CURVE_WITH_KNOTS ( ( 3, 2, 2, 2, 3 ),
 ( 0.6916666666666663188, 0.6958333333333329707, 0.6999999999999995115, 0.7041666666666662744, 0.7083333333333329263 ),
 .UNSPECIFIED. ) 
 CURVE ( )  GEOMETRIC_REPRESENTATION_ITEM ( )  RATIONAL_B_SPLINE_CURVE ( ( 1.000000000000005995, 0.9238795325112806323, 1.000000000000000000, 0.9238795325112867385, 1.000000000000000000, 0.9238795325112867385, 1.000000000000000000, 0.9238795325112948431, 0.9999999999999918954 ) ) 
 REPRESENTATION_ITEM ( '' )  );
#39451=CARTESIAN_POINT ( 'NONE',  ( -3.535250795749689387E-16, -82.25000000000000000, -5.773502691896257311 ) ) ;
#39452=CARTESIAN_POINT ( 'NONE',  ( -1.339745962155613812, 0.9196582014697067819, -5.000000000000000000 ) ) ;
#39455=CARTESIAN_POINT ( 'NONE',  ( 2.499999999999998668, -82.20833333060214443, -4.330127018922193649 ) ) ;
#39456=CARTESIAN_POINT ( 'NONE',  ( 6.123233995736766282E-16, -170.0000000000000000, -5.000000000000000000 ) ) ;
#39459=CARTESIAN_POINT ( 'NONE',  ( 4.458734124999998549, -28.97916666530107577, -2.574251347313721627 ) ) ;
#39461=EDGE_LOOP ( 'NONE', ( #37567, #43809, #51360, #45950 ) ) ;
#39462=CARTESIAN_POINT ( 'NONE',  ( 2.730187237215162345E-16, -164.4375000013655779, -4.458734124999999437 ) ) ;
#39464=CARTESIAN_POINT ( 'NONE',  ( 2.071067811865349828, -148.1874999999999716, 5.000000000000126121 ) ) ;
#39469=CARTESIAN_POINT ( 'NONE',  ( 3.152801135295366208, -145.8125000013655779, 3.152801135295367985 ) ) ;
#39470=DIRECTION ( 'NONE',  ( -0.000000000000000000, 1.000000000000000000, -0.000000000000000000 ) ) ;
#39475=VECTOR ( 'NONE', #6893, 1000.000000000000000 ) ;
#39476=CARTESIAN_POINT ( 'NONE',  ( 3.152801135295366208, -139.8125000013655779, 3.152801135295367985 ) ) ;
#39479=CARTESIAN_POINT ( 'NONE',  ( 0.000000000000000000, -170.0000000000000000, 0.000000000000000000 ) ) ;
#39481=CARTESIAN_POINT ( 'NONE',  ( -4.458734124999998549, -72.47916666530107932, 2.574251347313722516 ) ) ;
#39483=CARTESIAN_POINT ( 'NONE',  ( -4.999999999999998224, -69.91666666666667140, 2.886751345948131764 ) ) ;
#39487=CARTESIAN_POINT ( 'NONE',  ( -1.339745962155613812, -71.08034179853027013, -5.000000000000000000 ) ) ;
#39493=CARTESIAN_POINT ( 'NONE',  ( 4.458734124999998549, 16.02083333469892779, -2.574251347313721627 ) ) ;
#39494=DIRECTION ( 'NONE',  ( 0.000000000000000000, 0.000000000000000000, 1.000000000000000000 ) ) ;
#39499=CARTESIAN_POINT ( 'NONE',  ( -1.339745962155610925, -50.66965819600732601, 5.000000000000000000 ) ) ;
#39500=CARTESIAN_POINT ( 'NONE',  ( -4.458734124999999437, -0.3958333319677397322, -2.574251347313719407 ) ) ;
#39501=ORIENTED_EDGE ( 'NONE', *, *, #54619, .T. ) ;
#39502=CARTESIAN_POINT ( 'NONE',  ( 4.458734124999999437, -26.06249999863440792, -5.460374474430324690E-16 ) ) ;
#39506=CARTESIAN_POINT ( 'NONE',  ( -4.458734124999999437, 26.60416666803225993, -2.574251347313719407 ) ) ;
#39508=CARTESIAN_POINT ( 'NONE',  ( 0.000000000000000000, -170.0000000000000000, 5.000000000000000000 ) ) ;
#39509=CARTESIAN_POINT ( 'NONE',  ( 4.458734124999998549, -74.97916666530106511, -2.574251347313721627 ) ) ;
#39511=CARTESIAN_POINT ( 'NONE',  ( 5.000000000000000000, -73.50000000000000000, -6.123233995736766282E-16 ) ) ;
#39512=CARTESIAN_POINT ( 'NONE',  ( -5.000000000000000000, -10.95833333060214621, -2.886751345948128211 ) ) ;
#39513=ORIENTED_EDGE ( 'NONE', *, *, #55598, .F. ) ;
#39514=CARTESIAN_POINT ( 'NONE',  ( -2.500000000000000444, -57.04166666393548013, -4.330127018922193649 ) ) ;
#39515=CARTESIAN_POINT ( 'NONE',  ( -5.000000000000000000, -18.99999999999999645, 0.000000000000000000 ) ) ;
#39516=CARTESIAN_POINT ( 'NONE',  ( 9.457646018065525792E-16, -21.06249999863440436, 5.148502694627439702 ) ) ;
#39517=CARTESIAN_POINT ( 'NONE',  ( -2.229367062500000163, -82.47916666530106511, -3.861377020970580443 ) ) ;
#39518=AXIS2_PLACEMENT_3D ( 'NONE', #31157, #50139, #60766 ) ;
#39519=CARTESIAN_POINT ( 'NONE',  ( 1.846868145590735200, -167.5000000013655779, -4.458734125000000326 ) ) ;
#39520=CARTESIAN_POINT ( 'NONE',  ( 5.000000000000000000, -20.29166666393548368, -2.886751345948129988 ) ) ;
#39521=CARTESIAN_POINT ( 'NONE',  ( -2.229367062499996610, -49.14583333196772941, 3.861377020970582219 ) ) ;
#39522=ORIENTED_EDGE ( 'NONE', *, *, #46945, .T. ) ;
#39524=CARTESIAN_POINT ( 'NONE',  ( 2.229367062499998831, 3.104166668032259935, -3.861377020970580887 ) ) ;
#39527=CARTESIAN_POINT ( 'NONE',  ( 2.500000000000002220, -66.66666666666667140, 4.330127018922192761 ) ) ;
#39528=CARTESIAN_POINT ( 'NONE',  ( -4.458734124999999437, -154.1875000013656063, -5.460374474430324690E-16 ) ) ;
#39531=CARTESIAN_POINT ( 'NONE',  ( 3.061616997868383141E-16, -163.7500000000000000, -5.000000000000000000 ) ) ;
#39532=DIRECTION ( 'NONE',  ( -0.000000000000000000, 1.000000000000000000, -0.000000000000000000 ) ) ;
#39534=CARTESIAN_POINT ( 'NONE',  ( -2.229367062500000163, -11.72916666530107044, -3.861377020970580443 ) ) ;
#39535=CARTESIAN_POINT ( 'NONE',  ( -3.152548672688508926E-16, -43.81249999863440081, -5.148502694627439702 ) ) ;
#39537=CARTESIAN_POINT ( 'NONE',  ( -4.458734125000001214, -148.8750000013655495, 1.846868145590734089 ) ) ;
#39542=FACE_OUTER_BOUND ( 'NONE', #62062, .T. ) ;
#39545=ADVANCED_FACE ( 'NONE', ( #47684 ), #33216, .T. ) ;
#39546=ORIENTED_EDGE ( 'NONE', *, *, #48422, .F. ) ;
#39548=CYLINDRICAL_SURFACE ( 'NONE', #26569, 5.000000000000000000 ) ;
#39550=CARTESIAN_POINT ( 'NONE',  ( -5.000000000000000000, 9.000000000000001776, 0.000000000000000000 ) ) ;
#39551=CARTESIAN_POINT ( 'NONE',  ( -2.229367062500000163, -4.479166665301070438, -3.861377020970580443 ) ) ;
#39552=CARTESIAN_POINT ( 'NONE',  ( -6.972266317189433020E-16, -54.24999999999999289, -5.000000000000000000 ) ) ;
#39553=CARTESIAN_POINT ( 'NONE',  ( 3.152801135295367541, -148.3125000013655779, -3.152801135295367541 ) ) ;
#39560=CARTESIAN_POINT ( 'NONE',  ( -4.999999999999998224, 28.20833333606451987, 2.886751345948131764 ) ) ;
#39565=DIRECTION ( 'NONE',  ( -0.000000000000000000, 1.000000000000000000, -0.000000000000000000 ) ) ;
#39569=CARTESIAN_POINT ( 'NONE',  ( 9.457646018065525792E-16, 16.93750000136559564, 5.148502694627439702 ) ) ;
#39572=CARTESIAN_POINT ( 'NONE',  ( 4.458734125000000326, -10.14583333196773829, 2.574251347313718519 ) ) ;
#39573=CARTESIAN_POINT ( 'NONE',  ( 5.000000000000000888, -169.0625000027312126, -2.071067811865475505 ) ) ;
#39575=CARTESIAN_POINT ( 'NONE',  ( 4.458734124999999437, -169.4375000013656063, 0.000000000000000000 ) ) ;
#39576=CARTESIAN_POINT ( 'NONE',  ( -9.184850993605147944E-16, -154.3750000027311842, 5.000000000000000000 ) ) ;
#39582=CARTESIAN_POINT ( 'NONE',  ( 3.535533905932738197, -142.0000000027311842, -3.535533905932738197 ) ) ;
#39584=CARTESIAN_POINT ( 'NONE',  ( 2.730187237215162345E-16, -153.4375000013655779, -4.458734124999999437 ) ) ;
#39586=CARTESIAN_POINT ( 'NONE',  ( 2.788906526875773208E-15, 27.87500000273118772, -5.000000000000000000 ) ) ;
#39591=CARTESIAN_POINT ( 'NONE',  ( 1.975475456537005874E-15, -76.75000000000000000, 5.000000000000000000 ) ) ;
#39592=CARTESIAN_POINT ( 'NONE',  ( -5.000000000000000000, -3.000000000000002665, 0.000000000000000000 ) ) ;
#39593=CARTESIAN_POINT ( 'NONE',  ( -4.458734124999997661, -68.22916666530106511, 2.574251347313722516 ) ) ;
#39595=CARTESIAN_POINT ( 'NONE',  ( 5.000000000000000000, -0.2916666639354824619, -2.886751345948129988 ) ) ;
#39596=CARTESIAN_POINT ( 'NONE',  ( 4.458734125000001214, -31.89583333196773651, 2.574251347313718519 ) ) ;
#39597=ORIENTED_EDGE ( 'NONE', *, *, #60075, .F. ) ;
#39599=CARTESIAN_POINT ( 'NONE',  ( 3.535533905932736864, -157.1250000000000284, 3.535533905932738641 ) ) ;
#39600=VERTEX_POINT ( 'NONE', #52834 ) ;
#39601=LINE ( 'NONE', #38351, #44283 ) ;
#39602=CARTESIAN_POINT ( 'NONE',  ( -2.500000000000000444, -52.16666666666666430, -4.330127018922193649 ) ) ;
#39603=CARTESIAN_POINT ( 'NONE',  ( 5.000000000000000000, -17.29166666393548368, -2.886751345948130876 ) ) ;
#39605=CARTESIAN_POINT ( 'NONE',  ( -6.972266317189433020E-16, -4.249999999999997335, -5.000000000000000000 ) ) ;
#39606=CARTESIAN_POINT ( 'NONE',  ( 9.457646018065525792E-16, -72.06249999863439371, 5.148502694627439702 ) ) ;
#39607=CARTESIAN_POINT ( 'NONE',  ( 4.458734124999999437, -142.6875000013656063, 0.000000000000000000 ) ) ;
#39608=CARTESIAN_POINT ( 'NONE',  ( 4.458734124999999437, -82.81249999863440792, -5.460374474430324690E-16 ) ) ;
#39610=VECTOR ( 'NONE', #56914, 1000.000000000000000 ) ;
#39611=CARTESIAN_POINT ( 'NONE',  ( 2.229367062499998831, -27.89583333196774007, -3.861377020970580887 ) ) ;
#39612=CARTESIAN_POINT ( 'NONE',  ( -2.500000000000000444, -74.04166666393547303, -4.330127018922193649 ) ) ;
#39614=CARTESIAN_POINT ( 'NONE',  ( 0.000000000000000000, -170.0000000000000000, 5.000000000000000000 ) ) ;
#39615=EDGE_LOOP ( 'NONE', ( #30598, #51731, #62736, #45929 ) ) ;
#39617=ORIENTED_EDGE ( 'NONE', *, *, #58150, .F. ) ;
#39618=CARTESIAN_POINT ( 'NONE',  ( -5.000000000000000000, 17.00000000000000000, 0.000000000000000000 ) ) ;
#39619=CARTESIAN_POINT ( 'NONE',  ( 1.975475456537005874E-15, -12.74999999999999822, 5.000000000000000000 ) ) ;
#39620=CARTESIAN_POINT ( 'NONE',  ( -4.458734124999998549, -58.47916666530106511, 2.574251347313722516 ) ) ;
#39621=EDGE_CURVE ( 'NONE', #49284, #25405, #3635, .T. ) ;
#39624=CARTESIAN_POINT ( 'NONE',  ( 5.000000000000000000, -142.0625000000000000, 2.071067811865478614 ) ) ;
#39626=CARTESIAN_POINT ( 'NONE',  ( 2.229367062499998831, 14.35416666803226171, -3.861377020970580887 ) ) ;
#39628=CARTESIAN_POINT ( 'NONE',  ( 5.000000000000000888, -24.58333333333333215, 2.886751345948126879 ) ) ;
#39629=CARTESIAN_POINT ( 'NONE',  ( -4.458734124999999437, -159.9375000013655779, -5.460374474430324690E-16 ) ) ;
#39635=FACE_OUTER_BOUND ( 'NONE', #14780, .T. ) ;
#39638=ADVANCED_FACE ( 'NONE', ( #2686 ), #23246, .T. ) ;
#39644=CARTESIAN_POINT ( 'NONE',  ( 4.458734124999998549, 7.020833334698928674, -2.574251347313721627 ) ) ;
#39646=CARTESIAN_POINT ( 'NONE',  ( -2.500000000000000444, -10.04166666393547658, -4.330127018922193649 ) ) ;
#39648=CARTESIAN_POINT ( 'NONE',  ( 2.071067811865476394, -149.3125000027311842, 5.000000000000000000 ) ) ;
#39649=CARTESIAN_POINT ( 'NONE',  ( 0.000000000000000000, -170.0000000000000000, 5.000000000000000000 ) ) ;
#39654=CARTESIAN_POINT ( 'NONE',  ( -5.000000000000000888, -140.4375000000000000, 2.071067811865474617 ) ) ;
#39657=CARTESIAN_POINT ( 'NONE',  ( -4.458734124999999437, -165.2500000013655779, -1.846868145590735644 ) ) ;
#39661=CARTESIAN_POINT ( 'NONE',  ( -1.846868145590734756, -145.1250000013655779, -4.458734125000000326 ) ) ;
#39662=ORIENTED_EDGE ( 'NONE', *, *, #58551, .T. ) ;
#39663=CARTESIAN_POINT ( 'NONE',  ( 2.229367062500001939, 28.77083333469892779, 3.861377020970579999 ) ) ;
#39665=CARTESIAN_POINT ( 'NONE',  ( -4.458734124999999437, -63.64583333196773651, -2.574251347313719407 ) ) ;
#39667=CARTESIAN_POINT ( 'NONE',  ( 5.000000000000000888, -90.45833333060214443, 2.886751345948126879 ) ) ;
#39668=CARTESIAN_POINT ( 'NONE',  ( 5.000000000000000000, 15.58333333333333215, -2.886751345948129988 ) ) ;
#39669=CARTESIAN_POINT ( 'NONE',  ( 4.458734125000000326, -51.89583333196773651, 2.574251347313718519 ) ) ;
#39670=CARTESIAN_POINT ( 'NONE',  ( -4.458734124999999437, -5.312499998634402587, 0.000000000000000000 ) ) ;
#39671=CARTESIAN_POINT ( 'NONE',  ( -3.535533905932737309, -168.6250000000000284, -3.535533905932738197 ) ) ;
#39673=CARTESIAN_POINT ( 'NONE',  ( -6.972266317189433020E-16, -9.250000000000000000, -5.000000000000000000 ) ) ;
#39677=DIRECTION ( 'NONE',  ( -0.000000000000000000, 1.000000000000000000, -0.000000000000000000 ) ) ;
#39679=CARTESIAN_POINT ( 'NONE',  ( -5.000000000000000000, -31.95833333060214443, -2.886751345948128211 ) ) ;
#39680=CARTESIAN_POINT ( 'NONE',  ( 2.229367062499998831, -54.64583333196773651, -3.861377020970580887 ) ) ;
#39681=CARTESIAN_POINT ( 'NONE',  ( 4.458734124999999437, -154.7500000013656063, 1.846868145590737864 ) ) ;
#39682=CARTESIAN_POINT ( 'NONE',  ( 2.499999999999998668, -54.20833333060213732, -4.330127018922193649 ) ) ;
#39683=EDGE_LOOP ( 'NONE', ( #24209, #27664, #19689, #3286 ) ) ;
#39684=CARTESIAN_POINT ( 'NONE',  ( 1.975475456537005874E-15, -26.74999999999999645, 5.000000000000000000 ) ) ;
#39685=CARTESIAN_POINT ( 'NONE',  ( 4.458734124999999437, 3.937500001365595192, -5.460374474430324690E-16 ) ) ;
#39686=ORIENTED_EDGE ( 'NONE', *, *, #32676, .F. ) ;
#39688=CARTESIAN_POINT ( 'NONE',  ( -8.190561711645485556E-16, -155.6875000013655779, 4.458734124999999437 ) ) ;
#39694=CARTESIAN_POINT ( 'NONE',  ( -2.229367062499996610, -43.39583333196773651, 3.861377020970582219 ) ) ;
#39697=EDGE_CURVE ( 'NONE', #41789, #2557, #58566, .T. ) ;
#39701=CARTESIAN_POINT ( 'NONE',  ( 4.458734124999999437, -90.06249999863440792, -5.460374474430324690E-16 ) ) ;
#39703=CARTESIAN_POINT ( 'NONE',  ( -2.071067811865415109, -165.3125000000000284, 5.000000000000062172 ) ) ;
#39709=EDGE_CURVE ( 'NONE', #59564, #46451, #30573, .T. ) ;
#39714=EDGE_CURVE ( 'NONE', #60346, #32427, #10847, .T. ) ;
#39715=CARTESIAN_POINT ( 'NONE',  ( 0.000000000000000000, -170.0000000000000000, 5.000000000000000000 ) ) ;
#39717=CARTESIAN_POINT ( 'NONE',  ( -1.339745962155610925, 11.33034180399266511, 5.000000000000000000 ) ) ;
#39720=CARTESIAN_POINT ( 'NONE',  ( 5.000000000000000888, -31.58333333333333215, 2.886751345948126879 ) ) ;
#39722=CARTESIAN_POINT ( 'NONE',  ( -2.071067811865475061, -161.8125000027311842, -5.000000000000000888 ) ) ;
#39732=CARTESIAN_POINT ( 'NONE',  ( 2.229367062499998831, -19.64583333196774007, -3.861377020970580887 ) ) ;
#39733=CARTESIAN_POINT ( 'NONE',  ( -2.500000000000000444, -80.04166666393547303, -4.330127018922193649 ) ) ;
#39734=CARTESIAN_POINT ( 'NONE',  ( -3.535533905932737309, -154.6250000000000000, -3.535533905932738197 ) ) ;
#39736=CARTESIAN_POINT ( 'NONE',  ( -4.458734124999999437, -156.9375000013655779, -5.460374474430324690E-16 ) ) ;
#39737=ORIENTED_EDGE ( 'NONE', *, *, #18620, .F. ) ;
#39738=CARTESIAN_POINT ( 'NONE',  ( -3.152548672688508926E-16, -44.81249999863439371, -5.148502694627439702 ) ) ;
#39739=CARTESIAN_POINT ( 'NONE',  ( -1.339745962155564296, -12.20534180126147916, -5.000000000000028422 ) ) ;
#39740=CARTESIAN_POINT ( 'NONE',  ( -4.458734124999998549, -89.22916666530106511, 2.574251347313722516 ) ) ;
#39743=CARTESIAN_POINT ( 'NONE',  ( 9.457646018065525792E-16, 9.937500001365592084, 5.148502694627439702 ) ) ;
#39745=CARTESIAN_POINT ( 'NONE',  ( -5.000000000000000000, -69.08333333333332860, -2.886751345948128211 ) ) ;
#39747=CARTESIAN_POINT ( 'NONE',  ( 2.229367062499998831, 21.10416666803226349, -3.861377020970580887 ) ) ;
#39749=CARTESIAN_POINT ( 'NONE',  ( 5.000000000000000888, 6.541666669397851130, 2.886751345948126879 ) ) ;
#39751=VERTEX_POINT ( 'NONE', #707 ) ;
#39752=CARTESIAN_POINT ( 'NONE',  ( 2.499999999999998668, -85.33333333333332860, -4.330127018922193649 ) ) ;
#39753=CARTESIAN_POINT ( 'NONE',  ( 4.458734124999999437, -37.81249999863440792, -5.460374474430324690E-16 ) ) ;
#39755=CARTESIAN_POINT ( 'NONE',  ( -4.999999999999999112, -40.79166666393548724, 2.886751345948131764 ) ) ;
#39758=CARTESIAN_POINT ( 'NONE',  ( -3.152548672688508926E-16, -13.56249999863440259, -5.148502694627439702 ) ) ;
#39759=CARTESIAN_POINT ( 'NONE',  ( -2.229367062500000163, -13.72916666530107221, -3.861377020970580443 ) ) ;
#39760=ORIENTED_EDGE ( 'NONE', *, *, #44512, .F. ) ;
#39761=CARTESIAN_POINT ( 'NONE',  ( -4.999999999999999112, -80.91666666666667140, 2.886751345948131764 ) ) ;
#39762=CARTESIAN_POINT ( 'NONE',  ( 4.458734124999999437, -169.4375000013656063, 0.000000000000000000 ) ) ;
#39764=CARTESIAN_POINT ( 'NONE',  ( 5.000000000000000000, -87.29166666393548724, -2.886751345948129988 ) ) ;
#39765=CARTESIAN_POINT ( 'NONE',  ( 1.975475456537005874E-15, -48.62499999726880162, 5.000000000000000000 ) ) ;
#39766=ORIENTED_EDGE ( 'NONE', *, *, #548, .T. ) ;
#39768=CARTESIAN_POINT ( 'NONE',  ( -4.458734124999999437, -29.64583333196773651, -2.574251347313719407 ) ) ;
#39769=CARTESIAN_POINT ( 'NONE',  ( -5.000000000000000000, -50.08333333333332860, -2.886751345948128211 ) ) ;
#39770=ORIENTED_EDGE ( 'NONE', *, *, #53455, .F. ) ;
#39774=CARTESIAN_POINT ( 'NONE',  ( 3.152801135295366208, -163.8125000013656063, 3.152801135295367985 ) ) ;
#39776=CARTESIAN_POINT ( 'NONE',  ( 5.000000000000000888, -23.58333333333333215, 2.886751345948126879 ) ) ;
#39779=CARTESIAN_POINT ( 'NONE',  ( 4.458734124999999437, -76.06249999863440792, -5.460374474430324690E-16 ) ) ;
#39782=CARTESIAN_POINT ( 'NONE',  ( -4.458734125000000326, -145.1250000013656063, 1.846868145590734089 ) ) ;
#39786=CARTESIAN_POINT ( 'NONE',  ( -5.000000000000000000, -0.08333333333333454995, -2.886751345948128211 ) ) ;
#39787=VECTOR ( 'NONE', #42060, 1000.000000000000000 ) ;
#39791=CARTESIAN_POINT ( 'NONE',  ( -3.152801135295367985, -142.0625000013655779, 3.152801135295367096 ) ) ;
#39796=CARTESIAN_POINT ( 'NONE',  ( -3.152548672688508926E-16, -74.81249999863439371, -5.148502694627439702 ) ) ;
#39797=ADVANCED_FACE ( 'NONE', ( #39283 ), #58290, .T. ) ;
#39798=CARTESIAN_POINT ( 'NONE',  ( -6.972266317189433020E-16, -34.25000000000000000, -5.000000000000000000 ) ) ;
#39802=VERTEX_POINT ( 'NONE', #19353 ) ;
#39805=CARTESIAN_POINT ( 'NONE',  ( 1.975475456537005874E-15, -14.62499999726881228, 5.000000000000000000 ) ) ;
#39810=CARTESIAN_POINT ( 'NONE',  ( 2.229367062500001939, 17.77083333469892779, 3.861377020970579999 ) ) ;
#39818=CARTESIAN_POINT ( 'NONE',  ( -4.458734124999999437, -1.312499998634406140, 0.000000000000000000 ) ) ;
#39819=CARTESIAN_POINT ( 'NONE',  ( 9.457646018065525792E-16, -30.31249999863440436, 5.148502694627439702 ) ) ;
#39823=CARTESIAN_POINT ( 'NONE',  ( -2.229367062500000163, 25.52083333469892779, -3.861377020970580443 ) ) ;
#39824=CARTESIAN_POINT ( 'NONE',  ( 6.123233995736766282E-16, -170.0000000000000000, -5.000000000000000000 ) ) ;
#39826=CARTESIAN_POINT ( 'NONE',  ( 9.457646018065525792E-16, -76.31249999863440792, 5.148502694627439702 ) ) ;
#39829=CARTESIAN_POINT ( 'NONE',  ( 2.500000000000002220, 22.45833333606451987, 4.330127018922192761 ) ) ;
#39830=ORIENTED_EDGE ( 'NONE', *, *, #2066, .F. ) ;
#39831=CARTESIAN_POINT ( 'NONE',  ( 2.626220312808019583E-14, 14.87500000273118239, -5.000000000000000000 ) ) ;
#39832=( BOUNDED_CURVE ( )  B_SPLINE_CURVE ( 2, ( #20633, #11279, #55036, #15798, #40864, #45382, #10960, #1347, #60192 ),
 .UNSPECIFIED., .F., .F. ) 
 B_SPLINE_CURVE_WITH_KNOTS ( ( 3, 2, 2, 2, 3 ),
 ( 0.7229166666666666519, 0.7236111111111110938, 0.7249999999999999778, 0.7263888888888888618, 0.7270833333333333037 ),
 .UNSPECIFIED. ) 
 CURVE ( )  GEOMETRIC_REPRESENTATION_ITEM ( )  RATIONAL_B_SPLINE_CURVE ( ( 0.9330127018922194093, 0.9330127018922194093, 1.000000000000000000, 0.8660254037844387076, 1.000000000000000000, 0.8660254037844387076, 1.000000000000000000, 0.9330127018922194093, 0.9330127018922194093 ) ) 
 REPRESENTATION_ITEM ( '' )  );
#39833=VECTOR ( 'NONE', #12674, 1000.000000000000000 ) ;
#39834=CARTESIAN_POINT ( 'NONE',  ( 2.499999999999998668, -16.33333333333333215, -4.330127018922193649 ) ) ;
#39835=CARTESIAN_POINT ( 'NONE',  ( -4.458734124999999437, -22.31249999863440436, 0.000000000000000000 ) ) ;
#39836=VECTOR ( 'NONE', #28204, 1000.000000000000000 ) ;
#39837=CARTESIAN_POINT ( 'NONE',  ( -2.229367062500000163, -83.47916666530106511, -3.861377020970580443 ) ) ;
#39838=CARTESIAN_POINT ( 'NONE',  ( -4.999999999999999112, -21.79166666393547658, 2.886751345948131764 ) ) ;
#39839=CARTESIAN_POINT ( 'NONE',  ( 9.457646018065525792E-16, -48.06249999863440081, 5.148502694627439702 ) ) ;
#39843=CARTESIAN_POINT ( 'NONE',  ( 9.457646018065525792E-16, 2.687500001365594304, 5.148502694627439702 ) ) ;
#39846=CARTESIAN_POINT ( 'NONE',  ( 5.000000000000000888, -64.58333333333332860, 2.886751345948126879 ) ) ;
#39847=CARTESIAN_POINT ( 'NONE',  ( 3.152801135295366208, -150.8125000013655779, 3.152801135295367985 ) ) ;
#39850=CARTESIAN_POINT ( 'NONE',  ( 3.535533905932738197, -161.8750000000000284, -3.535533905932738197 ) ) ;
#39851=CARTESIAN_POINT ( 'NONE',  ( -5.000000000000000000, 11.00000000000000000, 0.000000000000000000 ) ) ;
#39853=CARTESIAN_POINT ( 'NONE',  ( -4.458734124999999437, -10.64583333196773829, -2.574251347313719407 ) ) ;
#39854=CARTESIAN_POINT ( 'NONE',  ( 4.458734125000001214, -47.14583333196774362, 2.574251347313718519 ) ) ;
#39855=CARTESIAN_POINT ( 'NONE',  ( 3.061616997868383141E-16, -165.8750000027312126, -5.000000000000000000 ) ) ;
#39856=CARTESIAN_POINT ( 'NONE',  ( -4.458734124999999437, -144.9375000013656063, -5.460374474430324690E-16 ) ) ;
#39859=EDGE_LOOP ( 'NONE', ( #40903, #61914, #2094, #13762 ) ) ;
#39863=FACE_OUTER_BOUND ( 'NONE', #3001, .T. ) ;
#39864=ORIENTED_EDGE ( 'NONE', *, *, #42915, .T. ) ;
#39869=CARTESIAN_POINT ( 'NONE',  ( -4.458734124999999437, -1.395833331967737179, -2.574251347313719407 ) ) ;
#39871=CARTESIAN_POINT ( 'NONE',  ( 1.846868145590736310, -147.6250000013655779, 4.458734124999997661 ) ) ;
#39872=VECTOR ( 'NONE', #8563, 1000.000000000000000 ) ;
#39875=VERTEX_POINT ( 'NONE', #58605 ) ;
#39885=CARTESIAN_POINT ( 'NONE',  ( 1.339745962155612702, -74.29465819873853150, -5.000000000000000000 ) ) ;
#39887=CARTESIAN_POINT ( 'NONE',  ( -5.000000000000000000, -89.95833333060214443, -2.886751345948128211 ) ) ;
#39888=CARTESIAN_POINT ( 'NONE',  ( 4.458734124999999437, 15.18750000136559564, -5.460374474430324690E-16 ) ) ;
#39890=VERTEX_POINT ( 'NONE', #9079 ) ;
#39891=CARTESIAN_POINT ( 'NONE',  ( 2.229367062499998831, -13.89583333196774184, -3.861377020970580887 ) ) ;
#39893=CARTESIAN_POINT ( 'NONE',  ( 3.152801135295366208, -163.5625000013656063, 3.152801135295367985 ) ) ;
#39894=CARTESIAN_POINT ( 'NONE',  ( 1.975475456537005874E-15, -63.62499999726880873, 5.000000000000000000 ) ) ;
#39898=AXIS2_PLACEMENT_3D ( 'NONE', #12921, #17449, #17757 ) ;
#39902=DIRECTION ( 'NONE',  ( -0.000000000000000000, 1.000000000000000000, -0.000000000000000000 ) ) ;
#39903=CARTESIAN_POINT ( 'NONE',  ( -3.152801135295367985, -153.0625000013656063, 3.152801135295367096 ) ) ;
#39905=CARTESIAN_POINT ( 'NONE',  ( 5.000000000000000888, -46.58333333333334991, 2.886751345948126879 ) ) ;
#39910=CARTESIAN_POINT ( 'NONE',  ( -1.339745962155610925, -8.669658196007331341, 5.000000000000000000 ) ) ;
#39911=CARTESIAN_POINT ( 'NONE',  ( 1.060575238724906964E-15, -4.749999999999997335, 5.773502691896257311 ) ) ;
#39912=CARTESIAN_POINT ( 'NONE',  ( 2.229367062499998831, -65.64583333196773651, -3.861377020970580887 ) ) ;
#39913=CARTESIAN_POINT ( 'NONE',  ( -5.000000000000000000, -30.87499999726881228, 0.000000000000000000 ) ) ;
#39914=CARTESIAN_POINT ( 'NONE',  ( 2.500000000000002220, -4.541666663935479242, 4.330127018922192761 ) ) ;
#39915=CARTESIAN_POINT ( 'NONE',  ( -4.458734124999998549, -32.22916666530106511, 2.574251347313722516 ) ) ;
#39921=CARTESIAN_POINT ( 'NONE',  ( 5.000000000000000000, -48.50000000000000000, -6.123233995736766282E-16 ) ) ;
#39922=CARTESIAN_POINT ( 'NONE',  ( -6.972266317189433020E-16, -46.12499999726880873, -5.000000000000000000 ) ) ;
#39925=CARTESIAN_POINT ( 'NONE',  ( -1.339745962155613812, -4.205341801261476498, -5.000000000000000000 ) ) ;
#39926=CARTESIAN_POINT ( 'NONE',  ( -2.229367062500000163, -75.47916666530106511, -3.861377020970580443 ) ) ;
#39927=CARTESIAN_POINT ( 'NONE',  ( -4.458734125000001214, -142.1250000013656063, 1.846868145590734089 ) ) ;
#39928=CARTESIAN_POINT ( 'NONE',  ( 9.457646018065525792E-16, -81.06249999863440792, 5.148502694627439702 ) ) ;
#39931=CARTESIAN_POINT ( 'NONE',  ( -4.458734124999999437, -29.56249999863440436, 0.000000000000000000 ) ) ;
#39932=CARTESIAN_POINT ( 'NONE',  ( 1.060575238724906964E-15, -69.62499999726880162, 5.773502691896257311 ) ) ;
#39939=CARTESIAN_POINT ( 'NONE',  ( -6.972266317189433020E-16, 27.74999999999999645, -5.000000000000000000 ) ) ;
#39941=CARTESIAN_POINT ( 'NONE',  ( 4.458734124999999437, -60.06249999863440081, -5.460374474430324690E-16 ) ) ;
#39945=CARTESIAN_POINT ( 'NONE',  ( -4.458734124999999437, 14.68750000136559386, 0.000000000000000000 ) ) ;
#39947=CARTESIAN_POINT ( 'NONE',  ( 1.339745962155612702, -24.29465819873852084, -5.000000000000000000 ) ) ;
#39948=CARTESIAN_POINT ( 'NONE',  ( 3.152801135295367541, -162.3125000013656063, -3.152801135295367541 ) ) ;
#39949=LINE ( 'NONE', #59597, #39872 ) ;
#39950=ORIENTED_EDGE ( 'NONE', *, *, #20766, .F. ) ;
#39952=CARTESIAN_POINT ( 'NONE',  ( 6.123233995736766282E-16, -170.0000000000000000, -5.000000000000000000 ) ) ;
#39954=CARTESIAN_POINT ( 'NONE',  ( 6.123233995736766282E-16, -170.0000000000000000, -5.000000000000000000 ) ) ;
#39955=( BOUNDED_CURVE ( )  B_SPLINE_CURVE ( 2, ( #338, #54684, #5154, #34404, #10928, #1316, #5791, #35379, #14792 ),
 .UNSPECIFIED., .F., .F. ) 
 B_SPLINE_CURVE_WITH_KNOTS ( ( 3, 2, 2, 2, 3 ),
 ( 0.2229166666666666796, 0.2236111111111111216, 0.2250000000000000056, 0.2263888888888888895, 0.2270833333333333315 ),
 .UNSPECIFIED. ) 
 CURVE ( )  GEOMETRIC_REPRESENTATION_ITEM ( )  RATIONAL_B_SPLINE_CURVE ( ( 0.9330127018922194093, 0.9330127018922207416, 1.000000000000000000, 0.8660254037844387076, 1.000000000000000000, 0.8660254037844387076, 1.000000000000000000, 0.9330127018922194093, 0.9330127018922194093 ) ) 
 REPRESENTATION_ITEM ( '' )  );
#39957=CYLINDRICAL_SURFACE ( 'NONE', #45965, 5.000000000000000000 ) ;
#39967=CARTESIAN_POINT ( 'NONE',  ( -4.458734124999997661, 4.520833334698926897, 2.574251347313722516 ) ) ;
#39969=DIRECTION ( 'NONE',  ( 0.000000000000000000, 0.000000000000000000, 1.000000000000000000 ) ) ;
#39971=CARTESIAN_POINT ( 'NONE',  ( 3.535533905932738197, -144.0000000027311842, -3.535533905932738197 ) ) ;
#39977=CARTESIAN_POINT ( 'NONE',  ( 2.071067811865476394, -140.1875000000000000, 5.000000000000000000 ) ) ;
#39979=CARTESIAN_POINT ( 'NONE',  ( 1.846868145590736310, -165.8750000013656063, 4.458734124999997661 ) ) ;
#39981=CARTESIAN_POINT ( 'NONE',  ( 1.339745962155612702, 7.705341801261479162, -5.000000000000000000 ) ) ;
#39983=CARTESIAN_POINT ( 'NONE',  ( 4.458734125000000326, -144.3750000013656063, -1.846868145590734978 ) ) ;
#39985=CARTESIAN_POINT ( 'NONE',  ( 2.229367062499998831, 25.10416666803225993, -3.861377020970580887 ) ) ;
#39987=CARTESIAN_POINT ( 'NONE',  ( -2.229367062500000163, -64.72916666530106511, -3.861377020970580443 ) ) ;
#39990=CARTESIAN_POINT ( 'NONE',  ( 1.060575238724906964E-15, 14.25000000000000178, 5.773502691896257311 ) ) ;
#39991=ADVANCED_FACE ( 'NONE', ( #43479 ), #9386, .T. ) ;
#39992=CARTESIAN_POINT ( 'NONE',  ( 4.458734125000000326, -48.89583333196772941, 2.574251347313718519 ) ) ;
#39993=CARTESIAN_POINT ( 'NONE',  ( 9.457646018065525792E-16, -10.06249999863440792, 5.148502694627439702 ) ) ;
#39994=CARTESIAN_POINT ( 'NONE',  ( -6.972266317189433020E-16, 13.74999999999999822, -5.000000000000000000 ) ) ;
#39995=CARTESIAN_POINT ( 'NONE',  ( -6.972266317189433020E-16, -60.12499999726880162, -5.000000000000000000 ) ) ;
#39997=CARTESIAN_POINT ( 'NONE',  ( 5.000000000000000000, -66.37499999726881583, -6.123233995736766282E-16 ) ) ;
#39998=CARTESIAN_POINT ( 'NONE',  ( -2.498395430326213474E-14, 15.25000000000000000, 5.000000000000000000 ) ) ;
#40001=CARTESIAN_POINT ( 'NONE',  ( -2.229367062499996610, -52.14583333196773651, 3.861377020970582219 ) ) ;
#40002=CARTESIAN_POINT ( 'NONE',  ( 3.152801135295366208, -157.8125000013656063, 3.152801135295367985 ) ) ;
#40004=CARTESIAN_POINT ( 'NONE',  ( -2.500000000000000444, -54.04166666393548013, -4.330127018922193649 ) ) ;
#40007=CARTESIAN_POINT ( 'NONE',  ( 2.229367062499998831, 6.104166668032262599, -3.861377020970580887 ) ) ;
#40008=ADVANCED_FACE ( 'NONE', ( #11610 ), #25784, .T. ) ;
#40012=CARTESIAN_POINT ( 'NONE',  ( -1.846868145590734756, -157.1250000013656063, -4.458734125000000326 ) ) ;
#40013=ORIENTED_EDGE ( 'NONE', *, *, #47653, .T. ) ;
#40015=CARTESIAN_POINT ( 'NONE',  ( 5.000000000000000000, -87.37499999726880162, -6.123233995736766282E-16 ) ) ;
#40017=CARTESIAN_POINT ( 'NONE',  ( 2.071067811865391572, -160.9375000027312126, -5.000000000000086153 ) ) ;
#40018=VECTOR ( 'NONE', #27122, 1000.000000000000227 ) ;
#40019=CARTESIAN_POINT ( 'NONE',  ( 4.458734125000001214, -42.14583333196773651, 2.574251347313718519 ) ) ;
#40021=DIRECTION ( 'NONE',  ( -0.000000000000000000, 1.000000000000000000, -0.000000000000000000 ) ) ;
#40023=CARTESIAN_POINT ( 'NONE',  ( 2.229367062500001939, -89.22916666530106511, 3.861377020970579999 ) ) ;
#40026=CARTESIAN_POINT ( 'NONE',  ( 1.339745962155612702, -61.16965819600733312, -5.000000000000000000 ) ) ;
#40030=CARTESIAN_POINT ( 'NONE',  ( -1.339745962155589165, 9.919658201469706782, -5.000000000000014211 ) ) ;
#40032=CARTESIAN_POINT ( 'NONE',  ( -1.339745962155613812, 6.794658198738520838, -5.000000000000000000 ) ) ;
#40034=ADVANCED_FACE ( 'NONE', ( #45395 ), #5844, .T. ) ;
#40037=DIRECTION ( 'NONE',  ( -0.000000000000000000, 1.000000000000000000, -0.000000000000000000 ) ) ;
#40038=CARTESIAN_POINT ( 'NONE',  ( -4.458734124999998549, -88.47916666530107932, 2.574251347313722516 ) ) ;
#40039=DIRECTION ( 'NONE',  ( 0.000000000000000000, 0.000000000000000000, 1.000000000000000000 ) ) ;
#40041=ORIENTED_EDGE ( 'NONE', *, *, #23178, .F. ) ;
#40044=CARTESIAN_POINT ( 'NONE',  ( -9.184850993605147944E-16, -161.3750000027311842, 5.000000000000000000 ) ) ;
#40047=CARTESIAN_POINT ( 'NONE',  ( -1.049326080737009628E-13, -19.75000000000000000, 5.000000000000000000 ) ) ;
#40056=CARTESIAN_POINT ( 'NONE',  ( -4.458734124999999437, -19.31249999863440081, 0.000000000000000000 ) ) ;
#40058=CARTESIAN_POINT ( 'NONE',  ( 5.000000000000000000, -155.0000000000000284, 0.000000000000000000 ) ) ;
#40060=CARTESIAN_POINT ( 'NONE',  ( 4.458734125000000326, -154.3750000013655779, -1.846868145590734978 ) ) ;
#40062=CARTESIAN_POINT ( 'NONE',  ( -2.229367062499996610, -44.39583333196774362, 3.861377020970582219 ) ) ;
#40063=( BOUNDED_CURVE ( )  B_SPLINE_CURVE ( 2, ( #44629, #14721, #589, #39166, #4756, #15373, #9897, #5081, #48506 ),
 .UNSPECIFIED., .F., .F. ) 
 B_SPLINE_CURVE_WITH_KNOTS ( ( 3, 2, 2, 2, 3 ),
 ( 0.6937499999999999778, 0.6944444444444444198, 0.6958333333333333037, 0.6972222222222221877, 0.6979166666666666297 ),
 .UNSPECIFIED. ) 
 CURVE ( )  GEOMETRIC_REPRESENTATION_ITEM ( )  RATIONAL_B_SPLINE_CURVE ( ( 0.9330127018922194093, 0.9330127018922194093, 1.000000000000000000, 0.8660254037844387076, 1.000000000000000000, 0.8660254037844387076, 1.000000000000000000, 0.9330127018922194093, 0.9330127018922194093 ) ) 
 REPRESENTATION_ITEM ( '' )  );
#40064=CARTESIAN_POINT ( 'NONE',  ( 1.975475456537005874E-15, -66.74999999999998579, 5.000000000000000000 ) ) ;
#40066=CARTESIAN_POINT ( 'NONE',  ( -2.499999999999996447, 29.16666666666666785, 4.330127018922195425 ) ) ;
#40067=AXIS2_PLACEMENT_3D ( 'NONE', #1727, #25512, #11350 ) ;
#40069=CARTESIAN_POINT ( 'NONE',  ( 9.457646018065525792E-16, 4.937500001365596525, 5.148502694627439702 ) ) ;
#40071=CARTESIAN_POINT ( 'NONE',  ( -5.000000000000000888, -165.5625000027312126, 2.071067811865474617 ) ) ;
#40072=CARTESIAN_POINT ( 'NONE',  ( -1.339745962155610925, -73.79465819873853150, 5.000000000000000000 ) ) ;
#40073=CARTESIAN_POINT ( 'NONE',  ( -2.229367062500000163, 21.27083333469892779, -3.861377020970580443 ) ) ;
#40075=CARTESIAN_POINT ( 'NONE',  ( 5.000000000000000888, 8.541666669397853795, 2.886751345948126879 ) ) ;
#40077=DIRECTION ( 'NONE',  ( -0.000000000000000000, 1.000000000000000000, -0.000000000000000000 ) ) ;
#40078=ORIENTED_EDGE ( 'NONE', *, *, #5119, .F. ) ;
#40080=CARTESIAN_POINT ( 'NONE',  ( 4.458734124999999437, -40.81249999863440081, -5.460374474430324690E-16 ) ) ;
#40081=CARTESIAN_POINT ( 'NONE',  ( 2.500000000000002220, -38.54166666393548013, 4.330127018922192761 ) ) ;
#40083=CARTESIAN_POINT ( 'NONE',  ( 4.458734125000001214, -10.89583333196773651, 2.574251347313718519 ) ) ;
#40085=CARTESIAN_POINT ( 'NONE',  ( 9.457646018065525792E-16, -21.31249999863440081, 5.148502694627439702 ) ) ;
#40087=CARTESIAN_POINT ( 'NONE',  ( 2.500000000000002220, -82.66666666666667140, 4.330127018922192761 ) ) ;
#40088=CARTESIAN_POINT ( 'NONE',  ( 3.152801135295366208, -166.5625000013656063, 3.152801135295367985 ) ) ;
#40091=CARTESIAN_POINT ( 'NONE',  ( -3.535250795749689387E-16, -89.12499999726880162, -5.773502691896257311 ) ) ;
#40093=ORIENTED_EDGE ( 'NONE', *, *, #39338, .T. ) ;
#40095=CARTESIAN_POINT ( 'NONE',  ( -4.458734124999998549, -25.47916666530106866, 2.574251347313722516 ) ) ;
#40097=ORIENTED_EDGE ( 'NONE', *, *, #23930, .F. ) ;
#40099=CARTESIAN_POINT ( 'NONE',  ( 1.846868145590735200, -164.5000000013655779, -4.458734125000000326 ) ) ;
#40101=CARTESIAN_POINT ( 'NONE',  ( 5.000000000000000888, -155.9375000000000000, -2.071067811865475505 ) ) ;
#40105=CARTESIAN_POINT ( 'NONE',  ( -4.458734124999999437, -76.56249999863440792, 0.000000000000000000 ) ) ;
#40108=CARTESIAN_POINT ( 'NONE',  ( 4.458734124999999437, -140.6250000013656063, -1.846868145590734978 ) ) ;
#40109=DIRECTION ( 'NONE',  ( 0.000000000000000000, 0.000000000000000000, 1.000000000000000000 ) ) ;
#40116=CARTESIAN_POINT ( 'NONE',  ( 3.061616997868383141E-16, -167.7500000000000000, -5.000000000000000000 ) ) ;
#40119=CARTESIAN_POINT ( 'NONE',  ( -4.999999999999998224, -52.91666666666666430, 2.886751345948131764 ) ) ;
#40121=CARTESIAN_POINT ( 'NONE',  ( -2.229367062499996610, -76.39583333196773651, 3.861377020970582219 ) ) ;
#40123=CARTESIAN_POINT ( 'NONE',  ( -4.999999999999998224, -0.7916666639354794643, 2.886751345948131764 ) ) ;
#40133=CARTESIAN_POINT ( 'NONE',  ( 2.229367062499998831, 16.10416666803225993, -3.861377020970580887 ) ) ;
#40134=CARTESIAN_POINT ( 'NONE',  ( 2.499999999999998668, -77.20833333060214443, -4.330127018922193649 ) ) ;
#40140=CARTESIAN_POINT ( 'NONE',  ( -2.229367062500000163, -83.47916666530106511, -3.861377020970580443 ) ) ;
#40141=CARTESIAN_POINT ( 'NONE',  ( -4.458734124999999437, -6.312499998634403475, 0.000000000000000000 ) ) ;
#40142=ORIENTED_EDGE ( 'NONE', *, *, #20488, .T. ) ;
#40143=CARTESIAN_POINT ( 'NONE',  ( 4.458734124999998549, -30.97916666530106866, -2.574251347313721627 ) ) ;
#40148=CARTESIAN_POINT ( 'NONE',  ( -3.152548672688508926E-16, 26.43750000136559208, -5.148502694627439702 ) ) ;
#40152=CYLINDRICAL_SURFACE ( 'NONE', #8047, 5.000000000000000000 ) ;
#40153=CARTESIAN_POINT ( 'NONE',  ( -4.458734124999999437, -78.64583333196773651, -2.574251347313719407 ) ) ;
#40156=FACE_OUTER_BOUND ( 'NONE', #3026, .T. ) ;
#40157=CARTESIAN_POINT ( 'NONE',  ( -4.999999999999999112, 26.20833333606451632, 2.886751345948131764 ) ) ;
#40158=VERTEX_POINT ( 'NONE', #56650 ) ;
#40159=CARTESIAN_POINT ( 'NONE',  ( 2.499999999999998668, -1.208333330602148870, -4.330127018922193649 ) ) ;
#40162=DIRECTION ( 'NONE',  ( -0.000000000000000000, 1.000000000000000000, -0.000000000000000000 ) ) ;
#40163=CARTESIAN_POINT ( 'NONE',  ( 1.060575238724906964E-15, -17.75000000000000355, 5.773502691896257311 ) ) ;
#40164=CARTESIAN_POINT ( 'NONE',  ( -2.229367062499996610, -23.14583333196773651, 3.861377020970582219 ) ) ;
#40165=EDGE_CURVE ( 'NONE', #52605, #39254, #23998, .T. ) ;
#40166=CARTESIAN_POINT ( 'NONE',  ( -4.458734124999999437, -84.39583333196773651, -2.574251347313719407 ) ) ;
#40167=EDGE_CURVE ( 'NONE', #14751, #51146, #32651, .T. ) ;
#40168=( BOUNDED_CURVE ( )  B_SPLINE_CURVE ( 2, ( #59614, #15546, #35167, #54782, #10713, #30320, #49942, #40613, #37077 ),
 .UNSPECIFIED., .F., .F. ) 
 B_SPLINE_CURVE_WITH_KNOTS ( ( 3, 2, 2, 2, 3 ),
 ( 0.2416666666666668628, 0.2458333333333335147, 0.2500000000000002220, 0.2541666666666668739, 0.2583333333333335813 ),
 .UNSPECIFIED. ) 
 CURVE ( )  GEOMETRIC_REPRESENTATION_ITEM ( )  RATIONAL_B_SPLINE_CURVE ( ( 0.9999999999999964473, 0.9238795325112902912, 1.000000000000000000, 0.9238795325112867385, 1.000000000000000000, 0.9238795325112867385, 1.000000000000000000, 0.9238795325112826307, 1.000000000000003997 ) ) 
 REPRESENTATION_ITEM ( '' )  );
#40169=CARTESIAN_POINT ( 'NONE',  ( 5.000000000000000888, -24.45833333060214088, 2.886751345948126879 ) ) ;
#40171=CARTESIAN_POINT ( 'NONE',  ( 2.229367062499998831, -51.64583333196773651, -3.861377020970580887 ) ) ;
#40172=ORIENTED_EDGE ( 'NONE', *, *, #38919, .F. ) ;
#40173=CARTESIAN_POINT ( 'NONE',  ( 5.000000000000000000, -65.50000000000000000, -6.123233995736766282E-16 ) ) ;
#40175=EDGE_CURVE ( 'NONE', #18747, #53481, #5984, .T. ) ;
#40176=CARTESIAN_POINT ( 'NONE',  ( -4.458734124999998549, -5.479166665301072214, 2.574251347313722516 ) ) ;
#40177=ORIENTED_EDGE ( 'NONE', *, *, #41053, .F. ) ;
#40179=CARTESIAN_POINT ( 'NONE',  ( -2.500000000000000444, -66.16666666666667140, -4.330127018922193649 ) ) ;
#40180=ADVANCED_FACE ( 'NONE', ( #7440 ), #27988, .T. ) ;
#40181=CARTESIAN_POINT ( 'NONE',  ( 1.846868145590736310, -153.8750000013655779, 4.458734124999999437 ) ) ;
#40183=CARTESIAN_POINT ( 'NONE',  ( -5.000000000000000000, -76.95833333060214443, -2.886751345948128211 ) ) ;
#40184=CARTESIAN_POINT ( 'NONE',  ( -5.000000000000000888, -157.5625000000000568, -2.071067811865475949 ) ) ;
#40188=CARTESIAN_POINT ( 'NONE',  ( 9.457646018065525792E-16, -12.31249999863440259, 5.148502694627439702 ) ) ;
#40189=CARTESIAN_POINT ( 'NONE',  ( -2.229367062500000163, -47.72916666530106511, -3.861377020970580443 ) ) ;
#40191=CARTESIAN_POINT ( 'NONE',  ( 1.846868145590735200, -146.2500000013656063, -4.458734125000000326 ) ) ;
#40196=CARTESIAN_POINT ( 'NONE',  ( 4.458734124999998549, 27.02083333469892423, -2.574251347313721627 ) ) ;
#40204=CARTESIAN_POINT ( 'NONE',  ( 4.458734124999999437, -9.812499998634406140, -5.460374474430324690E-16 ) ) ;
#40206=CARTESIAN_POINT ( 'NONE',  ( -8.190561711645485556E-16, -147.6875000013656063, 4.458734124999999437 ) ) ;
#40208=ORIENTED_EDGE ( 'NONE', *, *, #33158, .T. ) ;
#40209=CARTESIAN_POINT ( 'NONE',  ( -2.499999999999996447, -26.70833333060214798, 4.330127018922195425 ) ) ;
#40213=CARTESIAN_POINT ( 'NONE',  ( 5.000000000000000000, -25.37499999726881583, -6.123233995736766282E-16 ) ) ;
#40214=CARTESIAN_POINT ( 'NONE',  ( -6.972266317189433020E-16, -6.249999999999999112, -5.000000000000000000 ) ) ;
#40217=CARTESIAN_POINT ( 'NONE',  ( 5.000000000000000000, -74.41666666666665719, -2.886751345948130876 ) ) ;
#40219=DIRECTION ( 'NONE',  ( -0.000000000000000000, 1.000000000000000000, -0.000000000000000000 ) ) ;
#40220=PRODUCT_DEFINITION ( 'UNKNOWN', '', #56491, #23827 ) ;
#40222=CARTESIAN_POINT ( 'NONE',  ( 4.458734124999999437, 13.18750000136559208, -5.460374474430324690E-16 ) ) ;
#40225=CARTESIAN_POINT ( 'NONE',  ( 2.229367062499998831, -12.89583333196774007, -3.861377020970580887 ) ) ;
#40228=CARTESIAN_POINT ( 'NONE',  ( -4.458734124999999437, -163.9375000013655779, -5.460374474430324690E-16 ) ) ;
#40229=CARTESIAN_POINT ( 'NONE',  ( -5.000000000000000000, -37.99999999999999289, 0.000000000000000000 ) ) ;
#40236=CARTESIAN_POINT ( 'NONE',  ( -6.972266317189433020E-16, -83.12499999726878741, -5.000000000000000000 ) ) ;
#40237=CARTESIAN_POINT ( 'NONE',  ( 3.152801135295367541, -149.5625000013655779, -3.152801135295367541 ) ) ;
#40239=CARTESIAN_POINT ( 'NONE',  ( 1.975475456537005874E-15, 20.24999999999999645, 5.000000000000000000 ) ) ;
#40245=CARTESIAN_POINT ( 'NONE',  ( -2.500000000000000444, -1.166666666666666519, -4.330127018922193649 ) ) ;
#40246=CARTESIAN_POINT ( 'NONE',  ( -3.152548672688508926E-16, -64.56249999863440792, -5.148502694627439702 ) ) ;
#40247=DIRECTION ( 'NONE',  ( -0.000000000000000000, 1.000000000000000000, -0.000000000000000000 ) ) ;
#40248=CARTESIAN_POINT ( 'NONE',  ( 5.000000000000000000, -6.374999997268812280, -6.123233995736766282E-16 ) ) ;
#40249=CARTESIAN_POINT ( 'NONE',  ( -4.458734124999999437, -34.39583333196772941, -2.574251347313719407 ) ) ;
#40251=CYLINDRICAL_SURFACE ( 'NONE', #28635, 5.000000000000000000 ) ;
#40255=CARTESIAN_POINT ( 'NONE',  ( 1.060575238724906964E-15, -47.75000000000000000, 5.773502691896257311 ) ) ;
#40256=ADVANCED_FACE ( 'NONE', ( #17082 ), #61474, .T. ) ;
#40258=CARTESIAN_POINT ( 'NONE',  ( 2.500000000000002220, -32.54166666393547303, 4.330127018922192761 ) ) ;
#40259=CARTESIAN_POINT ( 'NONE',  ( -2.229367062500000163, -73.47916666530106511, -3.861377020970580443 ) ) ;
#40260=CARTESIAN_POINT ( 'NONE',  ( 3.152801135295367541, -141.5625000013655779, -3.152801135295367541 ) ) ;
#40261=CARTESIAN_POINT ( 'NONE',  ( -4.458734124999998549, -82.22916666530107932, 2.574251347313722516 ) ) ;
#40263=CARTESIAN_POINT ( 'NONE',  ( -2.229367062500000163, -27.72916666530107221, -3.861377020970580443 ) ) ;
#40265=VERTEX_POINT ( 'NONE', #24427 ) ;
#40267=ORIENTED_EDGE ( 'NONE', *, *, #35281, .T. ) ;
#40269=CARTESIAN_POINT ( 'NONE',  ( 2.499999999999998668, -21.33333333333333570, -4.330127018922193649 ) ) ;
#40270=ORIENTED_EDGE ( 'NONE', *, *, #35079, .F. ) ;
#40275=CARTESIAN_POINT ( 'NONE',  ( -2.229367062500000163, -66.72916666530106511, -3.861377020970580443 ) ) ;
#40277=ORIENTED_EDGE ( 'NONE', *, *, #13801, .T. ) ;
#40278=CARTESIAN_POINT ( 'NONE',  ( -6.972266317189433020E-16, -45.24999999999999289, -5.000000000000000000 ) ) ;
#40279=CARTESIAN_POINT ( 'NONE',  ( 0.000000000000000000, -170.0000000000000000, 0.000000000000000000 ) ) ;
#40280=CARTESIAN_POINT ( 'NONE',  ( 4.458734125000001214, 10.10416666803226171, 2.574251347313718519 ) ) ;
#40283=CARTESIAN_POINT ( 'NONE',  ( 3.152801135295367541, -161.3125000013656063, -3.152801135295367541 ) ) ;
#40289=DIRECTION ( 'NONE',  ( -0.000000000000000000, 1.000000000000000000, -0.000000000000000000 ) ) ;
#40290=DIRECTION ( 'NONE',  ( 0.000000000000000000, 0.000000000000000000, 1.000000000000000000 ) ) ;
#40293=DIRECTION ( 'NONE',  ( -0.000000000000000000, 1.000000000000000000, -0.000000000000000000 ) ) ;
#40294=CARTESIAN_POINT ( 'NONE',  ( 1.339745962155615144, -78.58034179853028434, 4.999999999999999112 ) ) ;
#40296=CARTESIAN_POINT ( 'NONE',  ( 5.000000000000000000, -82.37499999726881583, -6.123233995736766282E-16 ) ) ;
#40299=CARTESIAN_POINT ( 'NONE',  ( -3.152548672688508926E-16, 2.187500001365593416, -5.148502694627439702 ) ) ;
#40300=CARTESIAN_POINT ( 'NONE',  ( 3.535533905932738197, -150.8750000000000000, -3.535533905932738197 ) ) ;
#40302=CARTESIAN_POINT ( 'NONE',  ( -9.184850993605147944E-16, -146.3750000027312126, 5.000000000000000000 ) ) ;
#40303=CARTESIAN_POINT ( 'NONE',  ( -6.972266317189433020E-16, -84.24999999999998579, -5.000000000000000000 ) ) ;
#40307=CARTESIAN_POINT ( 'NONE',  ( -6.972266317189433020E-16, -70.12499999726880162, -5.000000000000000000 ) ) ;
#40311=CARTESIAN_POINT ( 'NONE',  ( 3.152801135295366208, -160.8125000013656063, 3.152801135295367985 ) ) ;
#40312=CARTESIAN_POINT ( 'NONE',  ( -5.000000000000000888, -160.4375000000000568, 2.071067811865474617 ) ) ;
#40315=CARTESIAN_POINT ( 'NONE',  ( 4.458734125000000326, -140.3750000013656063, -1.846868145590734978 ) ) ;
#40317=CARTESIAN_POINT ( 'NONE',  ( -2.229367062500000163, 23.27083333469892779, -3.861377020970580443 ) ) ;
#40318=ORIENTED_EDGE ( 'NONE', *, *, #38227, .T. ) ;
#40319=CARTESIAN_POINT ( 'NONE',  ( -4.458734124999997661, -60.47916666530106511, 2.574251347313722516 ) ) ;
#40322=CARTESIAN_POINT ( 'NONE',  ( -5.000000000000000000, 11.91666666666666607, -2.886751345948128211 ) ) ;
#40323=CARTESIAN_POINT ( 'NONE',  ( -3.152548672688508926E-16, -48.56249999863440792, -5.148502694627439702 ) ) ;
#40324=CARTESIAN_POINT ( 'NONE',  ( -4.458734124999999437, -12.31249999863440259, 0.000000000000000000 ) ) ;
#40329=CARTESIAN_POINT ( 'NONE',  ( 5.000000000000000000, -139.1250000027312126, 0.000000000000000000 ) ) ;
#40330=CARTESIAN_POINT ( 'NONE',  ( -2.229367062499996610, -60.14583333196774362, 3.861377020970582219 ) ) ;
#40331=CARTESIAN_POINT ( 'NONE',  ( 1.846868145590735200, -157.5000000013656063, -4.458734125000000326 ) ) ;
#40332=CARTESIAN_POINT ( 'NONE',  ( 2.499999999999998668, -55.20833333060214443, -4.330127018922193649 ) ) ;
#40333=ORIENTED_EDGE ( 'NONE', *, *, #27967, .F. ) ;
#40335=CARTESIAN_POINT ( 'NONE',  ( 2.229367062499998831, -0.8958333319677401763, -3.861377020970580887 ) ) ;
#40336=ORIENTED_EDGE ( 'NONE', *, *, #53716, .F. ) ;
#40338=CARTESIAN_POINT ( 'NONE',  ( 1.846868145590735200, -155.2500000013656063, -4.458734125000000326 ) ) ;
#40340=CARTESIAN_POINT ( 'NONE',  ( 1.339745962155612702, 25.70534180126147916, -5.000000000000000000 ) ) ;
#40342=CARTESIAN_POINT ( 'NONE',  ( 1.339745962155612702, -80.16965819600733312, -5.000000000000000000 ) ) ;
#40343=CARTESIAN_POINT ( 'NONE',  ( -3.152548672688508926E-16, -50.81249999863440792, -5.148502694627439702 ) ) ;
#40344=EDGE_LOOP ( 'NONE', ( #49402, #25166, #30257, #35374 ) ) ;
#40345=( BOUNDED_CURVE ( )  B_SPLINE_CURVE ( 2, ( #35704, #1625, #19938, #55331, #39550, #59191, #11248, #660, #20269 ),
 .UNSPECIFIED., .F., .F. ) 
 B_SPLINE_CURVE_WITH_KNOTS ( ( 3, 2, 2, 2, 3 ),
 ( 0.1729166666666666630, 0.1736111111111111049, 0.1749999999999999889, 0.1763888888888889006, 0.1770833333333333426 ),
 .UNSPECIFIED. ) 
 CURVE ( )  GEOMETRIC_REPRESENTATION_ITEM ( )  RATIONAL_B_SPLINE_CURVE ( ( 0.9330127018922194093, 0.9330127018922194093, 1.000000000000000000, 0.8660254037844387076, 1.000000000000000000, 0.8660254037844387076, 1.000000000000000000, 0.9330127018922194093, 0.9330127018922194093 ) ) 
 REPRESENTATION_ITEM ( '' )  );
#40348=CARTESIAN_POINT ( 'NONE',  ( -4.458734124999998549, 27.77083333469892423, 2.574251347313722516 ) ) ;
#40350=CARTESIAN_POINT ( 'NONE',  ( 3.061616997868383141E-16, -146.7500000000000284, -5.000000000000000000 ) ) ;
#40354=CARTESIAN_POINT ( 'NONE',  ( -2.499999999999996447, 1.166666666666666519, 4.330127018922195425 ) ) ;
#40356=EDGE_CURVE ( 'NONE', #51312, #55230, #9626, .T. ) ;
#40361=CARTESIAN_POINT ( 'NONE',  ( -2.499999999999996447, 25.16666666666666430, 4.330127018922195425 ) ) ;
#40363=CARTESIAN_POINT ( 'NONE',  ( 4.458734124999999437, -90.06249999863440792, -5.460374474430324690E-16 ) ) ;
#40364=CYLINDRICAL_SURFACE ( 'NONE', #61451, 5.000000000000000000 ) ;
#40366=ORIENTED_EDGE ( 'NONE', *, *, #25351, .F. ) ;
#40367=CARTESIAN_POINT ( 'NONE',  ( 5.000000000000000000, -31.50000000000000000, -6.123233995736766282E-16 ) ) ;
#40369=CARTESIAN_POINT ( 'NONE',  ( 2.071067811865475505, -155.9375000027312126, -5.000000000000000888 ) ) ;
#40381=CARTESIAN_POINT ( 'NONE',  ( 4.458734124999999437, -17.81249999863440792, -5.460374474430324690E-16 ) ) ;
#40383=CARTESIAN_POINT ( 'NONE',  ( -2.071067811865478170, -152.3125000000000000, 5.000000000000000000 ) ) ;
#40385=CARTESIAN_POINT ( 'NONE',  ( -4.458734125000000326, -151.0000000013656063, -1.846868145590735644 ) ) ;
#40387=CARTESIAN_POINT ( 'NONE',  ( 2.229367062500001939, -47.22916666530106511, 3.861377020970579999 ) ) ;
#40389=CARTESIAN_POINT ( 'NONE',  ( -2.500000000000000444, 28.83333333333333215, -4.330127018922193649 ) ) ;
#40390=CARTESIAN_POINT ( 'NONE',  ( -4.458734124999999437, 6.604166668032259047, -2.574251347313719407 ) ) ;
#40394=CARTESIAN_POINT ( 'NONE',  ( 2.229367062500001939, 18.77083333469892779, 3.861377020970579999 ) ) ;
#40397=CARTESIAN_POINT ( 'NONE',  ( -2.499999999999996447, 10.29166666939785024, 4.330127018922195425 ) ) ;
#40398=ORIENTED_EDGE ( 'NONE', *, *, #22697, .F. ) ;
#40402=CARTESIAN_POINT ( 'NONE',  ( 9.457646018065525792E-16, -42.06249999863440081, 5.148502694627439702 ) ) ;
#40404=CARTESIAN_POINT ( 'NONE',  ( 1.060575238724906964E-15, -41.62499999726880162, 5.773502691896257311 ) ) ;
#40406=CARTESIAN_POINT ( 'NONE',  ( -4.458734124999999437, -18.31249999863440792, 0.000000000000000000 ) ) ;
#40408=CARTESIAN_POINT ( 'NONE',  ( 5.000000000000000000, -80.50000000000000000, -6.123233995736766282E-16 ) ) ;
#40409=FACE_OUTER_BOUND ( 'NONE', #41253, .T. ) ;
#40410=CARTESIAN_POINT ( 'NONE',  ( 1.060575238724906964E-15, -88.62499999726880162, 5.773502691896257311 ) ) ;
#40414=CARTESIAN_POINT ( 'NONE',  ( 4.458734124999999437, -25.06249999863440792, -5.460374474430324690E-16 ) ) ;
#40415=EDGE_LOOP ( 'NONE', ( #41894, #46930, #47951, #26902 ) ) ;
#40417=CARTESIAN_POINT ( 'NONE',  ( 4.458734125000000326, -163.6250000013656063, -1.846868145590734978 ) ) ;
#40420=CARTESIAN_POINT ( 'NONE',  ( 5.000000000000000000, -55.37499999726880162, -6.123233995736766282E-16 ) ) ;
#40424=CARTESIAN_POINT ( 'NONE',  ( -4.458734124999999437, -75.56249999863440792, 0.000000000000000000 ) ) ;
#40427=CARTESIAN_POINT ( 'NONE',  ( 4.458734124999999437, -142.6250000013656063, -1.846868145590734978 ) ) ;
#40428=CARTESIAN_POINT ( 'NONE',  ( -1.339745962155610925, 6.330341803992665106, 5.000000000000000000 ) ) ;
#40430=CARTESIAN_POINT ( 'NONE',  ( 4.458734124999998549, -43.72916666530106511, -2.574251347313721627 ) ) ;
#40431=CARTESIAN_POINT ( 'NONE',  ( 6.123233995736766282E-16, -170.0000000000000000, -5.000000000000000000 ) ) ;
#40432=EDGE_CURVE ( 'NONE', #23954, #60539, #29234, .T. ) ;
#40435=CARTESIAN_POINT ( 'NONE',  ( -4.458734125000001214, -140.1250000013655779, 1.846868145590734089 ) ) ;
#40440=CARTESIAN_POINT ( 'NONE',  ( -4.458734124999999437, -75.64583333196775072, -2.574251347313719407 ) ) ;
#40445=ORIENTED_EDGE ( 'NONE', *, *, #19247, .F. ) ;
#40447=CARTESIAN_POINT ( 'NONE',  ( -1.127183054612291972E-14, 23.37500000273118772, 4.999999999999999112 ) ) ;
#40453=CARTESIAN_POINT ( 'NONE',  ( -4.458734124999997661, 17.52083333469892779, 2.574251347313722516 ) ) ;
#40462=CARTESIAN_POINT ( 'NONE',  ( 4.458734125000001214, -85.89583333196773651, 2.574251347313718519 ) ) ;
#40463=CARTESIAN_POINT ( 'NONE',  ( 2.229367062499998831, -2.645833331967738289, -3.861377020970580887 ) ) ;
#40465=CARTESIAN_POINT ( 'NONE',  ( 2.229367062499998831, -30.89583333196773651, -3.861377020970580887 ) ) ;
#40469=CARTESIAN_POINT ( 'NONE',  ( 4.458734124999998549, 22.27083333469893134, -2.574251347313721627 ) ) ;
#40470=CARTESIAN_POINT ( 'NONE',  ( 1.975475456537005874E-15, -77.75000000000000000, 5.000000000000000000 ) ) ;
#40471=CARTESIAN_POINT ( 'NONE',  ( -6.972266317189433020E-16, -66.24999999999998579, -5.000000000000000000 ) ) ;
#40472=CARTESIAN_POINT ( 'NONE',  ( 2.229367062500001939, -80.22916666530106511, 3.861377020970579999 ) ) ;
#40474=CARTESIAN_POINT ( 'NONE',  ( 1.060575238724906964E-15, 26.37500000273118417, 5.773502691896257311 ) ) ;
#40475=EDGE_LOOP ( 'NONE', ( #30335, #58117, #42010, #22486 ) ) ;
#40476=CARTESIAN_POINT ( 'NONE',  ( -1.339745962155610925, -65.79465819873851729, 5.000000000000000000 ) ) ;
#40478=DIRECTION ( 'NONE',  ( -0.000000000000000000, 1.000000000000000000, -0.000000000000000000 ) ) ;
#40479=CARTESIAN_POINT ( 'NONE',  ( 2.500000000000002220, -18.66666666666666430, 4.330127018922192761 ) ) ;
#40480=CARTESIAN_POINT ( 'NONE',  ( 4.458734125000001214, -22.89583333196773651, 2.574251347313718519 ) ) ;
#40481=CARTESIAN_POINT ( 'NONE',  ( 2.229367062500001939, -85.97916666530107932, 3.861377020970579999 ) ) ;
#40482=CARTESIAN_POINT ( 'NONE',  ( 2.500000000000002220, -24.54166666393548368, 4.330127018922192761 ) ) ;
#40483=EDGE_CURVE ( 'NONE', #27765, #42211, #52389, .T. ) ;
#40484=CARTESIAN_POINT ( 'NONE',  ( -4.458734124999999437, -56.31249999863440081, 0.000000000000000000 ) ) ;
#40486=CARTESIAN_POINT ( 'NONE',  ( 2.499999999999998668, -27.33333333333333570, -4.330127018922193649 ) ) ;
#40488=CARTESIAN_POINT ( 'NONE',  ( 9.457646018065525792E-16, -6.312499998634404363, 5.148502694627439702 ) ) ;
#40491=CARTESIAN_POINT ( 'NONE',  ( -5.000000000000000000, -64.00000000000000000, 0.000000000000000000 ) ) ;
#40492=CARTESIAN_POINT ( 'NONE',  ( 4.458734124999999437, -150.6875000013656063, 0.000000000000000000 ) ) ;
#40495=CARTESIAN_POINT ( 'NONE',  ( -5.000000000000000888, -159.4375000000000284, 2.071067811865474617 ) ) ;
#40498=CARTESIAN_POINT ( 'NONE',  ( -4.458734124999999437, -13.56249999863440259, 0.000000000000000000 ) ) ;
#40499=CARTESIAN_POINT ( 'NONE',  ( 4.458734125000001214, -53.14583333196773651, 2.574251347313718519 ) ) ;
#40502=CARTESIAN_POINT ( 'NONE',  ( 3.152801135295366208, -143.5625000013655779, 3.152801135295367985 ) ) ;
#40506=CARTESIAN_POINT ( 'NONE',  ( 1.975475456537005874E-15, -79.62499999726881583, 5.000000000000000000 ) ) ;
#40507=CARTESIAN_POINT ( 'NONE',  ( 9.457646018065525792E-16, 25.68750000136559208, 5.148502694627439702 ) ) ;
#40510=ORIENTED_EDGE ( 'NONE', *, *, #13795, .F. ) ;
#40513=EDGE_CURVE ( 'NONE', #48010, #28481, #1863, .T. ) ;
#40517=CARTESIAN_POINT ( 'NONE',  ( 9.457646018065525792E-16, -8.062499998634404363, 5.148502694627439702 ) ) ;
#40518=CARTESIAN_POINT ( 'NONE',  ( -4.458734124999999437, -148.0000000013656063, -1.846868145590735644 ) ) ;
#40520=VERTEX_POINT ( 'NONE', #58525 ) ;
#40526=CARTESIAN_POINT ( 'NONE',  ( 1.162044386198238837E-16, 29.25000000000000000, 5.000000000000000000 ) ) ;
#40527=( BOUNDED_CURVE ( )  B_SPLINE_CURVE ( 2, ( #51227, #56372, #27713, #7475, #3290 ),
 .UNSPECIFIED., .F., .F. ) 
 B_SPLINE_CURVE_WITH_KNOTS ( ( 3, 2, 3 ),
 ( 0.9916666666666665853, 0.9958333333333333481, 1.000000000000000000 ),
 .UNSPECIFIED. ) 
 CURVE ( )  GEOMETRIC_REPRESENTATION_ITEM ( )  RATIONAL_B_SPLINE_CURVE ( ( 1.000000000000001998, 0.9238795325112847401, 1.000000000000000000, 0.9238795325112867385, 1.000000000000000000 ) ) 
 REPRESENTATION_ITEM ( '' )  );
#40530=CARTESIAN_POINT ( 'NONE',  ( 0.000000000000000000, -170.0000000000000000, 0.000000000000000000 ) ) ;
#40535=CARTESIAN_POINT ( 'NONE',  ( -4.458734124999999437, 9.687500001365593860, 0.000000000000000000 ) ) ;
#40537=CARTESIAN_POINT ( 'NONE',  ( -2.229367062499996610, -15.39583333196773651, 3.861377020970582219 ) ) ;
#40539=CARTESIAN_POINT ( 'NONE',  ( -3.152801135295367985, -165.8125000013656063, 3.152801135295367096 ) ) ;
#40540=CARTESIAN_POINT ( 'NONE',  ( 1.339745962155618697, 23.70534180126147916, -4.999999999999998224 ) ) ;
#40545=( BOUNDED_CURVE ( )  B_SPLINE_CURVE ( 2, ( #63395, #57941, #23837, #39242, #28650, #49222, #24461, #23526, #5162 ),
 .UNSPECIFIED., .F., .F. ) 
 B_SPLINE_CURVE_WITH_KNOTS ( ( 3, 2, 2, 2, 3 ),
 ( 0.3437500000000000000, 0.3444444444444444420, 0.3458333333333333259, 0.3472222222222222099, 0.3479166666666666519 ),
 .UNSPECIFIED. ) 
 CURVE ( )  GEOMETRIC_REPRESENTATION_ITEM ( )  RATIONAL_B_SPLINE_CURVE ( ( 0.9330127018922194093, 0.9330127018922194093, 1.000000000000000000, 0.8660254037844387076, 1.000000000000000000, 0.8660254037844387076, 1.000000000000000000, 0.9330127018922194093, 0.9330127018922194093 ) ) 
 REPRESENTATION_ITEM ( '' )  );
#40547=CARTESIAN_POINT ( 'NONE',  ( -4.458734124999999437, -33.39583333196772941, -2.574251347313719407 ) ) ;
#40548=CARTESIAN_POINT ( 'NONE',  ( 0.000000000000000000, -170.0000000000000000, 0.000000000000000000 ) ) ;
#40549=CARTESIAN_POINT ( 'NONE',  ( -4.458734125000000326, -151.1250000013656347, 1.846868145590734089 ) ) ;
#40551=CARTESIAN_POINT ( 'NONE',  ( -1.339745962155613812, -14.20534180126148094, -5.000000000000000000 ) ) ;
#40553=ORIENTED_EDGE ( 'NONE', *, *, #40979, .T. ) ;
#40556=LINE ( 'NONE', #35743, #9305 ) ;
#40557=CARTESIAN_POINT ( 'NONE',  ( 5.000000000000000000, -3.416666666666665186, -2.886751345948129988 ) ) ;
#40558=CARTESIAN_POINT ( 'NONE',  ( -3.152548672688508926E-16, -68.56249999863439371, -5.148502694627439702 ) ) ;
#40559=CARTESIAN_POINT ( 'NONE',  ( 1.975475456537005874E-15, -16.74999999999999645, 5.000000000000000000 ) ) ;
#40560=CARTESIAN_POINT ( 'NONE',  ( 1.060575238724906964E-15, -5.624999997268811391, 5.773502691896257311 ) ) ;
#40561=CARTESIAN_POINT ( 'NONE',  ( 9.457646018065525792E-16, -40.06249999863439371, 5.148502694627439702 ) ) ;
#40563=CARTESIAN_POINT ( 'NONE',  ( 0.000000000000000000, -170.0000000000000000, 0.000000000000000000 ) ) ;
#40565=CARTESIAN_POINT ( 'NONE',  ( -4.458734124999999437, 10.43750000136559386, 0.000000000000000000 ) ) ;
#40566=ORIENTED_EDGE ( 'NONE', *, *, #59724, .F. ) ;
#40568=CARTESIAN_POINT ( 'NONE',  ( -2.500000000000000444, -50.16666666666666430, -4.330127018922193649 ) ) ;
#40570=CARTESIAN_POINT ( 'NONE',  ( 1.975475456537005874E-15, -34.75000000000000000, 5.000000000000000000 ) ) ;
#40571=CARTESIAN_POINT ( 'NONE',  ( -4.458734124999999437, -76.39583333196775072, -2.574251347313719407 ) ) ;
#40572=CARTESIAN_POINT ( 'NONE',  ( -1.846868145590737420, -140.0000000013655779, 4.458734124999999437 ) ) ;
#40573=CARTESIAN_POINT ( 'NONE',  ( -4.458734124999999437, -82.31249999863440792, 0.000000000000000000 ) ) ;
#40575=CARTESIAN_POINT ( 'NONE',  ( -4.458734124999999437, -34.56249999863440792, 0.000000000000000000 ) ) ;
#40578=VERTEX_POINT ( 'NONE', #50475 ) ;
#40580=CARTESIAN_POINT ( 'NONE',  ( 5.000000000000000888, -21.58333333333332860, 2.886751345948126879 ) ) ;
#40581=ORIENTED_EDGE ( 'NONE', *, *, #47998, .T. ) ;
#40584=CARTESIAN_POINT ( 'NONE',  ( 2.229367062500001939, -62.22916666530106511, 3.861377020970579999 ) ) ;
#40587=CARTESIAN_POINT ( 'NONE',  ( 5.000000000000000000, 3.708333336064517649, -2.886751345948130876 ) ) ;
#40588=ADVANCED_FACE ( 'NONE', ( #49817 ), #21196, .T. ) ;
#40589=DIRECTION ( 'NONE',  ( 0.000000000000000000, 0.000000000000000000, 1.000000000000000000 ) ) ;
#40591=CARTESIAN_POINT ( 'NONE',  ( -3.152548672688508926E-16, 5.437500001365592084, -5.148502694627439702 ) ) ;
#40593=CARTESIAN_POINT ( 'NONE',  ( 6.123233995736766282E-16, -170.0000000000000000, -5.000000000000000000 ) ) ;
#40594=CARTESIAN_POINT ( 'NONE',  ( 4.458734124999997661, -159.5000000013656063, 1.846868145590737864 ) ) ;
#40595=( BOUNDED_CURVE ( )  B_SPLINE_CURVE ( 2, ( #48073, #53843, #23646, #62882, #153, #58045, #33602, #58365, #19749 ),
 .UNSPECIFIED., .F., .F. ) 
 B_SPLINE_CURVE_WITH_KNOTS ( ( 3, 2, 2, 2, 3 ),
 ( 0.6854166666666666741, 0.6861111111111111160, 0.6875000000000000000, 0.6888888888888888840, 0.6895833333333333259 ),
 .UNSPECIFIED. ) 
 CURVE ( )  GEOMETRIC_REPRESENTATION_ITEM ( )  RATIONAL_B_SPLINE_CURVE ( ( 0.9330127018922194093, 0.9330127018922194093, 1.000000000000000000, 0.8660254037844387076, 1.000000000000000000, 0.8660254037844387076, 1.000000000000000000, 0.9330127018922194093, 0.9330127018922194093 ) ) 
 REPRESENTATION_ITEM ( '' )  );
#40596=FACE_OUTER_BOUND ( 'NONE', #15653, .T. ) ;
#40599=CARTESIAN_POINT ( 'NONE',  ( 3.061616997868383141E-16, -163.8750000027311842, -5.000000000000000000 ) ) ;
#40602=CYLINDRICAL_SURFACE ( 'NONE', #25391, 5.000000000000000000 ) ;
#40605=CARTESIAN_POINT ( 'NONE',  ( -6.972266317189433020E-16, -29.25000000000000000, -5.000000000000000000 ) ) ;
#40608=CARTESIAN_POINT ( 'NONE',  ( -4.458734124999999437, 26.60416666803225993, -2.574251347313719407 ) ) ;
#40609=EDGE_CURVE ( 'NONE', #39239, #33786, #12547, .T. ) ;
#40612=CARTESIAN_POINT ( 'NONE',  ( -4.458734124999997661, 2.520833334698928230, 2.574251347313722516 ) ) ;
#40613=CARTESIAN_POINT ( 'NONE',  ( -2.071067811865394237, -161.4375000027312410, 5.000000000000084377 ) ) ;
#40616=CARTESIAN_POINT ( 'NONE',  ( -5.000000000000000000, -143.6250000027312126, -6.123233995736766282E-16 ) ) ;
#40621=CARTESIAN_POINT ( 'NONE',  ( 0.000000000000000000, -170.0000000000000000, 5.000000000000000000 ) ) ;
#40625=CARTESIAN_POINT ( 'NONE',  ( 3.152801135295367541, -161.5625000013656063, -3.152801135295367541 ) ) ;
#40628=CARTESIAN_POINT ( 'NONE',  ( -1.339745962155610925, -56.79465819873851729, 5.000000000000000000 ) ) ;
#40630=CARTESIAN_POINT ( 'NONE',  ( -2.229367062500000163, 25.27083333469892779, -3.861377020970580443 ) ) ;
#40632=CARTESIAN_POINT ( 'NONE',  ( 2.229367062500001939, -61.22916666530106511, 3.861377020970579999 ) ) ;
#40633=( BOUNDED_CURVE ( )  B_SPLINE_CURVE ( 2, ( #14598, #63508, #54490, #13973, #43239, #44503, #53532, #63195, #20069 ),
 .UNSPECIFIED., .F., .F. ) 
 B_SPLINE_CURVE_WITH_KNOTS ( ( 3, 2, 2, 2, 3 ),
 ( 0.1250000000000001110, 0.1291666666666667906, 0.1333333333333334425, 0.1375000000000001221, 0.1416666666666667740 ),
 .UNSPECIFIED. ) 
 CURVE ( )  GEOMETRIC_REPRESENTATION_ITEM ( )  RATIONAL_B_SPLINE_CURVE ( ( 0.9999999999999980016, 0.9238795325112887369, 1.000000000000000000, 0.9238795325112867385, 1.000000000000000000, 0.9238795325112867385, 1.000000000000000000, 0.9238795325112847401, 1.000000000000001998 ) ) 
 REPRESENTATION_ITEM ( '' )  );
#40636=CARTESIAN_POINT ( 'NONE',  ( 2.499999999999998668, 13.66666666666666785, -4.330127018922193649 ) ) ;
#40637=CARTESIAN_POINT ( 'NONE',  ( 2.229367062500001939, -48.97916666530107221, 3.861377020970579999 ) ) ;
#40638=VECTOR ( 'NONE', #5884, 1000.000000000000000 ) ;
#40639=CARTESIAN_POINT ( 'NONE',  ( 2.229367062500001939, -11.97916666530107044, 3.861377020970579999 ) ) ;
#40640=CARTESIAN_POINT ( 'NONE',  ( 1.339745962155612702, -6.294658198738520838, -5.000000000000000000 ) ) ;
#40642=CARTESIAN_POINT ( 'NONE',  ( -2.499999999999996447, -36.83333333333332860, 4.330127018922195425 ) ) ;
#40643=DIRECTION ( 'NONE',  ( -0.000000000000000000, 1.000000000000000000, -0.000000000000000000 ) ) ;
#40644=CARTESIAN_POINT ( 'NONE',  ( 5.000000000000000888, -35.58333333333332860, 2.886751345948126879 ) ) ;
#40646=CARTESIAN_POINT ( 'NONE',  ( -2.498395430326213474E-14, 21.37500000273118062, 5.000000000000000000 ) ) ;
#40649=CARTESIAN_POINT ( 'NONE',  ( 4.458734124999998549, -59.72916666530106511, -2.574251347313721627 ) ) ;
#40650=CARTESIAN_POINT ( 'NONE',  ( -4.458734125000000326, -152.2500000013656347, -1.846868145590735644 ) ) ;
#40651=CARTESIAN_POINT ( 'NONE',  ( -4.458734124999998549, -64.22916666530107932, 2.574251347313722516 ) ) ;
#40652=CARTESIAN_POINT ( 'NONE',  ( -3.535250795749689387E-16, -57.12499999726880873, -5.773502691896257311 ) ) ;
#40653=ORIENTED_EDGE ( 'NONE', *, *, #8243, .F. ) ;
#40655=ORIENTED_EDGE ( 'NONE', *, *, #51089, .T. ) ;
#40658=CARTESIAN_POINT ( 'NONE',  ( -4.458734125000001214, -153.8750000013655779, 1.846868145590734089 ) ) ;
#40663=CARTESIAN_POINT ( 'NONE',  ( 2.229367062499998831, -47.89583333196774362, -3.861377020970580887 ) ) ;
#40664=ORIENTED_EDGE ( 'NONE', *, *, #14955, .F. ) ;
#40666=CARTESIAN_POINT ( 'NONE',  ( 2.229367062500001939, 24.02083333469892779, 3.861377020970579999 ) ) ;
#40669=CARTESIAN_POINT ( 'NONE',  ( 5.000000000000000888, -61.45833333060214443, 2.886751345948126879 ) ) ;
#40672=CARTESIAN_POINT ( 'NONE',  ( 1.062108568985190270E-13, -28.12499999726880873, -4.999999999999999112 ) ) ;
#40675=CARTESIAN_POINT ( 'NONE',  ( -5.000000000000000000, -26.99999999999999645, 0.000000000000000000 ) ) ;
#40679=FACE_OUTER_BOUND ( 'NONE', #6012, .T. ) ;
#40681=DIRECTION ( 'NONE',  ( -0.000000000000000000, 1.000000000000000000, -0.000000000000000000 ) ) ;
#40683=EDGE_LOOP ( 'NONE', ( #45638, #23863, #43760, #58307 ) ) ;
#40686=CARTESIAN_POINT ( 'NONE',  ( 3.061616997868383141E-16, -158.8750000027311842, -5.000000000000000000 ) ) ;
#40696=CARTESIAN_POINT ( 'NONE',  ( -4.458734124999999437, -20.31249999863440081, 0.000000000000000000 ) ) ;
#40698=CARTESIAN_POINT ( 'NONE',  ( -9.184850993605147944E-16, -150.2500000000000284, 5.000000000000000000 ) ) ;
#40700=CARTESIAN_POINT ( 'NONE',  ( -4.458734124999999437, -151.9375000013655779, -5.460374474430324690E-16 ) ) ;
#40702=CARTESIAN_POINT ( 'NONE',  ( -4.458734124999999437, -47.56249999863440792, 0.000000000000000000 ) ) ;
#40705=CARTESIAN_POINT ( 'NONE',  ( -5.000000000000000000, 27.91666666666666430, -2.886751345948128211 ) ) ;
#40706=CARTESIAN_POINT ( 'NONE',  ( -4.458734124999998549, 3.770833334698929562, 2.574251347313722516 ) ) ;
#40710=CARTESIAN_POINT ( 'NONE',  ( 2.229367062500001939, 16.77083333469892779, 3.861377020970579999 ) ) ;
#40712=CARTESIAN_POINT ( 'NONE',  ( 5.000000000000000888, 10.54166666939785202, 2.886751345948126879 ) ) ;
#40716=AXIS2_PLACEMENT_3D ( 'NONE', #26399, #11914, #5505 ) ;
#40718=CARTESIAN_POINT ( 'NONE',  ( 2.229367062499998831, -44.64583333196774362, -3.861377020970580887 ) ) ;
#40719=CARTESIAN_POINT ( 'NONE',  ( 1.846868145590736310, -162.8750000013655779, 4.458734124999999437 ) ) ;
#40722=CARTESIAN_POINT ( 'NONE',  ( 2.500000000000002220, -41.54166666393548013, 4.330127018922192761 ) ) ;
#40723=ORIENTED_EDGE ( 'NONE', *, *, #18493, .T. ) ;
#40724=CARTESIAN_POINT ( 'NONE',  ( -4.458734124999998549, -17.22916666530106866, 2.574251347313722516 ) ) ;
#40725=VERTEX_POINT ( 'NONE', #51108 ) ;
#40726=CARTESIAN_POINT ( 'NONE',  ( 5.000000000000000000, -89.41666666666667140, -2.886751345948129988 ) ) ;
#40727=CARTESIAN_POINT ( 'NONE',  ( 4.458734124999999437, -168.5000000013656063, 1.846868145590737864 ) ) ;
#40728=CARTESIAN_POINT ( 'NONE',  ( 2.500000000000002220, -85.54166666393547303, 4.330127018922192761 ) ) ;
#40729=CARTESIAN_POINT ( 'NONE',  ( -2.500000000000000444, -61.04166666393547303, -4.330127018922193649 ) ) ;
#40732=CARTESIAN_POINT ( 'NONE',  ( 4.458734124999999437, -35.06249999863440792, -5.460374474430324690E-16 ) ) ;
#40737=CARTESIAN_POINT ( 'NONE',  ( 5.000000000000000000, -23.41666666666667140, -2.886751345948130876 ) ) ;
#40738=ORIENTED_EDGE ( 'NONE', *, *, #21436, .F. ) ;
#40741=CARTESIAN_POINT ( 'NONE',  ( -2.229367062500000163, -81.72916666530106511, -3.861377020970580443 ) ) ;
#40744=CARTESIAN_POINT ( 'NONE',  ( -4.458734124999999437, -144.2500000013656063, -1.846868145590735644 ) ) ;
#40747=CARTESIAN_POINT ( 'NONE',  ( 2.229367062500001939, -45.97916666530106511, 3.861377020970579999 ) ) ;
#40751=CARTESIAN_POINT ( 'NONE',  ( -2.071067811865496378, -167.6875000000000284, -4.999999999999979572 ) ) ;
#40754=CARTESIAN_POINT ( 'NONE',  ( -5.000000000000000000, -39.95833333060214443, -2.886751345948128211 ) ) ;
#40756=CARTESIAN_POINT ( 'NONE',  ( -4.458734124999999437, -72.56249999863439371, 0.000000000000000000 ) ) ;
#40758=CARTESIAN_POINT ( 'NONE',  ( 2.500000000000002220, -76.66666666666665719, 4.330127018922192761 ) ) ;
#40761=VECTOR ( 'NONE', #18071, 1000.000000000000000 ) ;
#40762=LINE ( 'NONE', #15694, #56219 ) ;
#40763=CARTESIAN_POINT ( 'NONE',  ( 1.339745962155612702, -15.29465819873851906, -5.000000000000000000 ) ) ;
#40766=CARTESIAN_POINT ( 'NONE',  ( -6.972266317189433020E-16, 2.750000000000000000, -5.000000000000000000 ) ) ;
#40769=CARTESIAN_POINT ( 'NONE',  ( 2.229367062499998831, 15.10416666803225993, -3.861377020970580887 ) ) ;
#40775=( BOUNDED_CURVE ( )  B_SPLINE_CURVE ( 2, ( #28443, #41970, #18163, #38105, #23632, #17546, #12707, #47125, #56789 ),
 .UNSPECIFIED., .F., .F. ) 
 B_SPLINE_CURVE_WITH_KNOTS ( ( 3, 2, 2, 2, 3 ),
 ( 0.08541666666666666852, 0.08611111111111111049, 0.08749999999999999445, 0.08888888888888889228, 0.08958333333333333426 ),
 .UNSPECIFIED. ) 
 CURVE ( )  GEOMETRIC_REPRESENTATION_ITEM ( )  RATIONAL_B_SPLINE_CURVE ( ( 0.9330127018922194093, 0.9330127018922194093, 1.000000000000000000, 0.8660254037844387076, 1.000000000000000000, 0.8660254037844387076, 1.000000000000000000, 0.9330127018922194093, 0.9330127018922194093 ) ) 
 REPRESENTATION_ITEM ( '' )  );
#40776=CARTESIAN_POINT ( 'NONE',  ( 1.975475456537005874E-15, -15.62499999726881406, 5.000000000000000000 ) ) ;
#40777=CARTESIAN_POINT ( 'NONE',  ( -3.152548672688508926E-16, -86.56249999863440792, -5.148502694627439702 ) ) ;
#40778=CARTESIAN_POINT ( 'NONE',  ( -4.458734124999999437, -1.395833331967737179, -2.574251347313719407 ) ) ;
#40780=CARTESIAN_POINT ( 'NONE',  ( -2.229367062500000163, -30.72916666530107221, -3.861377020970580443 ) ) ;
#40784=CARTESIAN_POINT ( 'NONE',  ( 2.229367062499998831, 21.35416666803226349, -3.861377020970580887 ) ) ;
#40785=CARTESIAN_POINT ( 'NONE',  ( 5.000000000000000000, -53.49999999999999289, -6.123233995736766282E-16 ) ) ;
#40786=CARTESIAN_POINT ( 'NONE',  ( 1.339745962155612702, -28.29465819873851729, -5.000000000000000000 ) ) ;
#40787=CARTESIAN_POINT ( 'NONE',  ( -3.152548672688508926E-16, -75.81249999863440792, -5.148502694627439702 ) ) ;
#40790=CARTESIAN_POINT ( 'NONE',  ( -5.000000000000000000, 23.12500000273118417, 0.000000000000000000 ) ) ;
#40795=CARTESIAN_POINT ( 'NONE',  ( 5.000000000000000000, -21.41666666666666430, -2.886751345948129988 ) ) ;
#40796=CARTESIAN_POINT ( 'NONE',  ( 4.458734124999999437, -28.81249999863440436, -5.460374474430324690E-16 ) ) ;
#40798=CARTESIAN_POINT ( 'NONE',  ( 4.458734124999999437, -87.81249999863439371, -5.460374474430324690E-16 ) ) ;
#40799=CARTESIAN_POINT ( 'NONE',  ( 2.499999999999998668, -22.20833333060215153, -4.330127018922193649 ) ) ;
#40800=CARTESIAN_POINT ( 'NONE',  ( 4.458734124999999437, -57.81249999863440081, -5.460374474430324690E-16 ) ) ;
#40801=EDGE_LOOP ( 'NONE', ( #61476, #3723, #36813, #18405 ) ) ;
#40802=CARTESIAN_POINT ( 'NONE',  ( 2.500000000000002220, -74.54166666393547303, 4.330127018922192761 ) ) ;
#40803=CARTESIAN_POINT ( 'NONE',  ( 4.458734125000001214, -5.145833331967740065, 2.574251347313718519 ) ) ;
#40804=ORIENTED_EDGE ( 'NONE', *, *, #20940, .T. ) ;
#40805=CARTESIAN_POINT ( 'NONE',  ( -5.000000000000000000, -69.08333333333332860, -2.886751345948128211 ) ) ;
#40806=CARTESIAN_POINT ( 'NONE',  ( -3.152801135295367985, -151.0625000013655779, 3.152801135295367096 ) ) ;
#40809=CARTESIAN_POINT ( 'NONE',  ( -5.000000000000000888, -159.5625000000000568, -2.071067811865475949 ) ) ;
#40812=VECTOR ( 'NONE', #6475, 1000.000000000000000 ) ;
#40813=CARTESIAN_POINT ( 'NONE',  ( -4.458734124999998549, -14.47916666530107221, 2.574251347313722516 ) ) ;
#40814=CARTESIAN_POINT ( 'NONE',  ( 4.458734124999998549, -52.97916666530107932, -2.574251347313721627 ) ) ;
#40815=EDGE_CURVE ( 'NONE', #897, #27765, #967, .T. ) ;
#40817=CARTESIAN_POINT ( 'NONE',  ( -8.190561711645485556E-16, -142.6875000013656063, 4.458734124999999437 ) ) ;
#40818=ADVANCED_FACE ( 'NONE', ( #44670 ), #54654, .T. ) ;
#40820=CARTESIAN_POINT ( 'NONE',  ( -2.500000000000000444, 20.95833333606451987, -4.330127018922193649 ) ) ;
#40821=ORIENTED_EDGE ( 'NONE', *, *, #10507, .F. ) ;
#40823=CARTESIAN_POINT ( 'NONE',  ( -2.229367062499996610, 27.60416666803225993, 3.861377020970582219 ) ) ;
#40826=CARTESIAN_POINT ( 'NONE',  ( 1.339745962155612702, -50.29465819873851729, -5.000000000000000000 ) ) ;
#40828=EDGE_CURVE ( 'NONE', #45244, #8687, #26335, .T. ) ;
#40833=CARTESIAN_POINT ( 'NONE',  ( -4.458734124999998549, -8.229166665301073991, 2.574251347313722516 ) ) ;
#40835=CARTESIAN_POINT ( 'NONE',  ( 3.152801135295367541, -150.3125000013655779, -3.152801135295367541 ) ) ;
#40837=ORIENTED_EDGE ( 'NONE', *, *, #19300, .F. ) ;
#40838=CARTESIAN_POINT ( 'NONE',  ( -6.972266317189433020E-16, -63.12499999726880162, -5.000000000000000000 ) ) ;
#40841=CARTESIAN_POINT ( 'NONE',  ( -6.972266317189433020E-16, -85.12499999726880162, -5.000000000000000000 ) ) ;
#40842=FACE_OUTER_BOUND ( 'NONE', #58592, .T. ) ;
#40844=ADVANCED_FACE ( 'NONE', ( #1285 ), #30189, .T. ) ;
#40848=DIRECTION ( 'NONE',  ( 0.000000000000000000, 0.000000000000000000, 1.000000000000000000 ) ) ;
#40850=CARTESIAN_POINT ( 'NONE',  ( 4.458734124999998549, 11.27083333469893134, -2.574251347313721627 ) ) ;
#40852=CARTESIAN_POINT ( 'NONE',  ( -4.458734124999997661, -13.47916666530107221, 2.574251347313722516 ) ) ;
#40854=CARTESIAN_POINT ( 'NONE',  ( -3.152801135295367096, -164.0625000013656063, -3.152801135295367541 ) ) ;
#40861=CARTESIAN_POINT ( 'NONE',  ( -4.458734124999999437, -35.39583333196772941, -2.574251347313719407 ) ) ;
#40862=CARTESIAN_POINT ( 'NONE',  ( 1.975475456537005874E-15, -60.75000000000000000, 5.000000000000000000 ) ) ;
#40864=CARTESIAN_POINT ( 'NONE',  ( -5.000000000000000000, -57.87499999726880873, 0.000000000000000000 ) ) ;
#40870=CARTESIAN_POINT ( 'NONE',  ( 5.000000000000000000, -9.416666666666662522, -2.886751345948129988 ) ) ;
#40871=EDGE_CURVE ( 'NONE', #42718, #7443, #46181, .T. ) ;
#40872=CARTESIAN_POINT ( 'NONE',  ( -3.152548672688508926E-16, -70.56249999863439371, -5.148502694627439702 ) ) ;
#40873=CARTESIAN_POINT ( 'NONE',  ( 6.123233995736766282E-16, -170.0000000000000000, -5.000000000000000000 ) ) ;
#40876=CARTESIAN_POINT ( 'NONE',  ( 2.500000000000002220, -5.541666663935480130, 4.330127018922192761 ) ) ;
#40877=CARTESIAN_POINT ( 'NONE',  ( -2.229367062500000163, -38.47916666530107221, -3.861377020970580443 ) ) ;
#40880=CARTESIAN_POINT ( 'NONE',  ( -4.458734124999999437, 11.43750000136559564, 0.000000000000000000 ) ) ;
#40881=ORIENTED_EDGE ( 'NONE', *, *, #10072, .T. ) ;
#40882=CARTESIAN_POINT ( 'NONE',  ( 1.975475456537005874E-15, -39.75000000000000000, 5.000000000000000000 ) ) ;
#40883=CARTESIAN_POINT ( 'NONE',  ( 2.500000000000002220, -49.66666666666666430, 4.330127018922192761 ) ) ;
#40885=CARTESIAN_POINT ( 'NONE',  ( 1.975475456537005874E-15, -32.62499999726880873, 5.000000000000000000 ) ) ;
#40886=CARTESIAN_POINT ( 'NONE',  ( 4.458734124999998549, -74.72916666530106511, -2.574251347313721627 ) ) ;
#40887=CARTESIAN_POINT ( 'NONE',  ( 5.000000000000000888, -168.9375000000000284, -2.071067811865475505 ) ) ;
#40888=CARTESIAN_POINT ( 'NONE',  ( -2.229367062500000163, -88.47916666530106511, -3.861377020970580443 ) ) ;
#40890=CARTESIAN_POINT ( 'NONE',  ( 4.458734125000001214, -38.14583333196773651, 2.574251347313718519 ) ) ;
#40893=ADVANCED_FACE ( 'NONE', ( #3483 ), #52373, .T. ) ;
#40895=CARTESIAN_POINT ( 'NONE',  ( 1.339745962155612702, -21.29465819873852084, -5.000000000000000000 ) ) ;
#40896=ORIENTED_EDGE ( 'NONE', *, *, #62201, .T. ) ;
#40897=CARTESIAN_POINT ( 'NONE',  ( -1.339745962155613812, -4.080341798530293218, -5.000000000000000000 ) ) ;
#40898=VECTOR ( 'NONE', #15525, 1000.000000000000000 ) ;
#40900=CARTESIAN_POINT ( 'NONE',  ( 4.458734124999999437, -63.06249999863440792, -5.460374474430324690E-16 ) ) ;
#40901=VECTOR ( 'NONE', #25870, 1000.000000000000000 ) ;
#40903=ORIENTED_EDGE ( 'NONE', *, *, #61227, .F. ) ;
#40908=CARTESIAN_POINT ( 'NONE',  ( 2.229367062499998831, 5.354166668032261711, -3.861377020970580887 ) ) ;
#40909=CARTESIAN_POINT ( 'NONE',  ( 1.975475456537005874E-15, -32.62499999726880873, 5.000000000000000000 ) ) ;
#40910=CARTESIAN_POINT ( 'NONE',  ( -4.458734125000000326, -160.8750000013656063, 1.846868145590734089 ) ) ;
#40911=CARTESIAN_POINT ( 'NONE',  ( -2.500000000000000444, 18.95833333606451632, -4.330127018922193649 ) ) ;
#40912=ORIENTED_EDGE ( 'NONE', *, *, #4646, .F. ) ;
#40916=FACE_OUTER_BOUND ( 'NONE', #43095, .T. ) ;
#40921=CARTESIAN_POINT ( 'NONE',  ( -4.999999999999998224, -82.79166666393547303, 2.886751345948131764 ) ) ;
#40922=CARTESIAN_POINT ( 'NONE',  ( 2.229367062500001939, 26.02083333469892779, 3.861377020970579999 ) ) ;
#40925=CARTESIAN_POINT ( 'NONE',  ( -2.229367062499996610, 0.6041666680322611560, 3.861377020970582219 ) ) ;
#40927=CARTESIAN_POINT ( 'NONE',  ( 5.000000000000000000, -147.1875000027312126, 2.071067811865478614 ) ) ;
#40932=CARTESIAN_POINT ( 'NONE',  ( -2.071067811865478170, -140.3125000000000284, 5.000000000000000000 ) ) ;
#40933=CARTESIAN_POINT ( 'NONE',  ( 1.339745962155590275, 3.294658198738519950, 5.000000000000013323 ) ) ;
#40935=CARTESIAN_POINT ( 'NONE',  ( -1.846868145590737420, -163.0000000013655779, 4.458734124999997661 ) ) ;
#40936=CARTESIAN_POINT ( 'NONE',  ( 1.339745962155615144, 7.294658198738519950, 4.999999999999999112 ) ) ;
#40938=CARTESIAN_POINT ( 'NONE',  ( -3.152801135295367985, -139.8125000013655779, 3.152801135295367096 ) ) ;
#40940=CARTESIAN_POINT ( 'NONE',  ( 9.457646018065525792E-16, 23.68750000136559564, 5.148502694627439702 ) ) ;
#40941=ORIENTED_EDGE ( 'NONE', *, *, #22117, .T. ) ;
#40945=CYLINDRICAL_SURFACE ( 'NONE', #16530, 5.000000000000000000 ) ;
#40946=CARTESIAN_POINT ( 'NONE',  ( -5.000000000000000000, 6.916666666666664298, -2.886751345948128211 ) ) ;
#40948=CARTESIAN_POINT ( 'NONE',  ( -4.458734124999999437, -55.31249999863440081, 0.000000000000000000 ) ) ;
#40949=CARTESIAN_POINT ( 'NONE',  ( -4.458734124999998549, -12.22916666530106866, 2.574251347313722516 ) ) ;
#40951=EDGE_CURVE ( 'NONE', #53830, #46451, #51741, .T. ) ;
#40954=CYLINDRICAL_SURFACE ( 'NONE', #51258, 5.000000000000000000 ) ;
#40955=CARTESIAN_POINT ( 'NONE',  ( -4.999999999999998224, -36.91666666666667140, 2.886751345948131764 ) ) ;
#40958=CARTESIAN_POINT ( 'NONE',  ( 1.060575238724906964E-15, -34.75000000000000711, 5.773502691896257311 ) ) ;
#40963=CARTESIAN_POINT ( 'NONE',  ( 4.458734124999998549, -61.72916666530106511, -2.574251347313721627 ) ) ;
#40964=CARTESIAN_POINT ( 'NONE',  ( 1.846868145590735200, -153.5000000013656063, -4.458734125000000326 ) ) ;
#40965=CARTESIAN_POINT ( 'NONE',  ( -2.229367062500000163, -70.47916666530107932, -3.861377020970580443 ) ) ;
#40969=CARTESIAN_POINT ( 'NONE',  ( -2.499999999999996447, -61.70833333060214443, 4.330127018922195425 ) ) ;
#40970=ORIENTED_EDGE ( 'NONE', *, *, #13335, .T. ) ;
#40972=ORIENTED_EDGE ( 'NONE', *, *, #34250, .T. ) ;
#40975=CARTESIAN_POINT ( 'NONE',  ( -1.846868145590737420, -151.7500000013655779, 4.458734124999999437 ) ) ;
#40977=ORIENTED_EDGE ( 'NONE', *, *, #56305, .T. ) ;
#40979=EDGE_CURVE ( 'NONE', #8963, #12432, #37126, .T. ) ;
#40981=CARTESIAN_POINT ( 'NONE',  ( 5.000000000000000888, -54.58333333333332860, 2.886751345948126879 ) ) ;
#40983=CARTESIAN_POINT ( 'NONE',  ( 4.458734124999999437, -47.06249999863440792, -5.460374474430324690E-16 ) ) ;
#40985=CARTESIAN_POINT ( 'NONE',  ( -4.999999999999998224, 17.20833333606451987, 2.886751345948131764 ) ) ;
#40987=CARTESIAN_POINT ( 'NONE',  ( 4.458734124999998549, 24.27083333469892779, -2.574251347313721627 ) ) ;
#40990=FACE_OUTER_BOUND ( 'NONE', #3278, .T. ) ;
#40991=VERTEX_POINT ( 'NONE', #20590 ) ;
#40995=CARTESIAN_POINT ( 'NONE',  ( -6.972266317189433020E-16, -75.25000000000000000, -5.000000000000000000 ) ) ;
#41000=CARTESIAN_POINT ( 'NONE',  ( -6.972266317189433020E-16, -20.12499999726881228, -5.000000000000000000 ) ) ;
#41004=VERTEX_POINT ( 'NONE', #53713 ) ;
#41007=CARTESIAN_POINT ( 'NONE',  ( 3.535533905932738197, -158.0000000027312126, -3.535533905932738197 ) ) ;
#41008=VERTEX_POINT ( 'NONE', #650 ) ;
#41017=CARTESIAN_POINT ( 'NONE',  ( -2.229367062500000163, -21.47916666530107221, -3.861377020970580443 ) ) ;
#41018=CARTESIAN_POINT ( 'NONE',  ( 5.000000000000000000, -75.50000000000000000, -6.123233995736766282E-16 ) ) ;
#41019=CARTESIAN_POINT ( 'NONE',  ( 3.535533905932736864, -149.1250000000000000, 3.535533905932738641 ) ) ;
#41021=CARTESIAN_POINT ( 'NONE',  ( 3.152801135295367541, -153.3125000013656063, -3.152801135295367541 ) ) ;
#41022=ORIENTED_EDGE ( 'NONE', *, *, #33982, .F. ) ;
#41023=CARTESIAN_POINT ( 'NONE',  ( -3.152548672688508926E-16, -53.81249999863439371, -5.148502694627439702 ) ) ;
#41024=CARTESIAN_POINT ( 'NONE',  ( -6.972266317189433020E-16, -58.12499999726880162, -5.000000000000000000 ) ) ;
#41026=CARTESIAN_POINT ( 'NONE',  ( -3.152548672688508926E-16, -89.56249999863439371, -5.148502694627439702 ) ) ;
#41027=CARTESIAN_POINT ( 'NONE',  ( -2.229367062500000163, 5.520833334698927786, -3.861377020970580443 ) ) ;
#41028=CARTESIAN_POINT ( 'NONE',  ( -5.000000000000000000, -160.6250000027311842, -6.123233995736766282E-16 ) ) ;
#41029=LINE ( 'NONE', #10810, #53295 ) ;
#41031=CARTESIAN_POINT ( 'NONE',  ( -3.152548672688508926E-16, 17.18750000136559919, -5.148502694627439702 ) ) ;
#41032=CARTESIAN_POINT ( 'NONE',  ( 5.000000000000000000, 1.708333336064519425, -2.886751345948129988 ) ) ;
#41033=VERTEX_POINT ( 'NONE', #29575 ) ;
#41035=EDGE_LOOP ( 'NONE', ( #38052, #39501, #23027, #16870 ) ) ;
#41038=CARTESIAN_POINT ( 'NONE',  ( 4.458734124999998549, -45.72916666530106511, -2.574251347313721627 ) ) ;
#41039=CARTESIAN_POINT ( 'NONE',  ( -3.152801135295367096, -162.3125000013656063, -3.152801135295367541 ) ) ;
#41040=VECTOR ( 'NONE', #41428, 1000.000000000000000 ) ;
#41041=CARTESIAN_POINT ( 'NONE',  ( -3.535250795749689387E-16, -37.12499999726881583, -5.773502691896257311 ) ) ;
#41043=CARTESIAN_POINT ( 'NONE',  ( -4.458734124999998549, -16.22916666530107577, 2.574251347313722516 ) ) ;
#41046=CARTESIAN_POINT ( 'NONE',  ( 2.730187237215162345E-16, -165.1875000013655779, -4.458734124999999437 ) ) ;
#41047=CARTESIAN_POINT ( 'NONE',  ( -1.339745962155610925, -34.66965819600733312, 5.000000000000000000 ) ) ;
#41048=ORIENTED_EDGE ( 'NONE', *, *, #53478, .T. ) ;
#41050=CARTESIAN_POINT ( 'NONE',  ( 2.229367062499998831, -32.89583333196773651, -3.861377020970580887 ) ) ;
#41052=ORIENTED_EDGE ( 'NONE', *, *, #35438, .T. ) ;
#41053=EDGE_CURVE ( 'NONE', #41004, #14852, #23641, .T. ) ;
#41060=CARTESIAN_POINT ( 'NONE',  ( -4.458734124999999437, -78.56249999863440792, 0.000000000000000000 ) ) ;
#41063=CARTESIAN_POINT ( 'NONE',  ( -1.846868145590734756, -141.3750000013656063, -4.458734124999999437 ) ) ;
#41065=CARTESIAN_POINT ( 'NONE',  ( -2.229367062500000163, -46.47916666530106511, -3.861377020970580443 ) ) ;
#41071=CARTESIAN_POINT ( 'NONE',  ( -5.000000000000000000, -73.00000000000000000, 0.000000000000000000 ) ) ;
#41073=CARTESIAN_POINT ( 'NONE',  ( -2.229367062500000163, -81.72916666530106511, -3.861377020970580443 ) ) ;
#41078=ORIENTED_EDGE ( 'NONE', *, *, #31889, .T. ) ;
#41079=FACE_OUTER_BOUND ( 'NONE', #30878, .T. ) ;
#41084=CARTESIAN_POINT ( 'NONE',  ( 4.458734125000000326, 12.85416666803226171, 2.574251347313718519 ) ) ;
#41091=CARTESIAN_POINT ( 'NONE',  ( 9.457646018065525792E-16, -88.06249999863439371, 5.148502694627439702 ) ) ;
#41092=CARTESIAN_POINT ( 'NONE',  ( -4.458734124999999437, -2.395833331967737845, -2.574251347313719407 ) ) ;
#41094=ORIENTED_EDGE ( 'NONE', *, *, #9370, .F. ) ;
#41095=CARTESIAN_POINT ( 'NONE',  ( -4.458734124999999437, -30.56249999863440436, 0.000000000000000000 ) ) ;
#41100=( BOUNDED_CURVE ( )  B_SPLINE_CURVE ( 2, ( #17096, #61173, #22247, #61492, #21611, #51825, #7766, #12272, #42166 ),
 .UNSPECIFIED., .F., .F. ) 
 B_SPLINE_CURVE_WITH_KNOTS ( ( 3, 2, 2, 2, 3 ),
 ( 0.3770833333333333259, 0.3777777777777777679, 0.3791666666666666519, 0.3805555555555555358, 0.3812499999999999778 ),
 .UNSPECIFIED. ) 
 CURVE ( )  GEOMETRIC_REPRESENTATION_ITEM ( )  RATIONAL_B_SPLINE_CURVE ( ( 0.9330127018922194093, 0.9330127018922194093, 1.000000000000000000, 0.8660254037844387076, 1.000000000000000000, 0.8660254037844387076, 1.000000000000000000, 0.9330127018922194093, 0.9330127018922194093 ) ) 
 REPRESENTATION_ITEM ( '' )  );
#41101=CARTESIAN_POINT ( 'NONE',  ( -2.229367062500000163, 22.52083333469892423, -3.861377020970580443 ) ) ;
#41103=CARTESIAN_POINT ( 'NONE',  ( -4.999999999999998224, -25.79166666393547658, 2.886751345948131764 ) ) ;
#41104=CARTESIAN_POINT ( 'NONE',  ( -4.458734124999997661, -77.47916666530106511, 2.574251347313722516 ) ) ;
#41107=CARTESIAN_POINT ( 'NONE',  ( -2.500000000000000444, 19.95833333606451987, -4.330127018922193649 ) ) ;
#41108=ORIENTED_EDGE ( 'NONE', *, *, #54683, .T. ) ;
#41109=CARTESIAN_POINT ( 'NONE',  ( -3.535533905932737309, -168.7500000027312126, -3.535533905932738197 ) ) ;
#41111=CARTESIAN_POINT ( 'NONE',  ( 1.060575238724906964E-15, -22.75000000000000000, 5.773502691896257311 ) ) ;
#41112=CARTESIAN_POINT ( 'NONE',  ( -2.229367062500000163, -29.47916666530107221, -3.861377020970580443 ) ) ;
#41113=CARTESIAN_POINT ( 'NONE',  ( -4.458734124999999437, -89.31249999863440792, 0.000000000000000000 ) ) ;
#41114=CARTESIAN_POINT ( 'NONE',  ( 5.000000000000000888, -25.45833333060214443, 2.886751345948126879 ) ) ;
#41115=CARTESIAN_POINT ( 'NONE',  ( 2.229367062499998831, -56.64583333196773651, -3.861377020970580887 ) ) ;
#41117=CARTESIAN_POINT ( 'NONE',  ( 0.000000000000000000, -170.0000000000000000, 5.000000000000000000 ) ) ;
#41119=CARTESIAN_POINT ( 'NONE',  ( 4.458734124999999437, -4.062499998634408804, -5.460374474430324690E-16 ) ) ;
#41121=CARTESIAN_POINT ( 'NONE',  ( -2.500000000000000444, -71.16666666666667140, -4.330127018922193649 ) ) ;
#41125=CARTESIAN_POINT ( 'NONE',  ( 3.061616997868383141E-16, -159.7500000000000000, -5.000000000000000000 ) ) ;
#41126=CARTESIAN_POINT ( 'NONE',  ( 2.500000000000002220, -72.54166666393548724, 4.330127018922192761 ) ) ;
#41130=CARTESIAN_POINT ( 'NONE',  ( -3.152548672688508926E-16, -16.81249999863440436, -5.148502694627439702 ) ) ;
#41131=CARTESIAN_POINT ( 'NONE',  ( 4.458734124999999437, -54.06249999863440081, -5.460374474430324690E-16 ) ) ;
#41133=CARTESIAN_POINT ( 'NONE',  ( -4.458734125000000326, -144.0000000013655779, -1.846868145590735644 ) ) ;
#41135=CARTESIAN_POINT ( 'NONE',  ( 6.123233995736766282E-16, -170.0000000000000000, -5.000000000000000000 ) ) ;
#41137=CARTESIAN_POINT ( 'NONE',  ( -9.184850993605147944E-16, -155.2500000000000000, 5.000000000000000000 ) ) ;
#41138=CARTESIAN_POINT ( 'NONE',  ( -4.458734124999999437, 27.43750000136559208, 0.000000000000000000 ) ) ;
#41142=CARTESIAN_POINT ( 'NONE',  ( -4.458734125000001214, -149.1250000013656063, 1.846868145590734089 ) ) ;
#41144=( BOUNDED_CURVE ( )  B_SPLINE_CURVE ( 2, ( #31963, #17501, #22646, #57688, #61567, #56742, #8167, #47701, #8476 ),
 .UNSPECIFIED., .F., .F. ) 
 B_SPLINE_CURVE_WITH_KNOTS ( ( 3, 2, 2, 2, 3 ),
 ( 0.4187500000000000111, 0.4194444444444444531, 0.4208333333333333370, 0.4222222222222222210, 0.4229166666666666630 ),
 .UNSPECIFIED. ) 
 CURVE ( )  GEOMETRIC_REPRESENTATION_ITEM ( )  RATIONAL_B_SPLINE_CURVE ( ( 0.9330127018922194093, 0.9330127018922194093, 1.000000000000000000, 0.8660254037844387076, 1.000000000000000000, 0.8660254037844387076, 1.000000000000000000, 0.9330127018922194093, 0.9330127018922194093 ) ) 
 REPRESENTATION_ITEM ( '' )  );
#41145=CARTESIAN_POINT ( 'NONE',  ( -4.458734124999999437, -65.56249999863440792, 0.000000000000000000 ) ) ;
#41146=CARTESIAN_POINT ( 'NONE',  ( -1.339745962155613812, -84.08034179853027013, -5.000000000000000000 ) ) ;
#41147=CARTESIAN_POINT ( 'NONE',  ( 2.229367062499998831, -6.645833331967741842, -3.861377020970580887 ) ) ;
#41149=CARTESIAN_POINT ( 'NONE',  ( 4.458734124999999437, -146.3750000013655779, -1.846868145590734978 ) ) ;
#41156=EDGE_CURVE ( 'NONE', #35439, #44817, #35097, .T. ) ;
#41164=CARTESIAN_POINT ( 'NONE',  ( 4.458734124999999437, 12.18750000136559564, -5.460374474430324690E-16 ) ) ;
#41167=CARTESIAN_POINT ( 'NONE',  ( 2.229367062500001939, -15.22916666530107399, 3.861377020970579999 ) ) ;
#41169=CARTESIAN_POINT ( 'NONE',  ( -4.458734125000000326, -162.0000000013655779, -1.846868145590735644 ) ) ;
#41170=CARTESIAN_POINT ( 'NONE',  ( -1.339745962155613812, -38.20534180126147561, -5.000000000000000000 ) ) ;
#41174=DIRECTION ( 'NONE',  ( -0.000000000000000000, 1.000000000000000000, -0.000000000000000000 ) ) ;
#41176=CARTESIAN_POINT ( 'NONE',  ( -2.229367062499996610, -33.14583333196772941, 3.861377020970582219 ) ) ;
#41180=DIRECTION ( 'NONE',  ( -0.000000000000000000, 1.000000000000000000, -0.000000000000000000 ) ) ;
#41185=DIRECTION ( 'NONE',  ( -0.000000000000000000, 1.000000000000000000, -0.000000000000000000 ) ) ;
#41186=CARTESIAN_POINT ( 'NONE',  ( -2.500000000000000444, -9.166666666666662522, -4.330127018922193649 ) ) ;
#41187=CARTESIAN_POINT ( 'NONE',  ( -2.229367062499996610, -74.14583333196773651, 3.861377020970582219 ) ) ;
#41188=FACE_OUTER_BOUND ( 'NONE', #61778, .T. ) ;
#41189=CARTESIAN_POINT ( 'NONE',  ( -4.999999999999999112, -9.791666663935476578, 2.886751345948131764 ) ) ;
#41190=CARTESIAN_POINT ( 'NONE',  ( 4.458734124999998549, -40.72916666530107221, -2.574251347313721627 ) ) ;
#41193=CARTESIAN_POINT ( 'NONE',  ( -3.152548672688508926E-16, 13.18750000136559208, -5.148502694627439702 ) ) ;
#41195=LINE ( 'NONE', #55699, #28907 ) ;
#41196=CARTESIAN_POINT ( 'NONE',  ( -3.535250795749689387E-16, -55.24999999999998579, -5.773502691896257311 ) ) ;
#41199=CARTESIAN_POINT ( 'NONE',  ( -2.229367062499996610, -78.14583333196773651, 3.861377020970582219 ) ) ;
#41200=( BOUNDED_CURVE ( )  B_SPLINE_CURVE ( 2, ( #861, #20464, #11748, #61618, #32330, #57112, #12713, #60668, #42296 ),
 .UNSPECIFIED., .F., .F. ) 
 B_SPLINE_CURVE_WITH_KNOTS ( ( 3, 2, 2, 2, 3 ),
 ( 0.2687499999999999889, 0.2694444444444444309, 0.2708333333333333148, 0.2722222222222221988, 0.2729166666666666963 ),
 .UNSPECIFIED. ) 
 CURVE ( )  GEOMETRIC_REPRESENTATION_ITEM ( )  RATIONAL_B_SPLINE_CURVE ( ( 0.9330127018922194093, 0.9330127018922194093, 1.000000000000000000, 0.8660254037844387076, 1.000000000000000000, 0.8660254037844387076, 1.000000000000000000, 0.9330127018922167448, 0.9330127018922194093 ) ) 
 REPRESENTATION_ITEM ( '' )  );
#41201=CARTESIAN_POINT ( 'NONE',  ( -1.846868145590737420, -142.0000000013655495, 4.458734124999999437 ) ) ;
#41202=CARTESIAN_POINT ( 'NONE',  ( 9.457646018065525792E-16, -88.06249999863439371, 5.148502694627439702 ) ) ;
#41204=CARTESIAN_POINT ( 'NONE',  ( 2.229367062499998831, -33.89583333196772941, -3.861377020970580887 ) ) ;
#41205=VERTEX_POINT ( 'NONE', #34089 ) ;
#41207=CARTESIAN_POINT ( 'NONE',  ( 1.975475456537005874E-15, -84.74999999999998579, 5.000000000000000000 ) ) ;
#41209=CARTESIAN_POINT ( 'NONE',  ( -2.499999999999996447, -3.708333330602147537, 4.330127018922195425 ) ) ;
#41210=CARTESIAN_POINT ( 'NONE',  ( -4.999999999999998224, -11.79166666393547835, 2.886751345948131764 ) ) ;
#41211=VECTOR ( 'NONE', #40643, 1000.000000000000000 ) ;
#41212=CARTESIAN_POINT ( 'NONE',  ( 4.458734125000001214, -66.14583333196772230, 2.574251347313718519 ) ) ;
#41214=ORIENTED_EDGE ( 'NONE', *, *, #16200, .F. ) ;
#41219=CARTESIAN_POINT ( 'NONE',  ( -3.152548672688508926E-16, 9.437500001365593860, -5.148502694627439702 ) ) ;
#41220=CARTESIAN_POINT ( 'NONE',  ( 1.975475456537005874E-15, -15.75000000000000000, 5.000000000000000000 ) ) ;
#41221=CARTESIAN_POINT ( 'NONE',  ( -4.458734124999999437, -157.0000000013655779, -1.846868145590735644 ) ) ;
#41225=CARTESIAN_POINT ( 'NONE',  ( 5.000000000000000000, -164.1250000027311842, 0.000000000000000000 ) ) ;
#41233=CARTESIAN_POINT ( 'NONE',  ( -2.229367062499996610, 28.85416666803226349, 3.861377020970582219 ) ) ;
#41236=CARTESIAN_POINT ( 'NONE',  ( -4.458734124999999437, 2.354166668032262599, -2.574251347313719407 ) ) ;
#41239=CARTESIAN_POINT ( 'NONE',  ( 5.000000000000000888, -145.0625000027311842, -2.071067811865475505 ) ) ;
#41241=ADVANCED_FACE ( 'NONE', ( #44048 ), #48568, .T. ) ;
#41247=EDGE_CURVE ( 'NONE', #57124, #60836, #32921, .T. ) ;
#41249=CARTESIAN_POINT ( 'NONE',  ( -8.190561711645485556E-16, -160.9375000013655779, 4.458734124999999437 ) ) ;
#41250=CARTESIAN_POINT ( 'NONE',  ( 5.000000000000000000, 7.583333333333333925, -2.886751345948130876 ) ) ;
#41252=CARTESIAN_POINT ( 'NONE',  ( 2.730187237215162345E-16, -140.1875000013656063, -4.458734124999999437 ) ) ;
#41253=EDGE_LOOP ( 'NONE', ( #35530, #51843, #40804, #42075 ) ) ;
#41254=CARTESIAN_POINT ( 'NONE',  ( 4.458734125000001214, 21.85416666803225993, 2.574251347313718519 ) ) ;
#41259=FACE_OUTER_BOUND ( 'NONE', #58303, .T. ) ;
#41260=CARTESIAN_POINT ( 'NONE',  ( -3.535250795749689387E-16, 7.749999999999999112, -5.773502691896257311 ) ) ;
#41261=CARTESIAN_POINT ( 'NONE',  ( -3.152548672688508926E-16, -58.56249999863439371, -5.148502694627439702 ) ) ;
#41262=CARTESIAN_POINT ( 'NONE',  ( 4.458734124999998549, -10.72916666530106866, -2.574251347313721627 ) ) ;
#41268=CARTESIAN_POINT ( 'NONE',  ( -3.535250795749689387E-16, -41.25000000000000000, -5.773502691896257311 ) ) ;
#41272=CARTESIAN_POINT ( 'NONE',  ( -4.999999999999998224, 13.08333333333333215, 2.886751345948131764 ) ) ;
#41273=CARTESIAN_POINT ( 'NONE',  ( 9.457646018065525792E-16, -61.06249999863440081, 5.148502694627439702 ) ) ;
#41274=CARTESIAN_POINT ( 'NONE',  ( 4.458734124999999437, -150.7500000013655779, 1.846868145590737864 ) ) ;
#41275=ADVANCED_FACE ( 'NONE', ( #39542 ), #32271, .T. ) ;
#41276=CARTESIAN_POINT ( 'NONE',  ( -4.458734124999998549, -70.22916666530107932, 2.574251347313722516 ) ) ;
#41279=CARTESIAN_POINT ( 'NONE',  ( -4.458734124999998549, -21.47916666530107221, 2.574251347313722516 ) ) ;
#41280=CARTESIAN_POINT ( 'NONE',  ( -2.499999999999996447, -62.70833333060214443, 4.330127018922195425 ) ) ;
#41281=ORIENTED_EDGE ( 'NONE', *, *, #17576, .T. ) ;
#41284=CARTESIAN_POINT ( 'NONE',  ( -2.071067811865580754, -157.8125000027312126, -4.999999999999894307 ) ) ;
#41286=ADVANCED_FACE ( 'NONE', ( #58214 ), #14142, .T. ) ;
#41287=CARTESIAN_POINT ( 'NONE',  ( 1.846868145590736310, -150.6250000013655779, 4.458734124999999437 ) ) ;
#41288=ORIENTED_EDGE ( 'NONE', *, *, #18953, .T. ) ;
#41291=CARTESIAN_POINT ( 'NONE',  ( -6.972266317189433020E-16, -53.12499999726880162, -5.000000000000000000 ) ) ;
#41292=CARTESIAN_POINT ( 'NONE',  ( 9.457646018065525792E-16, -49.31249999863441502, 5.148502694627439702 ) ) ;
#41295=CARTESIAN_POINT ( 'NONE',  ( -5.000000000000000000, -145.5000000000000284, -6.123233995736766282E-16 ) ) ;
#41297=CARTESIAN_POINT ( 'NONE',  ( 2.229367062499998831, 24.35416666803225993, -3.861377020970580887 ) ) ;
#41300=CARTESIAN_POINT ( 'NONE',  ( 5.000000000000000000, -61.29166666393548013, -2.886751345948130876 ) ) ;
#41303=CARTESIAN_POINT ( 'NONE',  ( -4.999999999999998224, 1.083333333333331927, 2.886751345948131764 ) ) ;
#41305=CARTESIAN_POINT ( 'NONE',  ( -1.127183054612291972E-14, 24.25000000000000000, 4.999999999999999112 ) ) ;
#41306=EDGE_CURVE ( 'NONE', #8603, #21511, #38825, .T. ) ;
#41308=EDGE_CURVE ( 'NONE', #34317, #42312, #23179, .T. ) ;
#41313=EDGE_CURVE ( 'NONE', #4948, #48755, #18351, .T. ) ;
#41316=ORIENTED_EDGE ( 'NONE', *, *, #36910, .F. ) ;
#41319=CARTESIAN_POINT ( 'NONE',  ( -3.535533905932737309, -158.7500000027312126, -3.535533905932738197 ) ) ;
#41326=CARTESIAN_POINT ( 'NONE',  ( -5.000000000000000888, -148.5625000000000000, -2.071067811865475949 ) ) ;
#41328=EDGE_CURVE ( 'NONE', #51921, #25405, #45419, .T. ) ;
#41331=CARTESIAN_POINT ( 'NONE',  ( 9.457646018065525792E-16, -27.06249999863440081, 5.148502694627439702 ) ) ;
#41332=CARTESIAN_POINT ( 'NONE',  ( -2.071067811865475061, -152.6875000000000284, -5.000000000000000888 ) ) ;
#41334=CARTESIAN_POINT ( 'NONE',  ( 3.152801135295367541, -151.3125000013655779, -3.152801135295367541 ) ) ;
#41335=EDGE_LOOP ( 'NONE', ( #59923, #58130, #15752, #47399 ) ) ;
#41337=CARTESIAN_POINT ( 'NONE',  ( -4.458734124999997661, -51.47916666530107932, 2.574251347313722516 ) ) ;
#41338=CARTESIAN_POINT ( 'NONE',  ( 0.000000000000000000, -170.0000000000000000, 0.000000000000000000 ) ) ;
#41340=EDGE_CURVE ( 'NONE', #32024, #25786, #52001, .T. ) ;
#41341=CARTESIAN_POINT ( 'NONE',  ( -5.000000000000000000, 26.00000000000000000, 0.000000000000000000 ) ) ;
#41343=CARTESIAN_POINT ( 'NONE',  ( 2.229367062500001939, 3.020833334698928674, 3.861377020970579999 ) ) ;
#41344=PLANE ( 'NONE',  #55477 ) ;
#41345=CARTESIAN_POINT ( 'NONE',  ( 2.499999999999998668, -41.20833333060214443, -4.330127018922193649 ) ) ;
#41347=CARTESIAN_POINT ( 'NONE',  ( 4.458734124999998549, 14.02083333469892779, -2.574251347313721627 ) ) ;
#41348=CARTESIAN_POINT ( 'NONE',  ( 5.000000000000000000, 2.625000002731185500, -6.123233995736766282E-16 ) ) ;
#41349=ORIENTED_EDGE ( 'NONE', *, *, #61815, .F. ) ;
#41350=CARTESIAN_POINT ( 'NONE',  ( 1.339745962155615588, 26.70534180126147561, -4.999999999999997335 ) ) ;
#41351=ORIENTED_EDGE ( 'NONE', *, *, #24496, .T. ) ;
#41354=CARTESIAN_POINT ( 'NONE',  ( 4.458734124999998549, -42.72916666530107221, -2.574251347313721627 ) ) ;
#41355=CARTESIAN_POINT ( 'NONE',  ( -4.458734124999999437, -162.1875000013655779, -5.460374474430324690E-16 ) ) ;
#41356=CARTESIAN_POINT ( 'NONE',  ( -2.500000000000000444, -46.04166666393547303, -4.330127018922193649 ) ) ;
#41358=CARTESIAN_POINT ( 'NONE',  ( 9.457646018065525792E-16, -19.06249999863440792, 5.148502694627439702 ) ) ;
#41359=EDGE_LOOP ( 'NONE', ( #26337, #4982, #31859, #49466 ) ) ;
#41360=CARTESIAN_POINT ( 'NONE',  ( -4.999999999999999112, -88.91666666666667140, 2.886751345948131764 ) ) ;
#41361=CARTESIAN_POINT ( 'NONE',  ( -3.152801135295367096, -165.0625000013656063, -3.152801135295367541 ) ) ;
#41362=CARTESIAN_POINT ( 'NONE',  ( 0.000000000000000000, -170.0000000000000000, 5.000000000000000000 ) ) ;
#41365=CARTESIAN_POINT ( 'NONE',  ( -3.152548672688508926E-16, -33.81249999863440792, -5.148502694627439702 ) ) ;
#41366=DIRECTION ( 'NONE',  ( -0.000000000000000000, 1.000000000000000000, -0.000000000000000000 ) ) ;
#41367=ORIENTED_EDGE ( 'NONE', *, *, #44726, .F. ) ;
#41372=LINE ( 'NONE', #60386, #19172 ) ;
#41374=CARTESIAN_POINT ( 'NONE',  ( -3.152548672688508926E-16, -78.81249999863440792, -5.148502694627439702 ) ) ;
#41376=CARTESIAN_POINT ( 'NONE',  ( 2.071067811865517694, -142.8124999999999716, -4.999999999999958256 ) ) ;
#41377=CARTESIAN_POINT ( 'NONE',  ( 4.458734124999997661, -141.7500000013655779, 1.846868145590737864 ) ) ;
#41379=CARTESIAN_POINT ( 'NONE',  ( 5.000000000000000000, 20.49999999999999645, -6.123233995736766282E-16 ) ) ;
#41381=CARTESIAN_POINT ( 'NONE',  ( -2.229367062499996610, -45.14583333196774362, 3.861377020970582219 ) ) ;
#41382=CARTESIAN_POINT ( 'NONE',  ( -4.999999999999998224, 21.08333333333333215, 2.886751345948131764 ) ) ;
#41384=CARTESIAN_POINT ( 'NONE',  ( 5.000000000000000888, -154.0625000027312126, -2.071067811865475505 ) ) ;
#41388=CARTESIAN_POINT ( 'NONE',  ( -5.000000000000000888, -153.6875000027312126, -2.071067811865475949 ) ) ;
#41390=CARTESIAN_POINT ( 'NONE',  ( 4.458734124999999437, -77.06249999863440792, -5.460374474430324690E-16 ) ) ;
#41391=CARTESIAN_POINT ( 'NONE',  ( 2.500000000000002220, -34.66666666666666430, 4.330127018922192761 ) ) ;
#41396=CARTESIAN_POINT ( 'NONE',  ( -6.972266317189433020E-16, -9.124999997268814056, -5.000000000000000000 ) ) ;
#41398=CARTESIAN_POINT ( 'NONE',  ( -5.000000000000000888, -168.5625000027312410, 2.071067811865474617 ) ) ;
#41400=CARTESIAN_POINT ( 'NONE',  ( -2.229367062499996610, 14.60416666803226171, 3.861377020970582219 ) ) ;
#41401=CARTESIAN_POINT ( 'NONE',  ( 0.000000000000000000, -170.0000000000000000, 0.000000000000000000 ) ) ;
#41406=CARTESIAN_POINT ( 'NONE',  ( 1.339745962155612702, -38.16965819600732601, -5.000000000000000000 ) ) ;
#41407=CARTESIAN_POINT ( 'NONE',  ( 4.458734125000001214, -84.89583333196773651, 2.574251347313718519 ) ) ;
#41408=CARTESIAN_POINT ( 'NONE',  ( -3.152548672688508926E-16, -10.56249999863440792, -5.148502694627439702 ) ) ;
#41411=ORIENTED_EDGE ( 'NONE', *, *, #62460, .F. ) ;
#41412=CARTESIAN_POINT ( 'NONE',  ( -2.229367062499996610, -33.39583333196772941, 3.861377020970582219 ) ) ;
#41414=EDGE_CURVE ( 'NONE', #32917, #29720, #52754, .T. ) ;
#41417=CARTESIAN_POINT ( 'NONE',  ( 9.457646018065525792E-16, 17.93750000136559208, 5.148502694627439702 ) ) ;
#41419=CARTESIAN_POINT ( 'NONE',  ( 6.123233995736766282E-16, -170.0000000000000000, -5.000000000000000000 ) ) ;
#41420=CARTESIAN_POINT ( 'NONE',  ( -5.000000000000000000, -145.6250000027312126, -6.123233995736766282E-16 ) ) ;
#41421=CARTESIAN_POINT ( 'NONE',  ( 4.458734125000000326, -85.14583333196773651, 2.574251347313718519 ) ) ;
#41424=CARTESIAN_POINT ( 'NONE',  ( -5.000000000000000000, 21.12500000273118417, 0.000000000000000000 ) ) ;
#41425=VERTEX_POINT ( 'NONE', #10277 ) ;
#41427=CARTESIAN_POINT ( 'NONE',  ( -3.535533905932738641, -168.5000000027312126, 3.535533905932737309 ) ) ;
#41428=DIRECTION ( 'NONE',  ( -0.000000000000000000, -1.000000000000000000, -0.000000000000000000 ) ) ;
#41429=CARTESIAN_POINT ( 'NONE',  ( -3.535250795749689387E-16, -26.25000000000000355, -5.773502691896257311 ) ) ;
#41430=CARTESIAN_POINT ( 'NONE',  ( -2.229367062499996610, -29.14583333196774007, 3.861377020970582219 ) ) ;
#41431=CARTESIAN_POINT ( 'NONE',  ( -3.152548672688508926E-16, -87.56249999863440792, -5.148502694627439702 ) ) ;
#41432=CARTESIAN_POINT ( 'NONE',  ( -5.000000000000000000, -30.87499999726881228, 0.000000000000000000 ) ) ;
#41433=CARTESIAN_POINT ( 'NONE',  ( -4.458734124999998549, -53.22916666530107932, 2.574251347313722516 ) ) ;
#41434=ORIENTED_EDGE ( 'NONE', *, *, #50790, .F. ) ;
#41436=CARTESIAN_POINT ( 'NONE',  ( -4.458734124999998549, -1.479166665301071770, 2.574251347313722516 ) ) ;
#41438=CARTESIAN_POINT ( 'NONE',  ( 1.060575238724906964E-15, -73.75000000000000000, 5.773502691896257311 ) ) ;
#41442=CARTESIAN_POINT ( 'NONE',  ( 5.000000000000000888, -71.45833333060214443, 2.886751345948126879 ) ) ;
#41445=CARTESIAN_POINT ( 'NONE',  ( -4.458734124999999437, -16.64583333196773651, -2.574251347313719407 ) ) ;
#41446=CARTESIAN_POINT ( 'NONE',  ( -4.458734124999999437, -49.64583333196772941, -2.574251347313719407 ) ) ;
#41448=CARTESIAN_POINT ( 'NONE',  ( 3.152801135295367541, -141.3125000013655779, -3.152801135295367541 ) ) ;
#41450=CARTESIAN_POINT ( 'NONE',  ( 3.535533905932738197, -157.8750000000000284, -3.535533905932738197 ) ) ;
#41453=CARTESIAN_POINT ( 'NONE',  ( 2.229367062500001939, 25.77083333469892779, 3.861377020970579999 ) ) ;
#41455=CARTESIAN_POINT ( 'NONE',  ( -1.339745962155610925, -12.66965819600733134, 5.000000000000000000 ) ) ;
#41459=CARTESIAN_POINT ( 'NONE',  ( 1.846868145590736310, -148.8750000013655495, 4.458734124999999437 ) ) ;
#41462=CARTESIAN_POINT ( 'NONE',  ( 2.229367062499998831, -64.89583333196773651, -3.861377020970580887 ) ) ;
#41463=CARTESIAN_POINT ( 'NONE',  ( -3.535533905932737309, -154.7500000027312126, -3.535533905932738197 ) ) ;
#41465=CARTESIAN_POINT ( 'NONE',  ( -8.190561711645485556E-16, -143.6875000013656063, 4.458734124999999437 ) ) ;
#41467=ORIENTED_EDGE ( 'NONE', *, *, #48806, .T. ) ;
#41469=CARTESIAN_POINT ( 'NONE',  ( 2.500000000000002220, 16.33333333333333215, 4.330127018922192761 ) ) ;
#41472=CARTESIAN_POINT ( 'NONE',  ( -4.458734124999999437, 29.35416666803225993, -2.574251347313719407 ) ) ;
#41473=CARTESIAN_POINT ( 'NONE',  ( -5.000000000000000000, -5.999999999999998224, 0.000000000000000000 ) ) ;
#41474=( BOUNDED_CURVE ( )  B_SPLINE_CURVE ( 2, ( #4675, #24297, #63549, #34255, #53884, #54848, #6596, #16565, #41000 ),
 .UNSPECIFIED., .F., .F. ) 
 B_SPLINE_CURVE_WITH_KNOTS ( ( 3, 2, 2, 2, 3 ),
 ( 0.4062500000000000000, 0.4069444444444444420, 0.4083333333333333259, 0.4097222222222222099, 0.4104166666666666519 ),
 .UNSPECIFIED. ) 
 CURVE ( )  GEOMETRIC_REPRESENTATION_ITEM ( )  RATIONAL_B_SPLINE_CURVE ( ( 0.9330127018922194093, 0.9330127018922194093, 1.000000000000000000, 0.8660254037844387076, 1.000000000000000000, 0.8660254037844387076, 1.000000000000000000, 0.9330127018922194093, 0.9330127018922194093 ) ) 
 REPRESENTATION_ITEM ( '' )  );
#41477=CARTESIAN_POINT ( 'NONE',  ( 3.535533905932738197, -150.0000000027312126, -3.535533905932738197 ) ) ;
#41480=DIRECTION ( 'NONE',  ( 0.000000000000000000, 0.000000000000000000, 1.000000000000000000 ) ) ;
#41481=CARTESIAN_POINT ( 'NONE',  ( -2.229367062499996610, 13.85416666803226171, 3.861377020970582219 ) ) ;
#41483=CARTESIAN_POINT ( 'NONE',  ( 2.229367062500001939, -21.22916666530107221, 3.861377020970579999 ) ) ;
#41485=CARTESIAN_POINT ( 'NONE',  ( -4.458734125000000326, -160.0000000013656063, -1.846868145590735644 ) ) ;
#41486=CARTESIAN_POINT ( 'NONE',  ( -1.339745962155613812, -41.08034179853029144, -5.000000000000000000 ) ) ;
#41490=CARTESIAN_POINT ( 'NONE',  ( -5.000000000000000000, -36.08333333333332860, -2.886751345948128211 ) ) ;
#41491=CARTESIAN_POINT ( 'NONE',  ( -4.458734124999997661, -34.22916666530107221, 2.574251347313722516 ) ) ;
#41495=CARTESIAN_POINT ( 'NONE',  ( 5.000000000000000000, -152.1250000027312126, 0.000000000000000000 ) ) ;
#41500=CARTESIAN_POINT ( 'NONE',  ( 5.000000000000000888, -5.583333333333336590, 2.886751345948126879 ) ) ;
#41501=CARTESIAN_POINT ( 'NONE',  ( 2.229367062499998831, -73.64583333196773651, -3.861377020970580887 ) ) ;
#41503=CARTESIAN_POINT ( 'NONE',  ( -3.535250795749689387E-16, -8.124999997268814056, -5.773502691896257311 ) ) ;
#41504=CARTESIAN_POINT ( 'NONE',  ( 2.229367062500001939, -38.97916666530107221, 3.861377020970579999 ) ) ;
#41505=EDGE_LOOP ( 'NONE', ( #26099, #226, #51989, #19907 ) ) ;
#41507=CARTESIAN_POINT ( 'NONE',  ( -2.229367062499996610, 12.60416666803226171, 3.861377020970582219 ) ) ;
#41510=CARTESIAN_POINT ( 'NONE',  ( 5.000000000000000000, -57.49999999999999289, -6.123233995736766282E-16 ) ) ;
#41511=CARTESIAN_POINT ( 'NONE',  ( -1.846868145590734756, -159.3750000013656347, -4.458734125000000326 ) ) ;
#41514=CARTESIAN_POINT ( 'NONE',  ( -4.458734124999999437, -80.39583333196772230, -2.574251347313719407 ) ) ;
#41515=CARTESIAN_POINT ( 'NONE',  ( -3.152801135295367096, -141.3125000013655779, -3.152801135295367541 ) ) ;
#41516=CARTESIAN_POINT ( 'NONE',  ( 4.458734124999999437, -85.81249999863439371, -5.460374474430324690E-16 ) ) ;
#41519=CARTESIAN_POINT ( 'NONE',  ( -4.458734124999998549, -2.479166665301069550, 2.574251347313722516 ) ) ;
#41520=CARTESIAN_POINT ( 'NONE',  ( -2.229367062500000163, -33.72916666530107221, -3.861377020970580443 ) ) ;
#41523=CARTESIAN_POINT ( 'NONE',  ( 5.000000000000000000, -84.41666666666667140, -2.886751345948130876 ) ) ;
#41528=DIRECTION ( 'NONE',  ( -0.000000000000000000, 1.000000000000000000, -0.000000000000000000 ) ) ;
#41529=CARTESIAN_POINT ( 'NONE',  ( -4.458734124999999437, -66.56249999863440792, 0.000000000000000000 ) ) ;
#41531=ORIENTED_EDGE ( 'NONE', *, *, #32613, .T. ) ;
#41534=CARTESIAN_POINT ( 'NONE',  ( -1.339745962155636017, 3.205341801261477386, 4.999999999999985789 ) ) ;
#41535=CARTESIAN_POINT ( 'NONE',  ( 4.458734125000001214, 8.104166668032261711, 2.574251347313718519 ) ) ;
#41536=CARTESIAN_POINT ( 'NONE',  ( 3.535533905932738197, -153.8750000000000000, -3.535533905932738197 ) ) ;
#41537=CARTESIAN_POINT ( 'NONE',  ( 3.152801135295367541, -156.3125000013656063, -3.152801135295367541 ) ) ;
#41538=CARTESIAN_POINT ( 'NONE',  ( 0.000000000000000000, -170.0000000000000000, 0.000000000000000000 ) ) ;
#41539=ORIENTED_EDGE ( 'NONE', *, *, #41607, .T. ) ;
#41544=AXIS2_PLACEMENT_3D ( 'NONE', #14290, #19433, #59641 ) ;
#41549=CARTESIAN_POINT ( 'NONE',  ( 9.457646018065525792E-16, 28.93750000136558853, 5.148502694627439702 ) ) ;
#41552=CARTESIAN_POINT ( 'NONE',  ( -2.229367062500000163, 2.270833334698928230, -3.861377020970580443 ) ) ;
#41555=CARTESIAN_POINT ( 'NONE',  ( 3.535533905932738197, -141.0000000027311842, -3.535533905932738197 ) ) ;
#41556=CARTESIAN_POINT ( 'NONE',  ( 2.071067811865582087, -159.1875000000000000, 4.999999999999894307 ) ) ;
#41561=CARTESIAN_POINT ( 'NONE',  ( -5.000000000000000000, -88.00000000000000000, 0.000000000000000000 ) ) ;
#41563=CARTESIAN_POINT ( 'NONE',  ( -1.846868145590734756, -160.3750000013655779, -4.458734124999999437 ) ) ;
#41566=ORIENTED_EDGE ( 'NONE', *, *, #59421, .T. ) ;
#41567=CARTESIAN_POINT ( 'NONE',  ( 4.458734125000001214, 16.85416666803225638, 2.574251347313718519 ) ) ;
#41568=ORIENTED_EDGE ( 'NONE', *, *, #16235, .T. ) ;
#41573=( BOUNDED_CURVE ( )  B_SPLINE_CURVE ( 2, ( #51232, #46077, #6846, #21640, #16805, #60880, #7169, #2035, #25499, #41549, #41233, #26778, #36425, #46396, #36748, #55420, #31917, #56053, #60565, #45439, #55094, #31599, #2345, #59934, #56378, #21953, #61200, #1083, #15855, #1402, #35478, #30641, #50263, #6211, #25824, #26140, #21003, #40608, #60253, #11338, #36111, #30961, #1712, #21321, #40922, #16490, #55734, #11650, #50904, #46710, #3918, #17759, #47032, #12612, #13871, #28035, #52497, #51856, #37687, #47963, #27093, #7480, #23537, #47652, #8738, #3606, #52802, #18696, #61838, #51544, #23214, #42509, #27401, #37073, #27720, #43136, #18389, #7799, #57009, #42824, #38008, #62469, #2982, #28346, #57641, #62776, #13569, #33187, #52172, #41875, #38321, #2655, #22274, #18065, #57950, #61522, #13245, #17452, #57329, #22916, #56696, #32225, #22599, #42196, #37376, #12924, #32546, #8116, #47347, #8431, #3296, #32868, #62147, #9049, #29924, #25105, #29277, #48907, #49549, #63406, #33807, #15138, #43761, #28659, #38619, #14493, #38938, #29602, #48592, #4852, #24472, #19323, #19006, #44078, #356, #58574, #4533, #33495, #34115, #49232, #34760, #48275, #19642, #59534, #44397, #19958, #53736, #54052, #5174, #43449, #24791, #9989, #4231, #39569, #59209, #9669, #54386, #678, #14180, #10311, #5491, #39252, #42, #58878, #14809, #23846, #34423, #63094, #58255, #53423, #53113, #9357, #44715, #20287, #39888, #28969, #24158, #35085, #36354, #16098, #26708, #31204, #26385, #6774, #16737, #16421, #31518, #6460, #59857, #60811, #41481, #6138, #60176, #15782, #49861, #50520, #36039, #26069, #40222, #15467, #46002, #1967, #35398, #20930, #11585, #21568, #2281, #20615, #45687, #10625, #41164, #1644, #5809, #35721, #55670, #55984, #54705, #55351, #11898, #30238, #51161, #40850, #25426, #21243, #60493, #7094, #45045, #50834, #1012, #46323, #21885, #55020, #11265, #10942, #30561, #50186, #25752, #45366, #1333, #30889, #40535, #36672, #22843, #17989, #61132, #2586, #42750, #7729, #56302, #22205, #42121, #2910, #57256, #12538, #12855, #52103, #27334, #46641, #56934, #27959, #22525, #47582, #52730, #8358, #12230, #41804, #31844, #47276, #23467, #3533, #23142, #46965, #37615, #13173, #7413, #32797, #52426, #51476, #62393, #18314, #61763, #32151, #17377, #51787, #3225, #37305, #42433, #17690, #32474, #8044, #27023, #27649, #61448, #36998, #56624, #17055, #62075, #8662, #37939, #57571, #13497, #33113, #3846, #28274, #47889, #44004, #58808, #53986, #34355, #44324, #63651, #57877, #49157, #48209, #13802, #54304, #49481, #53352, #34047, #33734, #33422, #43686, #15071, #62708, #288, #63333, #10245, #34684, #9914, #53669, #29210, #48835, #59136, #9602, #23779, #24720, #5419, #9287, #24091, #43381, #53040, #19570, #4775, #18933, #28588, #19250, #29849, #29523, #63026, #48523, #39182, #5102, #43070, #4163, #24402, #38256, #19887, #14425, #8978, #38864, #14739, #39500, #18634, #38549, #58180, #14109, #28903, #4464, #58501, #30817, #60102, #31131, #39818, #40778, #606, #60423, #11195, #26305, #1257, #25357, #45613, #44975, #50449, #21494, #20216, #41092, #16660, #20860, #40463, #60739, #54948, #941, #11515, #36286, #25035, #16023, #16348, #20544, #55276, #10875, #30492, #35650, #35327, #10554, #6389, #55596, #50114, #59785, #44646, #6069, #21169, #6699, #55909, #15710, #59459, #25683, #25994, #35970, #50754, #1569, #45928, #1890, #11820, #15391, #31439, #51082, #45292, #35016, #54630, #5739, #30164, #49794, #40141, #27259, #7655, #51714, #36916, #27568, #22766, #16980, #42361, #8280, #22127, #36591, #62000, #17618, #41720, #26953, #61370, #12778, #46885, #32400, #32077, #2829, #22447, #46248, #37234, #56227, #12148, #46570, #26628, #61687, #17292, #21813, #56860, #31768, #42045, #13414, #52346, #47201, #7969, #17920, #37541, #57180, #27884, #3145, #2209, #42675, #13099, #47506, #32717, #52026, #7341, #41408, #3456, #23070, #62314, #51400, #7020, #18239, #37863, #61060, #57496, #33036, #2510, #56547, #12466, #48133, #9827, #58731, #53901, #23393, #9212, #53591, #39103, #52652, #28825, #49071, #3769, #29438, #8899, #9521, #43304, #24637, #5018, #19166, #14657, #47812, #44244, #18854, #4084, #48446, #52962, #29128, #8587, #208, #62940, #4693, #4386, #38474, #23707, #28197, #14349, #48751, #42993, #57801, #34276, #58101, #62635, #13723, #33659, #24315, #14030, #24005, #43608, #53277, #38179, #63250, #19489, #38783, #58422, #18557, #33971, #43922, #19806, #39415, #63569, #33347, #59053, #14981, #28515, #6615, #54221, #55518, #35248, #45848, #26228, #45528, #45210, #20776, #40381, #50673, #25597, #15306, #16269, #60660, #25273, #15631, #34928, #5342, #5992, #1176, #10472, #20133, #10798, #1810, #1489, #54549, #40056, #30737, #21092, #21414, #39732, #60022, #29764, #25910, #15945, #24960, #54867, #35567, #40696, #10159, #44565, #55191, #60341, #11112, #50358, #49398, #6306, #35888, #11432, #523, #31050, #59372, #41017, #34590, #30085, #30410, #49715, #5660, #44894, #854, #20457, #59699, #50034, #8206, #12392, #32006, #32639, #46489, #16898, #3071, #13021, #16584, #51640, #32320, #36514, #46802, #2437, #22046, #61610, #26876, #2132, #7574, #47123, #41639, #51325, #36204, #61291, #12705, #61928, #52269, #7263, #51000, #17213, #2749, #27494, #51951, #27186, #22368, #36840, #37164, #11741, #7890, #56787, #56470, #22688, #47434, #60977, #42288, #27809, #41968, #17544, #17847, #37470, #31359, #57103, #21735, #6940, #3386, #23003, #41331, #42604, #55826, #26551, #46171, #56145, #12065, #31690, #57418, #47743, #13339, #48371, #24564, #9444, #29053, #28441, #19089, #14274, #8515, #33893, #63492, #13653, #28125, #53515, #9137, #33273, #18481, #52892, #4313, #38405, #23933, #23630, #43225, #18778, #37788, #28745, #3699, #23314, #38103, #18160, #53203, #8828, #32959, #43534, #42914, #58028, #4941, #43846, #38707, #63178, #48677, #4617, #24242, #19417, #58346, #52584, #34202, #39031, #58658, #14580, #62866, #62562, #57727, #33584, #53825, #9754, #48056, #62242, #29361, #48994, #4009, #13957, #1978, #41176, #56316, #36364, #40547, #2292, #51172, #46335, #14901, #1655, #46015, #31532, #44169, #21255, #41491, #58974, #21894, #448, #21579, #35735, #17065, #61143, #11594, #7105, #39343, #36682, #11276, #60188, #40861, #44487, #60822, #136, #12240, #55363, #16747, #60505, #30902, #16109, #19730, #6786, #55995, #34510, #49322, #26719, #50529, #54141, #5266, #26080, #31215, #6472, #45699, #26395, #10080, #16432, #31852, #36052, #51486, #50844, #11909, #7424, #55680, #24886, #29691, #20945, #22535, #56944, #51796, #41812, #13183, #47285, #27342, #56634, #52112, #57581, #27969, #7738, #17699, #32806, #47591, #8670, #12549, #3235, #2596, #52435, #27658, #61458, #32483, #37624, #27033, #8056, #13508, #17390, #37948, #46973, #57265, #42131, #33123, #52740, #42442, #42760, #37006, #28283, #61773, #2921, #32161, #46650, #8368, #3543, #47896, #37314, #23151, #22852, #12865, #62085, #18001, #62402, #18324, #22215, #25964, #2485, #31104, #15995, #45581, #1860, #26276, #16952, #35941, #36254, #40430, #16320, #56519, #60712, #41695, #50725, #51374, #12440, #31742, #35619, #6360, #55246, #6994, #46855, #7314, #26926, #6669, #41381, #36565, #30789, #11793, #22098, #55569, #50414, #56196, #31411, #11485, #40747, #45899, #26604, #16633, #46220, #21466, #41065, #55882, #60070, #51049, #1537, #21142, #60395, #2183, #21787, #61027, #11166, #12117, #46543, #61343, #27233, #17265, #36890, #32052, #51688, #7629, #20829, #50291, #55447, #25529, #10095, #40323, #784, #16196, #20392, #39992, #40637, #54487, #24898, #11048, #21029, #24576, #59637, #59961, #44499, #54807, #10415, #30026, #5921, #44182, #20064, #60278, #15570, #49655, #59306, #148, #5593, #20718, #6239, #35826, #15241, #58986, #25209, #10736, #35504, #15884, #35189, #30342, #44822, #49968, #25849, #39669, #34522, #45146, #30673, #11362, #5278, #55123, #30986, #1111, #45465, #1430, #50612, #39356, #19743, #29703, #14913, #54154, #49334, #34867, #463, #60909, #21346, #7196, #42221, #26166, #27426, #26803, #17782, #61866, #17478, #17151, #56406, #12331, #22624, #61228, #50932, #51883, #32575, #16831, #51263, #6873, #40948, #46735, #36775, #46104, #55761, #46425, #37401, #37100, #26488, #11999, #2680, #56718, #57037, #11678, #31942, #1745, #61547, #41576, #60598, #2373, #7510, #12636, #45785, #16517, #51570, #32253, #22301, #27121, #36139, #41900, #7823, #47058, #31296, #3008, #2062, #12951, #6551, #21671, #21982, #41261, #36451, #56079, #31626, #47373, #38345, #14517, #63118, #19030, #18414, #9072, #4254, #62171, #23869, #28683, #3322, #43473, #48303, #13592, #58285, #19347, #32895, #57972, #28370, #13896, #33211, #52828, #8763, #27744, #18721, #18093, #37717, #8456, #8144, #13271, #63431, #38034, #38645, #47990, #24178, #22941, #9381, #14204, #53139, #33831, #53449, #28991, #48615, #4554, #42535, #43785, #38961, #58597, #52196, #57353, #52521, #62496, #28062, #47679, #43161, #3631, #23239, #42852, #57667, #3944, #23567, #62801, #33523, #45388, #25449, #29626, #55044, #40246, #35422, #30264, #45069, #34784, #24498, #20640, #53757, #4877, #701, #10649, #59559, #48928, #39912, #5513, #59885, #44102, #49886, #9692, #5836, #20312, #10970, #10337, #34446, #15805, #1354, #35113, #19664, #1036, #29947, #25778, #49572, #25127, #50211, #381, #54077, #30589, #6162, #34138, #44740, #20957, #10015, #15492, #19985, #39593, #54729, #29299, #49260, #40558, #60201, #59230, #5198, #66, #39277, #58904, #14832, #24816, #44420, #15162, #54408, #17076, #35746, #51805, #12251, #37018, #31865, #17403, #46984, #26406, #42147, #36695, #51183, #40872, #16119, #27044, #56330, #50539, #2931, #51498, #7434, #27350, #46661, #11604, #56645, #22225, #12560, #2606, #41824, #16758, #6482, #55371, #36374, #32172, #30912, #7747, #36062, #61469, #6799, #22545, #11286, #46345, #26090, #45712, #1665, #46025, #31224, #60515, #21266, #16442, #41501, #55691, #50855, #1988, #56005, #21590, #41187, #60832, #61154, #11919, #31547, #7114, #26731, #2302, #21904, #3250, #42772, #3555, #57898, #13195, #13521, #17710, #57278, #33754, #37959, #18952, #27983, #28608, #53371, #8997, #56955, #47297, #12876, #47909, #24110, #48224, #4182, #47602, #18651, #13822, #8067, #52753, #63043, #32818, #27669, #33441, #23164, #38569, #9306, #61782, #14127, #62417, #18336, #57593, #33139, #32494, #23796, #22863, #52125, #28920, #4482, #42454, #48543, #8683, #38273, #28296, #37325, #62097, #43398, #18013, #37637, #52447, #3864, #8382, #58199, #23485, #43088, #53058, #62728, #53687, #15414, #44997, #58826, #9620, #35037, #54648, #58519, #29868, #44023, #49498, #19903, #5437, #5120, #24739, #305, #19269, #10264, #29227, #48854, #63670, #63353, #34703, #34373, #14443, #25055, #4796, #39517, #50134, #25375, #625, #44664, #59478, #10573, #30183, #962, #20235, #38884, #15728, #39837, #20563, #49812, #44342, #19590, #34065, #15088, #5757, #54328, #24421, #43707, #40166, #59807, #39200, #10896, #35347, #54967, #30511, #6089, #14756, #54002, #9931, #29546, #49179, #59155, #26652, #12172, #25701, #45947, #22149, #40481, #2535, #45635, #46271, #16370, #61393, #41744, #55928, #51421, #20879, #17319, #55620, #21190, #1912, #26018, #7364, #56567, #2230, #11216, #41431, #21517, #35989, #40798, #1279, #51102, #21834, #45312, #30840, #26972, #11535, #60122, #50470, #6719, #11843, #31150, #50778, #7041, #16044, #60445, #36941, #41113, #46591, #26329, #56250, #31789, #12489, #61080, #17001, #60761, #35672, #32101, #55300, #6408 ),
 .UNSPECIFIED., .F., .F. ) 
 B_SPLINE_CURVE_WITH_KNOTS ( ( 3, 2, 2, 2, 2, 2, 2, 2, 2, 2, 2, 2, 2, 2, 2, 2, 2, 2, 2, 2, 2, 2, 2, 2, 2, 2, 2, 2, 2, 2, 2, 2, 2, 2, 2, 2, 2, 2, 2, 2, 2, 2, 2, 2, 2, 2, 2, 2, 2, 2, 2, 2, 2, 2, 2, 2, 2, 2, 2, 2, 2, 2, 2, 2, 2, 2, 2, 2, 2, 2, 2, 2, 2, 2, 2, 2, 2, 2, 2, 2, 2, 2, 2, 2, 2, 2, 2, 2, 2, 2, 2, 2, 2, 2, 2, 2, 2, 2, 2, 2, 2, 2, 2, 2, 2, 2, 2, 2, 2, 2, 2, 2, 2, 2, 2, 2, 2, 2, 2, 2, 2, 2, 2, 2, 2, 2, 2, 2, 2, 2, 2, 2, 2, 2, 2, 2, 2, 2, 2, 2, 2, 2, 2, 2, 2, 2, 2, 2, 2, 2, 2, 2, 2, 2, 2, 2, 2, 2, 2, 2, 2, 2, 2, 2, 2, 2, 2, 2, 2, 2, 2, 2, 2, 2, 2, 2, 2, 2, 2, 2, 2, 2, 2, 2, 2, 2, 2, 2, 2, 2, 2, 2, 2, 2, 2, 2, 2, 2, 2, 2, 2, 2, 2, 2, 2, 2, 2, 2, 2, 2, 2, 2, 2, 2, 2, 2, 2, 2, 2, 2, 2, 2, 2, 2, 2, 2, 2, 2, 2, 2, 2, 2, 2, 2, 2, 2, 2, 2, 2, 2, 2, 2, 2, 2, 2, 2, 2, 2, 2, 2, 2, 2, 2, 2, 2, 2, 2, 2, 2, 2, 2, 2, 2, 2, 2, 2, 2, 2, 2, 2, 2, 2, 2, 2, 2, 2, 2, 2, 2, 2, 2, 2, 2, 2, 2, 2, 2, 2, 2, 2, 2, 2, 2, 2, 2, 2, 2, 2, 2, 2, 2, 2, 2, 2, 2, 2, 2, 2, 2, 2, 2, 2, 2, 2, 2, 2, 2, 2, 2, 2, 2, 2, 2, 2, 2, 2, 2, 2, 2, 2, 2, 2, 2, 2, 2, 2, 2, 2, 2, 2, 2, 2, 2, 2, 2, 2, 2, 2, 2, 2, 2, 2, 2, 2, 2, 2, 2, 2, 2, 2, 2, 2, 2, 2, 2, 2, 2, 2, 2, 2, 2, 2, 2, 2, 2, 2, 2, 2, 2, 2, 2, 2, 2, 2, 2, 2, 2, 2, 2, 2, 2, 2, 2, 2, 2, 2, 2, 2, 2, 2, 2, 2, 2, 2, 2, 2, 2, 2, 2, 2, 2, 2, 2, 2, 2, 2, 2, 2, 2, 2, 2, 2, 2, 2, 2, 2, 2, 2, 2, 2, 2, 2, 2, 2, 2, 2, 2, 2, 2, 2, 2, 2, 2, 2, 2, 2, 2, 2, 2, 2, 2, 2, 2, 2, 2, 2, 2, 2, 2, 2, 2, 2, 2, 2, 2, 2, 2, 2, 2, 2, 2, 2, 2, 2, 2, 2, 2, 2, 2, 2, 2, 2, 2, 2, 2, 2, 2, 2, 2, 2, 2, 2, 2, 2, 2, 2, 2, 2, 2, 2, 2, 2, 2, 2, 2, 2, 2, 2, 2, 2, 2, 2, 2, 2, 2, 2, 2, 2, 2, 2, 2, 2, 2, 2, 2, 2, 2, 2, 2, 2, 2, 2, 2, 2, 2, 2, 2, 2, 2, 2, 2, 2, 2, 2, 2, 2, 2, 2, 2, 2, 2, 2, 2, 2, 2, 2, 2, 2, 2, 2, 2, 2, 2, 2, 2, 2, 2, 2, 2, 2, 2, 2, 2, 2, 2, 2, 2, 2, 2, 2, 2, 2, 2, 2, 2, 2, 2, 2, 2, 2, 2, 2, 2, 2, 2, 2, 2, 2, 2, 2, 2, 2, 2, 2, 2, 2, 2, 2, 2, 2, 2, 2, 2, 2, 2, 2, 2, 2, 2, 2, 2, 2, 2, 2, 2, 2, 2, 2, 2, 2, 2, 2, 2, 2, 2, 2, 2, 2, 2, 2, 2, 2, 2, 2, 2, 2, 2, 2, 2, 2, 2, 2, 2, 2, 2, 2, 2, 2, 2, 2, 2, 2, 2, 2, 2, 2, 2, 2, 2, 2, 2, 2, 2, 2, 2, 2, 2, 2, 2, 2, 2, 2, 2, 2, 2, 2, 2, 2, 2, 2, 2, 2, 2, 2, 2, 2, 2, 2, 2, 2, 2, 2, 2, 2, 2, 2, 2, 2, 2, 2, 2, 2, 2, 2, 2, 2, 2, 2, 2, 2, 3 ),
 ( 0.000000000000000000, 0.001388888888888888942, 0.002777777777777777884, 0.004166666666666666609, 0.005555555555555555768, 0.006944444444444444059, 0.008333333333333333218, 0.009722222222222222376, 0.01111111111111111154, 0.01250000000000000069, 0.01388888888888888812, 0.01527777777777777728, 0.01666666666666666644, 0.01805555555555555386, 0.01944444444444444475, 0.02083333333333333218, 0.02222222222222222307, 0.02361111111111111049, 0.02500000000000000139, 0.02638888888888888881, 0.02777777777777777624, 0.02916666666666666713, 0.03055555555555555455, 0.03194444444444444198, 0.03333333333333333287, 0.03472222222222222376, 0.03611111111111110772, 0.03749999999999999861, 0.03888888888888888951, 0.04027777777777778040, 0.04166666666666666435, 0.04305555555555555525, 0.04444444444444444614, 0.04583333333333333010, 0.04722222222222222099, 0.04861111111111111188, 0.05000000000000000278, 0.05138888888888888673, 0.05277777777777777762, 0.05416666666666666852, 0.05555555555555555247, 0.05694444444444444337, 0.05833333333333333426, 0.05972222222222222515, 0.06111111111111110911, 0.06250000000000000000, 0.06388888888888888395, 0.06527777777777778179, 0.06666666666666666574, 0.06805555555555554970, 0.06944444444444444753, 0.07083333333333333148, 0.07222222222222221544, 0.07361111111111111327, 0.07499999999999999722, 0.07638888888888889506, 0.07777777777777777901, 0.07916666666666666297, 0.08055555555555556080, 0.08194444444444444475, 0.08333333333333332871, 0.08472222222222222654, 0.08611111111111111049, 0.08749999999999999445, 0.08888888888888889228, 0.09027777777777777624, 0.09166666666666666019, 0.09305555555555555802, 0.09444444444444444198, 0.09583333333333333981, 0.09722222222222222376, 0.09861111111111110772, 0.1000000000000000056, 0.1013888888888888895, 0.1027777777777777735, 0.1041666666666666713, 0.1055555555555555552, 0.1069444444444444392, 0.1083333333333333370, 0.1097222222222222210, 0.1111111111111111049, 0.1125000000000000028, 0.1138888888888888867, 0.1152777777777777846, 0.1166666666666666685, 0.1180555555555555525, 0.1194444444444444503, 0.1208333333333333343, 0.1222222222222222182, 0.1236111111111111160, 0.1250000000000000000, 0.1263888888888888840, 0.1277777777777777679, 0.1291666666666666796, 0.1305555555555555636, 0.1319444444444444475, 0.1333333333333333315, 0.1347222222222222154, 0.1361111111111110994, 0.1375000000000000111, 0.1388888888888888951, 0.1402777777777777790, 0.1416666666666666630, 0.1430555555555555469, 0.1444444444444444309, 0.1458333333333333426, 0.1472222222222222265, 0.1486111111111111105, 0.1499999999999999944, 0.1513888888888888784, 0.1527777777777777901, 0.1541666666666666741, 0.1555555555555555580, 0.1569444444444444420, 0.1583333333333333259, 0.1597222222222222099, 0.1611111111111111216, 0.1625000000000000056, 0.1638888888888888895, 0.1652777777777777735, 0.1666666666666666574, 0.1680555555555555691, 0.1694444444444444531, 0.1708333333333333370, 0.1722222222222222210, 0.1736111111111111049, 0.1749999999999999889, 0.1763888888888889006, 0.1777777777777777846, 0.1791666666666666685, 0.1805555555555555525, 0.1819444444444444364, 0.1833333333333333204, 0.1847222222222222321, 0.1861111111111111160, 0.1875000000000000000, 0.1888888888888888840, 0.1902777777777777679, 0.1916666666666666796, 0.1930555555555555636, 0.1944444444444444475, 0.1958333333333333315, 0.1972222222222222154, 0.1986111111111110994, 0.2000000000000000111, 0.2013888888888888951, 0.2027777777777777790, 0.2041666666666666630, 0.2055555555555555469, 0.2069444444444444309, 0.2083333333333333426, 0.2097222222222222265, 0.2111111111111111105, 0.2124999999999999944, 0.2138888888888888784, 0.2152777777777777901, 0.2166666666666666741, 0.2180555555555555580, 0.2194444444444444420, 0.2208333333333333259, 0.2222222222222222099, 0.2236111111111111216, 0.2250000000000000056, 0.2263888888888888895, 0.2277777777777777735, 0.2291666666666666574, 0.2305555555555555691, 0.2319444444444444531, 0.2333333333333333370, 0.2347222222222222210, 0.2361111111111111049, 0.2374999999999999889, 0.2388888888888889006, 0.2402777777777777846, 0.2416666666666666685, 0.2430555555555555525, 0.2444444444444444364, 0.2458333333333333204, 0.2472222222222222321, 0.2486111111111111160, 0.2500000000000000000, 0.2513888888888888840, 0.2527777777777777679, 0.2541666666666666519, 0.2555555555555555358, 0.2569444444444444198, 0.2583333333333333592, 0.2597222222222222432, 0.2611111111111111271, 0.2625000000000000111, 0.2638888888888888951, 0.2652777777777777790, 0.2666666666666666630, 0.2680555555555555469, 0.2694444444444444309, 0.2708333333333333148, 0.2722222222222221988, 0.2736111111111111382, 0.2750000000000000222, 0.2763888888888889062, 0.2777777777777777901, 0.2791666666666666741, 0.2805555555555555580, 0.2819444444444444420, 0.2833333333333333259, 0.2847222222222222099, 0.2861111111111110938, 0.2874999999999999778, 0.2888888888888888618, 0.2902777777777778012, 0.2916666666666666852, 0.2930555555555555691, 0.2944444444444444531, 0.2958333333333333370, 0.2972222222222222210, 0.2986111111111111049, 0.2999999999999999889, 0.3013888888888888729, 0.3027777777777777568, 0.3041666666666666408, 0.3055555555555555802, 0.3069444444444444642, 0.3083333333333333481, 0.3097222222222222321, 0.3111111111111111160, 0.3125000000000000000, 0.3138888888888888840, 0.3152777777777777679, 0.3166666666666666519, 0.3180555555555555358, 0.3194444444444444198, 0.3208333333333333592, 0.3222222222222222432, 0.3236111111111111271, 0.3250000000000000111, 0.3263888888888888951, 0.3277777777777777790, 0.3291666666666666630, 0.3305555555555555469, 0.3319444444444444309, 0.3333333333333333148, 0.3347222222222221988, 0.3361111111111111382, 0.3375000000000000222, 0.3388888888888889062, 0.3402777777777777901, 0.3416666666666666741, 0.3430555555555555580, 0.3444444444444444420, 0.3458333333333333259, 0.3472222222222222099, 0.3486111111111110938, 0.3499999999999999778, 0.3513888888888888618, 0.3527777777777778012, 0.3541666666666666852, 0.3555555555555555691, 0.3569444444444444531, 0.3583333333333333370, 0.3597222222222222210, 0.3611111111111111049, 0.3624999999999999889, 0.3638888888888888729, 0.3652777777777777568, 0.3666666666666666408, 0.3680555555555555802, 0.3694444444444444642, 0.3708333333333333481, 0.3722222222222222321, 0.3736111111111111160, 0.3750000000000000000, 0.3763888888888888840, 0.3777777777777777679, 0.3791666666666666519, 0.3805555555555555358, 0.3819444444444444198, 0.3833333333333333592, 0.3847222222222222432, 0.3861111111111111271, 0.3875000000000000111, 0.3888888888888888951, 0.3902777777777777790, 0.3916666666666666630, 0.3930555555555555469, 0.3944444444444444309, 0.3958333333333333148, 0.3972222222222221988, 0.3986111111111111382, 0.4000000000000000222, 0.4013888888888889062, 0.4027777777777777901, 0.4041666666666666741, 0.4055555555555555580, 0.4069444444444444420, 0.4083333333333333259, 0.4097222222222222099, 0.4111111111111110938, 0.4124999999999999778, 0.4138888888888888618, 0.4152777777777778012, 0.4166666666666666852, 0.4180555555555555691, 0.4194444444444444531, 0.4208333333333333370, 0.4222222222222222210, 0.4236111111111111049, 0.4249999999999999889, 0.4263888888888888729, 0.4277777777777777568, 0.4291666666666666408, 0.4305555555555555802, 0.4319444444444444642, 0.4333333333333333481, 0.4347222222222222321, 0.4361111111111111160, 0.4375000000000000000, 0.4388888888888888840, 0.4402777777777777679, 0.4416666666666666519, 0.4430555555555555358, 0.4444444444444444198, 0.4458333333333333592, 0.4472222222222222432, 0.4486111111111111271, 0.4500000000000000111, 0.4513888888888888951, 0.4527777777777777790, 0.4541666666666666630, 0.4555555555555555469, 0.4569444444444444309, 0.4583333333333333148, 0.4597222222222221988, 0.4611111111111111382, 0.4625000000000000222, 0.4638888888888889062, 0.4652777777777777901, 0.4666666666666666741, 0.4680555555555555580, 0.4694444444444444420, 0.4708333333333333259, 0.4722222222222222099, 0.4736111111111110938, 0.4749999999999999778, 0.4763888888888888618, 0.4777777777777778012, 0.4791666666666666852, 0.4805555555555555691, 0.4819444444444444531, 0.4833333333333333370, 0.4847222222222222210, 0.4861111111111111049, 0.4874999999999999889, 0.4888888888888888729, 0.4902777777777777568, 0.4916666666666666408, 0.4930555555555555802, 0.4944444444444444642, 0.4958333333333333481, 0.4972222222222222321, 0.4986111111111111160, 0.5000000000000000000, 0.5013888888888888840, 0.5027777777777777679, 0.5041666666666666519, 0.5055555555555555358, 0.5069444444444444198, 0.5083333333333333037, 0.5097222222222221877, 0.5111111111111110716, 0.5124999999999999556, 0.5138888888888888395, 0.5152777777777777235, 0.5166666666666667185, 0.5180555555555556024, 0.5194444444444444864, 0.5208333333333333703, 0.5222222222222222543, 0.5236111111111111382, 0.5250000000000000222, 0.5263888888888889062, 0.5277777777777777901, 0.5291666666666666741, 0.5305555555555555580, 0.5319444444444444420, 0.5333333333333333259, 0.5347222222222222099, 0.5361111111111110938, 0.5374999999999999778, 0.5388888888888888618, 0.5402777777777777457, 0.5416666666666666297, 0.5430555555555555136, 0.5444444444444443976, 0.5458333333333332815, 0.5472222222222222765, 0.5486111111111111605, 0.5500000000000000444, 0.5513888888888889284, 0.5527777777777778123, 0.5541666666666666963, 0.5555555555555555802, 0.5569444444444444642, 0.5583333333333333481, 0.5597222222222222321, 0.5611111111111111160, 0.5625000000000000000, 0.5638888888888888840, 0.5652777777777777679, 0.5666666666666666519, 0.5680555555555555358, 0.5694444444444444198, 0.5708333333333333037, 0.5722222222222221877, 0.5736111111111110716, 0.5749999999999999556, 0.5763888888888888395, 0.5777777777777777235, 0.5791666666666667185, 0.5805555555555556024, 0.5819444444444444864, 0.5833333333333333703, 0.5847222222222222543, 0.5861111111111111382, 0.5875000000000000222, 0.5888888888888889062, 0.5902777777777777901, 0.5916666666666666741, 0.5930555555555555580, 0.5944444444444444420, 0.5958333333333333259, 0.5972222222222222099, 0.5986111111111110938, 0.5999999999999999778, 0.6013888888888888618, 0.6027777777777777457, 0.6041666666666666297, 0.6055555555555555136, 0.6069444444444443976, 0.6083333333333332815, 0.6097222222222222765, 0.6111111111111111605, 0.6125000000000000444, 0.6138888888888889284, 0.6152777777777778123, 0.6166666666666666963, 0.6180555555555555802, 0.6194444444444444642, 0.6208333333333333481, 0.6222222222222222321, 0.6236111111111111160, 0.6250000000000000000, 0.6263888888888888840, 0.6277777777777777679, 0.6291666666666666519, 0.6305555555555555358, 0.6319444444444444198, 0.6333333333333333037, 0.6347222222222221877, 0.6361111111111110716, 0.6374999999999999556, 0.6388888888888888395, 0.6402777777777777235, 0.6416666666666667185, 0.6430555555555556024, 0.6444444444444444864, 0.6458333333333333703, 0.6472222222222222543, 0.6486111111111111382, 0.6500000000000000222, 0.6513888888888889062, 0.6527777777777777901, 0.6541666666666666741, 0.6555555555555555580, 0.6569444444444444420, 0.6583333333333333259, 0.6597222222222222099, 0.6611111111111110938, 0.6624999999999999778, 0.6638888888888888618, 0.6652777777777777457, 0.6666666666666666297, 0.6680555555555555136, 0.6694444444444443976, 0.6708333333333332815, 0.6722222222222222765, 0.6736111111111111605, 0.6750000000000000444, 0.6763888888888889284, 0.6777777777777778123, 0.6791666666666666963, 0.6805555555555555802, 0.6819444444444444642, 0.6833333333333333481, 0.6847222222222222321, 0.6861111111111111160, 0.6875000000000000000, 0.6888888888888888840, 0.6902777777777777679, 0.6916666666666666519, 0.6930555555555555358, 0.6944444444444444198, 0.6958333333333333037, 0.6972222222222221877, 0.6986111111111110716, 0.6999999999999999556, 0.7013888888888888395, 0.7027777777777777235, 0.7041666666666667185, 0.7055555555555556024, 0.7069444444444444864, 0.7083333333333333703, 0.7097222222222222543, 0.7111111111111111382, 0.7125000000000000222, 0.7138888888888889062, 0.7152777777777777901, 0.7166666666666666741, 0.7180555555555555580, 0.7194444444444444420, 0.7208333333333333259, 0.7222222222222222099, 0.7236111111111110938, 0.7249999999999999778, 0.7263888888888888618, 0.7277777777777777457, 0.7291666666666666297, 0.7305555555555555136, 0.7319444444444443976, 0.7333333333333332815, 0.7347222222222222765, 0.7361111111111111605, 0.7375000000000000444, 0.7388888888888889284, 0.7402777777777778123, 0.7416666666666666963, 0.7430555555555555802, 0.7444444444444444642, 0.7458333333333333481, 0.7472222222222222321, 0.7486111111111111160, 0.7500000000000000000, 0.7513888888888888840, 0.7527777777777777679, 0.7541666666666666519, 0.7555555555555555358, 0.7569444444444444198, 0.7583333333333333037, 0.7597222222222221877, 0.7611111111111110716, 0.7624999999999999556, 0.7638888888888888395, 0.7652777777777777235, 0.7666666666666667185, 0.7680555555555556024, 0.7694444444444444864, 0.7708333333333333703, 0.7722222222222222543, 0.7736111111111111382, 0.7750000000000000222, 0.7763888888888889062, 0.7777777777777777901, 0.7791666666666666741, 0.7805555555555555580, 0.7819444444444444420, 0.7833333333333333259, 0.7847222222222222099, 0.7861111111111110938, 0.7874999999999999778, 0.7888888888888888618, 0.7902777777777777457, 0.7916666666666666297, 0.7930555555555555136, 0.7944444444444443976, 0.7958333333333332815, 0.7972222222222222765, 0.7986111111111111605, 0.8000000000000000444, 0.8013888888888889284, 0.8027777777777778123, 0.8041666666666666963, 0.8055555555555555802, 0.8069444444444444642, 0.8083333333333333481, 0.8097222222222222321, 0.8111111111111111160, 0.8125000000000000000, 0.8138888888888888840, 0.8152777777777777679, 0.8166666666666666519, 0.8180555555555555358, 0.8194444444444444198, 0.8208333333333333037, 0.8222222222222221877, 0.8236111111111110716, 0.8249999999999999556, 0.8263888888888888395, 0.8277777777777777235, 0.8291666666666667185, 0.8305555555555556024, 0.8319444444444444864, 0.8333333333333333703, 0.8347222222222222543, 0.8361111111111111382, 0.8375000000000000222, 0.8388888888888889062, 0.8402777777777777901, 0.8416666666666666741, 0.8430555555555555580, 0.8444444444444444420, 0.8458333333333333259, 0.8472222222222222099, 0.8486111111111110938, 0.8499999999999999778, 0.8513888888888888618, 0.8527777777777777457, 0.8541666666666666297, 0.8555555555555555136, 0.8569444444444443976, 0.8583333333333332815, 0.8597222222222222765, 0.8611111111111111605, 0.8625000000000000444, 0.8638888888888889284, 0.8652777777777778123, 0.8666666666666666963, 0.8680555555555555802, 0.8694444444444444642, 0.8708333333333333481, 0.8722222222222222321, 0.8736111111111111160, 0.8750000000000000000, 0.8763888888888888840, 0.8777777777777777679, 0.8791666666666666519, 0.8805555555555555358, 0.8819444444444444198, 0.8833333333333333037, 0.8847222222222221877, 0.8861111111111110716, 0.8874999999999999556, 0.8888888888888888395, 0.8902777777777777235, 0.8916666666666667185, 0.8930555555555556024, 0.8944444444444444864, 0.8958333333333333703, 0.8972222222222222543, 0.8986111111111111382, 0.9000000000000000222, 0.9013888888888889062, 0.9027777777777777901, 0.9041666666666666741, 0.9055555555555555580, 0.9069444444444444420, 0.9083333333333333259, 0.9097222222222222099, 0.9111111111111110938, 0.9124999999999999778, 0.9138888888888888618, 0.9152777777777777457, 0.9166666666666666297, 0.9180555555555555136, 0.9194444444444443976, 0.9208333333333332815, 0.9222222222222222765, 0.9236111111111111605, 0.9250000000000000444, 0.9263888888888889284, 0.9277777777777778123, 0.9291666666666666963, 0.9305555555555555802, 0.9319444444444444642, 0.9333333333333333481, 0.9347222222222222321, 0.9361111111111111160, 0.9375000000000000000, 0.9388888888888888840, 0.9402777777777777679, 0.9416666666666666519, 0.9430555555555555358, 0.9444444444444444198, 0.9458333333333333037, 0.9472222222222221877, 0.9486111111111110716, 0.9499999999999999556, 0.9513888888888888395, 0.9527777777777777235, 0.9541666666666667185, 0.9555555555555556024, 0.9569444444444444864, 0.9583333333333333703, 0.9597222222222222543, 0.9611111111111111382, 0.9625000000000000222, 0.9638888888888889062, 0.9652777777777777901, 0.9666666666666666741, 0.9680555555555555580, 0.9694444444444444420, 0.9708333333333333259, 0.9722222222222222099, 0.9736111111111110938, 0.9749999999999999778, 0.9763888888888888618, 0.9777777777777777457, 0.9791666666666666297, 0.9805555555555555136, 0.9819444444444443976, 0.9833333333333332815, 0.9847222222222222765, 0.9861111111111111605, 0.9875000000000000444, 0.9888888888888889284, 0.9902777777777778123, 0.9916666666666666963, 0.9930555555555555802, 0.9944444444444444642, 0.9958333333333333481, 0.9972222222222222321, 0.9986111111111111160, 1.000000000000000000 ),
 .UNSPECIFIED. ) 
 CURVE ( )  GEOMETRIC_REPRESENTATION_ITEM ( )  RATIONAL_B_SPLINE_CURVE ( ( 1.000000000000000000, 0.8660254037844387076, 1.000000000000000000, 0.8660254037844387076, 1.000000000000000000, 0.8660254037844387076, 1.000000000000000000, 0.8660254037844387076, 1.000000000000000000, 0.8660254037844387076, 1.000000000000000000, 0.8660254037844387076, 1.000000000000000000, 0.8660254037844387076, 1.000000000000000000, 0.8660254037844387076, 1.000000000000000000, 0.8660254037844387076, 1.000000000000000000, 0.8660254037844387076, 1.000000000000000000, 0.8660254037844387076, 1.000000000000000000, 0.8660254037844387076, 1.000000000000000000, 0.8660254037844387076, 1.000000000000000000, 0.8660254037844387076, 1.000000000000000000, 0.8660254037844387076, 1.000000000000000000, 0.8660254037844387076, 1.000000000000000000, 0.8660254037844387076, 1.000000000000000000, 0.8660254037844387076, 1.000000000000000000, 0.8660254037844387076, 1.000000000000000000, 0.8660254037844387076, 1.000000000000000000, 0.8660254037844387076, 1.000000000000000000, 0.8660254037844387076, 1.000000000000000000, 0.8660254037844387076, 1.000000000000000000, 0.8660254037844387076, 1.000000000000000000, 0.8660254037844387076, 1.000000000000000000, 0.8660254037844387076, 1.000000000000000000, 0.8660254037844387076, 1.000000000000000000, 0.8660254037844387076, 1.000000000000000000, 0.8660254037844387076, 1.000000000000000000, 0.8660254037844387076, 1.000000000000000000, 0.8660254037844387076, 1.000000000000000000, 0.8660254037844387076, 1.000000000000000000, 0.8660254037844387076, 1.000000000000000000, 0.8660254037844387076, 1.000000000000000000, 0.8660254037844387076, 1.000000000000000000, 0.8660254037844387076, 1.000000000000000000, 0.8660254037844387076, 1.000000000000000000, 0.8660254037844387076, 1.000000000000000000, 0.8660254037844387076, 1.000000000000000000, 0.8660254037844387076, 1.000000000000000000, 0.8660254037844387076, 1.000000000000000000, 0.8660254037844387076, 1.000000000000000000, 0.8660254037844387076, 1.000000000000000000, 0.8660254037844387076, 1.000000000000000000, 0.8660254037844387076, 1.000000000000000000, 0.8660254037844387076, 1.000000000000000000, 0.8660254037844387076, 1.000000000000000000, 0.8660254037844387076, 1.000000000000000000, 0.8660254037844387076, 1.000000000000000000, 0.8660254037844387076, 1.000000000000000000, 0.8660254037844387076, 1.000000000000000000, 0.8660254037844387076, 1.000000000000000000, 0.8660254037844387076, 1.000000000000000000, 0.8660254037844387076, 1.000000000000000000, 0.8660254037844387076, 1.000000000000000000, 0.8660254037844387076, 1.000000000000000000, 0.8660254037844387076, 1.000000000000000000, 0.8660254037844387076, 1.000000000000000000, 0.8660254037844387076, 1.000000000000000000, 0.8660254037844387076, 1.000000000000000000, 0.8660254037844387076, 1.000000000000000000, 0.8660254037844387076, 1.000000000000000000, 0.8660254037844387076, 1.000000000000000000, 0.8660254037844387076, 1.000000000000000000, 0.8660254037844387076, 1.000000000000000000, 0.8660254037844387076, 1.000000000000000000, 0.8660254037844387076, 1.000000000000000000, 0.8660254037844387076, 1.000000000000000000, 0.8660254037844387076, 1.000000000000000000, 0.8660254037844387076, 1.000000000000000000, 0.8660254037844387076, 1.000000000000000000, 0.8660254037844387076, 1.000000000000000000, 0.8660254037844387076, 1.000000000000000000, 0.8660254037844387076, 1.000000000000000000, 0.8660254037844387076, 1.000000000000000000, 0.8660254037844387076, 1.000000000000000000, 0.8660254037844387076, 1.000000000000000000, 0.8660254037844387076, 1.000000000000000000, 0.8660254037844387076, 1.000000000000000000, 0.8660254037844387076, 1.000000000000000000, 0.8660254037844387076, 1.000000000000000000, 0.8660254037844387076, 1.000000000000000000, 0.8660254037844387076, 1.000000000000000000, 0.8660254037844387076, 1.000000000000000000, 0.8660254037844387076, 1.000000000000000000, 0.8660254037844387076, 1.000000000000000000, 0.8660254037844387076, 1.000000000000000000, 0.8660254037844387076, 1.000000000000000000, 0.8660254037844387076, 1.000000000000000000, 0.8660254037844387076, 1.000000000000000000, 0.8660254037844387076, 1.000000000000000000, 0.8660254037844387076, 1.000000000000000000, 0.8660254037844387076, 1.000000000000000000, 0.8660254037844387076, 1.000000000000000000, 0.8660254037844387076, 1.000000000000000000, 0.8660254037844387076, 1.000000000000000000, 0.8660254037844387076, 1.000000000000000000, 0.8660254037844387076, 1.000000000000000000, 0.8660254037844387076, 1.000000000000000000, 0.8660254037844387076, 1.000000000000000000, 0.8660254037844387076, 1.000000000000000000, 0.8660254037844387076, 1.000000000000000000, 0.8660254037844387076, 1.000000000000000000, 0.8660254037844387076, 1.000000000000000000, 0.8660254037844387076, 1.000000000000000000, 0.8660254037844387076, 1.000000000000000000, 0.8660254037844387076, 1.000000000000000000, 0.8660254037844387076, 1.000000000000000000, 0.8660254037844387076, 1.000000000000000000, 0.8660254037844387076, 1.000000000000000000, 0.8660254037844387076, 1.000000000000000000, 0.8660254037844387076, 1.000000000000000000, 0.8660254037844387076, 1.000000000000000000, 0.8660254037844387076, 1.000000000000000000, 0.8660254037844387076, 1.000000000000000000, 0.8660254037844387076, 1.000000000000000000, 0.8660254037844387076, 1.000000000000000000, 0.8660254037844387076, 1.000000000000000000, 0.8660254037844387076, 1.000000000000000000, 0.8660254037844387076, 1.000000000000000000, 0.8660254037844387076, 1.000000000000000000, 0.8660254037844387076, 1.000000000000000000, 0.8660254037844387076, 1.000000000000000000, 0.8660254037844387076, 1.000000000000000000, 0.8660254037844387076, 1.000000000000000000, 0.8660254037844387076, 1.000000000000000000, 0.8660254037844387076, 1.000000000000000000, 0.8660254037844387076, 1.000000000000000000, 0.8660254037844387076, 1.000000000000000000, 0.8660254037844387076, 1.000000000000000000, 0.8660254037844387076, 1.000000000000000000, 0.8660254037844387076, 1.000000000000000000, 0.8660254037844387076, 1.000000000000000000, 0.8660254037844387076, 1.000000000000000000, 0.8660254037844387076, 1.000000000000000000, 0.8660254037844387076, 1.000000000000000000, 0.8660254037844387076, 1.000000000000000000, 0.8660254037844387076, 1.000000000000000000, 0.8660254037844387076, 1.000000000000000000, 0.8660254037844387076, 1.000000000000000000, 0.8660254037844387076, 1.000000000000000000, 0.8660254037844387076, 1.000000000000000000, 0.8660254037844387076, 1.000000000000000000, 0.8660254037844387076, 1.000000000000000000, 0.8660254037844387076, 1.000000000000000000, 0.8660254037844387076, 1.000000000000000000, 0.8660254037844387076, 1.000000000000000000, 0.8660254037844387076, 1.000000000000000000, 0.8660254037844387076, 1.000000000000000000, 0.8660254037844387076, 1.000000000000000000, 0.8660254037844387076, 1.000000000000000000, 0.8660254037844387076, 1.000000000000000000, 0.8660254037844387076, 1.000000000000000000, 0.8660254037844387076, 1.000000000000000000, 0.8660254037844387076, 1.000000000000000000, 0.8660254037844387076, 1.000000000000000000, 0.8660254037844387076, 1.000000000000000000, 0.8660254037844387076, 1.000000000000000000, 0.8660254037844387076, 1.000000000000000000, 0.8660254037844387076, 1.000000000000000000, 0.8660254037844387076, 1.000000000000000000, 0.8660254037844387076, 1.000000000000000000, 0.8660254037844387076, 1.000000000000000000, 0.8660254037844387076, 1.000000000000000000, 0.8660254037844387076, 1.000000000000000000, 0.8660254037844387076, 1.000000000000000000, 0.8660254037844387076, 1.000000000000000000, 0.8660254037844387076, 1.000000000000000000, 0.8660254037844387076, 1.000000000000000000, 0.8660254037844387076, 1.000000000000000000, 0.8660254037844387076, 1.000000000000000000, 0.8660254037844387076, 1.000000000000000000, 0.8660254037844387076, 1.000000000000000000, 0.8660254037844387076, 1.000000000000000000, 0.8660254037844387076, 1.000000000000000000, 0.8660254037844387076, 1.000000000000000000, 0.8660254037844387076, 1.000000000000000000, 0.8660254037844387076, 1.000000000000000000, 0.8660254037844387076, 1.000000000000000000, 0.8660254037844387076, 1.000000000000000000, 0.8660254037844387076, 1.000000000000000000, 0.8660254037844387076, 1.000000000000000000, 0.8660254037844387076, 1.000000000000000000, 0.8660254037844387076, 1.000000000000000000, 0.8660254037844387076, 1.000000000000000000, 0.8660254037844387076, 1.000000000000000000, 0.8660254037844387076, 1.000000000000000000, 0.8660254037844387076, 1.000000000000000000, 0.8660254037844387076, 1.000000000000000000, 0.8660254037844387076, 1.000000000000000000, 0.8660254037844387076, 1.000000000000000000, 0.8660254037844387076, 1.000000000000000000, 0.8660254037844387076, 1.000000000000000000, 0.8660254037844387076, 1.000000000000000000, 0.8660254037844387076, 1.000000000000000000, 0.8660254037844387076, 1.000000000000000000, 0.8660254037844387076, 1.000000000000000000, 0.8660254037844387076, 1.000000000000000000, 0.8660254037844387076, 1.000000000000000000, 0.8660254037844387076, 1.000000000000000000, 0.8660254037844387076, 1.000000000000000000, 0.8660254037844387076, 1.000000000000000000, 0.8660254037844387076, 1.000000000000000000, 0.8660254037844387076, 1.000000000000000000, 0.8660254037844387076, 1.000000000000000000, 0.8660254037844387076, 1.000000000000000000, 0.8660254037844387076, 1.000000000000000000, 0.8660254037844387076, 1.000000000000000000, 0.8660254037844387076, 1.000000000000000000, 0.8660254037844387076, 1.000000000000000000, 0.8660254037844387076, 1.000000000000000000, 0.8660254037844387076, 1.000000000000000000, 0.8660254037844387076, 1.000000000000000000, 0.8660254037844387076, 1.000000000000000000, 0.8660254037844387076, 1.000000000000000000, 0.8660254037844387076, 1.000000000000000000, 0.8660254037844387076, 1.000000000000000000, 0.8660254037844387076, 1.000000000000000000, 0.8660254037844387076, 1.000000000000000000, 0.8660254037844387076, 1.000000000000000000, 0.8660254037844387076, 1.000000000000000000, 0.8660254037844387076, 1.000000000000000000, 0.8660254037844387076, 1.000000000000000000, 0.8660254037844387076, 1.000000000000000000, 0.8660254037844387076, 1.000000000000000000, 0.8660254037844387076, 1.000000000000000000, 0.8660254037844387076, 1.000000000000000000, 0.8660254037844387076, 1.000000000000000000, 0.8660254037844387076, 1.000000000000000000, 0.8660254037844387076, 1.000000000000000000, 0.8660254037844387076, 1.000000000000000000, 0.8660254037844387076, 1.000000000000000000, 0.8660254037844387076, 1.000000000000000000, 0.8660254037844387076, 1.000000000000000000, 0.8660254037844387076, 1.000000000000000000, 0.8660254037844387076, 1.000000000000000000, 0.8660254037844387076, 1.000000000000000000, 0.8660254037844387076, 1.000000000000000000, 0.8660254037844387076, 1.000000000000000000, 0.8660254037844387076, 1.000000000000000000, 0.8660254037844387076, 1.000000000000000000, 0.8660254037844387076, 1.000000000000000000, 0.8660254037844387076, 1.000000000000000000, 0.8660254037844387076, 1.000000000000000000, 0.8660254037844387076, 1.000000000000000000, 0.8660254037844387076, 1.000000000000000000, 0.8660254037844387076, 1.000000000000000000, 0.8660254037844387076, 1.000000000000000000, 0.8660254037844387076, 1.000000000000000000, 0.8660254037844387076, 1.000000000000000000, 0.8660254037844387076, 1.000000000000000000, 0.8660254037844387076, 1.000000000000000000, 0.8660254037844387076, 1.000000000000000000, 0.8660254037844387076, 1.000000000000000000, 0.8660254037844387076, 1.000000000000000000, 0.8660254037844387076, 1.000000000000000000, 0.8660254037844387076, 1.000000000000000000, 0.8660254037844387076, 1.000000000000000000, 0.8660254037844387076, 1.000000000000000000, 0.8660254037844387076, 1.000000000000000000, 0.8660254037844387076, 1.000000000000000000, 0.8660254037844387076, 1.000000000000000000, 0.8660254037844387076, 1.000000000000000000, 0.8660254037844387076, 1.000000000000000000, 0.8660254037844387076, 1.000000000000000000, 0.8660254037844387076, 1.000000000000000000, 0.8660254037844387076, 1.000000000000000000, 0.8660254037844387076, 1.000000000000000000, 0.8660254037844387076, 1.000000000000000000, 0.8660254037844387076, 1.000000000000000000, 0.8660254037844387076, 1.000000000000000000, 0.8660254037844387076, 1.000000000000000000, 0.8660254037844387076, 1.000000000000000000, 0.8660254037844387076, 1.000000000000000000, 0.8660254037844387076, 1.000000000000000000, 0.8660254037844387076, 1.000000000000000000, 0.8660254037844387076, 1.000000000000000000, 0.8660254037844387076, 1.000000000000000000, 0.8660254037844387076, 1.000000000000000000, 0.8660254037844387076, 1.000000000000000000, 0.8660254037844387076, 1.000000000000000000, 0.8660254037844387076, 1.000000000000000000, 0.8660254037844387076, 1.000000000000000000, 0.8660254037844387076, 1.000000000000000000, 0.8660254037844387076, 1.000000000000000000, 0.8660254037844387076, 1.000000000000000000, 0.8660254037844387076, 1.000000000000000000, 0.8660254037844387076, 1.000000000000000000, 0.8660254037844387076, 1.000000000000000000, 0.8660254037844387076, 1.000000000000000000, 0.8660254037844387076, 1.000000000000000000, 0.8660254037844387076, 1.000000000000000000, 0.8660254037844387076, 1.000000000000000000, 0.8660254037844387076, 1.000000000000000000, 0.8660254037844387076, 1.000000000000000000, 0.8660254037844387076, 1.000000000000000000, 0.8660254037844387076, 1.000000000000000000, 0.8660254037844387076, 1.000000000000000000, 0.8660254037844387076, 1.000000000000000000, 0.8660254037844387076, 1.000000000000000000, 0.8660254037844387076, 1.000000000000000000, 0.8660254037844387076, 1.000000000000000000, 0.8660254037844387076, 1.000000000000000000, 0.8660254037844387076, 1.000000000000000000, 0.8660254037844387076, 1.000000000000000000, 0.8660254037844387076, 1.000000000000000000, 0.8660254037844387076, 1.000000000000000000, 0.8660254037844387076, 1.000000000000000000, 0.8660254037844387076, 1.000000000000000000, 0.8660254037844387076, 1.000000000000000000, 0.8660254037844387076, 1.000000000000000000, 0.8660254037844387076, 1.000000000000000000, 0.8660254037844387076, 1.000000000000000000, 0.8660254037844387076, 1.000000000000000000, 0.8660254037844387076, 1.000000000000000000, 0.8660254037844387076, 1.000000000000000000, 0.8660254037844387076, 1.000000000000000000, 0.8660254037844387076, 1.000000000000000000, 0.8660254037844387076, 1.000000000000000000, 0.8660254037844387076, 1.000000000000000000, 0.8660254037844387076, 1.000000000000000000, 0.8660254037844387076, 1.000000000000000000, 0.8660254037844387076, 1.000000000000000000, 0.8660254037844387076, 1.000000000000000000, 0.8660254037844387076, 1.000000000000000000, 0.8660254037844387076, 1.000000000000000000, 0.8660254037844387076, 1.000000000000000000, 0.8660254037844387076, 1.000000000000000000, 0.8660254037844387076, 1.000000000000000000, 0.8660254037844387076, 1.000000000000000000, 0.8660254037844387076, 1.000000000000000000, 0.8660254037844387076, 1.000000000000000000, 0.8660254037844387076, 1.000000000000000000, 0.8660254037844387076, 1.000000000000000000, 0.8660254037844387076, 1.000000000000000000, 0.8660254037844387076, 1.000000000000000000, 0.8660254037844387076, 1.000000000000000000, 0.8660254037844387076, 1.000000000000000000, 0.8660254037844387076, 1.000000000000000000, 0.8660254037844387076, 1.000000000000000000, 0.8660254037844387076, 1.000000000000000000, 0.8660254037844387076, 1.000000000000000000, 0.8660254037844387076, 1.000000000000000000, 0.8660254037844387076, 1.000000000000000000, 0.8660254037844387076, 1.000000000000000000, 0.8660254037844387076, 1.000000000000000000, 0.8660254037844387076, 1.000000000000000000, 0.8660254037844387076, 1.000000000000000000, 0.8660254037844387076, 1.000000000000000000, 0.8660254037844387076, 1.000000000000000000, 0.8660254037844387076, 1.000000000000000000, 0.8660254037844387076, 1.000000000000000000, 0.8660254037844387076, 1.000000000000000000, 0.8660254037844387076, 1.000000000000000000, 0.8660254037844387076, 1.000000000000000000, 0.8660254037844387076, 1.000000000000000000, 0.8660254037844387076, 1.000000000000000000, 0.8660254037844387076, 1.000000000000000000, 0.8660254037844387076, 1.000000000000000000, 0.8660254037844387076, 1.000000000000000000, 0.8660254037844387076, 1.000000000000000000, 0.8660254037844387076, 1.000000000000000000, 0.8660254037844387076, 1.000000000000000000, 0.8660254037844387076, 1.000000000000000000, 0.8660254037844387076, 1.000000000000000000, 0.8660254037844387076, 1.000000000000000000, 0.8660254037844387076, 1.000000000000000000, 0.8660254037844387076, 1.000000000000000000, 0.8660254037844387076, 1.000000000000000000, 0.8660254037844387076, 1.000000000000000000, 0.8660254037844387076, 1.000000000000000000, 0.8660254037844387076, 1.000000000000000000, 0.8660254037844387076, 1.000000000000000000, 0.8660254037844387076, 1.000000000000000000, 0.8660254037844387076, 1.000000000000000000, 0.8660254037844387076, 1.000000000000000000, 0.8660254037844387076, 1.000000000000000000, 0.8660254037844387076, 1.000000000000000000, 0.8660254037844387076, 1.000000000000000000, 0.8660254037844387076, 1.000000000000000000, 0.8660254037844387076, 1.000000000000000000, 0.8660254037844387076, 1.000000000000000000, 0.8660254037844387076, 1.000000000000000000, 0.8660254037844387076, 1.000000000000000000, 0.8660254037844387076, 1.000000000000000000, 0.8660254037844387076, 1.000000000000000000, 0.8660254037844387076, 1.000000000000000000, 0.8660254037844387076, 1.000000000000000000, 0.8660254037844387076, 1.000000000000000000, 0.8660254037844387076, 1.000000000000000000, 0.8660254037844387076, 1.000000000000000000, 0.8660254037844387076, 1.000000000000000000, 0.8660254037844387076, 1.000000000000000000, 0.8660254037844387076, 1.000000000000000000, 0.8660254037844387076, 1.000000000000000000, 0.8660254037844387076, 1.000000000000000000, 0.8660254037844387076, 1.000000000000000000, 0.8660254037844387076, 1.000000000000000000, 0.8660254037844387076, 1.000000000000000000, 0.8660254037844387076, 1.000000000000000000, 0.8660254037844387076, 1.000000000000000000, 0.8660254037844387076, 1.000000000000000000, 0.8660254037844387076, 1.000000000000000000, 0.8660254037844387076, 1.000000000000000000, 0.8660254037844387076, 1.000000000000000000, 0.8660254037844387076, 1.000000000000000000, 0.8660254037844387076, 1.000000000000000000, 0.8660254037844387076, 1.000000000000000000, 0.8660254037844387076, 1.000000000000000000, 0.8660254037844387076, 1.000000000000000000, 0.8660254037844387076, 1.000000000000000000, 0.8660254037844387076, 1.000000000000000000, 0.8660254037844387076, 1.000000000000000000, 0.8660254037844387076, 1.000000000000000000, 0.8660254037844387076, 1.000000000000000000, 0.8660254037844387076, 1.000000000000000000, 0.8660254037844387076, 1.000000000000000000, 0.8660254037844387076, 1.000000000000000000, 0.8660254037844387076, 1.000000000000000000, 0.8660254037844387076, 1.000000000000000000, 0.8660254037844387076, 1.000000000000000000, 0.8660254037844387076, 1.000000000000000000, 0.8660254037844387076, 1.000000000000000000, 0.8660254037844387076, 1.000000000000000000, 0.8660254037844387076, 1.000000000000000000, 0.8660254037844387076, 1.000000000000000000, 0.8660254037844387076, 1.000000000000000000, 0.8660254037844387076, 1.000000000000000000, 0.8660254037844387076, 1.000000000000000000, 0.8660254037844387076, 1.000000000000000000, 0.8660254037844387076, 1.000000000000000000, 0.8660254037844387076, 1.000000000000000000, 0.8660254037844387076, 1.000000000000000000, 0.8660254037844387076, 1.000000000000000000, 0.8660254037844387076, 1.000000000000000000, 0.8660254037844387076, 1.000000000000000000, 0.8660254037844387076, 1.000000000000000000, 0.8660254037844387076, 1.000000000000000000, 0.8660254037844387076, 1.000000000000000000, 0.8660254037844387076, 1.000000000000000000, 0.8660254037844387076, 1.000000000000000000, 0.8660254037844387076, 1.000000000000000000, 0.8660254037844387076, 1.000000000000000000, 0.8660254037844387076, 1.000000000000000000, 0.8660254037844387076, 1.000000000000000000, 0.8660254037844387076, 1.000000000000000000, 0.8660254037844387076, 1.000000000000000000, 0.8660254037844387076, 1.000000000000000000, 0.8660254037844387076, 1.000000000000000000, 0.8660254037844387076, 1.000000000000000000, 0.8660254037844387076, 1.000000000000000000, 0.8660254037844387076, 1.000000000000000000, 0.8660254037844387076, 1.000000000000000000, 0.8660254037844387076, 1.000000000000000000, 0.8660254037844387076, 1.000000000000000000, 0.8660254037844387076, 1.000000000000000000, 0.8660254037844387076, 1.000000000000000000, 0.8660254037844387076, 1.000000000000000000, 0.8660254037844387076, 1.000000000000000000, 0.8660254037844387076, 1.000000000000000000, 0.8660254037844387076, 1.000000000000000000, 0.8660254037844387076, 1.000000000000000000, 0.8660254037844387076, 1.000000000000000000, 0.8660254037844387076, 1.000000000000000000, 0.8660254037844387076, 1.000000000000000000, 0.8660254037844387076, 1.000000000000000000, 0.8660254037844387076, 1.000000000000000000, 0.8660254037844387076, 1.000000000000000000, 0.8660254037844387076, 1.000000000000000000, 0.8660254037844387076, 1.000000000000000000, 0.8660254037844387076, 1.000000000000000000, 0.8660254037844387076, 1.000000000000000000, 0.8660254037844387076, 1.000000000000000000, 0.8660254037844387076, 1.000000000000000000, 0.8660254037844387076, 1.000000000000000000, 0.8660254037844387076, 1.000000000000000000, 0.8660254037844387076, 1.000000000000000000, 0.8660254037844387076, 1.000000000000000000, 0.8660254037844387076, 1.000000000000000000, 0.8660254037844387076, 1.000000000000000000, 0.8660254037844387076, 1.000000000000000000, 0.8660254037844387076, 1.000000000000000000, 0.8660254037844387076, 1.000000000000000000, 0.8660254037844387076, 1.000000000000000000, 0.8660254037844387076, 1.000000000000000000, 0.8660254037844387076, 1.000000000000000000, 0.8660254037844387076, 1.000000000000000000, 0.8660254037844387076, 1.000000000000000000, 0.8660254037844387076, 1.000000000000000000, 0.8660254037844387076, 1.000000000000000000, 0.8660254037844387076, 1.000000000000000000, 0.8660254037844387076, 1.000000000000000000, 0.8660254037844387076, 1.000000000000000000, 0.8660254037844387076, 1.000000000000000000, 0.8660254037844387076, 1.000000000000000000, 0.8660254037844387076, 1.000000000000000000, 0.8660254037844387076, 1.000000000000000000, 0.8660254037844387076, 1.000000000000000000, 0.8660254037844387076, 1.000000000000000000, 0.8660254037844387076, 1.000000000000000000, 0.8660254037844387076, 1.000000000000000000, 0.8660254037844387076, 1.000000000000000000, 0.8660254037844387076, 1.000000000000000000, 0.8660254037844387076, 1.000000000000000000, 0.8660254037844387076, 1.000000000000000000, 0.8660254037844387076, 1.000000000000000000, 0.8660254037844387076, 1.000000000000000000, 0.8660254037844387076, 1.000000000000000000, 0.8660254037844387076, 1.000000000000000000, 0.8660254037844387076, 1.000000000000000000, 0.8660254037844387076, 1.000000000000000000, 0.8660254037844387076, 1.000000000000000000, 0.8660254037844387076, 1.000000000000000000, 0.8660254037844387076, 1.000000000000000000, 0.8660254037844387076, 1.000000000000000000, 0.8660254037844387076, 1.000000000000000000, 0.8660254037844387076, 1.000000000000000000, 0.8660254037844387076, 1.000000000000000000, 0.8660254037844387076, 1.000000000000000000, 0.8660254037844387076, 1.000000000000000000, 0.8660254037844387076, 1.000000000000000000, 0.8660254037844387076, 1.000000000000000000, 0.8660254037844387076, 1.000000000000000000, 0.8660254037844387076, 1.000000000000000000, 0.8660254037844387076, 1.000000000000000000, 0.8660254037844387076, 1.000000000000000000, 0.8660254037844387076, 1.000000000000000000, 0.8660254037844387076, 1.000000000000000000, 0.8660254037844387076, 1.000000000000000000, 0.8660254037844387076, 1.000000000000000000, 0.8660254037844387076, 1.000000000000000000, 0.8660254037844387076, 1.000000000000000000, 0.8660254037844387076, 1.000000000000000000, 0.8660254037844387076, 1.000000000000000000, 0.8660254037844387076, 1.000000000000000000, 0.8660254037844387076, 1.000000000000000000, 0.8660254037844387076, 1.000000000000000000, 0.8660254037844387076, 1.000000000000000000, 0.8660254037844387076, 1.000000000000000000, 0.8660254037844387076, 1.000000000000000000, 0.8660254037844387076, 1.000000000000000000, 0.8660254037844387076, 1.000000000000000000, 0.8660254037844387076, 1.000000000000000000, 0.8660254037844387076, 1.000000000000000000, 0.8660254037844387076, 1.000000000000000000, 0.8660254037844387076, 1.000000000000000000, 0.8660254037844387076, 1.000000000000000000, 0.8660254037844387076, 1.000000000000000000, 0.8660254037844387076, 1.000000000000000000, 0.8660254037844387076, 1.000000000000000000, 0.8660254037844387076, 1.000000000000000000, 0.8660254037844387076, 1.000000000000000000, 0.8660254037844387076, 1.000000000000000000, 0.8660254037844387076, 1.000000000000000000, 0.8660254037844387076, 1.000000000000000000, 0.8660254037844387076, 1.000000000000000000, 0.8660254037844387076, 1.000000000000000000, 0.8660254037844387076, 1.000000000000000000, 0.8660254037844387076, 1.000000000000000000, 0.8660254037844387076, 1.000000000000000000, 0.8660254037844387076, 1.000000000000000000, 0.8660254037844387076, 1.000000000000000000, 0.8660254037844387076, 1.000000000000000000, 0.8660254037844387076, 1.000000000000000000, 0.8660254037844387076, 1.000000000000000000, 0.8660254037844387076, 1.000000000000000000, 0.8660254037844387076, 1.000000000000000000, 0.8660254037844387076, 1.000000000000000000, 0.8660254037844387076, 1.000000000000000000, 0.8660254037844387076, 1.000000000000000000, 0.8660254037844387076, 1.000000000000000000, 0.8660254037844387076, 1.000000000000000000, 0.8660254037844387076, 1.000000000000000000, 0.8660254037844387076, 1.000000000000000000, 0.8660254037844387076, 1.000000000000000000, 0.8660254037844387076, 1.000000000000000000, 0.8660254037844387076, 1.000000000000000000, 0.8660254037844387076, 1.000000000000000000, 0.8660254037844387076, 1.000000000000000000, 0.8660254037844387076, 1.000000000000000000, 0.8660254037844387076, 1.000000000000000000, 0.8660254037844387076, 1.000000000000000000, 0.8660254037844387076, 1.000000000000000000, 0.8660254037844387076, 1.000000000000000000, 0.8660254037844387076, 1.000000000000000000, 0.8660254037844387076, 1.000000000000000000, 0.8660254037844387076, 1.000000000000000000, 0.8660254037844387076, 1.000000000000000000, 0.8660254037844387076, 1.000000000000000000, 0.8660254037844387076, 1.000000000000000000, 0.8660254037844387076, 1.000000000000000000, 0.8660254037844387076, 1.000000000000000000, 0.8660254037844387076, 1.000000000000000000, 0.8660254037844387076, 1.000000000000000000, 0.8660254037844387076, 1.000000000000000000, 0.8660254037844387076, 1.000000000000000000, 0.8660254037844387076, 1.000000000000000000, 0.8660254037844387076, 1.000000000000000000, 0.8660254037844387076, 1.000000000000000000, 0.8660254037844387076, 1.000000000000000000, 0.8660254037844387076, 1.000000000000000000, 0.8660254037844387076, 1.000000000000000000, 0.8660254037844387076, 1.000000000000000000, 0.8660254037844387076, 1.000000000000000000, 0.8660254037844387076, 1.000000000000000000, 0.8660254037844387076, 1.000000000000000000, 0.8660254037844387076, 1.000000000000000000, 0.8660254037844387076, 1.000000000000000000, 0.8660254037844387076, 1.000000000000000000, 0.8660254037844387076, 1.000000000000000000, 0.8660254037844387076, 1.000000000000000000, 0.8660254037844387076, 1.000000000000000000, 0.8660254037844387076, 1.000000000000000000, 0.8660254037844387076, 1.000000000000000000, 0.8660254037844387076, 1.000000000000000000, 0.8660254037844387076, 1.000000000000000000, 0.8660254037844387076, 1.000000000000000000, 0.8660254037844387076, 1.000000000000000000, 0.8660254037844387076, 1.000000000000000000, 0.8660254037844387076, 1.000000000000000000, 0.8660254037844387076, 1.000000000000000000, 0.8660254037844387076, 1.000000000000000000, 0.8660254037844387076, 1.000000000000000000, 0.8660254037844387076, 1.000000000000000000, 0.8660254037844387076, 1.000000000000000000, 0.8660254037844387076, 1.000000000000000000, 0.8660254037844387076, 1.000000000000000000, 0.8660254037844387076, 1.000000000000000000, 0.8660254037844387076, 1.000000000000000000, 0.8660254037844387076, 1.000000000000000000, 0.8660254037844387076, 1.000000000000000000, 0.8660254037844387076, 1.000000000000000000, 0.8660254037844387076, 1.000000000000000000, 0.8660254037844387076, 1.000000000000000000, 0.8660254037844387076, 1.000000000000000000, 0.8660254037844387076, 1.000000000000000000, 0.8660254037844387076, 1.000000000000000000, 0.8660254037844387076, 1.000000000000000000, 0.8660254037844387076, 1.000000000000000000, 0.8660254037844387076, 1.000000000000000000, 0.8660254037844387076, 1.000000000000000000, 0.8660254037844387076, 1.000000000000000000, 0.8660254037844387076, 1.000000000000000000, 0.8660254037844387076, 1.000000000000000000, 0.8660254037844387076, 1.000000000000000000, 0.8660254037844387076, 1.000000000000000000, 0.8660254037844387076, 1.000000000000000000, 0.8660254037844387076, 1.000000000000000000, 0.8660254037844387076, 1.000000000000000000, 0.8660254037844387076, 1.000000000000000000, 0.8660254037844387076, 1.000000000000000000, 0.8660254037844387076, 1.000000000000000000, 0.8660254037844387076, 1.000000000000000000, 0.8660254037844387076, 1.000000000000000000, 0.8660254037844387076, 1.000000000000000000, 0.8660254037844387076, 1.000000000000000000, 0.8660254037844387076, 1.000000000000000000, 0.8660254037844387076, 1.000000000000000000, 0.8660254037844387076, 1.000000000000000000, 0.8660254037844387076, 1.000000000000000000, 0.8660254037844387076, 1.000000000000000000, 0.8660254037844387076, 1.000000000000000000, 0.8660254037844387076, 1.000000000000000000, 0.8660254037844387076, 1.000000000000000000, 0.8660254037844387076, 1.000000000000000000, 0.8660254037844387076, 1.000000000000000000, 0.8660254037844387076, 1.000000000000000000, 0.8660254037844387076, 1.000000000000000000, 0.8660254037844387076, 1.000000000000000000, 0.8660254037844387076, 1.000000000000000000, 0.8660254037844387076, 1.000000000000000000, 0.8660254037844387076, 1.000000000000000000, 0.8660254037844387076, 1.000000000000000000, 0.8660254037844387076, 1.000000000000000000, 0.8660254037844387076, 1.000000000000000000, 0.8660254037844387076, 1.000000000000000000, 0.8660254037844387076, 1.000000000000000000, 0.8660254037844387076, 1.000000000000000000, 0.8660254037844387076, 1.000000000000000000, 0.8660254037844387076, 1.000000000000000000, 0.8660254037844387076, 1.000000000000000000, 0.8660254037844387076, 1.000000000000000000, 0.8660254037844387076, 1.000000000000000000, 0.8660254037844387076, 1.000000000000000000, 0.8660254037844387076, 1.000000000000000000, 0.8660254037844387076, 1.000000000000000000, 0.8660254037844387076, 1.000000000000000000, 0.8660254037844387076, 1.000000000000000000, 0.8660254037844387076, 1.000000000000000000, 0.8660254037844387076, 1.000000000000000000, 0.8660254037844387076, 1.000000000000000000, 0.8660254037844387076, 1.000000000000000000, 0.8660254037844387076, 1.000000000000000000, 0.8660254037844387076, 1.000000000000000000, 0.8660254037844387076, 1.000000000000000000, 0.8660254037844387076, 1.000000000000000000, 0.8660254037844387076, 1.000000000000000000, 0.8660254037844387076, 1.000000000000000000, 0.8660254037844387076, 1.000000000000000000, 0.8660254037844387076, 1.000000000000000000, 0.8660254037844387076, 1.000000000000000000, 0.8660254037844387076, 1.000000000000000000, 0.8660254037844387076, 1.000000000000000000, 0.8660254037844387076, 1.000000000000000000, 0.8660254037844387076, 1.000000000000000000, 0.8660254037844387076, 1.000000000000000000, 0.8660254037844387076, 1.000000000000000000, 0.8660254037844387076, 1.000000000000000000, 0.8660254037844387076, 1.000000000000000000, 0.8660254037844387076, 1.000000000000000000, 0.8660254037844387076, 1.000000000000000000, 0.8660254037844387076, 1.000000000000000000, 0.8660254037844387076, 1.000000000000000000, 0.8660254037844387076, 1.000000000000000000, 0.8660254037844387076, 1.000000000000000000, 0.8660254037844387076, 1.000000000000000000, 0.8660254037844387076, 1.000000000000000000, 0.8660254037844387076, 1.000000000000000000, 0.8660254037844387076, 1.000000000000000000, 0.8660254037844387076, 1.000000000000000000 ) ) 
 REPRESENTATION_ITEM ( '' )  );
#41575=CARTESIAN_POINT ( 'NONE',  ( -2.500000000000000444, 7.833333333333334814, -4.330127018922193649 ) ) ;
#41576=CARTESIAN_POINT ( 'NONE',  ( 4.458734124999998549, -56.72916666530107932, -2.574251347313721627 ) ) ;
#41579=CARTESIAN_POINT ( 'NONE',  ( -5.000000000000000000, -37.95833333060213022, -2.886751345948128211 ) ) ;
#41581=CARTESIAN_POINT ( 'NONE',  ( -9.184850993605147944E-16, -151.3750000027311842, 5.000000000000000000 ) ) ;
#41582=CARTESIAN_POINT ( 'NONE',  ( 5.000000000000000000, -38.41666666666667140, -2.886751345948129988 ) ) ;
#41583=CARTESIAN_POINT ( 'NONE',  ( 5.000000000000000888, -148.9375000000000000, -2.071067811865475505 ) ) ;
#41584=CARTESIAN_POINT ( 'NONE',  ( 3.061616997868383141E-16, -143.7500000000000284, -5.000000000000000000 ) ) ;
#41586=FACE_OUTER_BOUND ( 'NONE', #965, .T. ) ;
#41587=CARTESIAN_POINT ( 'NONE',  ( -3.152548672688508926E-16, -57.56249999863439371, -5.148502694627439702 ) ) ;
#41588=CARTESIAN_POINT ( 'NONE',  ( -3.152801135295367096, -150.3125000013655779, -3.152801135295367541 ) ) ;
#41589=CARTESIAN_POINT ( 'NONE',  ( 2.229367062500001939, -71.97916666530107932, 3.861377020970579999 ) ) ;
#41592=AXIS2_PLACEMENT_3D ( 'NONE', #28548, #48167, #38507 ) ;
#41593=CARTESIAN_POINT ( 'NONE',  ( 4.458734125000001214, -22.14583333196773296, 2.574251347313718519 ) ) ;
#41594=CARTESIAN_POINT ( 'NONE',  ( -2.500000000000000444, -61.04166666393547303, -4.330127018922193649 ) ) ;
#41595=ORIENTED_EDGE ( 'NONE', *, *, #41773, .F. ) ;
#41596=ORIENTED_EDGE ( 'NONE', *, *, #28667, .T. ) ;
#41599=CARTESIAN_POINT ( 'NONE',  ( 3.152801135295367541, -153.3125000013656063, -3.152801135295367541 ) ) ;
#41601=CARTESIAN_POINT ( 'NONE',  ( -2.500000000000000444, 2.958333336064520314, -4.330127018922193649 ) ) ;
#41603=CARTESIAN_POINT ( 'NONE',  ( -4.458734124999999437, -50.56249999863440792, 0.000000000000000000 ) ) ;
#41604=ORIENTED_EDGE ( 'NONE', *, *, #37764, .F. ) ;
#41607=EDGE_CURVE ( 'NONE', #11132, #2012, #59320, .T. ) ;
#41609=CARTESIAN_POINT ( 'NONE',  ( 9.457646018065525792E-16, 21.93750000136559208, 5.148502694627439702 ) ) ;
#41612=CARTESIAN_POINT ( 'NONE',  ( 2.730187237215162345E-16, -168.1875000013655779, -4.458734124999999437 ) ) ;
#41613=VERTEX_POINT ( 'NONE', #39217 ) ;
#41615=CARTESIAN_POINT ( 'NONE',  ( 2.499999999999998668, -28.20833333060214798, -4.330127018922193649 ) ) ;
#41618=CYLINDRICAL_SURFACE ( 'NONE', #43911, 5.000000000000000000 ) ;
#41622=CARTESIAN_POINT ( 'NONE',  ( -2.071067811865432873, -139.8125000027311842, -5.000000000000041744 ) ) ;
#41627=CARTESIAN_POINT ( 'NONE',  ( -5.000000000000000000, -158.6250000027311842, -6.123233995736766282E-16 ) ) ;
#41628=VERTEX_POINT ( 'NONE', #58842 ) ;
#41634=CARTESIAN_POINT ( 'NONE',  ( -2.071067811865475061, -146.6875000000000568, -5.000000000000000888 ) ) ;
#41635=ADVANCED_FACE ( 'NONE', ( #320 ), #15743, .T. ) ;
#41639=CARTESIAN_POINT ( 'NONE',  ( 9.457646018065525792E-16, -24.06249999863440436, 5.148502694627439702 ) ) ;
#41640=LINE ( 'NONE', #32640, #49180 ) ;
#41641=CARTESIAN_POINT ( 'NONE',  ( -3.535533905932737309, -150.6250000000000000, -3.535533905932738197 ) ) ;
#41643=CARTESIAN_POINT ( 'NONE',  ( 4.458734124999999437, -152.5000000013656347, 1.846868145590737864 ) ) ;
#41644=ORIENTED_EDGE ( 'NONE', *, *, #2169, .T. ) ;
#41646=CARTESIAN_POINT ( 'NONE',  ( -4.458734124999997661, -52.47916666530107221, 2.574251347313722516 ) ) ;
#41649=CARTESIAN_POINT ( 'NONE',  ( 5.000000000000000888, 23.41666666666666785, 2.886751345948126879 ) ) ;
#41652=CARTESIAN_POINT ( 'NONE',  ( -3.152548672688508926E-16, 1.437500001365596525, -5.148502694627439702 ) ) ;
#41653=CARTESIAN_POINT ( 'NONE',  ( 5.000000000000000000, 19.50000000000000000, -6.123233995736766282E-16 ) ) ;
#41656=CARTESIAN_POINT ( 'NONE',  ( 4.458734125000001214, 17.85416666803225993, 2.574251347313718519 ) ) ;
#41657=CARTESIAN_POINT ( 'NONE',  ( -3.535250795749689387E-16, 3.875000002731186832, -5.773502691896257311 ) ) ;
#41661=CARTESIAN_POINT ( 'NONE',  ( 5.000000000000000888, -168.0625000027312410, -2.071067811865475505 ) ) ;
#41662=CARTESIAN_POINT ( 'NONE',  ( 2.229367062500001939, -44.97916666530106511, 3.861377020970579999 ) ) ;
#41663=CARTESIAN_POINT ( 'NONE',  ( 4.458734125000000326, -163.6250000013656063, -1.846868145590734978 ) ) ;
#41667=CARTESIAN_POINT ( 'NONE',  ( 2.500000000000002220, -44.54166666393547303, 4.330127018922192761 ) ) ;
#41669=ORIENTED_EDGE ( 'NONE', *, *, #35079, .T. ) ;
#41670=CARTESIAN_POINT ( 'NONE',  ( 4.458734124999999437, -17.81249999863440792, -5.460374474430324690E-16 ) ) ;
#41672=CARTESIAN_POINT ( 'NONE',  ( 5.000000000000000000, -88.50000000000000000, -6.123233995736766282E-16 ) ) ;
#41673=CARTESIAN_POINT ( 'NONE',  ( 1.846868145590736310, -164.6250000013655779, 4.458734124999999437 ) ) ;
#41674=CARTESIAN_POINT ( 'NONE',  ( -2.500000000000000444, -19.16666666666666430, -4.330127018922193649 ) ) ;
#41677=CARTESIAN_POINT ( 'NONE',  ( -4.458734124999999437, -33.64583333196772941, -2.574251347313719407 ) ) ;
#41678=CARTESIAN_POINT ( 'NONE',  ( -3.535533905932737309, -147.7500000027311842, -3.535533905932738197 ) ) ;
#41680=ORIENTED_EDGE ( 'NONE', *, *, #3660, .F. ) ;
#41684=EDGE_CURVE ( 'NONE', #52679, #34612, #28507, .T. ) ;
#41688=CARTESIAN_POINT ( 'NONE',  ( -1.339745962155610925, -25.79465819873852084, 5.000000000000000000 ) ) ;
#41690=CARTESIAN_POINT ( 'NONE',  ( 9.457646018065525792E-16, -78.31249999863442213, 5.148502694627439702 ) ) ;
#41692=CARTESIAN_POINT ( 'NONE',  ( 1.339745962155612702, 22.70534180126147916, -5.000000000000000000 ) ) ;
#41695=CARTESIAN_POINT ( 'NONE',  ( 9.457646018065525792E-16, -44.06249999863439371, 5.148502694627439702 ) ) ;
#41696=CARTESIAN_POINT ( 'NONE',  ( -5.000000000000000000, 20.99999999999999645, 0.000000000000000000 ) ) ;
#41698=DIRECTION ( 'NONE',  ( -0.000000000000000000, 1.000000000000000000, -0.000000000000000000 ) ) ;
#41703=CARTESIAN_POINT ( 'NONE',  ( -2.229367062499996610, -79.39583333196773651, 3.861377020970582219 ) ) ;
#41704=CYLINDRICAL_SURFACE ( 'NONE', #48655, 5.000000000000000000 ) ;
#41707=ORIENTED_EDGE ( 'NONE', *, *, #60320, .F. ) ;
#41712=CARTESIAN_POINT ( 'NONE',  ( -4.458734124999999437, 13.43750000136559386, 0.000000000000000000 ) ) ;
#41718=CARTESIAN_POINT ( 'NONE',  ( 5.000000000000000000, -38.37499999726881583, -6.123233995736766282E-16 ) ) ;
#41720=CARTESIAN_POINT ( 'NONE',  ( -2.229367062500000163, -7.479166665301073991, -3.861377020970580443 ) ) ;
#41722=ORIENTED_EDGE ( 'NONE', *, *, #13736, .T. ) ;
#41723=CARTESIAN_POINT ( 'NONE',  ( -2.229367062500000163, -35.72916666530107221, -3.861377020970580443 ) ) ;
#41724=( BOUNDED_CURVE ( )  B_SPLINE_CURVE ( 2, ( #8514, #51950, #3070, #47122, #27493, #8827, #52583, #22687, #43224 ),
 .UNSPECIFIED., .F., .F. ) 
 B_SPLINE_CURVE_WITH_KNOTS ( ( 3, 2, 2, 2, 3 ),
 ( 0.05208333333333333565, 0.05277777777777777762, 0.05416666666666666852, 0.05555555555555555247, 0.05625000000000000139 ),
 .UNSPECIFIED. ) 
 CURVE ( )  GEOMETRIC_REPRESENTATION_ITEM ( )  RATIONAL_B_SPLINE_CURVE ( ( 0.9330127018922192983, 0.9330127018922196314, 1.000000000000000000, 0.8660254037844387076, 1.000000000000000000, 0.8660254037844387076, 1.000000000000000000, 0.9330127018922189652, 0.9330127018922192983 ) ) 
 REPRESENTATION_ITEM ( '' )  );
#41726=CARTESIAN_POINT ( 'NONE',  ( 1.975475456537005874E-15, -76.75000000000000000, 5.000000000000000000 ) ) ;
#41729=VECTOR ( 'NONE', #36896, 1000.000000000000000 ) ;
#41730=CARTESIAN_POINT ( 'NONE',  ( -3.152801135295367096, -148.3125000013655779, -3.152801135295367541 ) ) ;
#41731=CARTESIAN_POINT ( 'NONE',  ( 4.458734124999999437, 21.18750000136559208, -5.460374474430324690E-16 ) ) ;
#41733=CARTESIAN_POINT ( 'NONE',  ( 5.000000000000000888, 1.416666666666666741, 2.886751345948126879 ) ) ;
#41734=CARTESIAN_POINT ( 'NONE',  ( 4.458734124999999437, -85.06249999863439371, -5.460374474430324690E-16 ) ) ;
#41736=CARTESIAN_POINT ( 'NONE',  ( 2.499999999999998668, -72.20833333060214443, -4.330127018922193649 ) ) ;
#41737=CARTESIAN_POINT ( 'NONE',  ( 5.000000000000000000, 16.70833333606451987, -2.886751345948129988 ) ) ;
#41741=CARTESIAN_POINT ( 'NONE',  ( 0.000000000000000000, -170.0000000000000000, 0.000000000000000000 ) ) ;
#41742=CARTESIAN_POINT ( 'NONE',  ( 2.499999999999998668, -23.33333333333333215, -4.330127018922193649 ) ) ;
#41743=CARTESIAN_POINT ( 'NONE',  ( 4.458734124999998549, -28.72916666530107221, -2.574251347313721627 ) ) ;
#41744=CARTESIAN_POINT ( 'NONE',  ( -2.229367062500000163, -86.47916666530107932, -3.861377020970580443 ) ) ;
#41745=EDGE_CURVE ( 'NONE', #54676, #38746, #48225, .T. ) ;
#41746=CARTESIAN_POINT ( 'NONE',  ( 5.000000000000000000, -31.37499999726880873, -6.123233995736766282E-16 ) ) ;
#41747=CARTESIAN_POINT ( 'NONE',  ( 9.457646018065525792E-16, -55.06249999863439371, 5.148502694627439702 ) ) ;
#41750=CARTESIAN_POINT ( 'NONE',  ( 4.458734124999998549, -9.979166665301068662, -2.574251347313721627 ) ) ;
#41751=VERTEX_POINT ( 'NONE', #45648 ) ;
#41752=CARTESIAN_POINT ( 'NONE',  ( 5.000000000000000000, -69.41666666666667140, -2.886751345948129988 ) ) ;
#41755=( BOUNDED_CURVE ( )  B_SPLINE_CURVE ( 2, ( #53188, #48355, #23613, #62544, #58329, #48661, #28109, #9121, #43209 ),
 .UNSPECIFIED., .F., .F. ) 
 B_SPLINE_CURVE_WITH_KNOTS ( ( 3, 2, 2, 2, 3 ),
 ( 0.3937499999999999889, 0.3944444444444444309, 0.3958333333333333148, 0.3972222222222221988, 0.3979166666666666963 ),
 .UNSPECIFIED. ) 
 CURVE ( )  GEOMETRIC_REPRESENTATION_ITEM ( )  RATIONAL_B_SPLINE_CURVE ( ( 0.9330127018922194093, 0.9330127018922194093, 1.000000000000000000, 0.8660254037844387076, 1.000000000000000000, 0.8660254037844387076, 1.000000000000000000, 0.9330127018922167448, 0.9330127018922194093 ) ) 
 REPRESENTATION_ITEM ( '' )  );
#41756=EDGE_CURVE ( 'NONE', #43111, #7190, #15364, .T. ) ;
#41757=CARTESIAN_POINT ( 'NONE',  ( -5.000000000000000000, -78.95833333060213022, -2.886751345948128211 ) ) ;
#41758=EDGE_LOOP ( 'NONE', ( #39760, #59721, #52398, #27048 ) ) ;
#41760=ADVANCED_FACE ( 'NONE', ( #45962 ), #46921, .T. ) ;
#41761=CARTESIAN_POINT ( 'NONE',  ( -3.152548672688508926E-16, -18.81249999863440792, -5.148502694627439702 ) ) ;
#41763=CARTESIAN_POINT ( 'NONE',  ( -4.458734124999999437, -51.56249999863440792, 0.000000000000000000 ) ) ;
#41765=CARTESIAN_POINT ( 'NONE',  ( -8.190561711645485556E-16, -139.6875000013656063, 4.458734124999999437 ) ) ;
#41770=CARTESIAN_POINT ( 'NONE',  ( -5.000000000000000888, -155.5625000000000853, -2.071067811865475949 ) ) ;
#41772=AXIS2_PLACEMENT_3D ( 'NONE', #24643, #33976, #58737 ) ;
#41773=EDGE_CURVE ( 'NONE', #35874, #34281, #13848, .T. ) ;
#41774=CARTESIAN_POINT ( 'NONE',  ( 1.062108568985190270E-13, -13.12499999726881583, -4.999999999999999112 ) ) ;
#41778=EDGE_CURVE ( 'NONE', #37182, #24836, #4120, .T. ) ;
#41779=CARTESIAN_POINT ( 'NONE',  ( -4.458734125000001214, -150.1250000013655779, 1.846868145590734089 ) ) ;
#41784=CARTESIAN_POINT ( 'NONE',  ( -4.458734124999998549, -61.47916666530107221, 2.574251347313722516 ) ) ;
#41785=DIRECTION ( 'NONE',  ( 0.000000000000000000, 0.000000000000000000, 1.000000000000000000 ) ) ;
#41787=CARTESIAN_POINT ( 'NONE',  ( 4.458734124999999437, -143.3750000013656063, -1.846868145590734978 ) ) ;
#41789=VERTEX_POINT ( 'NONE', #42393 ) ;
#41790=CARTESIAN_POINT ( 'NONE',  ( -9.184850993605147944E-16, -164.3750000027311842, 5.000000000000000000 ) ) ;
#41791=DIRECTION ( 'NONE',  ( -0.000000000000000000, 1.000000000000000000, -0.000000000000000000 ) ) ;
#41796=CARTESIAN_POINT ( 'NONE',  ( 4.458734124999999437, 27.93750000136559208, -5.460374474430324690E-16 ) ) ;
#41797=FACE_OUTER_BOUND ( 'NONE', #28151, .T. ) ;
#41802=CARTESIAN_POINT ( 'NONE',  ( 6.123233995736766282E-16, -170.0000000000000000, -5.000000000000000000 ) ) ;
#41803=CARTESIAN_POINT ( 'NONE',  ( -2.498395430326213474E-14, 21.24999999999999289, 5.000000000000000000 ) ) ;
#41804=CARTESIAN_POINT ( 'NONE',  ( -4.458734124999999437, 7.604166668032259935, -2.574251347313719407 ) ) ;
#41806=CARTESIAN_POINT ( 'NONE',  ( 2.229367062499998831, -19.89583333196774007, -3.861377020970580887 ) ) ;
#41808=CARTESIAN_POINT ( 'NONE',  ( 1.846868145590735200, -161.2500000013655779, -4.458734125000000326 ) ) ;
#41812=CARTESIAN_POINT ( 'NONE',  ( 2.229367062499998831, -38.64583333196773651, -3.861377020970580887 ) ) ;
#41813=CARTESIAN_POINT ( 'NONE',  ( 5.000000000000000000, -60.50000000000000000, -6.123233995736766282E-16 ) ) ;
#41814=CARTESIAN_POINT ( 'NONE',  ( 2.229367062500001939, -67.22916666530106511, 3.861377020970579999 ) ) ;
#41817=CARTESIAN_POINT ( 'NONE',  ( 1.339745962155615144, -36.58034179853029855, 4.999999999999999112 ) ) ;
#41819=FACE_OUTER_BOUND ( 'NONE', #52790, .T. ) ;
#41820=VECTOR ( 'NONE', #2287, 1000.000000000000000 ) ;
#41822=CARTESIAN_POINT ( 'NONE',  ( -2.500000000000000444, -5.166666666666666963, -4.330127018922193649 ) ) ;
#41824=CARTESIAN_POINT ( 'NONE',  ( 4.458734124999999437, -71.81249999863439371, -5.460374474430324690E-16 ) ) ;
#41827=CARTESIAN_POINT ( 'NONE',  ( -2.500000000000000444, -15.04166666393548191, -4.330127018922193649 ) ) ;
#41828=CARTESIAN_POINT ( 'NONE',  ( -4.458734124999998549, -40.22916666530107932, 2.574251347313722516 ) ) ;
#41829=ORIENTED_EDGE ( 'NONE', *, *, #3867, .T. ) ;
#41830=VECTOR ( 'NONE', #8178, 1000.000000000000000 ) ;
#41832=CARTESIAN_POINT ( 'NONE',  ( -4.458734124999998549, 6.520833334698930450, 2.574251347313722516 ) ) ;
#41833=VERTEX_POINT ( 'NONE', #17951 ) ;
#41834=CARTESIAN_POINT ( 'NONE',  ( -4.999999999999999112, -53.91666666666667140, 2.886751345948131764 ) ) ;
#41835=CARTESIAN_POINT ( 'NONE',  ( -4.458734125000000326, -160.2500000013656063, -1.846868145590735644 ) ) ;
#41838=CARTESIAN_POINT ( 'NONE',  ( -2.229367062499996610, -81.14583333196773651, 3.861377020970582219 ) ) ;
#41839=CARTESIAN_POINT ( 'NONE',  ( -5.000000000000000000, -166.5000000000000000, -6.123233995736766282E-16 ) ) ;
#41840=CARTESIAN_POINT ( 'NONE',  ( 4.458734124999998549, -88.72916666530106511, -2.574251347313721627 ) ) ;
#41842=CARTESIAN_POINT ( 'NONE',  ( -4.458734124999999437, -0.5624999986344053626, 0.000000000000000000 ) ) ;
#41843=CARTESIAN_POINT ( 'NONE',  ( 4.458734124999999437, -37.06249999863440792, -5.460374474430324690E-16 ) ) ;
#41844=CARTESIAN_POINT ( 'NONE',  ( 2.500000000000002220, -72.66666666666667140, 4.330127018922192761 ) ) ;
#41846=CARTESIAN_POINT ( 'NONE',  ( -9.184850993605147944E-16, -145.2500000000000284, 5.000000000000000000 ) ) ;
#41848=CARTESIAN_POINT ( 'NONE',  ( -5.000000000000000888, -141.5625000000000568, -2.071067811865475949 ) ) ;
#41849=DIRECTION ( 'NONE',  ( -0.000000000000000000, 1.000000000000000000, -0.000000000000000000 ) ) ;
#41850=CARTESIAN_POINT ( 'NONE',  ( -4.458734124999999437, -68.56249999863439371, 0.000000000000000000 ) ) ;
#41853=CARTESIAN_POINT ( 'NONE',  ( 2.071067811865412445, -163.8125000000000000, -5.000000000000063949 ) ) ;
#41855=EDGE_CURVE ( 'NONE', #28232, #14051, #20814, .T. ) ;
#41859=CARTESIAN_POINT ( 'NONE',  ( 4.458734125000001214, 1.104166668032261711, 2.574251347313718519 ) ) ;
#41861=CARTESIAN_POINT ( 'NONE',  ( -4.458734124999999437, -157.9375000013655779, -5.460374474430324690E-16 ) ) ;
#41868=VECTOR ( 'NONE', #62481, 1000.000000000000000 ) ;
#41872=DIRECTION ( 'NONE',  ( -0.000000000000000000, 1.000000000000000000, -0.000000000000000000 ) ) ;
#41875=CARTESIAN_POINT ( 'NONE',  ( 4.458734124999998549, 22.27083333469892779, -2.574251347313721627 ) ) ;
#41877=CARTESIAN_POINT ( 'NONE',  ( -4.458734124999999437, -1.645833331967737401, -2.574251347313719407 ) ) ;
#41880=CARTESIAN_POINT ( 'NONE',  ( 2.071067811865476394, -142.3125000027312410, 5.000000000000000000 ) ) ;
#41881=CARTESIAN_POINT ( 'NONE',  ( 1.975475456537005874E-15, -51.75000000000000000, 5.000000000000000000 ) ) ;
#41889=CARTESIAN_POINT ( 'NONE',  ( 1.846868145590736310, -158.8750000013655779, 4.458734124999997661 ) ) ;
#41891=CARTESIAN_POINT ( 'NONE',  ( -5.000000000000000888, -147.5625000000000853, -2.071067811865475949 ) ) ;
#41893=CARTESIAN_POINT ( 'NONE',  ( -2.229367062499996610, 15.60416666803225993, 3.861377020970582219 ) ) ;
#41894=ORIENTED_EDGE ( 'NONE', *, *, #16203, .F. ) ;
#41898=CARTESIAN_POINT ( 'NONE',  ( 2.499999999999998668, -16.33333333333333215, -4.330127018922193649 ) ) ;
#41899=CARTESIAN_POINT ( 'NONE',  ( 5.000000000000000000, 6.583333333333333037, -2.886751345948129988 ) ) ;
#41900=CARTESIAN_POINT ( 'NONE',  ( 4.458734124999998549, -57.72916666530107932, -2.574251347313721627 ) ) ;
#41904=CARTESIAN_POINT ( 'NONE',  ( 6.123233995736766282E-16, -170.0000000000000000, -5.000000000000000000 ) ) ;
#41907=CARTESIAN_POINT ( 'NONE',  ( 5.000000000000000000, -41.49999999999999289, -6.123233995736766282E-16 ) ) ;
#41908=CARTESIAN_POINT ( 'NONE',  ( 0.000000000000000000, -170.0000000000000000, 0.000000000000000000 ) ) ;
#41912=AXIS2_PLACEMENT_3D ( 'NONE', #22352, #2118, #32303 ) ;
#41913=DIRECTION ( 'NONE',  ( -0.000000000000000000, 1.000000000000000000, -0.000000000000000000 ) ) ;
#41914=CARTESIAN_POINT ( 'NONE',  ( -3.152548672688508926E-16, -64.56249999863440792, -5.148502694627439702 ) ) ;
#41915=CARTESIAN_POINT ( 'NONE',  ( 4.458734124999999437, -153.6875000013656063, 0.000000000000000000 ) ) ;
#41916=CARTESIAN_POINT ( 'NONE',  ( 4.458734124999998549, -72.72916666530106511, -2.574251347313721627 ) ) ;
#41919=CARTESIAN_POINT ( 'NONE',  ( 4.458734124999998549, -20.97916666530107221, -2.574251347313721627 ) ) ;
#41920=CARTESIAN_POINT ( 'NONE',  ( 5.000000000000000000, -62.37499999726880873, -6.123233995736766282E-16 ) ) ;
#41922=FACE_OUTER_BOUND ( 'NONE', #52758, .T. ) ;
#41927=CARTESIAN_POINT ( 'NONE',  ( 2.730187237215162345E-16, -153.1875000013656063, -4.458734124999999437 ) ) ;
#41931=CARTESIAN_POINT ( 'NONE',  ( -2.499999999999996447, -55.70833333060214443, 4.330127018922195425 ) ) ;
#41932=CARTESIAN_POINT ( 'NONE',  ( -4.458734124999999437, -51.64583333196773651, -2.574251347313719407 ) ) ;
#41937=CARTESIAN_POINT ( 'NONE',  ( 4.458734124999998549, 21.27083333469892779, -2.574251347313721627 ) ) ;
#41940=CARTESIAN_POINT ( 'NONE',  ( -4.458734124999999437, -167.9375000013655779, -5.460374474430324690E-16 ) ) ;
#41941=VERTEX_POINT ( 'NONE', #58135 ) ;
#41944=DIRECTION ( 'NONE',  ( -0.000000000000000000, 1.000000000000000000, -0.000000000000000000 ) ) ;
#41949=CARTESIAN_POINT ( 'NONE',  ( -2.500000000000000444, 18.83333333333333215, -4.330127018922193649 ) ) ;
#41952=VERTEX_POINT ( 'NONE', #52064 ) ;
#41954=CARTESIAN_POINT ( 'NONE',  ( 6.123233995736766282E-16, -170.0000000000000000, -5.000000000000000000 ) ) ;
#41956=CARTESIAN_POINT ( 'NONE',  ( 2.071067811865476394, -154.3125000027312410, 5.000000000000000000 ) ) ;
#41959=ADVANCED_FACE ( 'NONE', ( #38215 ), #57838, .T. ) ;
#41960=AXIS2_PLACEMENT_3D ( 'NONE', #21683, #61876, #32265 ) ;
#41964=CARTESIAN_POINT ( 'NONE',  ( 3.061616997868383141E-16, -147.7500000000000284, -5.000000000000000000 ) ) ;
#41968=CARTESIAN_POINT ( 'NONE',  ( -4.458734124999997661, -26.22916666530106866, 2.574251347313722516 ) ) ;
#41969=CARTESIAN_POINT ( 'NONE',  ( 1.339745962155612702, 14.70534180126147916, -5.000000000000000000 ) ) ;
#41970=CARTESIAN_POINT ( 'NONE',  ( 1.339745962155612702, 18.83034180399265978, -5.000000000000000000 ) ) ;
#41972=CARTESIAN_POINT ( 'NONE',  ( -1.846868145590737420, -148.7500000013656063, 4.458734124999999437 ) ) ;
#41973=EDGE_LOOP ( 'NONE', ( #2457, #7357, #37527, #18991 ) ) ;
#41975=CARTESIAN_POINT ( 'NONE',  ( -4.458734124999999437, -52.64583333196773651, -2.574251347313719407 ) ) ;
#41978=CARTESIAN_POINT ( 'NONE',  ( -3.535250795749689387E-16, 21.75000000000000000, -5.773502691896257311 ) ) ;
#41980=DIRECTION ( 'NONE',  ( -0.000000000000000000, 1.000000000000000000, -0.000000000000000000 ) ) ;
#41981=CARTESIAN_POINT ( 'NONE',  ( 4.458734125000001214, -0.8958333319677401763, 2.574251347313718519 ) ) ;
#41982=ADVANCED_FACE ( 'NONE', ( #27606 ), #3181, .T. ) ;
#41983=CARTESIAN_POINT ( 'NONE',  ( 1.975475456537005874E-15, -0.7499999999999996669, 5.000000000000000000 ) ) ;
#41984=EDGE_CURVE ( 'NONE', #26202, #2867, #16686, .T. ) ;
#41986=DIRECTION ( 'NONE',  ( 0.000000000000000000, 0.000000000000000000, 1.000000000000000000 ) ) ;
#41987=CARTESIAN_POINT ( 'NONE',  ( -2.229367062499996610, 14.60416666803226171, 3.861377020970582219 ) ) ;
#41988=CARTESIAN_POINT ( 'NONE',  ( -5.000000000000000000, 3.041666669397851130, -2.886751345948128211 ) ) ;
#41992=CARTESIAN_POINT ( 'NONE',  ( -5.000000000000000000, -71.08333333333332860, -2.886751345948128211 ) ) ;
#41993=CARTESIAN_POINT ( 'NONE',  ( -4.458734124999999437, -48.31249999863440792, 0.000000000000000000 ) ) ;
#41994=CARTESIAN_POINT ( 'NONE',  ( 1.846868145590735200, -165.5000000013655779, -4.458734125000000326 ) ) ;
#41995=CARTESIAN_POINT ( 'NONE',  ( 2.500000000000002220, -47.54166666393547303, 4.330127018922192761 ) ) ;
#41997=CARTESIAN_POINT ( 'NONE',  ( -4.458734124999999437, -25.31249999863440792, 0.000000000000000000 ) ) ;
#41999=CARTESIAN_POINT ( 'NONE',  ( 2.500000000000002220, -86.66666666666667140, 4.330127018922192761 ) ) ;
#42000=CARTESIAN_POINT ( 'NONE',  ( 1.846868145590736310, -162.6250000013655779, 4.458734124999999437 ) ) ;
#42003=CARTESIAN_POINT ( 'NONE',  ( -4.458734124999999437, -30.64583333196774007, -2.574251347313719407 ) ) ;
#42004=CARTESIAN_POINT ( 'NONE',  ( -4.999999999999998224, 20.20833333606451987, 2.886751345948131764 ) ) ;
#42006=ADVANCED_FACE ( 'NONE', ( #48790 ), #59091, .T. ) ;
#42009=CARTESIAN_POINT ( 'NONE',  ( -6.972266317189433020E-16, -59.25000000000000000, -5.000000000000000000 ) ) ;
#42010=ORIENTED_EDGE ( 'NONE', *, *, #8635, .T. ) ;
#42011=CARTESIAN_POINT ( 'NONE',  ( -1.339745962155610925, -59.66965819600732601, 5.000000000000000000 ) ) ;
#42013=CARTESIAN_POINT ( 'NONE',  ( 4.458734124999999437, -80.06249999863440792, -5.460374474430324690E-16 ) ) ;
#42017=LINE ( 'NONE', #47173, #63060 ) ;
#42021=AXIS2_PLACEMENT_3D ( 'NONE', #19732, #34855, #1098 ) ;
#42023=CARTESIAN_POINT ( 'NONE',  ( 5.000000000000000000, -154.1875000027312126, 2.071067811865478614 ) ) ;
#42026=DIRECTION ( 'NONE',  ( -0.000000000000000000, 1.000000000000000000, -0.000000000000000000 ) ) ;
#42027=FACE_OUTER_BOUND ( 'NONE', #4273, .T. ) ;
#42028=CARTESIAN_POINT ( 'NONE',  ( -2.229367062500000163, -76.72916666530106511, -3.861377020970580443 ) ) ;
#42031=VERTEX_POINT ( 'NONE', #49749 ) ;
#42033=CARTESIAN_POINT ( 'NONE',  ( -5.000000000000000000, -163.6250000027311842, -6.123233995736766282E-16 ) ) ;
#42035=EDGE_CURVE ( 'NONE', #6571, #59835, #244, .T. ) ;
#42036=CARTESIAN_POINT ( 'NONE',  ( 2.229367062499998831, 12.10416666803226171, -3.861377020970580887 ) ) ;
#42044=CARTESIAN_POINT ( 'NONE',  ( -1.339745962155610925, -21.66965819600733312, 5.000000000000000000 ) ) ;
#42045=CARTESIAN_POINT ( 'NONE',  ( -2.229367062499996610, -9.145833331967736513, 3.861377020970582219 ) ) ;
#42046=ORIENTED_EDGE ( 'NONE', *, *, #63292, .T. ) ;
#42047=CARTESIAN_POINT ( 'NONE',  ( 2.229367062499998831, -34.89583333196772941, -3.861377020970580887 ) ) ;
#42053=CARTESIAN_POINT ( 'NONE',  ( -8.190561711645485556E-16, -150.9375000013656063, 4.458734124999999437 ) ) ;
#42054=CARTESIAN_POINT ( 'NONE',  ( -4.458734124999998549, 15.77083333469892601, 2.574251347313722516 ) ) ;
#42055=CARTESIAN_POINT ( 'NONE',  ( 2.500000000000002220, -53.66666666666667140, 4.330127018922192761 ) ) ;
#42058=CARTESIAN_POINT ( 'NONE',  ( 2.229367062500001939, -85.22916666530107932, 3.861377020970579999 ) ) ;
#42060=DIRECTION ( 'NONE',  ( -0.000000000000000000, 1.000000000000000000, -0.000000000000000000 ) ) ;
#42061=CARTESIAN_POINT ( 'NONE',  ( 5.000000000000000888, 21.54166666939785202, 2.886751345948126879 ) ) ;
#42063=CARTESIAN_POINT ( 'NONE',  ( 5.000000000000000000, -35.50000000000000711, -6.123233995736766282E-16 ) ) ;
#42064=EDGE_CURVE ( 'NONE', #28458, #63093, #38818, .T. ) ;
#42066=CYLINDRICAL_SURFACE ( 'NONE', #47074, 5.000000000000000000 ) ;
#42067=CARTESIAN_POINT ( 'NONE',  ( 5.000000000000000000, -29.41666666666666785, -2.886751345948129988 ) ) ;
#42068=CARTESIAN_POINT ( 'NONE',  ( -4.458734124999999437, -30.39583333196773651, -2.574251347313719407 ) ) ;
#42070=CARTESIAN_POINT ( 'NONE',  ( 5.000000000000000888, -26.45833333060214443, 2.886751345948126879 ) ) ;
#42071=CARTESIAN_POINT ( 'NONE',  ( -4.458734124999998549, -60.22916666530106511, 2.574251347313722516 ) ) ;
#42072=VERTEX_POINT ( 'NONE', #30442 ) ;
#42074=CARTESIAN_POINT ( 'NONE',  ( -2.229367062499996610, -10.39583333196773829, 3.861377020970582219 ) ) ;
#42075=ORIENTED_EDGE ( 'NONE', *, *, #2339, .F. ) ;
#42076=CARTESIAN_POINT ( 'NONE',  ( 1.060575238724906964E-15, -70.74999999999998579, 5.773502691896257311 ) ) ;
#42079=CARTESIAN_POINT ( 'NONE',  ( -5.000000000000000000, -76.95833333060214443, -2.886751345948128211 ) ) ;
#42084=CARTESIAN_POINT ( 'NONE',  ( -4.458734124999999437, -15.64583333196773474, -2.574251347313719407 ) ) ;
#42085=CARTESIAN_POINT ( 'NONE',  ( -2.229367062500000163, -57.72916666530107932, -3.861377020970580443 ) ) ;
#42086=CARTESIAN_POINT ( 'NONE',  ( -2.499999999999996447, -23.83333333333333215, 4.330127018922195425 ) ) ;
#42087=CARTESIAN_POINT ( 'NONE',  ( -4.458734124999999437, -139.9375000013656063, -5.460374474430324690E-16 ) ) ;
#42089=LINE ( 'NONE', #57224, #33785 ) ;
#42091=CARTESIAN_POINT ( 'NONE',  ( 3.061616997868383141E-16, -166.7500000000000000, -5.000000000000000000 ) ) ;
#42096=CARTESIAN_POINT ( 'NONE',  ( -8.190561711645485556E-16, -147.9375000013656063, 4.458734124999999437 ) ) ;
#42099=CARTESIAN_POINT ( 'NONE',  ( 2.229367062499998831, -61.89583333196774362, -3.861377020970580887 ) ) ;
#42101=CARTESIAN_POINT ( 'NONE',  ( -1.339745962155613812, -43.08034179853029144, -5.000000000000000000 ) ) ;
#42102=CARTESIAN_POINT ( 'NONE',  ( -4.458734124999999437, -144.9375000013656063, -5.460374474430324690E-16 ) ) ;
#42104=( BOUNDED_CURVE ( )  B_SPLINE_CURVE ( 2, ( #52344, #27882, #23068, #8898, #42673, #14348, #33970, #62312, #4385 ),
 .UNSPECIFIED., .F., .F. ) 
 B_SPLINE_CURVE_WITH_KNOTS ( ( 3, 2, 2, 2, 3 ),
 ( 0.4145833333333333592, 0.4152777777777778012, 0.4166666666666666852, 0.4180555555555555691, 0.4187500000000000111 ),
 .UNSPECIFIED. ) 
 CURVE ( )  GEOMETRIC_REPRESENTATION_ITEM ( )  RATIONAL_B_SPLINE_CURVE ( ( 0.9330127018922194093, 0.9330127018922220739, 1.000000000000000000, 0.8660254037844387076, 1.000000000000000000, 0.8660254037844387076, 1.000000000000000000, 0.9330127018922194093, 0.9330127018922194093 ) ) 
 REPRESENTATION_ITEM ( '' )  );
#42110=CARTESIAN_POINT ( 'NONE',  ( 2.500000000000002220, 4.458333336064518093, 4.330127018922192761 ) ) ;
#42112=CARTESIAN_POINT ( 'NONE',  ( 2.229367062499998831, 29.10416666803225993, -3.861377020970580887 ) ) ;
#42115=EDGE_CURVE ( 'NONE', #45853, #40725, #11780, .T. ) ;
#42116=EDGE_CURVE ( 'NONE', #18888, #49819, #56139, .T. ) ;
#42121=CARTESIAN_POINT ( 'NONE',  ( -2.229367062499996610, 8.854166668032261711, 3.861377020970582219 ) ) ;
#42123=CARTESIAN_POINT ( 'NONE',  ( 4.458734124999998549, -19.97916666530107221, -2.574251347313721627 ) ) ;
#42125=CARTESIAN_POINT ( 'NONE',  ( 3.152801135295367541, -158.3125000013656063, -3.152801135295367541 ) ) ;
#42126=CARTESIAN_POINT ( 'NONE',  ( -2.500000000000000444, 28.95833333606451987, -4.330127018922193649 ) ) ;
#42129=EDGE_CURVE ( 'NONE', #2367, #24664, #21191, .T. ) ;
#42131=CARTESIAN_POINT ( 'NONE',  ( 2.229367062500001939, -40.97916666530107221, 3.861377020970579999 ) ) ;
#42134=CARTESIAN_POINT ( 'NONE',  ( -4.458734124999997661, -66.47916666530106511, 2.574251347313722516 ) ) ;
#42137=EDGE_CURVE ( 'NONE', #11132, #41205, #2163, .T. ) ;
#42139=ORIENTED_EDGE ( 'NONE', *, *, #37737, .F. ) ;
#42140=CARTESIAN_POINT ( 'NONE',  ( -2.498395430326213474E-14, 15.37500000273118239, 5.000000000000000000 ) ) ;
#42142=( BOUNDED_CURVE ( )  B_SPLINE_CURVE ( 2, ( #12287, #12598, #50572, #2968, #21938, #22261, #6515, #16793, #16156 ),
 .UNSPECIFIED., .F., .F. ) 
 B_SPLINE_CURVE_WITH_KNOTS ( ( 3, 2, 2, 2, 3 ),
 ( 0.8812499999999999778, 0.8819444444444444198, 0.8833333333333333037, 0.8847222222222221877, 0.8854166666666666297 ),
 .UNSPECIFIED. ) 
 CURVE ( )  GEOMETRIC_REPRESENTATION_ITEM ( )  RATIONAL_B_SPLINE_CURVE ( ( 0.9330127018922194093, 0.9330127018922194093, 1.000000000000000000, 0.8660254037844387076, 1.000000000000000000, 0.8660254037844387076, 1.000000000000000000, 0.9330127018922194093, 0.9330127018922194093 ) ) 
 REPRESENTATION_ITEM ( '' )  );
#42143=CARTESIAN_POINT ( 'NONE',  ( 3.535533905932738197, -144.0000000027311842, -3.535533905932738197 ) ) ;
#42144=CARTESIAN_POINT ( 'NONE',  ( -4.999999999999999112, -7.916666666666668739, 2.886751345948131764 ) ) ;
#42146=VECTOR ( 'NONE', #21653, 1000.000000000000000 ) ;
#42147=CARTESIAN_POINT ( 'NONE',  ( -4.458734124999999437, -70.31249999863439371, 0.000000000000000000 ) ) ;
#42149=CARTESIAN_POINT ( 'NONE',  ( -2.500000000000000444, -14.04166666393548013, -4.330127018922193649 ) ) ;
#42150=CARTESIAN_POINT ( 'NONE',  ( 2.229367062500001939, -43.97916666530106511, 3.861377020970579999 ) ) ;
#42153=CARTESIAN_POINT ( 'NONE',  ( 4.458734125000001214, 5.854166668032262599, 2.574251347313718519 ) ) ;
#42155=CARTESIAN_POINT ( 'NONE',  ( 1.339745962155615144, -81.70534180126146850, 4.999999999999999112 ) ) ;
#42156=CARTESIAN_POINT ( 'NONE',  ( -2.499999999999996447, -53.83333333333332860, 4.330127018922195425 ) ) ;
#42157=CARTESIAN_POINT ( 'NONE',  ( -8.190561711645485556E-16, -158.9375000013655779, 4.458734124999999437 ) ) ;
#42160=CARTESIAN_POINT ( 'NONE',  ( -4.458734124999999437, -79.39583333196773651, -2.574251347313719407 ) ) ;
#42161=CARTESIAN_POINT ( 'NONE',  ( 5.000000000000000000, -167.0000000000000000, 0.000000000000000000 ) ) ;
#42162=CARTESIAN_POINT ( 'NONE',  ( 4.458734124999998549, -89.72916666530106511, -2.574251347313721627 ) ) ;
#42164=CARTESIAN_POINT ( 'NONE',  ( 4.458734124999998549, -1.979166665301068662, -2.574251347313721627 ) ) ;
#42165=CARTESIAN_POINT ( 'NONE',  ( -2.229367062499996610, -38.39583333196773651, 3.861377020970582219 ) ) ;
#42166=CARTESIAN_POINT ( 'NONE',  ( 1.975475456537005874E-15, -16.62499999726881583, 5.000000000000000000 ) ) ;
#42169=ORIENTED_EDGE ( 'NONE', *, *, #7496, .T. ) ;
#42170=CARTESIAN_POINT ( 'NONE',  ( -5.000000000000000000, -148.6250000027312126, -6.123233995736766282E-16 ) ) ;
#42171=CARTESIAN_POINT ( 'NONE',  ( 0.000000000000000000, -170.0000000000000000, 5.000000000000000000 ) ) ;
#42172=CARTESIAN_POINT ( 'NONE',  ( 4.458734125000001214, -68.14583333196773651, 2.574251347313718519 ) ) ;
#42175=EDGE_LOOP ( 'NONE', ( #43320, #46211, #5405, #56668, #42781, #26911, #51901, #22510, #27321, #23039, #39864, #59335, #13051, #27910, #407, #50137, #60207, #49443, #62821, #62756, #16555, #23232, #28397, #56506, #53292, #32402, #58450, #42978, #50251, #46793, #18957, #15053, #50018, #21596, #14764, #44132, #9940, #48821, #35233, #41539, #40972, #1479, #45064, #42305, #47535, #15001, #50953, #14122, #51128, #55323, #41351, #1614, #53790, #27919, #9926, #28855, #20007, #44272, #35923, #56749, #45018, #62584, #57998, #60377, #21432, #58689, #17549, #33301, #22449, #6233, #6264, #26114, #6311, #48716, #30177, #52929, #30427, #44918, #12601, #44195, #62455, #52865, #43330, #61176, #50859, #33748, #40267, #33918, #32643, #27214, #40277, #48082, #6828, #21690, #21453, #3595, #48178, #62166, #39522, #2365, #6806, #51424, #27480, #28237, #289, #7671, #58930, #46444, #45779, #53468, #7534, #44262, #37119, #5586, #29276, #61433, #62446, #29810, #37093, #54577, #36880, #40013, #50986, #51202, #24891, #27139, #5943, #44492, #46522, #62101, #35817, #37809, #34638, #26158, #32104, #27172, #32660, #41108, #50772, #40208, #47857, #22648, #1515, #44668, #708, #49219, #19851, #63112, #45249, #15169, #28531, #16724, #7776, #53928, #13994, #26124, #10539, #2088, #58527, #19128, #36083, #57556, #39130, #63530, #61805, #63436, #17579, #27297, #21404, #20265, #9238, #36767, #48254, #52964, #13527, #18820, #58898, #48651, #60703, #40655, #33380, #26630, #42046, #18205, #56778, #53654, #49024, #41596, #56208, #4828, #16925, #41722, #49189, #63303, #58603, #40581, #15040, #7343, #44097, #29013, #40881, #11779, #11130, #49416, #24706, #37268, #54095, #48159, #3936, #12989, #48484, #60650, #54174, #38576, #20474, #17819, #59910, #18486, #49720, #35464, #23960, #35779, #39766, #49996, #34880, #52913, #9813, #36534, #52333, #27599, #17714, #5506, #53470, #15255, #37850, #15722, #46388, #3350, #36080, #17342, #28844, #55831, #45215, #4585 ) ) ;
#42176=CARTESIAN_POINT ( 'NONE',  ( 1.339745962155612702, -5.294658198738519950, -5.000000000000000000 ) ) ;
#42180=CARTESIAN_POINT ( 'NONE',  ( -2.229367062499996610, 2.854166668032259935, 3.861377020970582219 ) ) ;
#42181=VECTOR ( 'NONE', #9522, 1000.000000000000000 ) ;
#42183=CARTESIAN_POINT ( 'NONE',  ( 3.152801135295366208, -156.5625000013656063, 3.152801135295367985 ) ) ;
#42185=ORIENTED_EDGE ( 'NONE', *, *, #22536, .F. ) ;
#42187=DIRECTION ( 'NONE',  ( -0.000000000000000000, 1.000000000000000000, -0.000000000000000000 ) ) ;
#42191=CARTESIAN_POINT ( 'NONE',  ( 1.975475456537005874E-15, -67.74999999999998579, 5.000000000000000000 ) ) ;
#42193=FACE_OUTER_BOUND ( 'NONE', #58032, .T. ) ;
#42195=CARTESIAN_POINT ( 'NONE',  ( 1.062108568985190270E-13, -10.25000000000000355, -4.999999999999999112 ) ) ;
#42196=CARTESIAN_POINT ( 'NONE',  ( 4.458734125000000326, 21.10416666803226704, 2.574251347313718519 ) ) ;
#42198=CARTESIAN_POINT ( 'NONE',  ( -2.229367062500000163, -5.729166665301072214, -3.861377020970580443 ) ) ;
#42199=CARTESIAN_POINT ( 'NONE',  ( 1.975475456537005874E-15, -62.74999999999998579, 5.000000000000000000 ) ) ;
#42201=CARTESIAN_POINT ( 'NONE',  ( 5.000000000000000000, -140.1875000027311842, 2.071067811865478614 ) ) ;
#42208=CARTESIAN_POINT ( 'NONE',  ( -1.846868145590737420, -159.0000000013656063, 4.458734124999997661 ) ) ;
#42211=VERTEX_POINT ( 'NONE', #31392 ) ;
#42212=EDGE_CURVE ( 'NONE', #17071, #55117, #23260, .T. ) ;
#42213=CARTESIAN_POINT ( 'NONE',  ( 2.229367062499998831, 20.10416666803225993, -3.861377020970580887 ) ) ;
#42218=EDGE_CURVE ( 'NONE', #42312, #2707, #36404, .T. ) ;
#42219=CARTESIAN_POINT ( 'NONE',  ( -3.535250795749689387E-16, 5.749999999999998224, -5.773502691896257311 ) ) ;
#42221=CARTESIAN_POINT ( 'NONE',  ( 4.458734124999999437, -53.81249999863439371, -5.460374474430324690E-16 ) ) ;
#42222=CYLINDRICAL_SURFACE ( 'NONE', #43143, 5.000000000000000000 ) ;
#42224=EDGE_CURVE ( 'NONE', #12246, #44127, #55760, .T. ) ;
#42228=CARTESIAN_POINT ( 'NONE',  ( -2.499999999999996447, -24.70833333060214443, 4.330127018922195425 ) ) ;
#42229=CARTESIAN_POINT ( 'NONE',  ( -2.500000000000000444, -37.16666666666666430, -4.330127018922193649 ) ) ;
#42230=FACE_OUTER_BOUND ( 'NONE', #34893, .T. ) ;
#42233=CARTESIAN_POINT ( 'NONE',  ( -3.535533905932738641, -143.3750000000000000, 3.535533905932737309 ) ) ;
#42234=CARTESIAN_POINT ( 'NONE',  ( -3.152548672688508926E-16, -62.56249999863440792, -5.148502694627439702 ) ) ;
#42235=CARTESIAN_POINT ( 'NONE',  ( 3.152801135295367541, -147.5625000013655779, -3.152801135295367541 ) ) ;
#42236=VECTOR ( 'NONE', #18216, 1000.000000000000000 ) ;
#42237=CARTESIAN_POINT ( 'NONE',  ( 4.458734125000001214, -69.89583333196773651, 2.574251347313718519 ) ) ;
#42239=CARTESIAN_POINT ( 'NONE',  ( -2.229367062500000163, -17.72916666530106866, -3.861377020970580443 ) ) ;
#42241=CARTESIAN_POINT ( 'NONE',  ( 2.499999999999998668, -60.20833333060214443, -4.330127018922193649 ) ) ;
#42243=CARTESIAN_POINT ( 'NONE',  ( -5.000000000000000888, -150.4375000000000000, 2.071067811865474617 ) ) ;
#42244=ORIENTED_EDGE ( 'NONE', *, *, #7588, .T. ) ;
#42246=DIRECTION ( 'NONE',  ( -0.000000000000000000, 1.000000000000000000, -0.000000000000000000 ) ) ;
#42247=DIRECTION ( 'NONE',  ( -0.000000000000000000, 1.000000000000000000, -0.000000000000000000 ) ) ;
#42252=CARTESIAN_POINT ( 'NONE',  ( -4.458734124999999437, -53.64583333196772941, -2.574251347313719407 ) ) ;
#42253=ORIENTED_EDGE ( 'NONE', *, *, #46518, .T. ) ;
#42256=CARTESIAN_POINT ( 'NONE',  ( 9.457646018065525792E-16, 19.93750000136559208, 5.148502694627439702 ) ) ;
#42258=CARTESIAN_POINT ( 'NONE',  ( 1.339745962155661996, -13.16965819600733489, -4.999999999999970690 ) ) ;
#42265=CARTESIAN_POINT ( 'NONE',  ( 3.535533905932736864, -140.2500000027311842, 3.535533905932738641 ) ) ;
#42269=CARTESIAN_POINT ( 'NONE',  ( 3.061616997868383141E-16, -162.7500000000000000, -5.000000000000000000 ) ) ;
#42271=CYLINDRICAL_SURFACE ( 'NONE', #41912, 5.000000000000000000 ) ;
#42274=VERTEX_POINT ( 'NONE', #3103 ) ;
#42275=CARTESIAN_POINT ( 'NONE',  ( -1.339745962155613812, -5.080341798530291442, -5.000000000000000000 ) ) ;
#42277=CARTESIAN_POINT ( 'NONE',  ( 5.000000000000000888, -153.0625000027311842, -2.071067811865475505 ) ) ;
#42284=CARTESIAN_POINT ( 'NONE',  ( 5.000000000000000000, -148.0625000000000284, 2.071067811865478614 ) ) ;
#42287=CARTESIAN_POINT ( 'NONE',  ( 1.846868145590735200, -169.5000000013655495, -4.458734124999999437 ) ) ;
#42288=CARTESIAN_POINT ( 'NONE',  ( 9.457646018065525792E-16, -26.06249999863440792, 5.148502694627439702 ) ) ;
#42289=CARTESIAN_POINT ( 'NONE',  ( 1.975475456537005874E-15, -25.62499999726881228, 5.000000000000000000 ) ) ;
#42291=CARTESIAN_POINT ( 'NONE',  ( 3.152801135295366208, -149.5625000013655779, 3.152801135295367985 ) ) ;
#42294=CARTESIAN_POINT ( 'NONE',  ( -2.229367062499996610, -51.39583333196773651, 3.861377020970582219 ) ) ;
#42296=CARTESIAN_POINT ( 'NONE',  ( -1.049326080737009628E-13, -2.750000000000003109, 5.000000000000000000 ) ) ;
#42298=CARTESIAN_POINT ( 'NONE',  ( 2.499999999999998668, 25.66666666666666430, -4.330127018922193649 ) ) ;
#42300=CARTESIAN_POINT ( 'NONE',  ( -4.458734124999999437, -3.312499998634407916, 0.000000000000000000 ) ) ;
#42301=CARTESIAN_POINT ( 'NONE',  ( -4.999999999999998224, -10.91666666666666607, 2.886751345948131764 ) ) ;
#42302=CARTESIAN_POINT ( 'NONE',  ( 3.061616997868383141E-16, -164.7500000000000000, -5.000000000000000000 ) ) ;
#42303=CARTESIAN_POINT ( 'NONE',  ( 6.123233995736766282E-16, -170.0000000000000000, -5.000000000000000000 ) ) ;
#42304=CARTESIAN_POINT ( 'NONE',  ( -4.458734124999998549, 7.520833334698926009, 2.574251347313722516 ) ) ;
#42305=ORIENTED_EDGE ( 'NONE', *, *, #37842, .T. ) ;
#42309=CARTESIAN_POINT ( 'NONE',  ( 4.458734124999999437, -48.81249999863440792, -5.460374474430324690E-16 ) ) ;
#42310=CARTESIAN_POINT ( 'NONE',  ( 4.458734124999999437, -158.6875000013655779, 0.000000000000000000 ) ) ;
#42311=CARTESIAN_POINT ( 'NONE',  ( 5.000000000000000000, -45.37499999726880873, -6.123233995736766282E-16 ) ) ;
#42312=VERTEX_POINT ( 'NONE', #42634 ) ;
#42313=CARTESIAN_POINT ( 'NONE',  ( -4.458734124999998549, -25.22916666530106866, 2.574251347313722516 ) ) ;
#42315=CARTESIAN_POINT ( 'NONE',  ( 2.071067811865472841, -169.8124999999999716, -5.000000000000002665 ) ) ;
#42316=CARTESIAN_POINT ( 'NONE',  ( 4.458734124999999437, -164.4375000013655779, 0.000000000000000000 ) ) ;
#42319=ADVANCED_FACE ( 'NONE', ( #47773 ), #27527, .T. ) ;
#42320=CARTESIAN_POINT ( 'NONE',  ( 2.229367062500001939, -40.22916666530107221, 3.861377020970579999 ) ) ;
#42325=LINE ( 'NONE', #43573, #26636 ) ;
#42329=CARTESIAN_POINT ( 'NONE',  ( -2.229367062500000163, -84.72916666530107932, -3.861377020970580443 ) ) ;
#42331=CARTESIAN_POINT ( 'NONE',  ( 5.000000000000000000, 22.50000000000000000, -6.123233995736766282E-16 ) ) ;
#42332=CARTESIAN_POINT ( 'NONE',  ( -1.339745962155610925, -6.794658198738519062, 5.000000000000000000 ) ) ;
#42334=CARTESIAN_POINT ( 'NONE',  ( -6.972266317189433020E-16, -52.12499999726880873, -5.000000000000000000 ) ) ;
#42339=CARTESIAN_POINT ( 'NONE',  ( 5.000000000000000000, -154.1250000027312126, 0.000000000000000000 ) ) ;
#42342=CARTESIAN_POINT ( 'NONE',  ( -5.000000000000000888, -153.5625000027312126, 2.071067811865474617 ) ) ;
#42345=CARTESIAN_POINT ( 'NONE',  ( 9.457646018065525792E-16, -83.31249999863440792, 5.148502694627439702 ) ) ;
#42348=VERTEX_POINT ( 'NONE', #62593 ) ;
#42349=CARTESIAN_POINT ( 'NONE',  ( 1.975475456537005874E-15, -86.62499999726880162, 5.000000000000000000 ) ) ;
#42351=CARTESIAN_POINT ( 'NONE',  ( 5.000000000000000000, -165.1875000027312126, 2.071067811865478614 ) ) ;
#42353=CARTESIAN_POINT ( 'NONE',  ( 2.229367062500001939, 13.77083333469892779, 3.861377020970579999 ) ) ;
#42360=CARTESIAN_POINT ( 'NONE',  ( -1.339745962155613812, -22.08034179853029855, -5.000000000000000000 ) ) ;
#42361=CARTESIAN_POINT ( 'NONE',  ( 2.229367062500001939, -6.979166665301073103, 3.861377020970579999 ) ) ;
#42364=CARTESIAN_POINT ( 'NONE',  ( -2.229367062499996610, -36.39583333196773651, 3.861377020970582219 ) ) ;
#42366=CARTESIAN_POINT ( 'NONE',  ( 1.339745962155615144, 0.4196582014697064489, 4.999999999999999112 ) ) ;
#42369=CARTESIAN_POINT ( 'NONE',  ( 4.458734125000001214, 17.10416666803225993, 2.574251347313718519 ) ) ;
#42371=CARTESIAN_POINT ( 'NONE',  ( 2.499999999999998668, -55.33333333333332860, -4.330127018922193649 ) ) ;
#42372=CARTESIAN_POINT ( 'NONE',  ( -2.229367062500000163, -83.72916666530106511, -3.861377020970580443 ) ) ;
#42375=CARTESIAN_POINT ( 'NONE',  ( -5.000000000000000000, 17.04166666939785202, -2.886751345948128211 ) ) ;
#42377=CARTESIAN_POINT ( 'NONE',  ( -6.972266317189433020E-16, -66.24999999999998579, -5.000000000000000000 ) ) ;
#42380=CARTESIAN_POINT ( 'NONE',  ( -5.000000000000000000, -28.08333333333333925, -2.886751345948128211 ) ) ;
#42381=CARTESIAN_POINT ( 'NONE',  ( 4.458734124999998549, -30.72916666530107221, -2.574251347313721627 ) ) ;
#42382=CARTESIAN_POINT ( 'NONE',  ( 1.975475456537005874E-15, -33.75000000000000000, 5.000000000000000000 ) ) ;
#42383=CARTESIAN_POINT ( 'NONE',  ( -2.499999999999996447, -29.70833333060215153, 4.330127018922195425 ) ) ;
#42384=CARTESIAN_POINT ( 'NONE',  ( -4.458734124999999437, -61.39583333196774362, -2.574251347313719407 ) ) ;
#42387=CARTESIAN_POINT ( 'NONE',  ( 2.229367062500001939, -11.22916666530107044, 3.861377020970579999 ) ) ;
#42388=EDGE_LOOP ( 'NONE', ( #43558, #58086, #60205, #60682 ) ) ;
#42389=CARTESIAN_POINT ( 'NONE',  ( 2.500000000000002220, -78.66666666666665719, 4.330127018922192761 ) ) ;
#42392=CARTESIAN_POINT ( 'NONE',  ( 5.000000000000000888, -79.45833333060214443, 2.886751345948126879 ) ) ;
#42393=CARTESIAN_POINT ( 'NONE',  ( -4.764381983412779477E-15, 26.37500000273118417, 5.000000000000000000 ) ) ;
#42397=CARTESIAN_POINT ( 'NONE',  ( 9.457646018065525792E-16, -21.31249999863440081, 5.148502694627439702 ) ) ;
#42398=CARTESIAN_POINT ( 'NONE',  ( 4.458734125000001214, -59.14583333196773651, 2.574251347313718519 ) ) ;
#42399=ORIENTED_EDGE ( 'NONE', *, *, #11487, .F. ) ;
#42400=CARTESIAN_POINT ( 'NONE',  ( -8.190561711645485556E-16, -168.9375000013656063, 4.458734124999999437 ) ) ;
#42405=DIRECTION ( 'NONE',  ( 0.000000000000000000, 0.000000000000000000, 1.000000000000000000 ) ) ;
#42409=CARTESIAN_POINT ( 'NONE',  ( -4.458734125000000326, -149.2500000013655779, -1.846868145590735644 ) ) ;
#42414=CARTESIAN_POINT ( 'NONE',  ( -4.458734124999999437, -63.64583333196773651, -2.574251347313719407 ) ) ;
#42415=CARTESIAN_POINT ( 'NONE',  ( 2.499999999999998668, -43.33333333333333570, -4.330127018922193649 ) ) ;
#42417=CARTESIAN_POINT ( 'NONE',  ( -4.458734125000000326, -144.8750000013656063, 1.846868145590734089 ) ) ;
#42419=VERTEX_POINT ( 'NONE', #13683 ) ;
#42420=CARTESIAN_POINT ( 'NONE',  ( -6.972266317189433020E-16, -49.12499999726880162, -5.000000000000000000 ) ) ;
#42426=CARTESIAN_POINT ( 'NONE',  ( -6.972266317189433020E-16, -72.25000000000000000, -5.000000000000000000 ) ) ;
#42427=CARTESIAN_POINT ( 'NONE',  ( -5.000000000000000000, -17.87499999726881583, 0.000000000000000000 ) ) ;
#42433=CARTESIAN_POINT ( 'NONE',  ( -2.229367062499996610, 5.854166668032262599, 3.861377020970582219 ) ) ;
#42435=CARTESIAN_POINT ( 'NONE',  ( -4.458734124999999437, -21.56249999863440436, 0.000000000000000000 ) ) ;
#42437=CARTESIAN_POINT ( 'NONE',  ( 3.152801135295367541, -159.3125000013656063, -3.152801135295367541 ) ) ;
#42438=CARTESIAN_POINT ( 'NONE',  ( 1.975475456537005874E-15, -36.62499999726880873, 5.000000000000000000 ) ) ;
#42441=CYLINDRICAL_SURFACE ( 'NONE', #57365, 5.000000000000000000 ) ;
#42442=CARTESIAN_POINT ( 'NONE',  ( -4.458734124999997661, -41.22916666530107932, 2.574251347313722516 ) ) ;
#42443=ADVANCED_FACE ( 'NONE', ( #12735 ), #32993, .T. ) ;
#42445=CARTESIAN_POINT ( 'NONE',  ( -4.458734124999999437, -65.64583333196773651, -2.574251347313719407 ) ) ;
#42447=CARTESIAN_POINT ( 'NONE',  ( -1.339745962155613812, -41.20534180126147561, -5.000000000000000000 ) ) ;
#42448=CARTESIAN_POINT ( 'NONE',  ( 2.500000000000002220, -68.54166666393547303, 4.330127018922192761 ) ) ;
#42449=EDGE_LOOP ( 'NONE', ( #49579, #301, #31483, #13962 ) ) ;
#42450=CARTESIAN_POINT ( 'NONE',  ( 1.975475456537005874E-15, -84.74999999999998579, 5.000000000000000000 ) ) ;
#42452=CARTESIAN_POINT ( 'NONE',  ( 2.499999999999998668, -11.33333333333333393, -4.330127018922193649 ) ) ;
#42453=CARTESIAN_POINT ( 'NONE',  ( -4.458734124999998549, -17.22916666530106866, 2.574251347313722516 ) ) ;
#42454=CARTESIAN_POINT ( 'NONE',  ( 4.458734124999998549, -78.72916666530106511, -2.574251347313721627 ) ) ;
#42456=CARTESIAN_POINT ( 'NONE',  ( 5.000000000000000000, -13.37499999726881050, -6.123233995736766282E-16 ) ) ;
#42457=CARTESIAN_POINT ( 'NONE',  ( -4.458734124999998549, -42.22916666530107932, 2.574251347313722516 ) ) ;
#42458=ORIENTED_EDGE ( 'NONE', *, *, #41607, .F. ) ;
#42460=CARTESIAN_POINT ( 'NONE',  ( -3.152548672688508926E-16, 9.187500001365593860, -5.148502694627439702 ) ) ;
#42461=EDGE_LOOP ( 'NONE', ( #17866, #60293, #28291, #53323 ) ) ;
#42462=( BOUNDED_CURVE ( )  B_SPLINE_CURVE ( 2, ( #26005, #61698, #1898, #22459, #45935, #21506, #26639, #46580, #12477 ),
 .UNSPECIFIED., .F., .F. ) 
 B_SPLINE_CURVE_WITH_KNOTS ( ( 3, 2, 2, 2, 3 ),
 ( 0.6062499999999999556, 0.6069444444444443976, 0.6083333333333332815, 0.6097222222222222765, 0.6104166666666667185 ),
 .UNSPECIFIED. ) 
 CURVE ( )  GEOMETRIC_REPRESENTATION_ITEM ( )  RATIONAL_B_SPLINE_CURVE ( ( 0.9330127018922194093, 0.9330127018922194093, 1.000000000000000000, 0.8660254037844387076, 1.000000000000000000, 0.8660254037844387076, 1.000000000000000000, 0.9330127018922194093, 0.9330127018922194093 ) ) 
 REPRESENTATION_ITEM ( '' )  );
#42464=CARTESIAN_POINT ( 'NONE',  ( 5.000000000000000888, -55.58333333333333570, 2.886751345948126879 ) ) ;
#42465=CARTESIAN_POINT ( 'NONE',  ( -3.152801135295367096, -158.3125000013656063, -3.152801135295367541 ) ) ;
#42468=CARTESIAN_POINT ( 'NONE',  ( -3.152548672688508926E-16, -82.56249999863442213, -5.148502694627439702 ) ) ;
#42469=CARTESIAN_POINT ( 'NONE',  ( 3.535533905932736864, -165.1250000000000284, 3.535533905932738641 ) ) ;
#42473=CARTESIAN_POINT ( 'NONE',  ( -2.229367062499996610, -8.395833331967736513, 3.861377020970582219 ) ) ;
#42474=CARTESIAN_POINT ( 'NONE',  ( -4.458734124999998549, -43.47916666530106511, 2.574251347313722516 ) ) ;
#42475=VECTOR ( 'NONE', #41528, 1000.000000000000000 ) ;
#42476=EDGE_CURVE ( 'NONE', #47715, #7044, #27760, .T. ) ;
#42478=CARTESIAN_POINT ( 'NONE',  ( 2.071067811865645591, -151.3125000027311842, 4.999999999999830358 ) ) ;
#42480=FACE_OUTER_BOUND ( 'NONE', #62426, .T. ) ;
#42481=ORIENTED_EDGE ( 'NONE', *, *, #8230, .F. ) ;
#42484=CARTESIAN_POINT ( 'NONE',  ( 9.457646018065525792E-16, -71.31249999863439371, 5.148502694627439702 ) ) ;
#42485=CARTESIAN_POINT ( 'NONE',  ( -4.458734124999999437, -146.2500000013656347, -1.846868145590735644 ) ) ;
#42488=LINE ( 'NONE', #47013, #63593 ) ;
#42491=EDGE_CURVE ( 'NONE', #5270, #36444, #29723, .T. ) ;
#42492=CARTESIAN_POINT ( 'NONE',  ( -2.500000000000000444, 2.833333333333333481, -4.330127018922193649 ) ) ;
#42493=CARTESIAN_POINT ( 'NONE',  ( -3.152548672688508926E-16, 3.437500001365594748, -5.148502694627439702 ) ) ;
#42495=CARTESIAN_POINT ( 'NONE',  ( 3.152801135295367541, -155.3125000013656063, -3.152801135295367541 ) ) ;
#42504=CARTESIAN_POINT ( 'NONE',  ( 5.000000000000000000, -67.41666666666667140, -2.886751345948130876 ) ) ;
#42506=FACE_OUTER_BOUND ( 'NONE', #7367, .T. ) ;
#42509=CARTESIAN_POINT ( 'NONE',  ( -4.458734124999997661, 23.77083333469892423, 2.574251347313722516 ) ) ;
#42511=CARTESIAN_POINT ( 'NONE',  ( 9.457646018065525792E-16, -4.312499998634408804, 5.148502694627439702 ) ) ;
#42513=DIRECTION ( 'NONE',  ( -0.000000000000000000, 1.000000000000000000, -0.000000000000000000 ) ) ;
#42515=CARTESIAN_POINT ( 'NONE',  ( -3.535533905932738641, -140.5000000027311842, 3.535533905932737309 ) ) ;
#42521=DIRECTION ( 'NONE',  ( -0.000000000000000000, 1.000000000000000000, -0.000000000000000000 ) ) ;
#42524=CARTESIAN_POINT ( 'NONE',  ( -3.152801135295367985, -157.0625000013656063, 3.152801135295367096 ) ) ;
#42528=CARTESIAN_POINT ( 'NONE',  ( 4.458734125000001214, 19.85416666803226349, 2.574251347313718519 ) ) ;
#42534=CARTESIAN_POINT ( 'NONE',  ( -4.999999999999999112, 3.083333333333333925, 2.886751345948131764 ) ) ;
#42535=CARTESIAN_POINT ( 'NONE',  ( 2.229367062499998831, -62.64583333196774362, -3.861377020970580887 ) ) ;
#42536=CARTESIAN_POINT ( 'NONE',  ( 4.729367062499999719, -139.2812500020483810, 0.000000000000000000 ) ) ;
#42538=CARTESIAN_POINT ( 'NONE',  ( 9.457646018065525792E-16, -26.06249999863440792, 5.148502694627439702 ) ) ;
#42540=CARTESIAN_POINT ( 'NONE',  ( -1.339745962155614034, 26.33034180399265978, 4.999999999999999112 ) ) ;
#42542=CARTESIAN_POINT ( 'NONE',  ( 1.060575238724906964E-15, -37.75000000000000000, 5.773502691896257311 ) ) ;
#42543=FACE_OUTER_BOUND ( 'NONE', #38739, .T. ) ;
#42547=CARTESIAN_POINT ( 'NONE',  ( 4.458734124999999437, -64.81249999863440792, -5.460374474430324690E-16 ) ) ;
#42548=CARTESIAN_POINT ( 'NONE',  ( 3.152801135295367541, -149.5625000013655779, -3.152801135295367541 ) ) ;
#42549=CARTESIAN_POINT ( 'NONE',  ( -4.458734124999999437, -78.39583333196772230, -2.574251347313719407 ) ) ;
#42551=CARTESIAN_POINT ( 'NONE',  ( -4.458734124999998549, -26.47916666530107221, 2.574251347313722516 ) ) ;
#42552=CARTESIAN_POINT ( 'NONE',  ( 5.000000000000000000, -67.29166666393547303, -2.886751345948129988 ) ) ;
#42554=ORIENTED_EDGE ( 'NONE', *, *, #25509, .F. ) ;
#42558=CARTESIAN_POINT ( 'NONE',  ( 5.000000000000000000, -149.1250000027312126, 0.000000000000000000 ) ) ;
#42560=ORIENTED_EDGE ( 'NONE', *, *, #11395, .F. ) ;
#42562=CARTESIAN_POINT ( 'NONE',  ( 5.000000000000000888, -8.583333333333332149, 2.886751345948126879 ) ) ;
#42563=CARTESIAN_POINT ( 'NONE',  ( -2.229367062500000163, -51.72916666530107221, -3.861377020970580443 ) ) ;
#42564=EDGE_CURVE ( 'NONE', #23493, #15636, #62713, .T. ) ;
#42566=VECTOR ( 'NONE', #53469, 1000.000000000000000 ) ;
#42570=CARTESIAN_POINT ( 'NONE',  ( 2.229367062500001939, 17.02083333469892779, 3.861377020970579999 ) ) ;
#42573=CARTESIAN_POINT ( 'NONE',  ( -1.846868145590734756, -168.1250000013656063, -4.458734124999999437 ) ) ;
#42574=ORIENTED_EDGE ( 'NONE', *, *, #6431, .T. ) ;
#42580=DIRECTION ( 'NONE',  ( 0.000000000000000000, 0.000000000000000000, 1.000000000000000000 ) ) ;
#42584=CARTESIAN_POINT ( 'NONE',  ( 1.339745962155615144, -45.70534180126146850, 4.999999999999999112 ) ) ;
#42587=CARTESIAN_POINT ( 'NONE',  ( -3.535533905932738641, -159.3750000000000284, 3.535533905932737309 ) ) ;
#42593=CARTESIAN_POINT ( 'NONE',  ( -3.535533905932738641, -152.5000000027312126, 3.535533905932737309 ) ) ;
#42600=CARTESIAN_POINT ( 'NONE',  ( 3.535533905932738197, -148.8750000000000000, -3.535533905932738197 ) ) ;
#42603=CARTESIAN_POINT ( 'NONE',  ( 2.730187237215162345E-16, -168.4375000013656063, -4.458734124999999437 ) ) ;
#42604=CARTESIAN_POINT ( 'NONE',  ( -2.229367062499996610, -27.14583333196774007, 3.861377020970582219 ) ) ;
#42605=DIRECTION ( 'NONE',  ( -0.000000000000000000, 1.000000000000000000, -0.000000000000000000 ) ) ;
#42608=CARTESIAN_POINT ( 'NONE',  ( 4.458734124999999437, -147.5000000013656063, 1.846868145590737864 ) ) ;
#42609=ORIENTED_EDGE ( 'NONE', *, *, #55776, .T. ) ;
#42611=CARTESIAN_POINT ( 'NONE',  ( 4.458734125000000326, -58.14583333196773651, 2.574251347313718519 ) ) ;
#42614=CARTESIAN_POINT ( 'NONE',  ( 5.000000000000000000, 23.50000000000000000, -6.123233995736766282E-16 ) ) ;
#42616=CARTESIAN_POINT ( 'NONE',  ( -2.229367062500000163, -0.4791666653010707710, -3.861377020970580443 ) ) ;
#42617=( BOUNDED_CURVE ( )  B_SPLINE_CURVE ( 2, ( #16885, #3058, #26537, #26863, #2736, #56775, #17835, #42275, #60647 ),
 .UNSPECIFIED., .F., .F. ) 
 B_SPLINE_CURVE_WITH_KNOTS ( ( 3, 2, 2, 2, 3 ),
 ( 0.2812500000000000000, 0.2819444444444444420, 0.2833333333333333259, 0.2847222222222222099, 0.2854166666666666519 ),
 .UNSPECIFIED. ) 
 CURVE ( )  GEOMETRIC_REPRESENTATION_ITEM ( )  RATIONAL_B_SPLINE_CURVE ( ( 0.9330127018922194093, 0.9330127018922194093, 1.000000000000000000, 0.8660254037844387076, 1.000000000000000000, 0.8660254037844387076, 1.000000000000000000, 0.9330127018922194093, 0.9330127018922194093 ) ) 
 REPRESENTATION_ITEM ( '' )  );
#42618=CARTESIAN_POINT ( 'NONE',  ( -1.339745962155613812, -11.20534180126147916, -5.000000000000000000 ) ) ;
#42620=CARTESIAN_POINT ( 'NONE',  ( -3.152548672688508926E-16, 10.18750000136559564, -5.148502694627439702 ) ) ;
#42622=CARTESIAN_POINT ( 'NONE',  ( 1.975475456537005874E-15, -65.74999999999998579, 5.000000000000000000 ) ) ;
#42624=CARTESIAN_POINT ( 'NONE',  ( 2.071067811865459962, -167.9375000027312126, -5.000000000000015987 ) ) ;
#42625=CARTESIAN_POINT ( 'NONE',  ( -2.229367062499996610, -47.14583333196774362, 3.861377020970582219 ) ) ;
#42626=CARTESIAN_POINT ( 'NONE',  ( 3.152801135295367541, -160.5625000013656063, -3.152801135295367541 ) ) ;
#42627=CARTESIAN_POINT ( 'NONE',  ( -4.999999999999999112, -44.79166666393547303, 2.886751345948131764 ) ) ;
#42629=CARTESIAN_POINT ( 'NONE',  ( 4.458734125000001214, -21.89583333196773296, 2.574251347313718519 ) ) ;
#42633=CARTESIAN_POINT ( 'NONE',  ( -1.846868145590737420, -159.7500000013656063, 4.458734124999999437 ) ) ;
#42634=CARTESIAN_POINT ( 'NONE',  ( -6.972266317189433020E-16, -20.12499999726881228, -5.000000000000000000 ) ) ;
#42636=CARTESIAN_POINT ( 'NONE',  ( 2.229367062499998831, -37.89583333196773651, -3.861377020970580887 ) ) ;
#42645=CARTESIAN_POINT ( 'NONE',  ( 2.229367062499998831, -84.89583333196773651, -3.861377020970580887 ) ) ;
#42648=CARTESIAN_POINT ( 'NONE',  ( 5.000000000000000000, -9.416666666666662522, -2.886751345948130876 ) ) ;
#42649=CARTESIAN_POINT ( 'NONE',  ( 1.975475456537005874E-15, -44.62499999726880162, 5.000000000000000000 ) ) ;
#42658=LINE ( 'NONE', #4065, #46895 ) ;
#42660=CARTESIAN_POINT ( 'NONE',  ( -3.152548672688508926E-16, -82.81249999863442213, -5.148502694627439702 ) ) ;
#42664=EDGE_LOOP ( 'NONE', ( #15963, #36488, #8548, #44759 ) ) ;
#42666=CARTESIAN_POINT ( 'NONE',  ( 5.000000000000000888, -167.0625000027311842, -2.071067811865475505 ) ) ;
#42668=CARTESIAN_POINT ( 'NONE',  ( -2.500000000000000444, -16.16666666666666785, -4.330127018922193649 ) ) ;
#42673=CARTESIAN_POINT ( 'NONE',  ( -5.000000000000000000, -19.99999999999999645, 0.000000000000000000 ) ) ;
#42674=CARTESIAN_POINT ( 'NONE',  ( 2.500000000000002220, 17.33333333333333215, 4.330127018922192761 ) ) ;
#42675=CARTESIAN_POINT ( 'NONE',  ( 9.457646018065525792E-16, -10.06249999863440614, 5.148502694627439702 ) ) ;
#42676=VERTEX_POINT ( 'NONE', #58379 ) ;
#42677=CARTESIAN_POINT ( 'NONE',  ( -2.229367062500000163, -37.72916666530107221, -3.861377020970580443 ) ) ;
#42680=CARTESIAN_POINT ( 'NONE',  ( -6.972266317189433020E-16, 9.750000000000000000, -5.000000000000000000 ) ) ;
#42683=CARTESIAN_POINT ( 'NONE',  ( -2.229367062499996610, 16.85416666803225993, 3.861377020970582219 ) ) ;
#42685=FACE_OUTER_BOUND ( 'NONE', #49383, .T. ) ;
#42686=CARTESIAN_POINT ( 'NONE',  ( 4.458734124999998549, -81.97916666530106511, -2.574251347313721627 ) ) ;
#42688=CARTESIAN_POINT ( 'NONE',  ( 2.500000000000002220, 11.45833333606451809, 4.330127018922192761 ) ) ;
#42689=EDGE_LOOP ( 'NONE', ( #50642, #58545, #48780, #24429 ) ) ;
#42690=CARTESIAN_POINT ( 'NONE',  ( 1.339745962155615144, -25.70534180126147916, 4.999999999999999112 ) ) ;
#42694=CARTESIAN_POINT ( 'NONE',  ( 5.000000000000000000, -31.41666666666667140, -2.886751345948129988 ) ) ;
#42695=CARTESIAN_POINT ( 'NONE',  ( -4.458734124999999437, -31.39583333196773296, -2.574251347313719407 ) ) ;
#42696=DIRECTION ( 'NONE',  ( -0.000000000000000000, 1.000000000000000000, -0.000000000000000000 ) ) ;
#42697=CARTESIAN_POINT ( 'NONE',  ( -2.499999999999996447, -26.70833333060214798, 4.330127018922195425 ) ) ;
#42698=CARTESIAN_POINT ( 'NONE',  ( 4.458734125000001214, -59.89583333196774362, 2.574251347313718519 ) ) ;
#42700=CARTESIAN_POINT ( 'NONE',  ( 1.339745962155612702, -62.16965819600734022, -5.000000000000000000 ) ) ;
#42701=CARTESIAN_POINT ( 'NONE',  ( 4.458734124999999437, -7.062499998634404363, -5.460374474430324690E-16 ) ) ;
#42702=ORIENTED_EDGE ( 'NONE', *, *, #17376, .F. ) ;
#42703=CARTESIAN_POINT ( 'NONE',  ( -4.999999999999999112, -74.91666666666665719, 2.886751345948131764 ) ) ;
#42704=CARTESIAN_POINT ( 'NONE',  ( 1.339745962155613146, 28.83034180399266688, -4.999999999999999112 ) ) ;
#42707=CARTESIAN_POINT ( 'NONE',  ( 5.000000000000000000, -78.37499999726881583, -6.123233995736766282E-16 ) ) ;
#42708=CARTESIAN_POINT ( 'NONE',  ( -6.972266317189433020E-16, -65.12499999726880162, -5.000000000000000000 ) ) ;
#42711=CARTESIAN_POINT ( 'NONE',  ( 4.458734125000001214, -21.14583333196774362, 2.574251347313718519 ) ) ;
#42712=CARTESIAN_POINT ( 'NONE',  ( -4.458734124999999437, -59.56249999863440081, 0.000000000000000000 ) ) ;
#42715=CARTESIAN_POINT ( 'NONE',  ( -1.846868145590734756, -169.3750000013656347, -4.458734125000000326 ) ) ;
#42717=CARTESIAN_POINT ( 'NONE',  ( -3.535533905932737309, -167.7500000027312126, -3.535533905932738197 ) ) ;
#42718=VERTEX_POINT ( 'NONE', #48401 ) ;
#42721=DIRECTION ( 'NONE',  ( -0.000000000000000000, 1.000000000000000000, -0.000000000000000000 ) ) ;
#42724=CARTESIAN_POINT ( 'NONE',  ( 3.152801135295367541, -143.5625000013655779, -3.152801135295367541 ) ) ;
#42726=CARTESIAN_POINT ( 'NONE',  ( -9.184850993605147944E-16, -163.3750000027311842, 5.000000000000000000 ) ) ;
#42728=CARTESIAN_POINT ( 'NONE',  ( 2.229367062500001939, -70.22916666530107932, 3.861377020970579999 ) ) ;
#42731=CARTESIAN_POINT ( 'NONE',  ( -1.846868145590734756, -141.1250000013656063, -4.458734124999999437 ) ) ;
#42734=AXIS2_PLACEMENT_3D ( 'NONE', #6953, #51962, #17556 ) ;
#42736=CARTESIAN_POINT ( 'NONE',  ( -5.000000000000000888, -144.4375000000000000, 2.071067811865474617 ) ) ;
#42741=VECTOR ( 'NONE', #7092, 1000.000000000000000 ) ;
#42742=CARTESIAN_POINT ( 'NONE',  ( 4.458734124999999437, 22.93750000136559564, -5.460374474430324690E-16 ) ) ;
#42743=CARTESIAN_POINT ( 'NONE',  ( 1.975475456537005874E-15, -34.75000000000000000, 5.000000000000000000 ) ) ;
#42750=CARTESIAN_POINT ( 'NONE',  ( 4.458734124999999437, 9.187500001365592084, -5.460374474430324690E-16 ) ) ;
#42752=CARTESIAN_POINT ( 'NONE',  ( 4.458734124999998549, -21.97916666530107221, -2.574251347313721627 ) ) ;
#42754=CARTESIAN_POINT ( 'NONE',  ( 4.458734125000000326, -161.3750000013656063, -1.846868145590734978 ) ) ;
#42755=CARTESIAN_POINT ( 'NONE',  ( 2.499999999999998668, 15.79166666939785202, -4.330127018922193649 ) ) ;
#42759=CARTESIAN_POINT ( 'NONE',  ( 4.458734124999998549, 29.27083333469892423, -2.574251347313721627 ) ) ;
#42760=CARTESIAN_POINT ( 'NONE',  ( -4.458734124999999437, -41.31249999863440081, 0.000000000000000000 ) ) ;
#42761=DIRECTION ( 'NONE',  ( -0.000000000000000000, 1.000000000000000000, -0.000000000000000000 ) ) ;
#42763=CARTESIAN_POINT ( 'NONE',  ( 4.458734125000000326, -67.14583333196773651, 2.574251347313718519 ) ) ;
#42765=CARTESIAN_POINT ( 'NONE',  ( 2.500000000000002220, -57.54166666393548013, 4.330127018922192761 ) ) ;
#42770=CARTESIAN_POINT ( 'NONE',  ( -5.000000000000000000, -14.08333333333333037, -2.886751345948128211 ) ) ;
#42771=CARTESIAN_POINT ( 'NONE',  ( -2.229367062499996610, -18.14583333196773651, 3.861377020970582219 ) ) ;
#42772=CARTESIAN_POINT ( 'NONE',  ( 2.229367062500001939, -74.97916666530106511, 3.861377020970579999 ) ) ;
#42774=EDGE_CURVE ( 'NONE', #28458, #55065, #24935, .T. ) ;
#42775=CARTESIAN_POINT ( 'NONE',  ( -5.000000000000000000, -11.87499999726881761, 0.000000000000000000 ) ) ;
#42776=CARTESIAN_POINT ( 'NONE',  ( -2.229367062499996610, -45.14583333196774362, 3.861377020970582219 ) ) ;
#42778=CARTESIAN_POINT ( 'NONE',  ( 5.000000000000000888, -41.58333333333333570, 2.886751345948126879 ) ) ;
#42779=ADVANCED_FACE ( 'NONE', ( #19123 ), #59983, .T. ) ;
#42780=CARTESIAN_POINT ( 'NONE',  ( 9.457646018065525792E-16, 7.687500001365596525, 5.148502694627439702 ) ) ;
#42781=ORIENTED_EDGE ( 'NONE', *, *, #14917, .T. ) ;
#42782=CARTESIAN_POINT ( 'NONE',  ( 6.123233995736766282E-16, -170.0000000000000000, -5.000000000000000000 ) ) ;
#42783=CARTESIAN_POINT ( 'NONE',  ( 2.500000000000002220, -63.66666666666666430, 4.330127018922192761 ) ) ;
#42784=CARTESIAN_POINT ( 'NONE',  ( 4.458734124999999437, -158.6875000013655779, 0.000000000000000000 ) ) ;
#42788=CARTESIAN_POINT ( 'NONE',  ( 5.000000000000000000, -165.0000000000000000, 0.000000000000000000 ) ) ;
#42789=CARTESIAN_POINT ( 'NONE',  ( 6.123233995736766282E-16, -170.0000000000000000, -5.000000000000000000 ) ) ;
#42791=VECTOR ( 'NONE', #16690, 1000.000000000000000 ) ;
#42792=CARTESIAN_POINT ( 'NONE',  ( -2.229367062500000163, -6.729166665301073103, -3.861377020970580443 ) ) ;
#42793=ADVANCED_FACE ( 'NONE', ( #25873 ), #31324, .T. ) ;
#42794=AXIS2_PLACEMENT_3D ( 'NONE', #38076, #8800, #42888 ) ;
#42795=CARTESIAN_POINT ( 'NONE',  ( 9.457646018065525792E-16, -40.31249999863440081, 5.148502694627439702 ) ) ;
#42796=( BOUNDED_CURVE ( )  B_SPLINE_CURVE ( 2, ( #27149, #52226, #41931, #27454, #26840, #3348, #22965, #12978, #17508 ),
 .UNSPECIFIED., .F., .F. ) 
 B_SPLINE_CURVE_WITH_KNOTS ( ( 3, 2, 2, 2, 3 ),
 ( 0.7062500000000000444, 0.7069444444444444864, 0.7083333333333333703, 0.7097222222222222543, 0.7104166666666666963 ),
 .UNSPECIFIED. ) 
 CURVE ( )  GEOMETRIC_REPRESENTATION_ITEM ( )  RATIONAL_B_SPLINE_CURVE ( ( 0.9330127018922194093, 0.9330127018922194093, 1.000000000000000000, 0.8660254037844387076, 1.000000000000000000, 0.8660254037844387076, 1.000000000000000000, 0.9330127018922194093, 0.9330127018922194093 ) ) 
 REPRESENTATION_ITEM ( '' )  );
#42802=CARTESIAN_POINT ( 'NONE',  ( -5.000000000000000000, -11.95833333060214798, -2.886751345948128211 ) ) ;
#42803=CARTESIAN_POINT ( 'NONE',  ( -4.458734124999998549, -67.47916666530106511, 2.574251347313722516 ) ) ;
#42804=CARTESIAN_POINT ( 'NONE',  ( -3.152801135295367985, -148.0625000013655779, 3.152801135295367096 ) ) ;
#42809=CARTESIAN_POINT ( 'NONE',  ( -2.229367062499996610, 3.854166668032260823, 3.861377020970582219 ) ) ;
#42810=CARTESIAN_POINT ( 'NONE',  ( 1.339745962155612702, -30.16965819600732956, -5.000000000000000000 ) ) ;
#42811=CARTESIAN_POINT ( 'NONE',  ( 4.458734124999997661, -153.5000000013656063, 1.846868145590737864 ) ) ;
#42813=ORIENTED_EDGE ( 'NONE', *, *, #42564, .T. ) ;
#42821=DIRECTION ( 'NONE',  ( 0.000000000000000000, 0.000000000000000000, 1.000000000000000000 ) ) ;
#42824=CARTESIAN_POINT ( 'NONE',  ( 4.458734125000000326, 23.10416666803225993, 2.574251347313718519 ) ) ;
#42826=CARTESIAN_POINT ( 'NONE',  ( -4.458734124999997661, -5.479166665301072214, 2.574251347313722516 ) ) ;
#42828=CARTESIAN_POINT ( 'NONE',  ( 6.123233995736766282E-16, -170.0000000000000000, -5.000000000000000000 ) ) ;
#42830=CARTESIAN_POINT ( 'NONE',  ( -2.071067811865478170, -142.4375000027311842, 5.000000000000000000 ) ) ;
#42841=CARTESIAN_POINT ( 'NONE',  ( -4.458734125000000326, -158.1250000013656063, 1.846868145590734089 ) ) ;
#42842=( BOUNDED_CURVE ( )  B_SPLINE_CURVE ( 2, ( #54143, #38407, #49644, #4315, #28748, #44489, #58660, #5581, #59296 ),
 .UNSPECIFIED., .F., .F. ) 
 B_SPLINE_CURVE_WITH_KNOTS ( ( 3, 2, 2, 2, 3 ),
 ( 0.6187500000000000222, 0.6194444444444444642, 0.6208333333333333481, 0.6222222222222222321, 0.6229166666666666741 ),
 .UNSPECIFIED. ) 
 CURVE ( )  GEOMETRIC_REPRESENTATION_ITEM ( )  RATIONAL_B_SPLINE_CURVE ( ( 0.9330127018922194093, 0.9330127018922194093, 1.000000000000000000, 0.8660254037844387076, 1.000000000000000000, 0.8660254037844387076, 1.000000000000000000, 0.9330127018922194093, 0.9330127018922194093 ) ) 
 REPRESENTATION_ITEM ( '' )  );
#42845=CARTESIAN_POINT ( 'NONE',  ( 4.458734124999998549, 20.02083333469892779, -2.574251347313721627 ) ) ;
#42846=EDGE_LOOP ( 'NONE', ( #19836, #42458, #665, #34913 ) ) ;
#42851=CARTESIAN_POINT ( 'NONE',  ( 2.499999999999998668, 2.666666666666667851, -4.330127018922193649 ) ) ;
#42852=CARTESIAN_POINT ( 'NONE',  ( 4.458734124999998549, -63.72916666530106511, -2.574251347313721627 ) ) ;
#42853=DIRECTION ( 'NONE',  ( 0.000000000000000000, 0.000000000000000000, 1.000000000000000000 ) ) ;
#42854=CARTESIAN_POINT ( 'NONE',  ( 4.458734124999998549, -26.72916666530106866, -2.574251347313721627 ) ) ;
#42856=FACE_OUTER_BOUND ( 'NONE', #38207, .T. ) ;
#42857=CARTESIAN_POINT ( 'NONE',  ( 5.000000000000000000, -42.49999999999999289, -6.123233995736766282E-16 ) ) ;
#42859=CARTESIAN_POINT ( 'NONE',  ( 1.975475456537005874E-15, -9.750000000000000000, 5.000000000000000000 ) ) ;
#42861=CARTESIAN_POINT ( 'NONE',  ( 5.000000000000000888, -154.9375000000000000, -2.071067811865475505 ) ) ;
#42862=CARTESIAN_POINT ( 'NONE',  ( -4.458734124999998549, -63.22916666530106511, 2.574251347313722516 ) ) ;
#42863=CARTESIAN_POINT ( 'NONE',  ( -4.458734124999999437, -147.1875000013656063, -5.460374474430324690E-16 ) ) ;
#42864=CARTESIAN_POINT ( 'NONE',  ( -3.152548672688508926E-16, -76.56249999863440792, -5.148502694627439702 ) ) ;
#42866=CARTESIAN_POINT ( 'NONE',  ( 4.458734124999999437, -24.06249999863440436, -5.460374474430324690E-16 ) ) ;
#42867=CARTESIAN_POINT ( 'NONE',  ( 2.500000000000002220, -65.54166666393547303, 4.330127018922192761 ) ) ;
#42868=VERTEX_POINT ( 'NONE', #35849 ) ;
#42869=CARTESIAN_POINT ( 'NONE',  ( -6.972266317189433020E-16, -22.24999999999999645, -5.000000000000000000 ) ) ;
#42872=CARTESIAN_POINT ( 'NONE',  ( 3.535533905932738197, -149.0000000027311842, -3.535533905932738197 ) ) ;
#42874=VERTEX_POINT ( 'NONE', #21698 ) ;
#42875=DIRECTION ( 'NONE',  ( -0.000000000000000000, 1.000000000000000000, -0.000000000000000000 ) ) ;
#42876=CARTESIAN_POINT ( 'NONE',  ( -3.152548672688508926E-16, -53.81249999863439371, -5.148502694627439702 ) ) ;
#42880=DIRECTION ( 'NONE',  ( -0.000000000000000000, 1.000000000000000000, -0.000000000000000000 ) ) ;
#42882=CARTESIAN_POINT ( 'NONE',  ( 4.458734124999998549, 18.27083333469893134, -2.574251347313721627 ) ) ;
#42884=CARTESIAN_POINT ( 'NONE',  ( -4.458734125000000326, -167.8750000013656063, 1.846868145590734089 ) ) ;
#42885=( BOUNDED_CURVE ( )  B_SPLINE_CURVE ( 2, ( #2023, #2331, #7783, #27386, #56041, #60238, #41536, #26441, #35783 ),
 .UNSPECIFIED., .F., .F. ) 
 B_SPLINE_CURVE_WITH_KNOTS ( ( 3, 2, 2, 2, 3 ),
 ( 0.5250000000000004663, 0.5291666666666671182, 0.5333333333333338810, 0.5375000000000005329, 0.5416666666666671848 ),
 .UNSPECIFIED. ) 
 CURVE ( )  GEOMETRIC_REPRESENTATION_ITEM ( )  RATIONAL_B_SPLINE_CURVE ( ( 0.9999999999999918954, 0.9238795325112948431, 1.000000000000000000, 0.9238795325112867385, 1.000000000000000000, 0.9238795325112867385, 1.000000000000000000, 0.9238795325112766355, 1.000000000000010214 ) ) 
 REPRESENTATION_ITEM ( '' )  );
#42888=DIRECTION ( 'NONE',  ( 0.000000000000000000, 0.000000000000000000, 1.000000000000000000 ) ) ;
#42894=CARTESIAN_POINT ( 'NONE',  ( 5.000000000000000000, -45.41666666666665719, -2.886751345948130876 ) ) ;
#42895=DIRECTION ( 'NONE',  ( 0.000000000000000000, 0.000000000000000000, 1.000000000000000000 ) ) ;
#42896=CARTESIAN_POINT ( 'NONE',  ( -2.071067811865308972, -156.3125000000000568, 5.000000000000169642 ) ) ;
#42902=CARTESIAN_POINT ( 'NONE',  ( 5.000000000000000000, -152.1875000027312126, 2.071067811865478614 ) ) ;
#42908=CARTESIAN_POINT ( 'NONE',  ( -5.000000000000000000, -144.5000000000000284, -6.123233995736766282E-16 ) ) ;
#42909=EDGE_CURVE ( 'NONE', #42031, #42211, #7223, .T. ) ;
#42910=EDGE_CURVE ( 'NONE', #57087, #33853, #18367, .T. ) ;
#42913=CARTESIAN_POINT ( 'NONE',  ( 4.458734124999999437, -169.6250000013656063, -1.846868145590734978 ) ) ;
#42914=CARTESIAN_POINT ( 'NONE',  ( 4.458734124999998549, -30.72916666530107221, -2.574251347313721627 ) ) ;
#42915=EDGE_CURVE ( 'NONE', #45427, #46757, #47117, .T. ) ;
#42919=CARTESIAN_POINT ( 'NONE',  ( -4.458734125000001214, -146.8750000013656063, 1.846868145590734089 ) ) ;
#42921=DIRECTION ( 'NONE',  ( -0.000000000000000000, 1.000000000000000000, -0.000000000000000000 ) ) ;
#42922=CARTESIAN_POINT ( 'NONE',  ( -2.229367062500000163, -58.72916666530106511, -3.861377020970580443 ) ) ;
#42926=CARTESIAN_POINT ( 'NONE',  ( 5.000000000000000000, 21.58333333333333215, -2.886751345948129988 ) ) ;
#42927=AXIS2_PLACEMENT_3D ( 'NONE', #41741, #54242, #53923 ) ;
#42929=EDGE_CURVE ( 'NONE', #53932, #31664, #38096, .T. ) ;
#42930=CARTESIAN_POINT ( 'NONE',  ( 1.975475456537005874E-15, -36.62499999726880873, 5.000000000000000000 ) ) ;
#42931=CARTESIAN_POINT ( 'NONE',  ( -4.458734124999999437, -2.312499998634407028, 0.000000000000000000 ) ) ;
#42932=CARTESIAN_POINT ( 'NONE',  ( 3.061616997868383141E-16, -154.7500000000000000, -5.000000000000000000 ) ) ;
#42934=CARTESIAN_POINT ( 'NONE',  ( 4.458734124999998549, 9.020833334698927786, -2.574251347313721627 ) ) ;
#42938=CARTESIAN_POINT ( 'NONE',  ( 4.458734124999998549, -46.72916666530106511, -2.574251347313721627 ) ) ;
#42940=CARTESIAN_POINT ( 'NONE',  ( -4.458734125000001214, -158.1250000013656063, 1.846868145590734089 ) ) ;
#42942=CARTESIAN_POINT ( 'NONE',  ( -5.000000000000000000, -51.95833333060213732, -2.886751345948128211 ) ) ;
#42944=CARTESIAN_POINT ( 'NONE',  ( -2.229367062499996610, -22.14583333196773651, 3.861377020970582219 ) ) ;
#42946=DIRECTION ( 'NONE',  ( 0.000000000000000000, 0.000000000000000000, 1.000000000000000000 ) ) ;
#42948=CARTESIAN_POINT ( 'NONE',  ( 1.846868145590736310, -160.6250000013655779, 4.458734124999999437 ) ) ;
#42949=ORIENTED_EDGE ( 'NONE', *, *, #25351, .T. ) ;
#42950=CARTESIAN_POINT ( 'NONE',  ( 1.339745962155612702, -39.16965819600733312, -5.000000000000000000 ) ) ;
#42952=CARTESIAN_POINT ( 'NONE',  ( 4.458734125000001214, -39.14583333196773651, 2.574251347313718519 ) ) ;
#42957=ORIENTED_EDGE ( 'NONE', *, *, #57781, .T. ) ;
#42959=CARTESIAN_POINT ( 'NONE',  ( -4.458734124999998549, -85.47916666530106511, 2.574251347313722516 ) ) ;
#42962=CARTESIAN_POINT ( 'NONE',  ( -2.071067811865372921, -158.4375000027312126, 5.000000000000104805 ) ) ;
#42965=CARTESIAN_POINT ( 'NONE',  ( 1.339745962155615144, -37.70534180126148271, 4.999999999999999112 ) ) ;
#42973=CARTESIAN_POINT ( 'NONE',  ( 0.000000000000000000, -170.0000000000000000, 0.000000000000000000 ) ) ;
#42974=CARTESIAN_POINT ( 'NONE',  ( 1.975475456537005874E-15, -60.75000000000000000, 5.000000000000000000 ) ) ;
#42975=CARTESIAN_POINT ( 'NONE',  ( -4.458734124999999437, -84.56249999863439371, 0.000000000000000000 ) ) ;
#42978=ORIENTED_EDGE ( 'NONE', *, *, #33339, .T. ) ;
#42979=CARTESIAN_POINT ( 'NONE',  ( -5.000000000000000000, -16.87499999726881583, 0.000000000000000000 ) ) ;
#42981=CARTESIAN_POINT ( 'NONE',  ( -2.071067811865475061, -164.8125000027312126, -5.000000000000000888 ) ) ;
#42987=( BOUNDED_CURVE ( )  B_SPLINE_CURVE ( 2, ( #12569, #32182, #51813, #7755, #27358, #22553, #12884, #33449, #38893 ),
 .UNSPECIFIED., .F., .F. ) 
 B_SPLINE_CURVE_WITH_KNOTS ( ( 3, 2, 2, 2, 3 ),
 ( 0.5270833333333333481, 0.5277777777777777901, 0.5291666666666666741, 0.5305555555555555580, 0.5312500000000000000 ),
 .UNSPECIFIED. ) 
 CURVE ( )  GEOMETRIC_REPRESENTATION_ITEM ( )  RATIONAL_B_SPLINE_CURVE ( ( 0.9330127018922194093, 0.9330127018922194093, 1.000000000000000000, 0.8660254037844387076, 1.000000000000000000, 0.8660254037844387076, 1.000000000000000000, 0.9330127018922194093, 0.9330127018922194093 ) ) 
 REPRESENTATION_ITEM ( '' )  );
#42992=CARTESIAN_POINT ( 'NONE',  ( 1.255007937094098239E-14, 23.75000000000000000, -4.999999999999999112 ) ) ;
#42993=CARTESIAN_POINT ( 'NONE',  ( 4.458734124999999437, -14.81249999863440436, -5.460374474430324690E-16 ) ) ;
#42996=CARTESIAN_POINT ( 'NONE',  ( 2.229367062499998831, -40.89583333196773651, -3.861377020970580887 ) ) ;
#42998=CARTESIAN_POINT ( 'NONE',  ( 2.500000000000002220, 0.4583333360645182042, 4.330127018922192761 ) ) ;
#43002=CARTESIAN_POINT ( 'NONE',  ( 4.458734124999999437, 15.18750000136559564, -5.460374474430324690E-16 ) ) ;
#43004=CARTESIAN_POINT ( 'NONE',  ( -5.000000000000000000, -64.95833333060213022, -2.886751345948128211 ) ) ;
#43005=CARTESIAN_POINT ( 'NONE',  ( -2.229367062499996610, -87.39583333196773651, 3.861377020970582219 ) ) ;
#43007=CARTESIAN_POINT ( 'NONE',  ( 5.000000000000000000, 11.70833333606451809, -2.886751345948129988 ) ) ;
#43008=EDGE_CURVE ( 'NONE', #31402, #12840, #60277, .T. ) ;
#43010=CARTESIAN_POINT ( 'NONE',  ( 5.000000000000000000, -25.50000000000000355, -6.123233995736766282E-16 ) ) ;
#43011=PRODUCT_DEFINITION_SHAPE ( 'NONE', 'NONE',  #40220 ) ;
#43012=VECTOR ( 'NONE', #46185, 1000.000000000000000 ) ;
#43015=CARTESIAN_POINT ( 'NONE',  ( -2.500000000000000444, -30.16666666666666785, -4.330127018922193649 ) ) ;
#43016=CARTESIAN_POINT ( 'NONE',  ( -4.458734124999998549, -33.22916666530107221, 2.574251347313722516 ) ) ;
#43019=CARTESIAN_POINT ( 'NONE',  ( 5.000000000000000888, -35.45833333060213732, 2.886751345948126879 ) ) ;
#43020=CARTESIAN_POINT ( 'NONE',  ( -3.152548672688508926E-16, -62.56249999863440792, -5.148502694627439702 ) ) ;
#43021=ORIENTED_EDGE ( 'NONE', *, *, #55147, .F. ) ;
#43023=CARTESIAN_POINT ( 'NONE',  ( 4.458734125000001214, -9.145833331967736513, 2.574251347313718519 ) ) ;
#43025=CARTESIAN_POINT ( 'NONE',  ( 5.000000000000000000, -78.50000000000000000, -6.123233995736766282E-16 ) ) ;
#43028=CARTESIAN_POINT ( 'NONE',  ( 1.060575238724906964E-15, -75.62499999726880162, 5.773502691896257311 ) ) ;
#43029=CARTESIAN_POINT ( 'NONE',  ( 5.000000000000000000, -65.37499999726881583, -6.123233995736766282E-16 ) ) ;
#43030=ORIENTED_EDGE ( 'NONE', *, *, #8682, .F. ) ;
#43032=CARTESIAN_POINT ( 'NONE',  ( -4.458734124999998549, -19.47916666530107221, 2.574251347313722516 ) ) ;
#43033=CARTESIAN_POINT ( 'NONE',  ( 2.229367062499998831, -55.89583333196773651, -3.861377020970580887 ) ) ;
#43036=CARTESIAN_POINT ( 'NONE',  ( -4.458734125000001214, -167.1250000013656063, 1.846868145590734089 ) ) ;
#43046=CARTESIAN_POINT ( 'NONE',  ( 2.730187237215162345E-16, -144.4375000013656063, -4.458734124999999437 ) ) ;
#43050=CARTESIAN_POINT ( 'NONE',  ( 9.457646018065525792E-16, -67.31249999863440792, 5.148502694627439702 ) ) ;
#43053=CARTESIAN_POINT ( 'NONE',  ( -1.846868145590734756, -140.1250000013656347, -4.458734124999999437 ) ) ;
#43054=AXIS2_PLACEMENT_3D ( 'NONE', #62200, #38367, #13919 ) ;
#43061=CARTESIAN_POINT ( 'NONE',  ( 0.000000000000000000, -170.0000000000000000, 0.000000000000000000 ) ) ;
#43063=CARTESIAN_POINT ( 'NONE',  ( -4.458734124999999437, 21.43750000136559208, 0.000000000000000000 ) ) ;
#43064=DIRECTION ( 'NONE',  ( -0.000000000000000000, 1.000000000000000000, -0.000000000000000000 ) ) ;
#43069=CARTESIAN_POINT ( 'NONE',  ( -6.972266317189433020E-16, -80.24999999999998579, -5.000000000000000000 ) ) ;
#43070=CARTESIAN_POINT ( 'NONE',  ( 2.229367062499998831, 0.3541666680322609340, -3.861377020970580887 ) ) ;
#43071=CARTESIAN_POINT ( 'NONE',  ( -4.458734124999997661, -22.47916666530107221, 2.574251347313722516 ) ) ;
#43073=CARTESIAN_POINT ( 'NONE',  ( -3.152801135295367985, -154.8125000013656063, 3.152801135295367096 ) ) ;
#43076=CARTESIAN_POINT ( 'NONE',  ( 1.339745962155624914, 15.70534180126147561, -4.999999999999991118 ) ) ;
#43079=CARTESIAN_POINT ( 'NONE',  ( -2.229367062500000163, -69.72916666530107932, -3.861377020970580443 ) ) ;
#43081=CARTESIAN_POINT ( 'NONE',  ( 1.975475456537005874E-15, -73.75000000000000000, 5.000000000000000000 ) ) ;
#43082=CARTESIAN_POINT ( 'NONE',  ( 2.500000000000002220, 27.45833333606451632, 4.330127018922192761 ) ) ;
#43083=ORIENTED_EDGE ( 'NONE', *, *, #31000, .F. ) ;
#43085=CARTESIAN_POINT ( 'NONE',  ( -1.339745962155613812, 11.91965820146970678, -5.000000000000000000 ) ) ;
#43086=CARTESIAN_POINT ( 'NONE',  ( 2.500000000000002220, -13.66666666666666785, 4.330127018922192761 ) ) ;
#43087=CARTESIAN_POINT ( 'NONE',  ( -4.458734124999999437, -16.31249999863440436, 0.000000000000000000 ) ) ;
#43088=CARTESIAN_POINT ( 'NONE',  ( 2.229367062500001939, -79.97916666530106511, 3.861377020970579999 ) ) ;
#43089=CARTESIAN_POINT ( 'NONE',  ( -4.458734124999999437, -169.1875000013656063, -5.460374474430324690E-16 ) ) ;
#43090=CARTESIAN_POINT ( 'NONE',  ( -4.999999999999999112, -19.79166666393547658, 2.886751345948131764 ) ) ;
#43091=CARTESIAN_POINT ( 'NONE',  ( -3.152548672688508926E-16, -43.56249999863440081, -5.148502694627439702 ) ) ;
#43094=CARTESIAN_POINT ( 'NONE',  ( -4.458734124999999437, 7.354166668032259935, -2.574251347313719407 ) ) ;
#43095=EDGE_LOOP ( 'NONE', ( #51427, #45805, #55582, #63050 ) ) ;
#43097=CARTESIAN_POINT ( 'NONE',  ( 5.000000000000000888, -60.58333333333332860, 2.886751345948126879 ) ) ;
#43098=CARTESIAN_POINT ( 'NONE',  ( 1.846868145590735200, -156.5000000013656347, -4.458734125000000326 ) ) ;
#43102=CARTESIAN_POINT ( 'NONE',  ( -3.535533905932738641, -166.3750000000000284, 3.535533905932737309 ) ) ;
#43103=AXIS2_PLACEMENT_3D ( 'NONE', #46378, #12593, #2326 ) ;
#43105=CARTESIAN_POINT ( 'NONE',  ( 4.458734124999999437, -5.062499998634402587, -5.460374474430324690E-16 ) ) ;
#43106=CARTESIAN_POINT ( 'NONE',  ( 2.229367062500001939, -39.22916666530107221, 3.861377020970579999 ) ) ;
#43108=CARTESIAN_POINT ( 'NONE',  ( -1.846868145590737420, -148.7500000013656063, 4.458734124999999437 ) ) ;
#43111=VERTEX_POINT ( 'NONE', #51909 ) ;
#43112=CARTESIAN_POINT ( 'NONE',  ( -3.535533905932738641, -141.3750000000000000, 3.535533905932737309 ) ) ;
#43114=CARTESIAN_POINT ( 'NONE',  ( -2.229367062500000163, -70.72916666530107932, -3.861377020970580443 ) ) ;
#43120=CARTESIAN_POINT ( 'NONE',  ( -4.458734124999999437, 3.604166668032260379, -2.574251347313719407 ) ) ;
#43122=CARTESIAN_POINT ( 'NONE',  ( 4.458734124999999437, -151.4375000013655779, 0.000000000000000000 ) ) ;
#43135=CARTESIAN_POINT ( 'NONE',  ( 5.000000000000000000, -44.41666666666665719, -2.886751345948130876 ) ) ;
#43136=CARTESIAN_POINT ( 'NONE',  ( -3.152548672688508926E-16, 23.43750000136559564, -5.148502694627439702 ) ) ;
#43138=CARTESIAN_POINT ( 'NONE',  ( 2.229367062500001939, -6.229166665301072214, 3.861377020970579999 ) ) ;
#43141=CARTESIAN_POINT ( 'NONE',  ( -1.846868145590737420, -166.7500000013655779, 4.458734124999999437 ) ) ;
#43143=AXIS2_PLACEMENT_3D ( 'NONE', #47374, #56720, #52198 ) ;
#43150=CARTESIAN_POINT ( 'NONE',  ( -3.152801135295367985, -159.0625000013656063, 3.152801135295367096 ) ) ;
#43152=CARTESIAN_POINT ( 'NONE',  ( 0.000000000000000000, -170.0000000000000000, 0.000000000000000000 ) ) ;
#43155=ORIENTED_EDGE ( 'NONE', *, *, #44875, .F. ) ;
#43159=CYLINDRICAL_SURFACE ( 'NONE', #27820, 5.000000000000000000 ) ;
#43160=CARTESIAN_POINT ( 'NONE',  ( -4.999999999999999112, 2.083333333333333037, 2.886751345948131764 ) ) ;
#43161=CARTESIAN_POINT ( 'NONE',  ( -2.229367062500000163, -63.47916666530106511, -3.861377020970580443 ) ) ;
#43162=( BOUNDED_CURVE ( )  B_SPLINE_CURVE ( 2, ( #46454, #2399, #14544, #32922, #14232, #34164, #28708, #13298, #29016 ),
 .UNSPECIFIED., .F., .F. ) 
 B_SPLINE_CURVE_WITH_KNOTS ( ( 3, 2, 2, 2, 3 ),
 ( 0.8895833333333332815, 0.8902777777777777235, 0.8916666666666667185, 0.8930555555555556024, 0.8937500000000000444 ),
 .UNSPECIFIED. ) 
 CURVE ( )  GEOMETRIC_REPRESENTATION_ITEM ( )  RATIONAL_B_SPLINE_CURVE ( ( 0.9330127018922194093, 0.9330127018922194093, 1.000000000000000000, 0.8660254037844387076, 1.000000000000000000, 0.8660254037844387076, 1.000000000000000000, 0.9330127018922194093, 0.9330127018922194093 ) ) 
 REPRESENTATION_ITEM ( '' )  );
#43163=CARTESIAN_POINT ( 'NONE',  ( -2.499999999999996447, -7.833333333333331261, 4.330127018922195425 ) ) ;
#43164=CARTESIAN_POINT ( 'NONE',  ( -5.000000000000000000, 4.125000002731186832, 0.000000000000000000 ) ) ;
#43165=CARTESIAN_POINT ( 'NONE',  ( -3.152548672688508926E-16, -27.56249999863440081, -5.148502694627439702 ) ) ;
#43167=CARTESIAN_POINT ( 'NONE',  ( -5.000000000000000000, 26.12500000273118417, 0.000000000000000000 ) ) ;
#43169=CARTESIAN_POINT ( 'NONE',  ( 2.499999999999998668, -45.33333333333333570, -4.330127018922193649 ) ) ;
#43172=CARTESIAN_POINT ( 'NONE',  ( 5.000000000000000000, -155.0000000000000284, 0.000000000000000000 ) ) ;
#43173=CARTESIAN_POINT ( 'NONE',  ( -2.229367062500000163, -70.47916666530107932, -3.861377020970580443 ) ) ;
#43174=CARTESIAN_POINT ( 'NONE',  ( 4.458734125000000326, -149.6250000013655779, -1.846868145590734978 ) ) ;
#43175=CARTESIAN_POINT ( 'NONE',  ( -3.152548672688508926E-16, -75.56249999863439371, -5.148502694627439702 ) ) ;
#43177=CARTESIAN_POINT ( 'NONE',  ( -4.458734124999999437, -27.64583333196774007, -2.574251347313719407 ) ) ;
#43178=CARTESIAN_POINT ( 'NONE',  ( -3.535250795749689387E-16, -66.12499999726881583, -5.773502691896257311 ) ) ;
#43179=VERTEX_POINT ( 'NONE', #25078 ) ;
#43180=CARTESIAN_POINT ( 'NONE',  ( -6.972266317189433020E-16, -74.25000000000000000, -5.000000000000000000 ) ) ;
#43183=CARTESIAN_POINT ( 'NONE',  ( -5.000000000000000000, 8.125000002731187720, 0.000000000000000000 ) ) ;
#43186=AXIS2_PLACEMENT_3D ( 'NONE', #14889, #44798, #39969 ) ;
#43187=DIRECTION ( 'NONE',  ( 0.000000000000000000, 0.000000000000000000, 1.000000000000000000 ) ) ;
#43188=CARTESIAN_POINT ( 'NONE',  ( 9.457646018065525792E-16, -55.31249999863439371, 5.148502694627439702 ) ) ;
#43193=CARTESIAN_POINT ( 'NONE',  ( 2.229367062500001939, 21.02083333469892779, 3.861377020970579999 ) ) ;
#43195=CARTESIAN_POINT ( 'NONE',  ( -5.000000000000000000, -2.083333333333333037, -2.886751345948128211 ) ) ;
#43196=CARTESIAN_POINT ( 'NONE',  ( -3.152801135295367096, -167.0625000013656063, -3.152801135295367541 ) ) ;
#43197=ORIENTED_EDGE ( 'NONE', *, *, #59421, .F. ) ;
#43200=CARTESIAN_POINT ( 'NONE',  ( -4.999999999999998224, -39.91666666666667140, 2.886751345948131764 ) ) ;
#43207=CARTESIAN_POINT ( 'NONE',  ( 1.975475456537005874E-15, -61.74999999999999289, 5.000000000000000000 ) ) ;
#43209=CARTESIAN_POINT ( 'NONE',  ( -1.049326080737009628E-13, -18.62499999726881583, 5.000000000000000000 ) ) ;
#43213=( BOUNDED_CURVE ( )  B_SPLINE_CURVE ( 2, ( #36784, #37111, #57361, #41272, #56417, #51894, #8156, #46747, #2383 ),
 .UNSPECIFIED., .F., .F. ) 
 B_SPLINE_CURVE_WITH_KNOTS ( ( 3, 2, 2, 2, 3 ),
 ( 0.1395833333333333370, 0.1402777777777777790, 0.1416666666666666630, 0.1430555555555555469, 0.1437499999999999889 ),
 .UNSPECIFIED. ) 
 CURVE ( )  GEOMETRIC_REPRESENTATION_ITEM ( )  RATIONAL_B_SPLINE_CURVE ( ( 0.9330127018922194093, 0.9330127018922194093, 1.000000000000000000, 0.8660254037844387076, 1.000000000000000000, 0.8660254037844387076, 1.000000000000000000, 0.9330127018922194093, 0.9330127018922194093 ) ) 
 REPRESENTATION_ITEM ( '' )  );
#43214=CARTESIAN_POINT ( 'NONE',  ( 2.500000000000002220, 11.33333333333333393, 4.330127018922192761 ) ) ;
#43216=CARTESIAN_POINT ( 'NONE',  ( -5.000000000000000888, -154.5625000027311842, 2.071067811865474617 ) ) ;
#43217=EDGE_LOOP ( 'NONE', ( #12729, #36234, #9780, #16363, #63290, #23433, #62591, #45803 ) ) ;
#43222=CARTESIAN_POINT ( 'NONE',  ( 3.061616997868383141E-16, -143.7500000000000284, -5.000000000000000000 ) ) ;
#43224=CARTESIAN_POINT ( 'NONE',  ( -1.127183054612291972E-14, 22.37500000273118417, 4.999999999999999112 ) ) ;
#43225=CARTESIAN_POINT ( 'NONE',  ( 4.458734124999998549, -29.72916666530107221, -2.574251347313721627 ) ) ;
#43229=CARTESIAN_POINT ( 'NONE',  ( -4.458734125000001214, -145.8750000013656063, 1.846868145590734089 ) ) ;
#43231=CARTESIAN_POINT ( 'NONE',  ( -4.458734124999997661, -59.47916666530106511, 2.574251347313722516 ) ) ;
#43233=CARTESIAN_POINT ( 'NONE',  ( -2.071067811865394237, -162.3125000000000568, 5.000000000000084377 ) ) ;
#43234=CARTESIAN_POINT ( 'NONE',  ( 1.060575238724906964E-15, 17.25000000000000000, 5.773502691896257311 ) ) ;
#43236=CARTESIAN_POINT ( 'NONE',  ( -4.458734124999998549, -4.229166665301070438, 2.574251347313722516 ) ) ;
#43239=CARTESIAN_POINT ( 'NONE',  ( 5.000000000000000000, -165.1250000027311842, 0.000000000000000000 ) ) ;
#43240=CARTESIAN_POINT ( 'NONE',  ( 4.458734124999998549, 11.02083333469892779, -2.574251347313721627 ) ) ;
#43242=CARTESIAN_POINT ( 'NONE',  ( 0.000000000000000000, -170.0000000000000000, 0.000000000000000000 ) ) ;
#43245=CARTESIAN_POINT ( 'NONE',  ( 2.229367062499998831, -48.64583333196772941, -3.861377020970580887 ) ) ;
#43246=CARTESIAN_POINT ( 'NONE',  ( 3.152801135295367541, -159.5625000013656063, -3.152801135295367541 ) ) ;
#43247=CARTESIAN_POINT ( 'NONE',  ( -5.000000000000000000, -47.95833333060214443, -2.886751345948128211 ) ) ;
#43248=ORIENTED_EDGE ( 'NONE', *, *, #20924, .F. ) ;
#43249=CARTESIAN_POINT ( 'NONE',  ( 2.229367062499998831, -22.64583333196773651, -3.861377020970580887 ) ) ;
#43253=CARTESIAN_POINT ( 'NONE',  ( 1.846868145590735200, -159.2500000013656063, -4.458734125000000326 ) ) ;
#43254=ORIENTED_EDGE ( 'NONE', *, *, #38463, .T. ) ;
#43259=CARTESIAN_POINT ( 'NONE',  ( -3.152548672688508926E-16, -35.81249999863440792, -5.148502694627439702 ) ) ;
#43260=VERTEX_POINT ( 'NONE', #40506 ) ;
#43261=EDGE_CURVE ( 'NONE', #22693, #46689, #54992, .T. ) ;
#43265=CYLINDRICAL_SURFACE ( 'NONE', #6076, 5.000000000000000000 ) ;
#43267=ORIENTED_EDGE ( 'NONE', *, *, #17229, .F. ) ;
#43269=CARTESIAN_POINT ( 'NONE',  ( 2.229367062500001939, -87.22916666530107932, 3.861377020970579999 ) ) ;
#43272=CARTESIAN_POINT ( 'NONE',  ( 1.975475456537005874E-15, -8.624999997268812280, 5.000000000000000000 ) ) ;
#43278=ADVANCED_FACE ( 'NONE', ( #49522 ), #50492, .T. ) ;
#43280=DIRECTION ( 'NONE',  ( -0.000000000000000000, 1.000000000000000000, -0.000000000000000000 ) ) ;
#43283=DIRECTION ( 'NONE',  ( -0.000000000000000000, 1.000000000000000000, -0.000000000000000000 ) ) ;
#43286=CARTESIAN_POINT ( 'NONE',  ( 2.229367062499998831, -85.89583333196773651, -3.861377020970580887 ) ) ;
#43289=ORIENTED_EDGE ( 'NONE', *, *, #58542, .T. ) ;
#43293=CARTESIAN_POINT ( 'NONE',  ( 3.535533905932738197, -164.0000000027312126, -3.535533905932738197 ) ) ;
#43302=CARTESIAN_POINT ( 'NONE',  ( -6.972266317189433020E-16, -76.24999999999998579, -5.000000000000000000 ) ) ;
#43304=CARTESIAN_POINT ( 'NONE',  ( 2.229367062500001939, -12.97916666530107221, 3.861377020970579999 ) ) ;
#43305=CARTESIAN_POINT ( 'NONE',  ( 1.975475456537005874E-15, -71.75000000000000000, 5.000000000000000000 ) ) ;
#43307=CARTESIAN_POINT ( 'NONE',  ( -4.458734124999999437, -42.56249999863440081, 0.000000000000000000 ) ) ;
#43314=CARTESIAN_POINT ( 'NONE',  ( -4.458734124999999437, 16.60416666803225993, -2.574251347313719407 ) ) ;
#43317=CARTESIAN_POINT ( 'NONE',  ( -2.229367062499996610, -88.39583333196773651, 3.861377020970582219 ) ) ;
#43319=CARTESIAN_POINT ( 'NONE',  ( -2.500000000000000444, 13.95833333606451809, -4.330127018922193649 ) ) ;
#43320=ORIENTED_EDGE ( 'NONE', *, *, #45337, .T. ) ;
#43322=CARTESIAN_POINT ( 'NONE',  ( -6.972266317189433020E-16, -3.250000000000001332, -5.000000000000000000 ) ) ;
#43323=CARTESIAN_POINT ( 'NONE',  ( 5.000000000000000888, -26.58333333333333570, 2.886751345948126879 ) ) ;
#43324=CARTESIAN_POINT ( 'NONE',  ( 2.229367062500001939, -32.97916666530106511, 3.861377020970579999 ) ) ;
#43325=CARTESIAN_POINT ( 'NONE',  ( 1.060575238724906964E-15, -31.62499999726880873, 5.773502691896257311 ) ) ;
#43326=CARTESIAN_POINT ( 'NONE',  ( -4.458734124999998549, -63.22916666530106511, 2.574251347313722516 ) ) ;
#43329=CARTESIAN_POINT ( 'NONE',  ( -4.458734124999999437, -13.64583333196774007, -2.574251347313719407 ) ) ;
#43330=ORIENTED_EDGE ( 'NONE', *, *, #3220, .T. ) ;
#43331=CARTESIAN_POINT ( 'NONE',  ( -2.500000000000000444, -79.16666666666665719, -4.330127018922193649 ) ) ;
#43332=CARTESIAN_POINT ( 'NONE',  ( 6.972266317189433020E-16, 28.87500000273118417, -5.000000000000000000 ) ) ;
#43334=CARTESIAN_POINT ( 'NONE',  ( -4.999999999999999112, -83.79166666393547303, 2.886751345948131764 ) ) ;
#43336=VERTEX_POINT ( 'NONE', #5779 ) ;
#43338=CARTESIAN_POINT ( 'NONE',  ( -2.229367062500000163, -22.72916666530107221, -3.861377020970580443 ) ) ;
#43339=CARTESIAN_POINT ( 'NONE',  ( -3.152548672688508926E-16, -57.81249999863440081, -5.148502694627439702 ) ) ;
#43340=ORIENTED_EDGE ( 'NONE', *, *, #22117, .F. ) ;
#43342=EDGE_CURVE ( 'NONE', #18684, #61278, #16306, .T. ) ;
#43344=CARTESIAN_POINT ( 'NONE',  ( -3.152801135295367096, -166.3125000013656063, -3.152801135295367541 ) ) ;
#43346=CARTESIAN_POINT ( 'NONE',  ( -4.999999999999998224, 18.08333333333333215, 2.886751345948131764 ) ) ;
#43351=CARTESIAN_POINT ( 'NONE',  ( 1.975475456537005874E-15, -32.62499999726880873, 5.000000000000000000 ) ) ;
#43354=( BOUNDED_CURVE ( )  B_SPLINE_CURVE ( 2, ( #17718, #27991, #21912, #51507, #46670, #51191, #7123, #52134, #47610 ),
 .UNSPECIFIED., .F., .F. ) 
 B_SPLINE_CURVE_WITH_KNOTS ( ( 3, 2, 2, 2, 3 ),
 ( 0.9187499999999999556, 0.9194444444444443976, 0.9208333333333332815, 0.9222222222222222765, 0.9229166666666667185 ),
 .UNSPECIFIED. ) 
 CURVE ( )  GEOMETRIC_REPRESENTATION_ITEM ( )  RATIONAL_B_SPLINE_CURVE ( ( 0.9330127018922194093, 0.9330127018922194093, 1.000000000000000000, 0.8660254037844387076, 1.000000000000000000, 0.8660254037844387076, 1.000000000000000000, 0.9330127018922194093, 0.9330127018922194093 ) ) 
 REPRESENTATION_ITEM ( '' )  );
#43355=CARTESIAN_POINT ( 'NONE',  ( -8.190561711645485556E-16, -143.9375000013656063, 4.458734124999999437 ) ) ;
#43357=CARTESIAN_POINT ( 'NONE',  ( 2.500000000000002220, -70.66666666666667140, 4.330127018922192761 ) ) ;
#43359=CARTESIAN_POINT ( 'NONE',  ( -4.458734124999999437, -70.56249999863439371, 0.000000000000000000 ) ) ;
#43362=CARTESIAN_POINT ( 'NONE',  ( 0.000000000000000000, -170.0000000000000000, 0.000000000000000000 ) ) ;
#43363=CARTESIAN_POINT ( 'NONE',  ( -4.458734124999999437, -141.0000000013655779, -1.846868145590735644 ) ) ;
#43366=CYLINDRICAL_SURFACE ( 'NONE', #35690, 5.000000000000000000 ) ;
#43367=ADVANCED_FACE ( 'NONE', ( #26993 ), #36641, .T. ) ;
#43373=CARTESIAN_POINT ( 'NONE',  ( 2.229367062499998831, 24.10416666803225993, -3.861377020970580887 ) ) ;
#43376=EDGE_CURVE ( 'NONE', #48933, #41789, #51129, .T. ) ;
#43380=DIRECTION ( 'NONE',  ( 0.000000000000000000, 0.000000000000000000, 1.000000000000000000 ) ) ;
#43381=CARTESIAN_POINT ( 'NONE',  ( -3.152548672688508926E-16, 1.437500001365596525, -5.148502694627439702 ) ) ;
#43382=CARTESIAN_POINT ( 'NONE',  ( 2.229367062500001939, -24.22916666530107577, 3.861377020970579999 ) ) ;
#43383=CARTESIAN_POINT ( 'NONE',  ( -4.458734125000000326, -154.0000000013655779, -1.846868145590735644 ) ) ;
#43386=CARTESIAN_POINT ( 'NONE',  ( -3.152548672688508926E-16, 28.43750000136559208, -5.148502694627439702 ) ) ;
#43389=CARTESIAN_POINT ( 'NONE',  ( -2.229367062500000163, -72.72916666530107932, -3.861377020970580443 ) ) ;
#43391=CARTESIAN_POINT ( 'NONE',  ( -5.000000000000000000, -65.95833333060213022, -2.886751345948128211 ) ) ;
#43392=LINE ( 'NONE', #28602, #26355 ) ;
#43396=CARTESIAN_POINT ( 'NONE',  ( 2.500000000000002220, -10.66666666666666430, 4.330127018922192761 ) ) ;
#43397=CARTESIAN_POINT ( 'NONE',  ( 9.457646018065525792E-16, -16.06249999863440436, 5.148502694627439702 ) ) ;
#43398=CARTESIAN_POINT ( 'NONE',  ( -4.458734124999999437, -79.31249999863440792, 0.000000000000000000 ) ) ;
#43399=CARTESIAN_POINT ( 'NONE',  ( -3.152801135295367096, -166.3125000013656063, -3.152801135295367541 ) ) ;
#43400=CARTESIAN_POINT ( 'NONE',  ( -5.000000000000000000, -16.87499999726881583, 0.000000000000000000 ) ) ;
#43401=CARTESIAN_POINT ( 'NONE',  ( -4.458734124999998549, -47.22916666530106511, 2.574251347313722516 ) ) ;
#43403=CARTESIAN_POINT ( 'NONE',  ( 1.339745962155612702, -15.16965819600733134, -5.000000000000000000 ) ) ;
#43404=CARTESIAN_POINT ( 'NONE',  ( 4.458734124999999437, 1.937500001365593416, -5.460374474430324690E-16 ) ) ;
#43407=CARTESIAN_POINT ( 'NONE',  ( 5.000000000000000000, -58.41666666666665719, -2.886751345948129988 ) ) ;
#43408=CARTESIAN_POINT ( 'NONE',  ( 4.458734124999999437, -154.7500000013656063, 1.846868145590737864 ) ) ;
#43410=CARTESIAN_POINT ( 'NONE',  ( -5.000000000000000000, -79.08333333333332860, -2.886751345948128211 ) ) ;
#43412=CARTESIAN_POINT ( 'NONE',  ( 2.071067811865475505, -163.8125000000000284, -5.000000000000000888 ) ) ;
#43413=CARTESIAN_POINT ( 'NONE',  ( 5.000000000000000000, -11.49999999999999645, -6.123233995736766282E-16 ) ) ;
#43415=CARTESIAN_POINT ( 'NONE',  ( -4.458734124999999437, -5.645833331967740953, -2.574251347313719407 ) ) ;
#43416=CARTESIAN_POINT ( 'NONE',  ( 4.458734124999998549, -41.97916666530107932, -2.574251347313721627 ) ) ;
#43419=CARTESIAN_POINT ( 'NONE',  ( -4.458734125000000326, -149.0000000013656063, -1.846868145590735644 ) ) ;
#43422=VERTEX_POINT ( 'NONE', #42091 ) ;
#43426=CARTESIAN_POINT ( 'NONE',  ( -6.972266317189433020E-16, -2.124999997268814056, -5.000000000000000000 ) ) ;
#43427=CARTESIAN_POINT ( 'NONE',  ( -3.152548672688508926E-16, -77.81249999863440792, -5.148502694627439702 ) ) ;
#43431=CARTESIAN_POINT ( 'NONE',  ( 2.499999999999998668, -79.20833333060213022, -4.330127018922193649 ) ) ;
#43432=CARTESIAN_POINT ( 'NONE',  ( -2.229367062499996610, -2.145833331967737845, 3.861377020970582219 ) ) ;
#43433=CARTESIAN_POINT ( 'NONE',  ( 2.499999999999998668, -30.20833333060214443, -4.330127018922193649 ) ) ;
#43434=CARTESIAN_POINT ( 'NONE',  ( -1.846868145590734756, -151.1250000013656347, -4.458734124999999437 ) ) ;
#43435=( BOUNDED_CURVE ( )  B_SPLINE_CURVE ( 2, ( #58780, #44948, #14710, #15036, #34328, #39786, #29494, #49766, #34653 ),
 .UNSPECIFIED., .F., .T. ) 
 B_SPLINE_CURVE_WITH_KNOTS ( ( 3, 2, 2, 2, 3 ),
 ( 0.2479166666666666741, 0.2486111111111111160, 0.2500000000000000000, 0.2513888888888888840, 0.2520833333333333259 ),
 .UNSPECIFIED. ) 
 CURVE ( )  GEOMETRIC_REPRESENTATION_ITEM ( )  RATIONAL_B_SPLINE_CURVE ( ( 0.9330127018922194093, 0.9330127018922194093, 1.000000000000000000, 0.8660254037844387076, 1.000000000000000000, 0.8660254037844387076, 1.000000000000000000, 0.9330127018922194093, 0.9330127018922194093 ) ) 
 REPRESENTATION_ITEM ( '' )  );
#43446=DIRECTION ( 'NONE',  ( -0.000000000000000000, 1.000000000000000000, -0.000000000000000000 ) ) ;
#43449=CARTESIAN_POINT ( 'NONE',  ( 4.458734124999998549, 17.27083333469892779, -2.574251347313721627 ) ) ;
#43451=CARTESIAN_POINT ( 'NONE',  ( 2.229367062499998831, -7.895833331967735624, -3.861377020970580887 ) ) ;
#43452=CARTESIAN_POINT ( 'NONE',  ( -6.972266317189433020E-16, -34.12499999726881583, -5.000000000000000000 ) ) ;
#43454=CARTESIAN_POINT ( 'NONE',  ( -8.190561711645485556E-16, -167.6875000013655779, 4.458734124999999437 ) ) ;
#43455=CARTESIAN_POINT ( 'NONE',  ( -2.500000000000000444, -21.04166666393548013, -4.330127018922193649 ) ) ;
#43460=CARTESIAN_POINT ( 'NONE',  ( 0.000000000000000000, -170.0000000000000000, 5.000000000000000000 ) ) ;
#43462=CARTESIAN_POINT ( 'NONE',  ( 1.846868145590735200, -152.5000000013656347, -4.458734124999999437 ) ) ;
#43465=CARTESIAN_POINT ( 'NONE',  ( 3.535533905932736864, -163.1250000000000284, 3.535533905932738641 ) ) ;
#43470=CYLINDRICAL_SURFACE ( 'NONE', #20623, 5.000000000000000000 ) ;
#43471=CARTESIAN_POINT ( 'NONE',  ( 5.000000000000000000, 0.5833333333333314830, -2.886751345948129988 ) ) ;
#43473=CARTESIAN_POINT ( 'NONE',  ( 4.458734125000000326, -59.89583333196774362, 2.574251347313718519 ) ) ;
#43475=CARTESIAN_POINT ( 'NONE',  ( -1.339745962155613812, 19.79465819873851729, -5.000000000000000000 ) ) ;
#43476=CARTESIAN_POINT ( 'NONE',  ( 5.000000000000000000, -2.291666663935477466, -2.886751345948129988 ) ) ;
#43477=CARTESIAN_POINT ( 'NONE',  ( 9.457646018065525792E-16, -27.06249999863440081, 5.148502694627439702 ) ) ;
#43479=FACE_OUTER_BOUND ( 'NONE', #37436, .T. ) ;
#43480=CARTESIAN_POINT ( 'NONE',  ( 1.339745962155612702, 5.705341801261479162, -5.000000000000000000 ) ) ;
#43481=CARTESIAN_POINT ( 'NONE',  ( -5.000000000000000000, -44.08333333333334281, -2.886751345948128211 ) ) ;
#43484=DIRECTION ( 'NONE',  ( -0.000000000000000000, 1.000000000000000000, -0.000000000000000000 ) ) ;
#43485=CARTESIAN_POINT ( 'NONE',  ( -4.458734124999998549, -71.22916666530106511, 2.574251347313722516 ) ) ;
#43486=CARTESIAN_POINT ( 'NONE',  ( -1.846868145590734756, -145.3750000013656347, -4.458734125000000326 ) ) ;
#43487=CARTESIAN_POINT ( 'NONE',  ( 2.229367062500001939, -74.97916666530106511, 3.861377020970579999 ) ) ;
#43489=CARTESIAN_POINT ( 'NONE',  ( -3.152548672688508926E-16, -24.81249999863440436, -5.148502694627439702 ) ) ;
#43490=CARTESIAN_POINT ( 'NONE',  ( 5.000000000000000888, -66.45833333060214443, 2.886751345948126879 ) ) ;
#43495=CARTESIAN_POINT ( 'NONE',  ( 2.071067811865518582, -166.1875000000000000, 4.999999999999957367 ) ) ;
#43498=CARTESIAN_POINT ( 'NONE',  ( -4.999999999999998224, -82.91666666666667140, 2.886751345948131764 ) ) ;
#43499=CARTESIAN_POINT ( 'NONE',  ( -3.152548672688508926E-16, -60.81249999863440081, -5.148502694627439702 ) ) ;
#43501=ORIENTED_EDGE ( 'NONE', *, *, #3851, .F. ) ;
#43502=CARTESIAN_POINT ( 'NONE',  ( 5.000000000000000888, -141.9375000000000284, -2.071067811865475505 ) ) ;
#43503=CARTESIAN_POINT ( 'NONE',  ( -4.458734124999999437, 16.60416666803225993, -2.574251347313719407 ) ) ;
#43506=CARTESIAN_POINT ( 'NONE',  ( 4.458734124999997661, -164.5000000013655779, 1.846868145590737864 ) ) ;
#43509=CARTESIAN_POINT ( 'NONE',  ( 5.000000000000000000, -39.49999999999999289, -6.123233995736766282E-16 ) ) ;
#43511=AXIS2_PLACEMENT_3D ( 'NONE', #3205, #55966, #41785 ) ;
#43522=CARTESIAN_POINT ( 'NONE',  ( -4.458734124999997661, 9.520833334698927786, 2.574251347313722516 ) ) ;
#43523=CARTESIAN_POINT ( 'NONE',  ( 1.975475456537005874E-15, 11.24999999999999822, 5.000000000000000000 ) ) ;
#43525=CARTESIAN_POINT ( 'NONE',  ( -3.535533905932737309, -149.7500000027312126, -3.535533905932738197 ) ) ;
#43530=( BOUNDED_CURVE ( )  B_SPLINE_CURVE ( 2, ( #10799, #54222, #25598, #21093, #41018, #26229, #5661, #30738, #10473 ),
 .UNSPECIFIED., .F., .F. ) 
 B_SPLINE_CURVE_WITH_KNOTS ( ( 3, 2, 2, 2, 3 ),
 ( 0.8770833333333333259, 0.8777777777777777679, 0.8791666666666666519, 0.8805555555555555358, 0.8812499999999999778 ),
 .UNSPECIFIED. ) 
 CURVE ( )  GEOMETRIC_REPRESENTATION_ITEM ( )  RATIONAL_B_SPLINE_CURVE ( ( 0.9330127018922194093, 0.9330127018922194093, 1.000000000000000000, 0.8660254037844387076, 1.000000000000000000, 0.8660254037844387076, 1.000000000000000000, 0.9330127018922194093, 0.9330127018922194093 ) ) 
 REPRESENTATION_ITEM ( '' )  );
#43531=CARTESIAN_POINT ( 'NONE',  ( -2.071067811865478170, -144.3125000000000284, 5.000000000000000000 ) ) ;
#43534=CARTESIAN_POINT ( 'NONE',  ( 2.229367062499998831, -30.64583333196773651, -3.861377020970580887 ) ) ;
#43535=DIRECTION ( 'NONE',  ( -0.000000000000000000, 1.000000000000000000, -0.000000000000000000 ) ) ;
#43538=CARTESIAN_POINT ( 'NONE',  ( 3.152801135295367541, -143.3125000013655779, -3.152801135295367541 ) ) ;
#43540=CARTESIAN_POINT ( 'NONE',  ( 2.229367062499998831, 28.10416666803225993, -3.861377020970580887 ) ) ;
#43542=CARTESIAN_POINT ( 'NONE',  ( 2.229367062499998831, -55.89583333196773651, -3.861377020970580887 ) ) ;
#43544=CARTESIAN_POINT ( 'NONE',  ( 2.499999999999998668, 13.79166666939785202, -4.330127018922193649 ) ) ;
#43545=CARTESIAN_POINT ( 'NONE',  ( 2.500000000000002220, 17.33333333333333215, 4.330127018922192761 ) ) ;
#43547=CARTESIAN_POINT ( 'NONE',  ( -1.339745962155610925, -36.66965819600732601, 5.000000000000000000 ) ) ;
#43548=CARTESIAN_POINT ( 'NONE',  ( 2.229367062499998831, -7.645833331967735624, -3.861377020970580887 ) ) ;
#43549=CARTESIAN_POINT ( 'NONE',  ( -5.000000000000000000, -23.00000000000000000, 0.000000000000000000 ) ) ;
#43551=CARTESIAN_POINT ( 'NONE',  ( 3.061616997868383141E-16, -157.8750000027311842, -5.000000000000000000 ) ) ;
#43554=CARTESIAN_POINT ( 'NONE',  ( -2.229367062499996610, -53.14583333196773651, 3.861377020970582219 ) ) ;
#43555=CARTESIAN_POINT ( 'NONE',  ( 1.846868145590735200, -159.5000000013655779, -4.458734125000000326 ) ) ;
#43556=ADVANCED_FACE ( 'NONE', ( #47061 ), #51265, .T. ) ;
#43557=CARTESIAN_POINT ( 'NONE',  ( -5.000000000000000000, -52.87499999726881583, 0.000000000000000000 ) ) ;
#43558=ORIENTED_EDGE ( 'NONE', *, *, #5165, .F. ) ;
#43559=CARTESIAN_POINT ( 'NONE',  ( 4.458734124999999437, 6.937500001365594748, -5.460374474430324690E-16 ) ) ;
#43560=ADVANCED_FACE ( 'NONE', ( #7198 ), #37103, .T. ) ;
#43562=CARTESIAN_POINT ( 'NONE',  ( -9.184850993605147944E-16, -143.3750000027312126, 5.000000000000000000 ) ) ;
#43563=CARTESIAN_POINT ( 'NONE',  ( 3.152801135295366208, -158.5625000013656063, 3.152801135295367985 ) ) ;
#43568=CARTESIAN_POINT ( 'NONE',  ( -3.152548672688508926E-16, -40.81249999863440081, -5.148502694627439702 ) ) ;
#43571=CARTESIAN_POINT ( 'NONE',  ( 2.071067811865392461, -143.3125000027312410, 5.000000000000084377 ) ) ;
#43573=CARTESIAN_POINT ( 'NONE',  ( 0.000000000000000000, -170.0000000000000000, 5.000000000000000000 ) ) ;
#43574=( BOUNDED_CURVE ( )  B_SPLINE_CURVE ( 2, ( #54433, #40895, #40269, #45735, #59583, #40580, #15185, #10675, #15517 ),
 .UNSPECIFIED., .F., .F. ) 
 B_SPLINE_CURVE_WITH_KNOTS ( ( 3, 2, 2, 2, 3 ),
 ( 0.4270833333333333148, 0.4277777777777777568, 0.4291666666666666408, 0.4305555555555555802, 0.4312500000000000222 ),
 .UNSPECIFIED. ) 
 CURVE ( )  GEOMETRIC_REPRESENTATION_ITEM ( )  RATIONAL_B_SPLINE_CURVE ( ( 0.9330127018922194093, 0.9330127018922194093, 1.000000000000000000, 0.8660254037844387076, 1.000000000000000000, 0.8660254037844387076, 1.000000000000000000, 0.9330127018922194093, 0.9330127018922194093 ) ) 
 REPRESENTATION_ITEM ( '' )  );
#43575=VERTEX_POINT ( 'NONE', #61195 ) ;
#43576=CARTESIAN_POINT ( 'NONE',  ( -4.458734124999998549, -87.47916666530107932, 2.574251347313722516 ) ) ;
#43583=DIRECTION ( 'NONE',  ( -0.000000000000000000, 1.000000000000000000, -0.000000000000000000 ) ) ;
#43585=CARTESIAN_POINT ( 'NONE',  ( -9.184850993605147944E-16, -149.2500000000000284, 5.000000000000000000 ) ) ;
#43586=CARTESIAN_POINT ( 'NONE',  ( 6.123233995736766282E-16, -170.0000000000000000, -5.000000000000000000 ) ) ;
#43588=EDGE_CURVE ( 'NONE', #9066, #17838, #17117, .T. ) ;
#43592=CARTESIAN_POINT ( 'NONE',  ( 9.457646018065525792E-16, -84.31249999863437949, 5.148502694627439702 ) ) ;
#43595=CARTESIAN_POINT ( 'NONE',  ( -5.000000000000000000, 18.12500000273118417, 0.000000000000000000 ) ) ;
#43597=CARTESIAN_POINT ( 'NONE',  ( -5.000000000000000888, -160.5625000027312126, 2.071067811865474617 ) ) ;
#43605=( BOUNDED_CURVE ( )  B_SPLINE_CURVE ( 2, ( #8529, #47447, #57119, #42301, #38417, #57741, #17558, #42618, #32654 ),
 .UNSPECIFIED., .F., .F. ) 
 B_SPLINE_CURVE_WITH_KNOTS ( ( 3, 2, 2, 2, 3 ),
 ( 0.3395833333333333481, 0.3402777777777777901, 0.3416666666666666741, 0.3430555555555555580, 0.3437500000000000000 ),
 .UNSPECIFIED. ) 
 CURVE ( )  GEOMETRIC_REPRESENTATION_ITEM ( )  RATIONAL_B_SPLINE_CURVE ( ( 0.9330127018922194093, 0.9330127018922194093, 1.000000000000000000, 0.8660254037844387076, 1.000000000000000000, 0.8660254037844387076, 1.000000000000000000, 0.9330127018922194093, 0.9330127018922194093 ) ) 
 REPRESENTATION_ITEM ( '' )  );
#43608=CARTESIAN_POINT ( 'NONE',  ( 2.229367062499998831, -15.64583333196773651, -3.861377020970580887 ) ) ;
#43610=CARTESIAN_POINT ( 'NONE',  ( 3.535533905932736864, -155.1250000000000000, 3.535533905932738641 ) ) ;
#43612=CARTESIAN_POINT ( 'NONE',  ( -4.458734124999997661, -40.47916666530107221, 2.574251347313722516 ) ) ;
#43613=CARTESIAN_POINT ( 'NONE',  ( 1.339745962155612702, -83.16965819600733312, -5.000000000000000000 ) ) ;
#43614=CARTESIAN_POINT ( 'NONE',  ( 1.062108568985190270E-13, -12.25000000000000000, -4.999999999999999112 ) ) ;
#43619=CARTESIAN_POINT ( 'NONE',  ( -4.458734124999999437, 11.68750000136559564, 0.000000000000000000 ) ) ;
#43623=CARTESIAN_POINT ( 'NONE',  ( -3.152548672688508926E-16, -87.81249999863437949, -5.148502694627439702 ) ) ;
#43625=CARTESIAN_POINT ( 'NONE',  ( -5.000000000000000000, 15.12500000273118417, 0.000000000000000000 ) ) ;
#43626=VERTEX_POINT ( 'NONE', #23206 ) ;
#43628=EDGE_LOOP ( 'NONE', ( #34466, #43254, #16068, #26768 ) ) ;
#43630=( BOUNDED_CURVE ( )  B_SPLINE_CURVE ( 2, ( #41881, #47353, #22924, #37081, #23543, #61846, #47660, #17458, #3613 ),
 .UNSPECIFIED., .F., .F. ) 
 B_SPLINE_CURVE_WITH_KNOTS ( ( 3, 2, 2, 2, 3 ),
 ( 0.6812500000000000222, 0.6819444444444444642, 0.6833333333333333481, 0.6847222222222222321, 0.6854166666666666741 ),
 .UNSPECIFIED. ) 
 CURVE ( )  GEOMETRIC_REPRESENTATION_ITEM ( )  RATIONAL_B_SPLINE_CURVE ( ( 0.9330127018922194093, 0.9330127018922194093, 1.000000000000000000, 0.8660254037844387076, 1.000000000000000000, 0.8660254037844387076, 1.000000000000000000, 0.9330127018922194093, 0.9330127018922194093 ) ) 
 REPRESENTATION_ITEM ( '' )  );
#43632=CARTESIAN_POINT ( 'NONE',  ( -5.000000000000000000, -36.08333333333332860, -2.886751345948128211 ) ) ;
#43633=CARTESIAN_POINT ( 'NONE',  ( 2.229367062499998831, -38.64583333196773651, -3.861377020970580887 ) ) ;
#43634=CARTESIAN_POINT ( 'NONE',  ( 1.060575238724906964E-15, -34.62499999726880873, 5.773502691896257311 ) ) ;
#43635=CARTESIAN_POINT ( 'NONE',  ( 4.458734125000001214, -65.89583333196772230, 2.574251347313718519 ) ) ;
#43638=CARTESIAN_POINT ( 'NONE',  ( 4.458734124999998549, -13.72916666530107399, -2.574251347313721627 ) ) ;
#43640=CARTESIAN_POINT ( 'NONE',  ( -4.458734124999998549, -15.47916666530107399, 2.574251347313722516 ) ) ;
#43641=ORIENTED_EDGE ( 'NONE', *, *, #50029, .F. ) ;
#43642=CARTESIAN_POINT ( 'NONE',  ( -5.000000000000000000, -75.00000000000000000, 0.000000000000000000 ) ) ;
#43645=CARTESIAN_POINT ( 'NONE',  ( 5.000000000000000000, -84.37499999726880162, -6.123233995736766282E-16 ) ) ;
#43649=CARTESIAN_POINT ( 'NONE',  ( 2.229367062499998831, -22.89583333196773651, -3.861377020970580887 ) ) ;
#43650=ORIENTED_EDGE ( 'NONE', *, *, #50396, .T. ) ;
#43651=CARTESIAN_POINT ( 'NONE',  ( 1.846868145590735200, -168.5000000013656063, -4.458734125000000326 ) ) ;
#43653=CARTESIAN_POINT ( 'NONE',  ( 2.500000000000002220, -8.541666663935483683, 4.330127018922192761 ) ) ;
#43654=ORIENTED_EDGE ( 'NONE', *, *, #11348, .F. ) ;
#43663=CARTESIAN_POINT ( 'NONE',  ( -4.458734124999999437, -144.1875000013656063, -5.460374474430324690E-16 ) ) ;
#43665=CARTESIAN_POINT ( 'NONE',  ( 5.000000000000000888, -70.58333333333332860, 2.886751345948126879 ) ) ;
#43667=CARTESIAN_POINT ( 'NONE',  ( 9.457646018065525792E-16, -68.31249999863442213, 5.148502694627439702 ) ) ;
#43669=CARTESIAN_POINT ( 'NONE',  ( -5.000000000000000000, -0.9583333306021485365, -2.886751345948128211 ) ) ;
#43670=CARTESIAN_POINT ( 'NONE',  ( 1.846868145590735200, -140.2500000013656063, -4.458734124999999437 ) ) ;
#43673=CARTESIAN_POINT ( 'NONE',  ( -6.972266317189433020E-16, -50.12499999726881583, -5.000000000000000000 ) ) ;
#43679=CARTESIAN_POINT ( 'NONE',  ( -4.458734124999999437, 20.43750000136559208, 0.000000000000000000 ) ) ;
#43680=DIRECTION ( 'NONE',  ( -0.000000000000000000, 1.000000000000000000, -0.000000000000000000 ) ) ;
#43686=CARTESIAN_POINT ( 'NONE',  ( 9.457646018065525792E-16, 2.937500001365594304, 5.148502694627439702 ) ) ;
#43688=CARTESIAN_POINT ( 'NONE',  ( -4.458734124999997661, -27.47916666530107221, 2.574251347313722516 ) ) ;
#43689=CARTESIAN_POINT ( 'NONE',  ( -1.846868145590737420, -156.7500000013656063, 4.458734124999999437 ) ) ;
#43692=CARTESIAN_POINT ( 'NONE',  ( 4.458734124999998549, 23.27083333469892423, -2.574251347313721627 ) ) ;
#43693=ADVANCED_FACE ( 'NONE', ( #22907 ), #62139, .T. ) ;
#43694=CARTESIAN_POINT ( 'NONE',  ( -6.972266317189433020E-16, -84.24999999999998579, -5.000000000000000000 ) ) ;
#43696=CARTESIAN_POINT ( 'NONE',  ( -2.229367062499996610, -72.39583333196773651, 3.861377020970582219 ) ) ;
#43698=EDGE_CURVE ( 'NONE', #17322, #16392, #40527, .T. ) ;
#43699=CARTESIAN_POINT ( 'NONE',  ( 5.000000000000000000, 28.62500000273118417, -6.123233995736766282E-16 ) ) ;
#43700=EDGE_LOOP ( 'NONE', ( #31389, #58486, #10899, #45397 ) ) ;
#43701=DIRECTION ( 'NONE',  ( 0.000000000000000000, -1.000000000000000000, 0.000000000000000000 ) ) ;
#43703=CARTESIAN_POINT ( 'NONE',  ( -5.000000000000000000, 12.04166666939785202, -2.886751345948128211 ) ) ;
#43704=CARTESIAN_POINT ( 'NONE',  ( 5.000000000000000888, -15.58333333333333215, 2.886751345948126879 ) ) ;
#43705=CARTESIAN_POINT ( 'NONE',  ( -2.229367062500000163, -17.47916666530106866, -3.861377020970580443 ) ) ;
#43707=CARTESIAN_POINT ( 'NONE',  ( -4.458734124999999437, -84.31249999863439371, 0.000000000000000000 ) ) ;
#43709=( BOUNDED_CURVE ( )  B_SPLINE_CURVE ( 2, ( #5293, #59323, #22001, #55782, #51593, #17168, #36794, #7529, #27141 ),
 .UNSPECIFIED., .F., .F. ) 
 B_SPLINE_CURVE_WITH_KNOTS ( ( 3, 2, 2, 2, 3 ),
 ( 0.6562500000000000000, 0.6569444444444444420, 0.6583333333333333259, 0.6597222222222222099, 0.6604166666666666519 ),
 .UNSPECIFIED. ) 
 CURVE ( )  GEOMETRIC_REPRESENTATION_ITEM ( )  RATIONAL_B_SPLINE_CURVE ( ( 0.9330127018922194093, 0.9330127018922194093, 1.000000000000000000, 0.8660254037844387076, 1.000000000000000000, 0.8660254037844387076, 1.000000000000000000, 0.9330127018922194093, 0.9330127018922194093 ) ) 
 REPRESENTATION_ITEM ( '' )  );
#43710=CARTESIAN_POINT ( 'NONE',  ( 4.458734125000000326, -167.6250000013655779, -1.846868145590734978 ) ) ;
#43711=CARTESIAN_POINT ( 'NONE',  ( 5.000000000000000000, -17.29166666393548368, -2.886751345948129988 ) ) ;
#43712=CARTESIAN_POINT ( 'NONE',  ( -3.152548672688508926E-16, -50.56249999863440792, -5.148502694627439702 ) ) ;
#43714=CARTESIAN_POINT ( 'NONE',  ( 6.123233995736766282E-16, -170.0000000000000000, -5.000000000000000000 ) ) ;
#43715=CARTESIAN_POINT ( 'NONE',  ( -2.229367062500000163, 4.270833334698926897, -3.861377020970580443 ) ) ;
#43716=VERTEX_POINT ( 'NONE', #12606 ) ;
#43717=CARTESIAN_POINT ( 'NONE',  ( -2.499999999999996447, -86.70833333060214443, 4.330127018922195425 ) ) ;
#43718=CARTESIAN_POINT ( 'NONE',  ( 5.000000000000000000, -60.41666666666666430, -2.886751345948129988 ) ) ;
#43719=EDGE_CURVE ( 'NONE', #42072, #61537, #18058, .T. ) ;
#43720=CARTESIAN_POINT ( 'NONE',  ( -1.846868145590734756, -156.3750000013655779, -4.458734125000000326 ) ) ;
#43722=CARTESIAN_POINT ( 'NONE',  ( -1.339745962155613812, -56.20534180126148271, -5.000000000000000000 ) ) ;
#43723=CARTESIAN_POINT ( 'NONE',  ( -9.184850993605147944E-16, -162.2500000000000000, 5.000000000000000000 ) ) ;
#43724=ADVANCED_FACE ( 'NONE', ( #32537 ), #57322, .T. ) ;
#43727=CARTESIAN_POINT ( 'NONE',  ( -4.458734124999998549, -5.479166665301072214, 2.574251347313722516 ) ) ;
#43728=CARTESIAN_POINT ( 'NONE',  ( -4.458734124999999437, -44.56249999863440081, 0.000000000000000000 ) ) ;
#43730=ADVANCED_FACE ( 'NONE', ( #2975 ), #17753, .T. ) ;
#43731=CARTESIAN_POINT ( 'NONE',  ( 1.975475456537005874E-15, -67.62499999726881583, 5.000000000000000000 ) ) ;
#43732=CARTESIAN_POINT ( 'NONE',  ( 4.458734125000000326, -150.3750000013655779, -1.846868145590734978 ) ) ;
#43737=CARTESIAN_POINT ( 'NONE',  ( -2.229367062500000163, 29.27083333469892779, -3.861377020970580443 ) ) ;
#43744=CARTESIAN_POINT ( 'NONE',  ( -2.229367062499996610, -3.145833331967738733, 3.861377020970582219 ) ) ;
#43746=CARTESIAN_POINT ( 'NONE',  ( 1.846868145590735200, -152.2500000013656063, -4.458734124999999437 ) ) ;
#43748=VERTEX_POINT ( 'NONE', #14801 ) ;
#43750=CARTESIAN_POINT ( 'NONE',  ( -2.071067811865306307, -148.6875000000000000, -5.000000000000171418 ) ) ;
#43753=DIRECTION ( 'NONE',  ( -0.000000000000000000, 1.000000000000000000, -0.000000000000000000 ) ) ;
#43760=ORIENTED_EDGE ( 'NONE', *, *, #4629, .T. ) ;
#43761=CARTESIAN_POINT ( 'NONE',  ( -2.229367062500000163, 19.52083333469893134, -3.861377020970580443 ) ) ;
#43763=CARTESIAN_POINT ( 'NONE',  ( 4.458734124999999437, -10.06249999863440614, -5.460374474430324690E-16 ) ) ;
#43764=CARTESIAN_POINT ( 'NONE',  ( -2.499999999999996447, -30.83333333333333215, 4.330127018922195425 ) ) ;
#43766=CARTESIAN_POINT ( 'NONE',  ( -4.458734124999999437, -165.9375000013655779, -5.460374474430324690E-16 ) ) ;
#43774=CARTESIAN_POINT ( 'NONE',  ( -4.458734125000000326, -155.1250000013656063, 1.846868145590734089 ) ) ;
#43776=CARTESIAN_POINT ( 'NONE',  ( 0.000000000000000000, -170.0000000000000000, 0.000000000000000000 ) ) ;
#43781=( BOUNDED_CURVE ( )  B_SPLINE_CURVE ( 2, ( #40776, #31437, #55594, #51398, #22446, #22126, #26626, #2207, #27566 ),
 .UNSPECIFIED., .F., .F. ) 
 B_SPLINE_CURVE_WITH_KNOTS ( ( 3, 2, 2, 2, 3 ),
 ( 0.3729166666666666741, 0.3736111111111111160, 0.3750000000000000000, 0.3763888888888888840, 0.3770833333333333259 ),
 .UNSPECIFIED. ) 
 CURVE ( )  GEOMETRIC_REPRESENTATION_ITEM ( )  RATIONAL_B_SPLINE_CURVE ( ( 0.9330127018922194093, 0.9330127018922194093, 1.000000000000000000, 0.8660254037844387076, 1.000000000000000000, 0.8660254037844387076, 1.000000000000000000, 0.9330127018922194093, 0.9330127018922194093 ) ) 
 REPRESENTATION_ITEM ( '' )  );
#43783=CARTESIAN_POINT ( 'NONE',  ( -2.500000000000000444, 0.8333333333333317050, -4.330127018922193649 ) ) ;
#43785=CARTESIAN_POINT ( 'NONE',  ( 4.458734124999998549, -62.72916666530106511, -2.574251347313721627 ) ) ;
#43786=CARTESIAN_POINT ( 'NONE',  ( -5.000000000000000000, -30.95833333060214443, -2.886751345948128211 ) ) ;
#43787=CARTESIAN_POINT ( 'NONE',  ( 2.499999999999998668, -2.208333330602146205, -4.330127018922193649 ) ) ;
#43788=CARTESIAN_POINT ( 'NONE',  ( 2.229367062499998831, -26.64583333196774007, -3.861377020970580887 ) ) ;
#43790=CARTESIAN_POINT ( 'NONE',  ( 2.500000000000002220, 17.45833333606451987, 4.330127018922192761 ) ) ;
#43791=CARTESIAN_POINT ( 'NONE',  ( 5.000000000000000000, -157.0625000000000284, 2.071067811865478614 ) ) ;
#43793=CARTESIAN_POINT ( 'NONE',  ( -2.500000000000000444, -45.16666666666665719, -4.330127018922193649 ) ) ;
#43796=CARTESIAN_POINT ( 'NONE',  ( 5.000000000000000888, -4.458333330602147981, 2.886751345948126879 ) ) ;
#43797=CARTESIAN_POINT ( 'NONE',  ( -2.229367062499996610, -71.14583333196773651, 3.861377020970582219 ) ) ;
#43798=CARTESIAN_POINT ( 'NONE',  ( -1.846868145590734756, -144.3750000013656063, -4.458734125000000326 ) ) ;
#43799=CARTESIAN_POINT ( 'NONE',  ( 9.457646018065525792E-16, -79.06249999863440792, 5.148502694627439702 ) ) ;
#43801=CARTESIAN_POINT ( 'NONE',  ( -4.458734124999998549, -28.47916666530107221, 2.574251347313722516 ) ) ;
#43802=CARTESIAN_POINT ( 'NONE',  ( -3.535250795749689387E-16, -67.12499999726881583, -5.773502691896257311 ) ) ;
#43803=EDGE_CURVE ( 'NONE', #52130, #10973, #24150, .T. ) ;
#43804=EDGE_LOOP ( 'NONE', ( #11837, #14377, #18375, #11356 ) ) ;
#43805=CARTESIAN_POINT ( 'NONE',  ( -9.184850993605147944E-16, -152.3750000027311842, 5.000000000000000000 ) ) ;
#43809=ORIENTED_EDGE ( 'NONE', *, *, #33015, .F. ) ;
#43810=CARTESIAN_POINT ( 'NONE',  ( 5.000000000000000000, 27.58333333333333215, -2.886751345948130876 ) ) ;
#43813=CARTESIAN_POINT ( 'NONE',  ( -4.458734124999998549, -61.47916666530107221, 2.574251347313722516 ) ) ;
#43815=VERTEX_POINT ( 'NONE', #13861 ) ;
#43818=CARTESIAN_POINT ( 'NONE',  ( -4.458734124999999437, 10.60416666803225993, -2.574251347313719407 ) ) ;
#43821=CARTESIAN_POINT ( 'NONE',  ( 4.458734124999997661, -165.5000000013655779, 1.846868145590737864 ) ) ;
#43823=VERTEX_POINT ( 'NONE', #34414 ) ;
#43827=CARTESIAN_POINT ( 'NONE',  ( 3.061616997868383141E-16, -162.8750000027311842, -5.000000000000000000 ) ) ;
#43830=CARTESIAN_POINT ( 'NONE',  ( 1.975475456537005874E-15, -20.74999999999999645, 5.000000000000000000 ) ) ;
#43831=DIRECTION ( 'NONE',  ( -0.000000000000000000, 1.000000000000000000, -0.000000000000000000 ) ) ;
#43832=CARTESIAN_POINT ( 'NONE',  ( 5.000000000000000000, -58.41666666666665719, -2.886751345948130876 ) ) ;
#43835=CARTESIAN_POINT ( 'NONE',  ( -4.458734124999999437, 7.437500001365594748, 0.000000000000000000 ) ) ;
#43838=CARTESIAN_POINT ( 'NONE',  ( 5.000000000000000000, -151.1250000027312126, 0.000000000000000000 ) ) ;
#43843=CARTESIAN_POINT ( 'NONE',  ( 5.000000000000000000, -144.0000000000000284, 0.000000000000000000 ) ) ;
#43845=CARTESIAN_POINT ( 'NONE',  ( 4.458734124999999437, -166.6250000013656063, -1.846868145590734978 ) ) ;
#43846=CARTESIAN_POINT ( 'NONE',  ( 2.229367062500001939, -30.97916666530107221, 3.861377020970579999 ) ) ;
#43848=FACE_OUTER_BOUND ( 'NONE', #58067, .T. ) ;
#43850=CARTESIAN_POINT ( 'NONE',  ( -1.846868145590734756, -144.1250000013655779, -4.458734125000000326 ) ) ;
#43852=CARTESIAN_POINT ( 'NONE',  ( 4.458734124999999437, 25.93750000136559564, -5.460374474430324690E-16 ) ) ;
#43854=CARTESIAN_POINT ( 'NONE',  ( -4.458734124999999437, -57.64583333196773651, -2.574251347313719407 ) ) ;
#43857=CARTESIAN_POINT ( 'NONE',  ( 5.000000000000000000, 18.58333333333333215, -2.886751345948129988 ) ) ;
#43859=CARTESIAN_POINT ( 'NONE',  ( -2.229367062500000163, -6.479166665301072214, -3.861377020970580443 ) ) ;
#43861=CYLINDRICAL_SURFACE ( 'NONE', #61542, 5.000000000000000000 ) ;
#43866=CARTESIAN_POINT ( 'NONE',  ( 2.229367062499998831, -51.64583333196773651, -3.861377020970580887 ) ) ;
#43867=CARTESIAN_POINT ( 'NONE',  ( 2.730187237215162345E-16, -157.4375000013655779, -4.458734124999999437 ) ) ;
#43869=CARTESIAN_POINT ( 'NONE',  ( -3.535250795749689387E-16, -51.12499999726880873, -5.773502691896257311 ) ) ;
#43870=VERTEX_POINT ( 'NONE', #29593 ) ;
#43871=VECTOR ( 'NONE', #25662, 1000.000000000000114 ) ;
#43872=CARTESIAN_POINT ( 'NONE',  ( -4.458734124999999437, 5.437500001365592972, 0.000000000000000000 ) ) ;
#43873=ORIENTED_EDGE ( 'NONE', *, *, #16216, .F. ) ;
#43876=CARTESIAN_POINT ( 'NONE',  ( -1.846868145590737420, -158.7500000013656063, 4.458734124999999437 ) ) ;
#43877=ORIENTED_EDGE ( 'NONE', *, *, #14917, .F. ) ;
#43880=DIRECTION ( 'NONE',  ( 0.000000000000000000, 0.000000000000000000, 1.000000000000000000 ) ) ;
#43881=CARTESIAN_POINT ( 'NONE',  ( 4.458734124999998549, -40.97916666530107932, -2.574251347313721627 ) ) ;
#43883=CARTESIAN_POINT ( 'NONE',  ( -4.999999999999998224, -45.91666666666665719, 2.886751345948131764 ) ) ;
#43887=CARTESIAN_POINT ( 'NONE',  ( 4.458734124999998549, 29.27083333469892423, -2.574251347313721627 ) ) ;
#43891=CARTESIAN_POINT ( 'NONE',  ( 5.000000000000000888, -168.9375000000000284, -2.071067811865475505 ) ) ;
#43901=CARTESIAN_POINT ( 'NONE',  ( -2.499999999999996447, -66.70833333060214443, 4.330127018922195425 ) ) ;
#43902=CARTESIAN_POINT ( 'NONE',  ( 2.229367062499998831, -88.89583333196773651, -3.861377020970580887 ) ) ;
#43906=VECTOR ( 'NONE', #15928, 1000.000000000000000 ) ;
#43907=CARTESIAN_POINT ( 'NONE',  ( -2.500000000000000444, 17.95833333606451632, -4.330127018922193649 ) ) ;
#43909=CARTESIAN_POINT ( 'NONE',  ( -9.184850993605147944E-16, -160.3750000027311842, 5.000000000000000000 ) ) ;
#43911=AXIS2_PLACEMENT_3D ( 'NONE', #33250, #52870, #13631 ) ;
#43912=CARTESIAN_POINT ( 'NONE',  ( -5.000000000000000000, 22.00000000000000000, 0.000000000000000000 ) ) ;
#43914=CARTESIAN_POINT ( 'NONE',  ( 3.061616997868383141E-16, -152.7500000000000000, -5.000000000000000000 ) ) ;
#43921=CARTESIAN_POINT ( 'NONE',  ( -5.000000000000000000, -54.08333333333332860, -2.886751345948128211 ) ) ;
#43922=CARTESIAN_POINT ( 'NONE',  ( -4.458734124999999437, -16.39583333196773651, -2.574251347313719407 ) ) ;
#43923=DIRECTION ( 'NONE',  ( -0.000000000000000000, 1.000000000000000000, -0.000000000000000000 ) ) ;
#43924=CARTESIAN_POINT ( 'NONE',  ( -5.000000000000000888, -153.4375000000000000, 2.071067811865474617 ) ) ;
#43927=CARTESIAN_POINT ( 'NONE',  ( 4.458734124999998549, -40.97916666530106511, -2.574251347313721627 ) ) ;
#43932=VECTOR ( 'NONE', #26430, 1000.000000000000000 ) ;
#43933=CARTESIAN_POINT ( 'NONE',  ( -2.229367062500000163, 8.520833334698926009, -3.861377020970580443 ) ) ;
#43935=CARTESIAN_POINT ( 'NONE',  ( -6.972266317189433020E-16, -69.24999999999998579, -5.000000000000000000 ) ) ;
#43936=CARTESIAN_POINT ( 'NONE',  ( -4.458734124999999437, -86.56249999863439371, 0.000000000000000000 ) ) ;
#43937=CARTESIAN_POINT ( 'NONE',  ( -4.458734124999999437, 20.43750000136559208, 0.000000000000000000 ) ) ;
#43939=CARTESIAN_POINT ( 'NONE',  ( -5.000000000000000000, 13.12500000273118417, 0.000000000000000000 ) ) ;
#43942=ORIENTED_EDGE ( 'NONE', *, *, #41414, .T. ) ;
#43943=DIRECTION ( 'NONE',  ( 0.000000000000000000, 0.000000000000000000, 1.000000000000000000 ) ) ;
#43944=CARTESIAN_POINT ( 'NONE',  ( 5.000000000000000000, -33.41666666666666430, -2.886751345948129988 ) ) ;
#43945=CARTESIAN_POINT ( 'NONE',  ( 2.229367062499998831, -36.64583333196773651, -3.861377020970580887 ) ) ;
#43946=CARTESIAN_POINT ( 'NONE',  ( 2.500000000000002220, -32.54166666393547303, 4.330127018922192761 ) ) ;
#43947=CARTESIAN_POINT ( 'NONE',  ( -3.152548672688508926E-16, -65.56249999863440792, -5.148502694627439702 ) ) ;
#43950=CARTESIAN_POINT ( 'NONE',  ( 2.229367062500001939, -14.97916666530107399, 3.861377020970579999 ) ) ;
#43951=CARTESIAN_POINT ( 'NONE',  ( -2.229367062500000163, -14.72916666530107221, -3.861377020970580443 ) ) ;
#43952=ORIENTED_EDGE ( 'NONE', *, *, #54346, .F. ) ;
#43953=CARTESIAN_POINT ( 'NONE',  ( 1.060575238724906964E-15, -79.74999999999998579, 5.773502691896257311 ) ) ;
#43957=CARTESIAN_POINT ( 'NONE',  ( -4.999999999999999112, -84.79166666393547303, 2.886751345948131764 ) ) ;
#43958=DIRECTION ( 'NONE',  ( -0.000000000000000000, 1.000000000000000000, -0.000000000000000000 ) ) ;
#43962=CARTESIAN_POINT ( 'NONE',  ( -3.152548672688508926E-16, -28.81249999863440436, -5.148502694627439702 ) ) ;
#43965=CARTESIAN_POINT ( 'NONE',  ( -4.458734125000000326, -165.2500000013655779, -1.846868145590735644 ) ) ;
#43972=CARTESIAN_POINT ( 'NONE',  ( -4.458734124999999437, -146.1875000013656063, -5.460374474430324690E-16 ) ) ;
#43973=CARTESIAN_POINT ( 'NONE',  ( -1.339745962155613812, 22.79465819873851729, -5.000000000000000000 ) ) ;
#43979=CARTESIAN_POINT ( 'NONE',  ( 4.458734125000000326, -145.6250000013655779, -1.846868145590734978 ) ) ;
#43983=CARTESIAN_POINT ( 'NONE',  ( 4.458734125000001214, -67.14583333196773651, 2.574251347313718519 ) ) ;
#43985=CARTESIAN_POINT ( 'NONE',  ( 0.000000000000000000, -170.0000000000000000, 0.000000000000000000 ) ) ;
#43986=CARTESIAN_POINT ( 'NONE',  ( 1.846868145590736310, -139.6250000013656347, 4.458734124999997661 ) ) ;
#43990=CARTESIAN_POINT ( 'NONE',  ( 3.535533905932738197, -159.8750000000000284, -3.535533905932738197 ) ) ;
#43996=CARTESIAN_POINT ( 'NONE',  ( 2.229367062500001939, 23.77083333469892779, 3.861377020970579999 ) ) ;
#43997=CARTESIAN_POINT ( 'NONE',  ( -2.500000000000000444, 26.83333333333333570, -4.330127018922193649 ) ) ;
#44001=EDGE_CURVE ( 'NONE', #11807, #7607, #9709, .T. ) ;
#44003=CARTESIAN_POINT ( 'NONE',  ( 1.339745962155615144, -43.58034179853029144, 4.999999999999999112 ) ) ;
#44004=CARTESIAN_POINT ( 'NONE',  ( 4.458734124999998549, 4.270833334698926897, -2.574251347313721627 ) ) ;
#44005=VERTEX_POINT ( 'NONE', #8729 ) ;
#44006=CARTESIAN_POINT ( 'NONE',  ( -3.152548672688508926E-16, -22.81249999863440436, -5.148502694627439702 ) ) ;
#44007=( BOUNDED_CURVE ( )  B_SPLINE_CURVE ( 2, ( #30549, #61751, #7082, #56922, #52092, #31502, #36660, #13160, #41790 ),
 .UNSPECIFIED., .F., .F. ) 
 B_SPLINE_CURVE_WITH_KNOTS ( ( 3, 2, 2, 2, 3 ),
 ( 0.1416666666666667740, 0.1458333333333334814, 0.1500000000000001332, 0.1541666666666668406, 0.1583333333333334925 ),
 .UNSPECIFIED. ) 
 CURVE ( )  GEOMETRIC_REPRESENTATION_ITEM ( )  RATIONAL_B_SPLINE_CURVE ( ( 0.9999999999999980016, 0.9238795325112887369, 1.000000000000000000, 0.9238795325112867385, 1.000000000000000000, 0.9238795325112867385, 1.000000000000000000, 0.9238795325112837409, 1.000000000000003109 ) ) 
 REPRESENTATION_ITEM ( '' )  );
#44010=CARTESIAN_POINT ( 'NONE',  ( -4.458734124999999437, 27.60416666803226349, -2.574251347313719407 ) ) ;
#44013=CARTESIAN_POINT ( 'NONE',  ( -2.229367062500000163, -74.72916666530106511, -3.861377020970580443 ) ) ;
#44016=DIRECTION ( 'NONE',  ( -0.000000000000000000, 1.000000000000000000, -0.000000000000000000 ) ) ;
#44017=ORIENTED_EDGE ( 'NONE', *, *, #1576, .T. ) ;
#44019=CARTESIAN_POINT ( 'NONE',  ( 1.339745962155615144, -6.580341798530292330, 4.999999999999999112 ) ) ;
#44020=CARTESIAN_POINT ( 'NONE',  ( -3.535250795749689387E-16, -19.24999999999999645, -5.773502691896257311 ) ) ;
#44021=CARTESIAN_POINT ( 'NONE',  ( -4.458734124999998549, -22.22916666530107221, 2.574251347313722516 ) ) ;
#44023=CARTESIAN_POINT ( 'NONE',  ( 2.229367062500001939, -80.97916666530106511, 3.861377020970579999 ) ) ;
#44024=CARTESIAN_POINT ( 'NONE',  ( 4.458734124999999437, -166.6875000013655779, 0.000000000000000000 ) ) ;
#44025=CARTESIAN_POINT ( 'NONE',  ( -3.535250795749689387E-16, -17.12499999726881583, -5.773502691896257311 ) ) ;
#44026=CARTESIAN_POINT ( 'NONE',  ( 4.458734124999998549, -48.72916666530107221, -2.574251347313721627 ) ) ;
#44027=VERTEX_POINT ( 'NONE', #58871 ) ;
#44030=CARTESIAN_POINT ( 'NONE',  ( -2.229367062500000163, -0.7291666653010709931, -3.861377020970580443 ) ) ;
#44033=CARTESIAN_POINT ( 'NONE',  ( 5.000000000000000888, -66.58333333333332860, 2.886751345948126879 ) ) ;
#44034=CARTESIAN_POINT ( 'NONE',  ( 3.152801135295366208, -156.8125000013656063, 3.152801135295367985 ) ) ;
#44037=CARTESIAN_POINT ( 'NONE',  ( -5.000000000000000000, -160.5000000000000000, -6.123233995736766282E-16 ) ) ;
#44040=CARTESIAN_POINT ( 'NONE',  ( 9.457646018065525792E-16, -10.31249999863440614, 5.148502694627439702 ) ) ;
#44041=CARTESIAN_POINT ( 'NONE',  ( 4.458734124999999437, -46.06249999863440081, -5.460374474430324690E-16 ) ) ;
#44043=CARTESIAN_POINT ( 'NONE',  ( -3.152801135295367985, -148.8125000013655779, 3.152801135295367096 ) ) ;
#44045=CARTESIAN_POINT ( 'NONE',  ( 5.000000000000000888, -167.0625000027312126, -2.071067811865475505 ) ) ;
#44048=FACE_OUTER_BOUND ( 'NONE', #5299, .T. ) ;
#44050=CARTESIAN_POINT ( 'NONE',  ( -6.972266317189433020E-16, -29.12499999726880873, -5.000000000000000000 ) ) ;
#44051=VECTOR ( 'NONE', #24604, 1000.000000000000000 ) ;
#44052=ORIENTED_EDGE ( 'NONE', *, *, #25126, .T. ) ;
#44054=EDGE_CURVE ( 'NONE', #29478, #7305, #44068, .T. ) ;
#44059=CARTESIAN_POINT ( 'NONE',  ( -5.000000000000000000, -51.08333333333332860, -2.886751345948128211 ) ) ;
#44060=CARTESIAN_POINT ( 'NONE',  ( -4.458734124999998549, -2.229166665301068662, 2.574251347313722516 ) ) ;
#44061=CARTESIAN_POINT ( 'NONE',  ( -3.152801135295367096, -152.0625000013655779, -3.152801135295367541 ) ) ;
#44066=DIRECTION ( 'NONE',  ( 0.000000000000000000, 0.000000000000000000, 1.000000000000000000 ) ) ;
#44068=LINE ( 'NONE', #23529, #16030 ) ;
#44069=EDGE_CURVE ( 'NONE', #30129, #29621, #51634, .T. ) ;
#44070=CARTESIAN_POINT ( 'NONE',  ( 3.061616997868383141E-16, -156.7500000000000000, -5.000000000000000000 ) ) ;
#44076=EDGE_CURVE ( 'NONE', #26245, #18754, #45038, .T. ) ;
#44077=ORIENTED_EDGE ( 'NONE', *, *, #48740, .F. ) ;
#44078=CARTESIAN_POINT ( 'NONE',  ( -4.458734124999999437, 18.60416666803225993, -2.574251347313719407 ) ) ;
#44081=CARTESIAN_POINT ( 'NONE',  ( -3.152548672688508926E-16, -9.812499998634406140, -5.148502694627439702 ) ) ;
#44083=CARTESIAN_POINT ( 'NONE',  ( 3.152801135295367541, -169.3125000013656063, -3.152801135295367541 ) ) ;
#44089=( BOUNDED_CURVE ( )  B_SPLINE_CURVE ( 2, ( #42649, #4057, #28799, #58072, #18212, #37208, #37835, #33631, #53250 ),
 .UNSPECIFIED., .F., .F. ) 
 B_SPLINE_CURVE_WITH_KNOTS ( ( 3, 2, 2, 2, 3 ),
 ( 0.6145833333333333703, 0.6152777777777778123, 0.6166666666666666963, 0.6180555555555555802, 0.6187500000000000222 ),
 .UNSPECIFIED. ) 
 CURVE ( )  GEOMETRIC_REPRESENTATION_ITEM ( )  RATIONAL_B_SPLINE_CURVE ( ( 0.9330127018922194093, 0.9330127018922194093, 1.000000000000000000, 0.8660254037844387076, 1.000000000000000000, 0.8660254037844387076, 1.000000000000000000, 0.9330127018922194093, 0.9330127018922194093 ) ) 
 REPRESENTATION_ITEM ( '' )  );
#44093=CARTESIAN_POINT ( 'NONE',  ( 3.152801135295367541, -152.5625000013655779, -3.152801135295367541 ) ) ;
#44096=LINE ( 'NONE', #38953, #62318 ) ;
#44097=ORIENTED_EDGE ( 'NONE', *, *, #2353, .T. ) ;
#44100=CARTESIAN_POINT ( 'NONE',  ( -5.000000000000000000, -87.87499999726880162, 0.000000000000000000 ) ) ;
#44101=CARTESIAN_POINT ( 'NONE',  ( -5.000000000000000000, -1.083333333333331927, -2.886751345948128211 ) ) ;
#44102=CARTESIAN_POINT ( 'NONE',  ( 4.458734125000000326, -65.89583333196773651, 2.574251347313718519 ) ) ;
#44104=CARTESIAN_POINT ( 'NONE',  ( -4.999999999999999112, -3.791666663935478798, 2.886751345948131764 ) ) ;
#44105=CARTESIAN_POINT ( 'NONE',  ( -2.229367062500000163, -35.47916666530107221, -3.861377020970580443 ) ) ;
#44106=EDGE_LOOP ( 'NONE', ( #62664, #8631, #14811, #14854 ) ) ;
#44108=CARTESIAN_POINT ( 'NONE',  ( 2.071067811865603403, -157.1875000000000284, 4.999999999999872990 ) ) ;
#44110=CARTESIAN_POINT ( 'NONE',  ( -3.535250795749689387E-16, -44.25000000000000000, -5.773502691896257311 ) ) ;
#44114=CARTESIAN_POINT ( 'NONE',  ( 2.229367062499998831, -68.64583333196773651, -3.861377020970580887 ) ) ;
#44115=CARTESIAN_POINT ( 'NONE',  ( 4.458734124999999437, -145.6875000013656063, 0.000000000000000000 ) ) ;
#44116=CARTESIAN_POINT ( 'NONE',  ( -2.229367062499996610, -82.14583333196773651, 3.861377020970582219 ) ) ;
#44118=CARTESIAN_POINT ( 'NONE',  ( 2.229367062500001939, -28.22916666530107221, 3.861377020970579999 ) ) ;
#44119=CARTESIAN_POINT ( 'NONE',  ( -3.535250795749689387E-16, -71.12499999726880162, -5.773502691896257311 ) ) ;
#44121=CYLINDRICAL_SURFACE ( 'NONE', #14543, 5.000000000000000000 ) ;
#44122=ORIENTED_EDGE ( 'NONE', *, *, #48885, .F. ) ;
#44127=VERTEX_POINT ( 'NONE', #50825 ) ;
#44129=CARTESIAN_POINT ( 'NONE',  ( 1.975475456537005874E-15, -82.74999999999998579, 5.000000000000000000 ) ) ;
#44130=CARTESIAN_POINT ( 'NONE',  ( 9.457646018065525792E-16, -59.31249999863440081, 5.148502694627439702 ) ) ;
#44132=ORIENTED_EDGE ( 'NONE', *, *, #12938, .T. ) ;
#44134=CARTESIAN_POINT ( 'NONE',  ( -1.339745962155610925, -22.66965819600732956, 5.000000000000000000 ) ) ;
#44135=CARTESIAN_POINT ( 'NONE',  ( -3.152548672688508926E-16, 13.43750000136559386, -5.148502694627439702 ) ) ;
#44137=CARTESIAN_POINT ( 'NONE',  ( 2.499999999999998668, -27.20833333060214798, -4.330127018922193649 ) ) ;
#44138=CARTESIAN_POINT ( 'NONE',  ( -1.846868145590734756, -164.1250000013656063, -4.458734124999999437 ) ) ;
#44143=AXIS2_PLACEMENT_3D ( 'NONE', #1355, #15493, #21592 ) ;
#44154=CARTESIAN_POINT ( 'NONE',  ( 2.229367062500001939, 7.770833334698926009, 3.861377020970579999 ) ) ;
#44155=( BOUNDED_CURVE ( )  B_SPLINE_CURVE ( 2, ( #11431, #56469, #2436, #51324, #16897 ),
 .UNSPECIFIED., .F., .F. ) 
 B_SPLINE_CURVE_WITH_KNOTS ( ( 3, 2, 3 ),
 ( 0.9979166666666666741, 0.9986111111111111160, 1.000000000000000000 ),
 .UNSPECIFIED. ) 
 CURVE ( )  GEOMETRIC_REPRESENTATION_ITEM ( )  RATIONAL_B_SPLINE_CURVE ( ( 0.9330127018922194093, 0.9330127018922194093, 1.000000000000000000, 0.8660254037844387076, 1.000000000000000000 ) ) 
 REPRESENTATION_ITEM ( '' )  );
#44159=CARTESIAN_POINT ( 'NONE',  ( -5.000000000000000888, -149.6875000027312126, -2.071067811865475949 ) ) ;
#44163=AXIS2_PLACEMENT_3D ( 'NONE', #44375, #28639, #19302 ) ;
#44165=CARTESIAN_POINT ( 'NONE',  ( 3.061616997868383141E-16, -144.7500000000000284, -5.000000000000000000 ) ) ;
#44166=EDGE_CURVE ( 'NONE', #51005, #44449, #20608, .T. ) ;
#44168=CARTESIAN_POINT ( 'NONE',  ( 4.458734124999997661, -166.7500000013655779, 1.846868145590737864 ) ) ;
#44169=CARTESIAN_POINT ( 'NONE',  ( 9.457646018065525792E-16, -34.06249999863440792, 5.148502694627439702 ) ) ;
#44171=CARTESIAN_POINT ( 'NONE',  ( 0.000000000000000000, -170.0000000000000000, 0.000000000000000000 ) ) ;
#44173=CARTESIAN_POINT ( 'NONE',  ( -4.458734125000000326, -143.0000000013655779, -1.846868145590735644 ) ) ;
#44175=CARTESIAN_POINT ( 'NONE',  ( -5.000000000000000000, -90.87499999726880162, 0.000000000000000000 ) ) ;
#44177=CARTESIAN_POINT ( 'NONE',  ( -4.458734124999999437, -60.64583333196774362, -2.574251347313719407 ) ) ;
#44179=CARTESIAN_POINT ( 'NONE',  ( 2.500000000000002220, 13.45833333606451987, 4.330127018922192761 ) ) ;
#44180=CARTESIAN_POINT ( 'NONE',  ( -2.499999999999996447, 17.16666666666666430, 4.330127018922195425 ) ) ;
#44182=CARTESIAN_POINT ( 'NONE',  ( 9.457646018065525792E-16, -50.06249999863440792, 5.148502694627439702 ) ) ;
#44183=CARTESIAN_POINT ( 'NONE',  ( 4.458734124999999437, -8.812499998634406140, -5.460374474430324690E-16 ) ) ;
#44184=CARTESIAN_POINT ( 'NONE',  ( -2.071067811865491493, -168.6875000000000853, -4.999999999999985789 ) ) ;
#44186=CARTESIAN_POINT ( 'NONE',  ( 1.975475456537005874E-15, -41.74999999999999289, 5.000000000000000000 ) ) ;
#44191=CARTESIAN_POINT ( 'NONE',  ( -4.458734124999999437, 29.56250000136559208, 0.000000000000000000 ) ) ;
#44192=CARTESIAN_POINT ( 'NONE',  ( -2.229367062500000163, -56.47916666530107221, -3.861377020970580443 ) ) ;
#44193=CARTESIAN_POINT ( 'NONE',  ( -4.458734125000001214, -157.1250000013656063, 1.846868145590734089 ) ) ;
#44194=CARTESIAN_POINT ( 'NONE',  ( 2.500000000000002220, -54.54166666393548013, 4.330127018922192761 ) ) ;
#44195=ORIENTED_EDGE ( 'NONE', *, *, #62146, .T. ) ;
#44197=CARTESIAN_POINT ( 'NONE',  ( 9.457646018065525792E-16, 5.687500001365592972, 5.148502694627439702 ) ) ;
#44199=DIRECTION ( 'NONE',  ( -0.000000000000000000, 1.000000000000000000, -0.000000000000000000 ) ) ;
#44201=CARTESIAN_POINT ( 'NONE',  ( -4.458734125000001214, -156.8750000013655779, 1.846868145590734089 ) ) ;
#44202=EDGE_LOOP ( 'NONE', ( #49907, #10426, #30726, #32361 ) ) ;
#44206=CARTESIAN_POINT ( 'NONE',  ( 4.458734124999999437, -45.06249999863440081, -5.460374474430324690E-16 ) ) ;
#44211=ORIENTED_EDGE ( 'NONE', *, *, #43008, .T. ) ;
#44212=CARTESIAN_POINT ( 'NONE',  ( 4.458734124999999437, -89.06249999863439371, -5.460374474430324690E-16 ) ) ;
#44220=CARTESIAN_POINT ( 'NONE',  ( 0.000000000000000000, -170.0000000000000000, 0.000000000000000000 ) ) ;
#44223=DIRECTION ( 'NONE',  ( -0.000000000000000000, 1.000000000000000000, -0.000000000000000000 ) ) ;
#44224=CARTESIAN_POINT ( 'NONE',  ( -4.999999999999998224, -66.79166666393547303, 2.886751345948131764 ) ) ;
#44229=EDGE_LOOP ( 'NONE', ( #36442, #27146, #53000, #25865 ) ) ;
#44230=CARTESIAN_POINT ( 'NONE',  ( -5.000000000000000000, -169.5000000000000000, -6.123233995736766282E-16 ) ) ;
#44232=CARTESIAN_POINT ( 'NONE',  ( -3.535533905932738641, -159.5000000027312126, 3.535533905932737309 ) ) ;
#44235=CARTESIAN_POINT ( 'NONE',  ( 0.000000000000000000, -170.0000000000000000, 5.000000000000000000 ) ) ;
#44244=CARTESIAN_POINT ( 'NONE',  ( -2.229367062500000163, -13.47916666530107221, -3.861377020970580443 ) ) ;
#44246=CARTESIAN_POINT ( 'NONE',  ( -9.184850993605147944E-16, -154.2500000000000000, 5.000000000000000000 ) ) ;
#44249=CARTESIAN_POINT ( 'NONE',  ( -4.458734124999997661, -38.47916666530107221, 2.574251347313722516 ) ) ;
#44252=CARTESIAN_POINT ( 'NONE',  ( -1.127183054612291972E-14, 24.37500000273118417, 4.999999999999999112 ) ) ;
#44255=CARTESIAN_POINT ( 'NONE',  ( -4.458734124999999437, 7.604166668032259935, -2.574251347313719407 ) ) ;
#44257=CARTESIAN_POINT ( 'NONE',  ( -1.339745962155589165, 11.79465819873852084, -5.000000000000014211 ) ) ;
#44259=CARTESIAN_POINT ( 'NONE',  ( -2.229367062499996610, 22.60416666803225993, 3.861377020970582219 ) ) ;
#44261=CARTESIAN_POINT ( 'NONE',  ( 2.500000000000002220, 7.458333336064517205, 4.330127018922192761 ) ) ;
#44262=ORIENTED_EDGE ( 'NONE', *, *, #49227, .T. ) ;
#44266=CARTESIAN_POINT ( 'NONE',  ( 2.500000000000002220, -36.66666666666666430, 4.330127018922192761 ) ) ;
#44267=CARTESIAN_POINT ( 'NONE',  ( 2.229367062499998831, -39.64583333196773651, -3.861377020970580887 ) ) ;
#44268=ADVANCED_FACE ( 'NONE', ( #61440 ), #12220, .T. ) ;
#44269=( BOUNDED_CURVE ( )  B_SPLINE_CURVE ( 2, ( #21793, #47182, #2492, #41388, #22745, #42342, #61981, #55888, #46226 ),
 .UNSPECIFIED., .F., .F. ) 
 B_SPLINE_CURVE_WITH_KNOTS ( ( 3, 2, 2, 2, 3 ),
 ( 0.5083333333333337478, 0.5125000000000003997, 0.5166666666666671626, 0.5208333333333338144, 0.5250000000000004663 ),
 .UNSPECIFIED. ) 
 CURVE ( )  GEOMETRIC_REPRESENTATION_ITEM ( )  RATIONAL_B_SPLINE_CURVE ( ( 0.9999999999999918954, 0.9238795325112948431, 1.000000000000000000, 0.9238795325112867385, 1.000000000000000000, 0.9238795325112867385, 1.000000000000000000, 0.9238795325112786339, 1.000000000000008216 ) ) 
 REPRESENTATION_ITEM ( '' )  );
#44270=CARTESIAN_POINT ( 'NONE',  ( -4.999999999999999112, -34.79166666393547303, 2.886751345948131764 ) ) ;
#44271=CARTESIAN_POINT ( 'NONE',  ( 9.457646018065525792E-16, -68.06249999863440792, 5.148502694627439702 ) ) ;
#44272=ORIENTED_EDGE ( 'NONE', *, *, #6708, .T. ) ;
#44274=CARTESIAN_POINT ( 'NONE',  ( 2.229367062500001939, -13.97916666530107221, 3.861377020970579999 ) ) ;
#44275=CARTESIAN_POINT ( 'NONE',  ( 4.458734124999998549, -15.97916666530107221, -2.574251347313721627 ) ) ;
#44277=CARTESIAN_POINT ( 'NONE',  ( -5.000000000000000000, -82.99999999999998579, 0.000000000000000000 ) ) ;
#44278=CARTESIAN_POINT ( 'NONE',  ( -1.846868145590734756, -167.1250000013656063, -4.458734125000000326 ) ) ;
#44280=CARTESIAN_POINT ( 'NONE',  ( 2.499999999999998668, -83.20833333060214443, -4.330127018922193649 ) ) ;
#44282=ORIENTED_EDGE ( 'NONE', *, *, #44891, .F. ) ;
#44283=VECTOR ( 'NONE', #39285, 1000.000000000000000 ) ;
#44285=CARTESIAN_POINT ( 'NONE',  ( -2.229367062499996610, -29.39583333196774007, 3.861377020970582219 ) ) ;
#44286=ORIENTED_EDGE ( 'NONE', *, *, #45236, .F. ) ;
#44288=CARTESIAN_POINT ( 'NONE',  ( 1.846868145590735200, -166.5000000013655779, -4.458734125000000326 ) ) ;
#44290=CARTESIAN_POINT ( 'NONE',  ( -4.999999999999998224, -38.79166666393548013, 2.886751345948131764 ) ) ;
#44295=CARTESIAN_POINT ( 'NONE',  ( 1.846868145590736310, -147.8750000013655779, 4.458734124999997661 ) ) ;
#44296=LINE ( 'NONE', #259, #13775 ) ;
#44300=CARTESIAN_POINT ( 'NONE',  ( -3.152801135295367096, -141.3125000013655779, -3.152801135295367541 ) ) ;
#44305=CARTESIAN_POINT ( 'NONE',  ( 2.229367062499998831, -74.89583333196773651, -3.861377020970580887 ) ) ;
#44307=CARTESIAN_POINT ( 'NONE',  ( -5.000000000000000000, 29.12500000273118417, 0.000000000000000000 ) ) ;
#44308=CARTESIAN_POINT ( 'NONE',  ( 4.729367062499999719, -139.8437500006828031, 0.000000000000000000 ) ) ;
#44317=CARTESIAN_POINT ( 'NONE',  ( -2.229367062499996610, 16.60416666803225638, 3.861377020970582219 ) ) ;
#44323=CARTESIAN_POINT ( 'NONE',  ( 1.975475456537005874E-15, -80.74999999999998579, 5.000000000000000000 ) ) ;
#44324=CARTESIAN_POINT ( 'NONE',  ( 9.457646018065525792E-16, 3.937500001365595192, 5.148502694627439702 ) ) ;
#44325=VERTEX_POINT ( 'NONE', #7406 ) ;
#44326=CARTESIAN_POINT ( 'NONE',  ( 4.458734125000000326, -26.14583333196773651, 2.574251347313718519 ) ) ;
#44329=CARTESIAN_POINT ( 'NONE',  ( -2.229367062500000163, 27.52083333469892779, -3.861377020970580443 ) ) ;
#44331=CARTESIAN_POINT ( 'NONE',  ( -4.458734124999999437, -73.64583333196773651, -2.574251347313719407 ) ) ;
#44334=CARTESIAN_POINT ( 'NONE',  ( -2.500000000000000444, 27.95833333606451987, -4.330127018922193649 ) ) ;
#44335=VERTEX_POINT ( 'NONE', #17047 ) ;
#44336=CARTESIAN_POINT ( 'NONE',  ( 0.000000000000000000, -170.0000000000000000, 0.000000000000000000 ) ) ;
#44338=CARTESIAN_POINT ( 'NONE',  ( -4.999999999999998224, -56.79166666393547303, 2.886751345948131764 ) ) ;
#44339=CARTESIAN_POINT ( 'NONE',  ( 2.499999999999998668, -18.33333333333333215, -4.330127018922193649 ) ) ;
#44340=CARTESIAN_POINT ( 'NONE',  ( 2.229367062500001939, -19.97916666530107221, 3.861377020970579999 ) ) ;
#44342=CARTESIAN_POINT ( 'NONE',  ( 4.458734124999998549, -83.72916666530106511, -2.574251347313721627 ) ) ;
#44343=CARTESIAN_POINT ( 'NONE',  ( 4.458734124999999437, -167.7500000013655779, 1.846868145590737864 ) ) ;
#44344=CARTESIAN_POINT ( 'NONE',  ( -5.000000000000000000, -19.95833333060214798, -2.886751345948128211 ) ) ;
#44345=CARTESIAN_POINT ( 'NONE',  ( 4.458734125000001214, -47.89583333196775072, 2.574251347313718519 ) ) ;
#44346=ORIENTED_EDGE ( 'NONE', *, *, #55157, .F. ) ;
#44349=CARTESIAN_POINT ( 'NONE',  ( -3.152548672688508926E-16, 4.187500001365595637, -5.148502694627439702 ) ) ;
#44350=VERTEX_POINT ( 'NONE', #42426 ) ;
#44351=CARTESIAN_POINT ( 'NONE',  ( -2.500000000000000444, -87.04166666393547303, -4.330127018922193649 ) ) ;
#44352=CARTESIAN_POINT ( 'NONE',  ( -5.000000000000000000, -64.08333333333332860, -2.886751345948128211 ) ) ;
#44353=CARTESIAN_POINT ( 'NONE',  ( 4.458734124999999437, -157.6875000013655779, 0.000000000000000000 ) ) ;
#44355=CARTESIAN_POINT ( 'NONE',  ( -1.339745962155613812, -77.08034179853029855, -5.000000000000000000 ) ) ;
#44356=CARTESIAN_POINT ( 'NONE',  ( 5.000000000000000000, -162.0000000000000000, 0.000000000000000000 ) ) ;
#44359=CARTESIAN_POINT ( 'NONE',  ( -4.458734124999998549, -9.479166665301070438, 2.574251347313722516 ) ) ;
#44360=CARTESIAN_POINT ( 'NONE',  ( -2.229367062499996610, -44.39583333196774362, 3.861377020970582219 ) ) ;
#44362=CARTESIAN_POINT ( 'NONE',  ( -5.000000000000000000, -7.874999997268813168, 0.000000000000000000 ) ) ;
#44363=CARTESIAN_POINT ( 'NONE',  ( -3.152801135295367096, -150.0625000013655779, -3.152801135295367541 ) ) ;
#44364=EDGE_CURVE ( 'NONE', #15422, #21297, #20433, .T. ) ;
#44369=CARTESIAN_POINT ( 'NONE',  ( -1.339745962155613812, -69.08034179853028434, -5.000000000000000000 ) ) ;
#44371=CARTESIAN_POINT ( 'NONE',  ( -2.500000000000000444, -62.16666666666666430, -4.330127018922193649 ) ) ;
#44372=ORIENTED_EDGE ( 'NONE', *, *, #21656, .F. ) ;
#44375=CARTESIAN_POINT ( 'NONE',  ( 0.000000000000000000, -170.0000000000000000, 0.000000000000000000 ) ) ;
#44378=CARTESIAN_POINT ( 'NONE',  ( -2.229367062499996610, -4.145833331967739177, 3.861377020970582219 ) ) ;
#44380=CARTESIAN_POINT ( 'NONE',  ( -4.458734124999999437, -148.9375000013656063, -5.460374474430324690E-16 ) ) ;
#44381=( BOUNDED_CURVE ( )  B_SPLINE_CURVE ( 2, ( #46112, #12007, #31634, #51271, #21991, #7204, #23251, #62810, #23575 ),
 .UNSPECIFIED., .F., .F. ) 
 B_SPLINE_CURVE_WITH_KNOTS ( ( 3, 2, 2, 2, 3 ),
 ( 0.6229166666666666741, 0.6236111111111111160, 0.6250000000000000000, 0.6263888888888888840, 0.6270833333333333259 ),
 .UNSPECIFIED. ) 
 CURVE ( )  GEOMETRIC_REPRESENTATION_ITEM ( )  RATIONAL_B_SPLINE_CURVE ( ( 0.9330127018922194093, 0.9330127018922194093, 1.000000000000000000, 0.8660254037844387076, 1.000000000000000000, 0.8660254037844387076, 1.000000000000000000, 0.9330127018922194093, 0.9330127018922194093 ) ) 
 REPRESENTATION_ITEM ( '' )  );
#44386=CARTESIAN_POINT ( 'NONE',  ( 0.000000000000000000, -170.0000000000000000, 0.000000000000000000 ) ) ;
#44396=CARTESIAN_POINT ( 'NONE',  ( 0.000000000000000000, -170.0000000000000000, 5.000000000000000000 ) ) ;
#44397=CARTESIAN_POINT ( 'NONE',  ( -4.458734124999999437, 17.68750000136559208, 0.000000000000000000 ) ) ;
#44399=ORIENTED_EDGE ( 'NONE', *, *, #20929, .F. ) ;
#44400=CARTESIAN_POINT ( 'NONE',  ( -4.458734124999999437, -7.645833331967734736, -2.574251347313719407 ) ) ;
#44401=CARTESIAN_POINT ( 'NONE',  ( -1.339745962155613812, -31.20534180126147916, -5.000000000000000000 ) ) ;
#44403=CARTESIAN_POINT ( 'NONE',  ( -2.071067811865478170, -139.4375000027312410, 5.000000000000000000 ) ) ;
#44409=DIRECTION ( 'NONE',  ( -0.000000000000000000, 1.000000000000000000, -0.000000000000000000 ) ) ;
#44410=CARTESIAN_POINT ( 'NONE',  ( -3.152801135295367985, -154.0625000013656063, 3.152801135295367096 ) ) ;
#44417=CARTESIAN_POINT ( 'NONE',  ( 1.975475456537005874E-15, -8.624999997268812280, 5.000000000000000000 ) ) ;
#44418=CARTESIAN_POINT ( 'NONE',  ( 2.499999999999998668, -2.333333333333333037, -4.330127018922193649 ) ) ;
#44420=CARTESIAN_POINT ( 'NONE',  ( -4.458734124999999437, -69.31249999863439371, 0.000000000000000000 ) ) ;
#44421=DIRECTION ( 'NONE',  ( -0.000000000000000000, 1.000000000000000000, -0.000000000000000000 ) ) ;
#44424=CARTESIAN_POINT ( 'NONE',  ( 2.499999999999998668, -1.208333330602148870, -4.330127018922193649 ) ) ;
#44425=CARTESIAN_POINT ( 'NONE',  ( 9.457646018065525792E-16, -35.06249999863440792, 5.148502694627439702 ) ) ;
#44426=ORIENTED_EDGE ( 'NONE', *, *, #41684, .F. ) ;
#44431=CARTESIAN_POINT ( 'NONE',  ( 5.000000000000000000, -48.41666666666665719, -2.886751345948129988 ) ) ;
#44432=CARTESIAN_POINT ( 'NONE',  ( 0.000000000000000000, -170.0000000000000000, 0.000000000000000000 ) ) ;
#44434=CARTESIAN_POINT ( 'NONE',  ( 1.975475456537005874E-15, -3.750000000000001776, 5.000000000000000000 ) ) ;
#44435=CARTESIAN_POINT ( 'NONE',  ( -3.152548672688508926E-16, -72.56249999863439371, -5.148502694627439702 ) ) ;
#44436=CARTESIAN_POINT ( 'NONE',  ( -1.846868145590737420, -146.0000000013655779, 4.458734124999999437 ) ) ;
#44437=CARTESIAN_POINT ( 'NONE',  ( -4.458734124999999437, -80.39583333196772230, -2.574251347313719407 ) ) ;
#44440=CARTESIAN_POINT ( 'NONE',  ( 4.458734125000001214, -31.14583333196773651, 2.574251347313718519 ) ) ;
#44441=CARTESIAN_POINT ( 'NONE',  ( 2.499999999999998668, -70.20833333060214443, -4.330127018922193649 ) ) ;
#44447=CARTESIAN_POINT ( 'NONE',  ( 5.000000000000000000, 28.58333333333333215, -2.886751345948130876 ) ) ;
#44449=VERTEX_POINT ( 'NONE', #50050 ) ;
#44452=CARTESIAN_POINT ( 'NONE',  ( -4.458734124999998549, -57.47916666530108643, 2.574251347313722516 ) ) ;
#44455=CARTESIAN_POINT ( 'NONE',  ( -2.071067811865391128, -146.6875000000000568, -5.000000000000086153 ) ) ;
#44457=CARTESIAN_POINT ( 'NONE',  ( -2.229367062499996610, 11.85416666803225993, 3.861377020970582219 ) ) ;
#44459=CARTESIAN_POINT ( 'NONE',  ( 1.975475456537005874E-15, -0.7499999999999996669, 5.000000000000000000 ) ) ;
#44460=CARTESIAN_POINT ( 'NONE',  ( -3.152801135295367096, -162.0625000013656063, -3.152801135295367541 ) ) ;
#44461=ORIENTED_EDGE ( 'NONE', *, *, #15856, .T. ) ;
#44463=CARTESIAN_POINT ( 'NONE',  ( -4.999999999999998224, -69.79166666393547303, 2.886751345948131764 ) ) ;
#44465=( BOUNDED_CURVE ( )  B_SPLINE_CURVE ( 2, ( #44050, #44691, #24447, #20906, #39230, #332, #59509, #10599, #29895 ),
 .UNSPECIFIED., .F., .F. ) 
 B_SPLINE_CURVE_WITH_KNOTS ( ( 3, 2, 2, 2, 3 ),
 ( 0.4854166666666666630, 0.4861111111111111049, 0.4874999999999999889, 0.4888888888888888729, 0.4895833333333333148 ),
 .UNSPECIFIED. ) 
 CURVE ( )  GEOMETRIC_REPRESENTATION_ITEM ( )  RATIONAL_B_SPLINE_CURVE ( ( 0.9330127018922194093, 0.9330127018922194093, 1.000000000000000000, 0.8660254037844387076, 1.000000000000000000, 0.8660254037844387076, 1.000000000000000000, 0.9330127018922194093, 0.9330127018922194093 ) ) 
 REPRESENTATION_ITEM ( '' )  );
#44467=CARTESIAN_POINT ( 'NONE',  ( -6.972266317189433020E-16, 1.750000000000000444, -5.000000000000000000 ) ) ;
#44471=CARTESIAN_POINT ( 'NONE',  ( 1.339745962155612702, -78.16965819600731891, -5.000000000000000000 ) ) ;
#44472=DIRECTION ( 'NONE',  ( -0.000000000000000000, 1.000000000000000000, -0.000000000000000000 ) ) ;
#44475=CARTESIAN_POINT ( 'NONE',  ( 4.458734124999998549, 9.020833334698927786, -2.574251347313721627 ) ) ;
#44476=CARTESIAN_POINT ( 'NONE',  ( 2.071067811865644703, -150.8125000000000284, -4.999999999999831246 ) ) ;
#44478=CARTESIAN_POINT ( 'NONE',  ( 3.535533905932738197, -148.0000000027311842, -3.535533905932738197 ) ) ;
#44486=CARTESIAN_POINT ( 'NONE',  ( -4.458734124999999437, -167.2500000013655779, -1.846868145590735644 ) ) ;
#44487=CARTESIAN_POINT ( 'NONE',  ( -2.229367062500000163, -35.47916666530107221, -3.861377020970580443 ) ) ;
#44488=CARTESIAN_POINT ( 'NONE',  ( -5.000000000000000000, -33.08333333333332860, -2.886751345948128211 ) ) ;
#44489=CARTESIAN_POINT ( 'NONE',  ( 5.000000000000000888, -45.45833333060214443, 2.886751345948126879 ) ) ;
#44491=CARTESIAN_POINT ( 'NONE',  ( -4.458734125000001214, -141.8750000013656063, 1.846868145590734089 ) ) ;
#44492=ORIENTED_EDGE ( 'NONE', *, *, #29931, .T. ) ;
#44493=CARTESIAN_POINT ( 'NONE',  ( -2.499999999999996447, -89.70833333060214443, 4.330127018922195425 ) ) ;
#44494=VERTEX_POINT ( 'NONE', #59715 ) ;
#44495=CARTESIAN_POINT ( 'NONE',  ( 9.457646018065525792E-16, -61.31249999863440792, 5.148502694627439702 ) ) ;
#44497=CARTESIAN_POINT ( 'NONE',  ( -9.184850993605147944E-16, -162.2500000000000000, 5.000000000000000000 ) ) ;
#44498=CARTESIAN_POINT ( 'NONE',  ( 5.000000000000000000, 13.58333333333333215, -2.886751345948129988 ) ) ;
#44499=CARTESIAN_POINT ( 'NONE',  ( 2.229367062499998831, -49.64583333196772941, -3.861377020970580887 ) ) ;
#44500=CARTESIAN_POINT ( 'NONE',  ( -3.152548672688508926E-16, -7.562499998634404363, -5.148502694627439702 ) ) ;
#44501=CARTESIAN_POINT ( 'NONE',  ( -1.339745962155613812, 3.919658201469705894, -5.000000000000000000 ) ) ;
#44502=EDGE_CURVE ( 'NONE', #12181, #27389, #33578, .T. ) ;
#44503=CARTESIAN_POINT ( 'NONE',  ( 5.000000000000000888, -165.0625000027312126, -2.071067811865475505 ) ) ;
#44504=CARTESIAN_POINT ( 'NONE',  ( 5.000000000000000888, -158.0625000027312126, -2.071067811865475505 ) ) ;
#44505=DIRECTION ( 'NONE',  ( -0.000000000000000000, 1.000000000000000000, -0.000000000000000000 ) ) ;
#44506=CARTESIAN_POINT ( 'NONE',  ( 1.339745962155602488, 21.41965820146970145, 5.000000000000007105 ) ) ;
#44509=CARTESIAN_POINT ( 'NONE',  ( -1.049326080737009628E-13, -3.624999997268818053, 5.000000000000000000 ) ) ;
#44510=CARTESIAN_POINT ( 'NONE',  ( -2.229367062500000163, -53.47916666530107221, -3.861377020970580443 ) ) ;
#44511=CARTESIAN_POINT ( 'NONE',  ( 1.846868145590736310, -154.8750000013655779, 4.458734124999999437 ) ) ;
#44512=EDGE_CURVE ( 'NONE', #14934, #45853, #31897, .T. ) ;
#44513=CARTESIAN_POINT ( 'NONE',  ( 2.500000000000002220, -53.54166666393548013, 4.330127018922192761 ) ) ;
#44514=ORIENTED_EDGE ( 'NONE', *, *, #31853, .F. ) ;
#44515=CARTESIAN_POINT ( 'NONE',  ( 1.339745962155612702, -26.29465819873852084, -5.000000000000000000 ) ) ;
#44516=CARTESIAN_POINT ( 'NONE',  ( 2.229367062499998831, 3.104166668032259935, -3.861377020970580887 ) ) ;
#44518=( BOUNDED_CURVE ( )  B_SPLINE_CURVE ( 2, ( #19850, #39464, #34643, #54267, #60060, #10207, #29809, #49442, #6350 ),
 .UNSPECIFIED., .F., .F. ) 
 B_SPLINE_CURVE_WITH_KNOTS ( ( 3, 2, 2, 2, 3 ),
 ( 0.7249999999999996447, 0.7291666666666662966, 0.7333333333333329485, 0.7374999999999998224, 0.7416666666666664742 ),
 .UNSPECIFIED. ) 
 CURVE ( )  GEOMETRIC_REPRESENTATION_ITEM ( )  RATIONAL_B_SPLINE_CURVE ( ( 1.000000000000005995, 0.9238795325112806323, 1.000000000000000000, 0.9238795325112867385, 1.000000000000000000, 0.9238795325112867385, 1.000000000000000000, 0.9238795325112908463, 0.9999999999999958922 ) ) 
 REPRESENTATION_ITEM ( '' )  );
#44520=CARTESIAN_POINT ( 'NONE',  ( 4.458734125000000326, -156.3750000013655779, -1.846868145590734978 ) ) ;
#44521=EDGE_CURVE ( 'NONE', #56591, #39148, #46734, .T. ) ;
#44522=EDGE_LOOP ( 'NONE', ( #46311, #61704, #37250, #24997 ) ) ;
#44523=ADVANCED_FACE ( 'NONE', ( #36529 ), #56161, .T. ) ;
#44527=CARTESIAN_POINT ( 'NONE',  ( -2.229367062499996610, -42.39583333196773651, 3.861377020970582219 ) ) ;
#44528=ORIENTED_EDGE ( 'NONE', *, *, #10172, .T. ) ;
#44530=EDGE_CURVE ( 'NONE', #44325, #1513, #54045, .T. ) ;
#44531=CARTESIAN_POINT ( 'NONE',  ( 2.500000000000002220, 9.458333336064519870, 4.330127018922192761 ) ) ;
#44533=LINE ( 'NONE', #29403, #44051 ) ;
#44535=CARTESIAN_POINT ( 'NONE',  ( -4.458734124999999437, 28.60416666803226349, -2.574251347313719407 ) ) ;
#44539=LINE ( 'NONE', #10771, #52812 ) ;
#44541=CARTESIAN_POINT ( 'NONE',  ( -2.499999999999996447, 10.29166666939785024, 4.330127018922195425 ) ) ;
#44546=CARTESIAN_POINT ( 'NONE',  ( 0.000000000000000000, -170.0000000000000000, 0.000000000000000000 ) ) ;
#44554=CARTESIAN_POINT ( 'NONE',  ( -3.535533905932737309, -162.7500000027312126, -3.535533905932738197 ) ) ;
#44564=CARTESIAN_POINT ( 'NONE',  ( -2.071067811865432873, -141.8125000027311842, -5.000000000000041744 ) ) ;
#44565=CARTESIAN_POINT ( 'NONE',  ( -2.229367062500000163, -20.47916666530107221, -3.861377020970580443 ) ) ;
#44566=CARTESIAN_POINT ( 'NONE',  ( -5.000000000000000000, -79.87499999726881583, 0.000000000000000000 ) ) ;
#44567=CARTESIAN_POINT ( 'NONE',  ( 2.071067811865475505, -156.8125000000000284, -5.000000000000000888 ) ) ;
#44570=CARTESIAN_POINT ( 'NONE',  ( 2.229367062500001939, -44.22916666530106511, 3.861377020970579999 ) ) ;
#44574=CARTESIAN_POINT ( 'NONE',  ( 5.000000000000000000, 28.58333333333333215, -2.886751345948129988 ) ) ;
#44577=VECTOR ( 'NONE', #17108, 1000.000000000000000 ) ;
#44578=CARTESIAN_POINT ( 'NONE',  ( 2.229367062499998831, 7.354166668032259935, -3.861377020970580887 ) ) ;
#44580=CARTESIAN_POINT ( 'NONE',  ( 3.061616997868383141E-16, -165.8750000027312126, -5.000000000000000000 ) ) ;
#44581=CARTESIAN_POINT ( 'NONE',  ( 5.000000000000000000, -82.50000000000000000, -6.123233995736766282E-16 ) ) ;
#44582=CARTESIAN_POINT ( 'NONE',  ( -3.152548672688508926E-16, 21.18750000136559208, -5.148502694627439702 ) ) ;
#44584=CARTESIAN_POINT ( 'NONE',  ( 5.000000000000000000, 6.708333336064521646, -2.886751345948129988 ) ) ;
#44587=ORIENTED_EDGE ( 'NONE', *, *, #21251, .F. ) ;
#44588=CARTESIAN_POINT ( 'NONE',  ( 6.123233995736766282E-16, -170.0000000000000000, -5.000000000000000000 ) ) ;
#44589=CARTESIAN_POINT ( 'NONE',  ( -4.458734124999998549, -36.22916666530106511, 2.574251347313722516 ) ) ;
#44590=CARTESIAN_POINT ( 'NONE',  ( -2.500000000000000444, -37.04166666393548013, -4.330127018922193649 ) ) ;
#44591=ORIENTED_EDGE ( 'NONE', *, *, #95, .F. ) ;
#44593=CARTESIAN_POINT ( 'NONE',  ( -4.458734124999999437, -10.31249999863440792, 0.000000000000000000 ) ) ;
#44594=CARTESIAN_POINT ( 'NONE',  ( 4.458734124999998549, -12.97916666530107044, -2.574251347313721627 ) ) ;
#44595=ORIENTED_EDGE ( 'NONE', *, *, #36609, .T. ) ;
#44596=CARTESIAN_POINT ( 'NONE',  ( -5.000000000000000000, -81.08333333333332860, -2.886751345948128211 ) ) ;
#44597=CARTESIAN_POINT ( 'NONE',  ( -3.152801135295367985, -167.8125000013656063, 3.152801135295367096 ) ) ;
#44599=CARTESIAN_POINT ( 'NONE',  ( 1.060575238724906964E-15, -79.62499999726881583, 5.773502691896257311 ) ) ;
#44600=CARTESIAN_POINT ( 'NONE',  ( -2.499999999999996447, -17.83333333333333215, 4.330127018922195425 ) ) ;
#44603=CARTESIAN_POINT ( 'NONE',  ( 4.458734124999998549, -26.97916666530107221, -2.574251347313721627 ) ) ;
#44604=CARTESIAN_POINT ( 'NONE',  ( 5.000000000000000888, -29.58333333333332860, 2.886751345948126879 ) ) ;
#44605=ORIENTED_EDGE ( 'NONE', *, *, #6773, .T. ) ;
#44607=CARTESIAN_POINT ( 'NONE',  ( 2.730187237215162345E-16, -163.4375000013655779, -4.458734124999999437 ) ) ;
#44609=CARTESIAN_POINT ( 'NONE',  ( 5.000000000000000000, -23.50000000000000000, -6.123233995736766282E-16 ) ) ;
#44612=CARTESIAN_POINT ( 'NONE',  ( 4.458734124999998549, -74.97916666530106511, -2.574251347313721627 ) ) ;
#44615=CARTESIAN_POINT ( 'NONE',  ( 4.458734124999999437, -146.6875000013656063, 0.000000000000000000 ) ) ;
#44622=CARTESIAN_POINT ( 'NONE',  ( 1.846868145590736310, -141.8750000013656063, 4.458734124999999437 ) ) ;
#44627=CARTESIAN_POINT ( 'NONE',  ( -4.458734124999999437, -73.56249999863439371, 0.000000000000000000 ) ) ;
#44628=CARTESIAN_POINT ( 'NONE',  ( -9.184850993605147944E-16, -144.3750000027312126, 5.000000000000000000 ) ) ;
#44629=CARTESIAN_POINT ( 'NONE',  ( -6.972266317189433020E-16, -54.12499999726880162, -5.000000000000000000 ) ) ;
#44639=CARTESIAN_POINT ( 'NONE',  ( -2.229367062499996610, 19.60416666803225993, 3.861377020970582219 ) ) ;
#44640=DIRECTION ( 'NONE',  ( -0.000000000000000000, 1.000000000000000000, -0.000000000000000000 ) ) ;
#44645=CYLINDRICAL_SURFACE ( 'NONE', #34606, 5.000000000000000000 ) ;
#44646=CARTESIAN_POINT ( 'NONE',  ( -4.458734124999999437, -4.312499998634401699, 0.000000000000000000 ) ) ;
#44647=VERTEX_POINT ( 'NONE', #13037 ) ;
#44648=CARTESIAN_POINT ( 'NONE',  ( -2.229367062499996610, -29.39583333196774007, 3.861377020970582219 ) ) ;
#44652=CARTESIAN_POINT ( 'NONE',  ( -4.458734124999998549, 23.77083333469892423, 2.574251347313722516 ) ) ;
#44653=CARTESIAN_POINT ( 'NONE',  ( 1.339745962155612702, 26.83034180399266333, -5.000000000000000000 ) ) ;
#44655=CARTESIAN_POINT ( 'NONE',  ( -4.458734124999999437, -72.64583333196773651, -2.574251347313719407 ) ) ;
#44657=CARTESIAN_POINT ( 'NONE',  ( 2.499999999999998668, 25.79166666939785202, -4.330127018922193649 ) ) ;
#44661=CARTESIAN_POINT ( 'NONE',  ( 0.000000000000000000, -170.0000000000000000, 0.000000000000000000 ) ) ;
#44662=CARTESIAN_POINT ( 'NONE',  ( 1.060575238724906964E-15, -16.75000000000000355, 5.773502691896257311 ) ) ;
#44663=CARTESIAN_POINT ( 'NONE',  ( 2.229367062499998831, -22.64583333196773651, -3.861377020970580887 ) ) ;
#44664=CARTESIAN_POINT ( 'NONE',  ( 4.458734124999999437, -82.81249999863440792, -5.460374474430324690E-16 ) ) ;
#44665=( BOUNDED_CURVE ( )  B_SPLINE_CURVE ( 2, ( #18841, #38459, #44877, #59037, #45515, #50019, #50346, #15292, #25582 ),
 .UNSPECIFIED., .F., .F. ) 
 B_SPLINE_CURVE_WITH_KNOTS ( ( 3, 2, 2, 2, 3 ),
 ( 0.1750000000000001554, 0.1791666666666668351, 0.1833333333333334869, 0.1875000000000001665, 0.1916666666666668462 ),
 .UNSPECIFIED. ) 
 CURVE ( )  GEOMETRIC_REPRESENTATION_ITEM ( )  RATIONAL_B_SPLINE_CURVE ( ( 0.9999999999999970024, 0.9238795325112897361, 1.000000000000000000, 0.9238795325112867385, 1.000000000000000000, 0.9238795325112867385, 1.000000000000000000, 0.9238795325112837409, 1.000000000000003109 ) ) 
 REPRESENTATION_ITEM ( '' )  );
#44666=CARTESIAN_POINT ( 'NONE',  ( 5.000000000000000000, -21.29166666393548013, -2.886751345948129988 ) ) ;
#44667=CARTESIAN_POINT ( 'NONE',  ( -3.152548672688508926E-16, -51.56249999863441502, -5.148502694627439702 ) ) ;
#44668=ORIENTED_EDGE ( 'NONE', *, *, #8230, .T. ) ;
#44669=CARTESIAN_POINT ( 'NONE',  ( 5.000000000000000888, -70.45833333060214443, 2.886751345948126879 ) ) ;
#44670=FACE_OUTER_BOUND ( 'NONE', #52190, .T. ) ;
#44671=CARTESIAN_POINT ( 'NONE',  ( -2.229367062499996610, -0.3958333319677397322, 3.861377020970582219 ) ) ;
#44674=CARTESIAN_POINT ( 'NONE',  ( 5.000000000000000000, -68.41666666666667140, -2.886751345948129988 ) ) ;
#44675=CARTESIAN_POINT ( 'NONE',  ( -3.152801135295367985, -154.0625000013656063, 3.152801135295367096 ) ) ;
#44677=CARTESIAN_POINT ( 'NONE',  ( -5.000000000000000000, -80.95833333060214443, -2.886751345948128211 ) ) ;
#44678=CARTESIAN_POINT ( 'NONE',  ( 3.535533905932738197, -162.8750000000000284, -3.535533905932738197 ) ) ;
#44681=CARTESIAN_POINT ( 'NONE',  ( 2.229367062500001939, -12.22916666530107044, 3.861377020970579999 ) ) ;
#44682=CARTESIAN_POINT ( 'NONE',  ( -3.152548672688508926E-16, -46.81249999863440081, -5.148502694627439702 ) ) ;
#44684=CARTESIAN_POINT ( 'NONE',  ( -8.190561711645485556E-16, -144.6875000013656063, 4.458734124999999437 ) ) ;
#44687=VERTEX_POINT ( 'NONE', #60992 ) ;
#44689=DIRECTION ( 'NONE',  ( -0.000000000000000000, 1.000000000000000000, -0.000000000000000000 ) ) ;
#44691=CARTESIAN_POINT ( 'NONE',  ( 1.339745962155612702, -29.16965819600733312, -5.000000000000000000 ) ) ;
#44694=CARTESIAN_POINT ( 'NONE',  ( 5.000000000000000888, -19.58333333333333215, 2.886751345948126879 ) ) ;
#44697=CARTESIAN_POINT ( 'NONE',  ( -4.458734124999998549, -5.229166665301072214, 2.574251347313722516 ) ) ;
#44698=CARTESIAN_POINT ( 'NONE',  ( 4.458734124999997661, -150.5000000013656347, 1.846868145590737864 ) ) ;
#44700=EDGE_LOOP ( 'NONE', ( #14548, #47550, #57109, #50877 ) ) ;
#44706=CARTESIAN_POINT ( 'NONE',  ( 1.975475456537005874E-15, -85.62499999726880162, 5.000000000000000000 ) ) ;
#44707=CARTESIAN_POINT ( 'NONE',  ( 1.975475456537005874E-15, -58.75000000000000000, 5.000000000000000000 ) ) ;
#44708=AXIS2_PLACEMENT_3D ( 'NONE', #27840, #37819, #7922 ) ;
#44713=CARTESIAN_POINT ( 'NONE',  ( 0.000000000000000000, -170.0000000000000000, 0.000000000000000000 ) ) ;
#44715=CARTESIAN_POINT ( 'NONE',  ( 2.229367062499998831, 15.35416666803225993, -3.861377020970580887 ) ) ;
#44718=CARTESIAN_POINT ( 'NONE',  ( -2.229367062500000163, -14.72916666530107221, -3.861377020970580443 ) ) ;
#44721=CARTESIAN_POINT ( 'NONE',  ( 4.458734124999999437, -164.4375000013655779, 0.000000000000000000 ) ) ;
#44726=EDGE_CURVE ( 'NONE', #25339, #47748, #16912, .T. ) ;
#44727=CARTESIAN_POINT ( 'NONE',  ( -9.184850993605147944E-16, -142.3750000027312126, 5.000000000000000000 ) ) ;
#44728=CARTESIAN_POINT ( 'NONE',  ( -2.499999999999996447, -88.70833333060214443, 4.330127018922195425 ) ) ;
#44730=CARTESIAN_POINT ( 'NONE',  ( 4.458734124999999437, -152.6875000013656063, 0.000000000000000000 ) ) ;
#44738=CARTESIAN_POINT ( 'NONE',  ( 5.000000000000000000, -2.416666666666664298, -2.886751345948129988 ) ) ;
#44740=CARTESIAN_POINT ( 'NONE',  ( 4.458734124999999437, -67.81249999863440792, -5.460374474430324690E-16 ) ) ;
#44742=CARTESIAN_POINT ( 'NONE',  ( 5.000000000000000000, -4.291666663935479242, -2.886751345948129988 ) ) ;
#44743=CARTESIAN_POINT ( 'NONE',  ( -3.152548672688508926E-16, -33.56249999863440792, -5.148502694627439702 ) ) ;
#44745=DIRECTION ( 'NONE',  ( -0.000000000000000000, 1.000000000000000000, -0.000000000000000000 ) ) ;
#44747=ORIENTED_EDGE ( 'NONE', *, *, #18953, .F. ) ;
#44749=CARTESIAN_POINT ( 'NONE',  ( 2.499999999999998668, -49.33333333333332860, -4.330127018922193649 ) ) ;
#44750=CYLINDRICAL_SURFACE ( 'NONE', #45967, 5.000000000000000000 ) ;
#44752=CARTESIAN_POINT ( 'NONE',  ( -1.339745962155610925, -3.794658198738523058, 5.000000000000000000 ) ) ;
#44753=CARTESIAN_POINT ( 'NONE',  ( 4.458734124999998549, -75.72916666530106511, -2.574251347313721627 ) ) ;
#44754=CARTESIAN_POINT ( 'NONE',  ( -3.152801135295367096, -142.3125000013655779, -3.152801135295367541 ) ) ;
#44755=CARTESIAN_POINT ( 'NONE',  ( 4.458734124999999437, -79.81249999863440792, -5.460374474430324690E-16 ) ) ;
#44757=CARTESIAN_POINT ( 'NONE',  ( 2.229367062500001939, -30.22916666530107221, 3.861377020970579999 ) ) ;
#44758=CARTESIAN_POINT ( 'NONE',  ( -5.000000000000000000, -69.87499999726880162, 0.000000000000000000 ) ) ;
#44759=ORIENTED_EDGE ( 'NONE', *, *, #18620, .T. ) ;
#44761=CARTESIAN_POINT ( 'NONE',  ( 5.000000000000000000, -51.50000000000000711, -6.123233995736766282E-16 ) ) ;
#44762=VERTEX_POINT ( 'NONE', #46071 ) ;
#44768=( BOUNDED_CURVE ( )  B_SPLINE_CURVE ( 2, ( #38858, #48829, #15064, #4768, #10237, #24394, #43997, #29842, #19564 ),
 .UNSPECIFIED., .F., .F. ) 
 B_SPLINE_CURVE_WITH_KNOTS ( ( 3, 2, 2, 2, 3 ),
 ( 0.02291666666666666852, 0.02361111111111111049, 0.02500000000000000139, 0.02638888888888888881, 0.02708333333333333426 ),
 .UNSPECIFIED. ) 
 CURVE ( )  GEOMETRIC_REPRESENTATION_ITEM ( )  RATIONAL_B_SPLINE_CURVE ( ( 0.9330127018922194093, 0.9330127018922195203, 1.000000000000000000, 0.8660254037844387076, 1.000000000000000000, 0.8660254037844387076, 1.000000000000000000, 0.9330127018922191873, 0.9330127018922194093 ) ) 
 REPRESENTATION_ITEM ( '' )  );
#44770=CARTESIAN_POINT ( 'NONE',  ( -4.458734124999999437, -59.64583333196773651, -2.574251347313719407 ) ) ;
#44772=ORIENTED_EDGE ( 'NONE', *, *, #19304, .F. ) ;
#44775=CARTESIAN_POINT ( 'NONE',  ( 4.458734124999999437, 11.18750000136559386, -5.460374474430324690E-16 ) ) ;
#44777=CARTESIAN_POINT ( 'NONE',  ( -2.500000000000000444, -1.166666666666666519, -4.330127018922193649 ) ) ;
#44778=CARTESIAN_POINT ( 'NONE',  ( -3.152801135295367985, -161.8125000013656063, 3.152801135295367096 ) ) ;
#44779=LINE ( 'NONE', #741, #884 ) ;
#44780=ORIENTED_EDGE ( 'NONE', *, *, #58233, .T. ) ;
#44782=CARTESIAN_POINT ( 'NONE',  ( -1.339745962155610925, -51.66965819600733312, 5.000000000000000000 ) ) ;
#44784=EDGE_CURVE ( 'NONE', #11542, #55337, #21635, .T. ) ;
#44785=CARTESIAN_POINT ( 'NONE',  ( 5.000000000000000000, -71.29166666393547303, -2.886751345948130876 ) ) ;
#44790=LINE ( 'NONE', #1081, #32711 ) ;
#44791=LINE ( 'NONE', #60251, #18271 ) ;
#44796=CARTESIAN_POINT ( 'NONE',  ( 4.458734125000000326, 6.854166668032259935, 2.574251347313718519 ) ) ;
#44797=VECTOR ( 'NONE', #34218, 1000.000000000000000 ) ;
#44798=DIRECTION ( 'NONE',  ( -0.000000000000000000, 1.000000000000000000, -0.000000000000000000 ) ) ;
#44800=CARTESIAN_POINT ( 'NONE',  ( -2.071067811865478170, -151.4375000027312410, 5.000000000000000000 ) ) ;
#44801=FACE_OUTER_BOUND ( 'NONE', #34746, .T. ) ;
#44806=CARTESIAN_POINT ( 'NONE',  ( 3.061616997868383141E-16, -140.7500000000000000, -5.000000000000000000 ) ) ;
#44810=CARTESIAN_POINT ( 'NONE',  ( 1.846868145590735200, -167.5000000013655779, -4.458734124999999437 ) ) ;
#44811=CARTESIAN_POINT ( 'NONE',  ( -6.972266317189433020E-16, -25.12499999726881228, -5.000000000000000000 ) ) ;
#44812=CARTESIAN_POINT ( 'NONE',  ( 6.123233995736766282E-16, -170.0000000000000000, -5.000000000000000000 ) ) ;
#44814=CARTESIAN_POINT ( 'NONE',  ( -4.458734125000000326, -145.0000000013656063, -1.846868145590735644 ) ) ;
#44815=ORIENTED_EDGE ( 'NONE', *, *, #13302, .T. ) ;
#44816=CARTESIAN_POINT ( 'NONE',  ( -2.229367062500000163, 27.27083333469892779, -3.861377020970580443 ) ) ;
#44817=VERTEX_POINT ( 'NONE', #55088 ) ;
#44818=CARTESIAN_POINT ( 'NONE',  ( -3.152548672688508926E-16, -63.81249999863440792, -5.148502694627439702 ) ) ;
#44821=CARTESIAN_POINT ( 'NONE',  ( 5.000000000000000888, 11.41666666666666607, 2.886751345948126879 ) ) ;
#44822=CARTESIAN_POINT ( 'NONE',  ( 2.229367062499998831, -51.64583333196773651, -3.861377020970580887 ) ) ;
#44823=CARTESIAN_POINT ( 'NONE',  ( 2.229367062499998831, -10.64583333196773829, -3.861377020970580887 ) ) ;
#44824=CARTESIAN_POINT ( 'NONE',  ( -6.972266317189433020E-16, -67.12499999726881583, -5.000000000000000000 ) ) ;
#44825=FACE_OUTER_BOUND ( 'NONE', #55219, .T. ) ;
#44828=CARTESIAN_POINT ( 'NONE',  ( 5.000000000000000000, -66.29166666393547303, -2.886751345948130876 ) ) ;
#44831=CARTESIAN_POINT ( 'NONE',  ( -5.000000000000000888, -140.5625000027312410, 2.071067811865474617 ) ) ;
#44832=CARTESIAN_POINT ( 'NONE',  ( 2.229367062499998831, -55.64583333196773651, -3.861377020970580887 ) ) ;
#44833=CARTESIAN_POINT ( 'NONE',  ( -3.152801135295367985, -154.0625000013656063, 3.152801135295367096 ) ) ;
#44834=ADVANCED_FACE ( 'NONE', ( #40916 ), #60874, .T. ) ;
#44835=CARTESIAN_POINT ( 'NONE',  ( -5.000000000000000000, -55.87499999726880162, 0.000000000000000000 ) ) ;
#44836=VERTEX_POINT ( 'NONE', #11329 ) ;
#44837=CARTESIAN_POINT ( 'NONE',  ( 0.000000000000000000, -170.0000000000000000, 0.000000000000000000 ) ) ;
#44838=CARTESIAN_POINT ( 'NONE',  ( -2.229367062500000163, 2.270833334698928230, -3.861377020970580443 ) ) ;
#44839=EDGE_LOOP ( 'NONE', ( #2735, #29211, #9356, #9648 ) ) ;
#44841=CYLINDRICAL_SURFACE ( 'NONE', #58359, 5.000000000000000000 ) ;
#44842=CARTESIAN_POINT ( 'NONE',  ( -8.190561711645485556E-16, -156.6875000013655779, 4.458734124999999437 ) ) ;
#44845=CARTESIAN_POINT ( 'NONE',  ( 5.000000000000000000, -83.49999999999998579, -6.123233995736766282E-16 ) ) ;
#44848=CARTESIAN_POINT ( 'NONE',  ( -4.458734124999999437, -44.64583333196773651, -2.574251347313719407 ) ) ;
#44849=AXIS2_PLACEMENT_3D ( 'NONE', #3016, #56727, #12647 ) ;
#44851=AXIS2_PLACEMENT_3D ( 'NONE', #45920, #31124, #30483 ) ;
#44855=CARTESIAN_POINT ( 'NONE',  ( -4.458734124999999437, -88.64583333196773651, -2.574251347313719407 ) ) ;
#44857=CARTESIAN_POINT ( 'NONE',  ( -5.000000000000000000, -165.5000000000000000, -6.123233995736766282E-16 ) ) ;
#44858=DIRECTION ( 'NONE',  ( 0.000000000000000000, -1.000000000000000000, 0.000000000000000000 ) ) ;
#44864=ADVANCED_FACE ( 'NONE', ( #55729 ), #35790, .T. ) ;
#44865=CARTESIAN_POINT ( 'NONE',  ( 2.071067811865603403, -157.3125000027311842, 4.999999999999872990 ) ) ;
#44866=ADVANCED_FACE ( 'NONE', ( #2030 ), #16485, .T. ) ;
#44870=LINE ( 'NONE', #833, #47089 ) ;
#44871=CARTESIAN_POINT ( 'NONE',  ( 9.457646018065525792E-16, -88.31249999863439371, 5.148502694627439702 ) ) ;
#44872=EDGE_CURVE ( 'NONE', #2557, #28361, #60654, .T. ) ;
#44873=FACE_OUTER_BOUND ( 'NONE', #1362, .T. ) ;
#44875=EDGE_CURVE ( 'NONE', #6056, #24978, #22890, .T. ) ;
#44876=VERTEX_POINT ( 'NONE', #20356 ) ;
#44877=CARTESIAN_POINT ( 'NONE',  ( -3.535533905932737309, -163.7500000027312126, -3.535533905932738197 ) ) ;
#44879=CARTESIAN_POINT ( 'NONE',  ( -2.071067811865478170, -162.4375000027311842, 5.000000000000000000 ) ) ;
#44882=CARTESIAN_POINT ( 'NONE',  ( 2.071067811865412445, -162.9375000027312126, -5.000000000000063949 ) ) ;
#44884=EDGE_CURVE ( 'NONE', #21524, #18684, #36418, .T. ) ;
#44891=EDGE_CURVE ( 'NONE', #18516, #24077, #30309, .T. ) ;
#44893=CARTESIAN_POINT ( 'NONE',  ( -2.071067811865562991, -141.4375000027311842, 4.999999999999913847 ) ) ;
#44894=CARTESIAN_POINT ( 'NONE',  ( 2.229367062500001939, -21.97916666530107221, 3.861377020970579999 ) ) ;
#44896=CARTESIAN_POINT ( 'NONE',  ( -2.071067811865478170, -154.3125000000000284, 5.000000000000000000 ) ) ;
#44899=CARTESIAN_POINT ( 'NONE',  ( -4.458734124999999437, -154.9375000013655779, -5.460374474430324690E-16 ) ) ;
#44901=CARTESIAN_POINT ( 'NONE',  ( 2.229367062500001939, -48.22916666530106511, 3.861377020970579999 ) ) ;
#44902=ADVANCED_FACE ( 'NONE', ( #8022 ), #7710, .T. ) ;
#44905=CARTESIAN_POINT ( 'NONE',  ( -5.000000000000000000, 28.99999999999999645, 0.000000000000000000 ) ) ;
#44908=CARTESIAN_POINT ( 'NONE',  ( 2.229367062500001939, 12.02083333469892601, 3.861377020970579999 ) ) ;
#44911=CARTESIAN_POINT ( 'NONE',  ( 0.000000000000000000, -170.0000000000000000, 0.000000000000000000 ) ) ;
#44912=CARTESIAN_POINT ( 'NONE',  ( -2.229367062499996610, 19.60416666803225993, 3.861377020970582219 ) ) ;
#44914=( BOUNDED_CURVE ( )  B_SPLINE_CURVE ( 2, ( #9537, #29141, #34291, #10809, #29777, #4708, #14994, #6006, #24332 ),
 .UNSPECIFIED., .F., .F. ) 
 B_SPLINE_CURVE_WITH_KNOTS ( ( 3, 2, 2, 2, 3 ),
 ( 0.6145833333333333703, 0.6152777777777778123, 0.6166666666666666963, 0.6180555555555555802, 0.6187500000000000222 ),
 .UNSPECIFIED. ) 
 CURVE ( )  GEOMETRIC_REPRESENTATION_ITEM ( )  RATIONAL_B_SPLINE_CURVE ( ( 0.9330127018922194093, 0.9330127018922194093, 1.000000000000000000, 0.8660254037844387076, 1.000000000000000000, 0.8660254037844387076, 1.000000000000000000, 0.9330127018922194093, 0.9330127018922194093 ) ) 
 REPRESENTATION_ITEM ( '' )  );
#44915=CARTESIAN_POINT ( 'NONE',  ( 5.000000000000000888, 9.541666669397852019, 2.886751345948126879 ) ) ;
#44917=CARTESIAN_POINT ( 'NONE',  ( 3.535533905932738197, -162.0000000027312126, -3.535533905932738197 ) ) ;
#44918=ORIENTED_EDGE ( 'NONE', *, *, #19755, .T. ) ;
#44920=CARTESIAN_POINT ( 'NONE',  ( -2.229367062500000163, -40.47916666530107221, -3.861377020970580443 ) ) ;
#44921=CARTESIAN_POINT ( 'NONE',  ( -5.000000000000000000, -38.87499999726880162, 0.000000000000000000 ) ) ;
#44923=CARTESIAN_POINT ( 'NONE',  ( 2.229367062499998831, -12.64583333196774007, -3.861377020970580887 ) ) ;
#44924=CARTESIAN_POINT ( 'NONE',  ( 4.458734125000001214, -19.14583333196774007, 2.574251347313718519 ) ) ;
#44926=CARTESIAN_POINT ( 'NONE',  ( -2.500000000000000444, -82.16666666666667140, -4.330127018922193649 ) ) ;
#44927=FACE_OUTER_BOUND ( 'NONE', #58140, .T. ) ;
#44929=CARTESIAN_POINT ( 'NONE',  ( -5.000000000000000000, -88.87499999726880162, 0.000000000000000000 ) ) ;
#44931=ORIENTED_EDGE ( 'NONE', *, *, #20497, .T. ) ;
#44933=CARTESIAN_POINT ( 'NONE',  ( 4.458734124999998549, -24.97916666530106511, -2.574251347313721627 ) ) ;
#44935=ORIENTED_EDGE ( 'NONE', *, *, #40951, .F. ) ;
#44936=CARTESIAN_POINT ( 'NONE',  ( 3.152801135295367541, -163.5625000013656063, -3.152801135295367541 ) ) ;
#44938=CARTESIAN_POINT ( 'NONE',  ( 3.535533905932736864, -156.1250000000000000, 3.535533905932738641 ) ) ;
#44941=CARTESIAN_POINT ( 'NONE',  ( 4.458734124999998549, -76.97916666530106511, -2.574251347313721627 ) ) ;
#44944=CARTESIAN_POINT ( 'NONE',  ( -1.846868145590737420, -141.0000000013655779, 4.458734124999997661 ) ) ;
#44945=AXIS2_PLACEMENT_3D ( 'NONE', #3115, #61971, #51045 ) ;
#44946=DIRECTION ( 'NONE',  ( -0.8660254037844410391, -0.4999999999999958367, -0.000000000000000000 ) ) ;
#44948=CARTESIAN_POINT ( 'NONE',  ( -1.339745962155610925, 0.2053418012614791066, 5.000000000000000000 ) ) ;
#44950=VECTOR ( 'NONE', #39677, 1000.000000000000000 ) ;
#44952=CARTESIAN_POINT ( 'NONE',  ( 1.846868145590736310, -139.8750000013656063, 4.458734124999999437 ) ) ;
#44957=CARTESIAN_POINT ( 'NONE',  ( 4.458734124999998549, -71.97916666530107932, -2.574251347313721627 ) ) ;
#44958=CARTESIAN_POINT ( 'NONE',  ( -3.535533905932737309, -166.6250000000000284, -3.535533905932738197 ) ) ;
#44959=CARTESIAN_POINT ( 'NONE',  ( 1.975475456537005874E-15, -0.6249999972688137229, 5.000000000000000000 ) ) ;
#44964=CARTESIAN_POINT ( 'NONE',  ( -4.999999999999998224, -14.79166666393548546, 2.886751345948131764 ) ) ;
#44968=CARTESIAN_POINT ( 'NONE',  ( -4.458734124999999437, 18.43750000136559564, 0.000000000000000000 ) ) ;
#44969=CARTESIAN_POINT ( 'NONE',  ( 2.626220312808019583E-14, 21.75000000000000000, -5.000000000000000000 ) ) ;
#44975=CARTESIAN_POINT ( 'NONE',  ( 9.457646018065525792E-16, -2.062499998634406584, 5.148502694627439702 ) ) ;
#44978=CARTESIAN_POINT ( 'NONE',  ( -4.458734124999999437, -29.64583333196773651, -2.574251347313719407 ) ) ;
#44982=CARTESIAN_POINT ( 'NONE',  ( 2.229367062499998831, 28.35416666803225993, -3.861377020970580887 ) ) ;
#44986=CARTESIAN_POINT ( 'NONE',  ( -2.229367062500000163, -80.72916666530106511, -3.861377020970580443 ) ) ;
#44989=CARTESIAN_POINT ( 'NONE',  ( -2.500000000000000444, 21.95833333606451987, -4.330127018922193649 ) ) ;
#44991=DIRECTION ( 'NONE',  ( 0.000000000000000000, 0.000000000000000000, 1.000000000000000000 ) ) ;
#44994=CARTESIAN_POINT ( 'NONE',  ( 1.060575238724906964E-15, -20.74999999999999645, 5.773502691896257311 ) ) ;
#44995=CARTESIAN_POINT ( 'NONE',  ( -2.229367062499996610, -20.14583333196774007, 3.861377020970582219 ) ) ;
#44997=CARTESIAN_POINT ( 'NONE',  ( -4.458734124999999437, -80.39583333196773651, -2.574251347313719407 ) ) ;
#44998=CARTESIAN_POINT ( 'NONE',  ( -4.999999999999999112, -22.79166666393548013, 2.886751345948131764 ) ) ;
#44999=CARTESIAN_POINT ( 'NONE',  ( 2.229367062500001939, -51.97916666530107221, 3.861377020970579999 ) ) ;
#45001=CARTESIAN_POINT ( 'NONE',  ( -6.972266317189433020E-16, -74.12499999726878741, -5.000000000000000000 ) ) ;
#45002=CARTESIAN_POINT ( 'NONE',  ( 4.458734124999998549, -4.979166665301072214, -2.574251347313721627 ) ) ;
#45005=CARTESIAN_POINT ( 'NONE',  ( -4.999999999999999112, -64.91666666666667140, 2.886751345948131764 ) ) ;
#45006=CARTESIAN_POINT ( 'NONE',  ( 4.458734124999999437, -150.7500000013655779, 1.846868145590737864 ) ) ;
#45008=LINE ( 'NONE', #50481, #26587 ) ;
#45009=CARTESIAN_POINT ( 'NONE',  ( 3.535533905932738197, -157.8750000000000284, -3.535533905932738197 ) ) ;
#45010=CARTESIAN_POINT ( 'NONE',  ( -5.000000000000000000, 7.041666669397852019, -2.886751345948128211 ) ) ;
#45012=CARTESIAN_POINT ( 'NONE',  ( -2.229367062500000163, -9.729166665301068662, -3.861377020970580443 ) ) ;
#45013=CARTESIAN_POINT ( 'NONE',  ( -3.152548672688508926E-16, -44.81249999863440792, -5.148502694627439702 ) ) ;
#45015=CARTESIAN_POINT ( 'NONE',  ( 4.458734124999999437, -144.4375000013656063, 0.000000000000000000 ) ) ;
#45018=ORIENTED_EDGE ( 'NONE', *, *, #50916, .T. ) ;
#45019=DIRECTION ( 'NONE',  ( 0.000000000000000000, 0.000000000000000000, 1.000000000000000000 ) ) ;
#45020=CARTESIAN_POINT ( 'NONE',  ( -3.152548672688508926E-16, 28.18750000136559564, -5.148502694627439702 ) ) ;
#45025=EDGE_CURVE ( 'NONE', #20174, #59584, #26688, .T. ) ;
#45026=CARTESIAN_POINT ( 'NONE',  ( -6.972266317189433020E-16, -31.12499999726880873, -5.000000000000000000 ) ) ;
#45029=CARTESIAN_POINT ( 'NONE',  ( -2.229367062500000163, -7.479166665301073991, -3.861377020970580443 ) ) ;
#45030=CARTESIAN_POINT ( 'NONE',  ( 1.846868145590735200, -147.2500000013656063, -4.458734124999999437 ) ) ;
#45032=EDGE_LOOP ( 'NONE', ( #19598, #53922, #33779, #8782 ) ) ;
#45033=CYLINDRICAL_SURFACE ( 'NONE', #12030, 5.000000000000000000 ) ;
#45037=DIRECTION ( 'NONE',  ( -0.000000000000000000, 1.000000000000000000, -0.000000000000000000 ) ) ;
#45038=( BOUNDED_CURVE ( )  B_SPLINE_CURVE ( 2, ( #40841, #11576, #1634, #16413, #10617, #60168, #21235, #5482, #44706 ),
 .UNSPECIFIED., .F., .F. ) 
 B_SPLINE_CURVE_WITH_KNOTS ( ( 3, 2, 2, 2, 3 ),
 ( 0.9520833333333332815, 0.9527777777777777235, 0.9541666666666667185, 0.9555555555555556024, 0.9562500000000000444 ),
 .UNSPECIFIED. ) 
 CURVE ( )  GEOMETRIC_REPRESENTATION_ITEM ( )  RATIONAL_B_SPLINE_CURVE ( ( 0.9330127018922194093, 0.9330127018922194093, 1.000000000000000000, 0.8660254037844387076, 1.000000000000000000, 0.8660254037844387076, 1.000000000000000000, 0.9330127018922194093, 0.9330127018922194093 ) ) 
 REPRESENTATION_ITEM ( '' )  );
#45043=DIRECTION ( 'NONE',  ( -0.000000000000000000, 1.000000000000000000, -0.000000000000000000 ) ) ;
#45045=CARTESIAN_POINT ( 'NONE',  ( -2.229367062499996610, 10.85416666803225993, 3.861377020970582219 ) ) ;
#45048=CARTESIAN_POINT ( 'NONE',  ( 9.457646018065525792E-16, -13.31249999863440259, 5.148502694627439702 ) ) ;
#45050=CARTESIAN_POINT ( 'NONE',  ( -4.458734125000001214, -164.8750000013655779, 1.846868145590734089 ) ) ;
#45057=CARTESIAN_POINT ( 'NONE',  ( 2.071067811865517694, -141.9375000027312126, -4.999999999999958256 ) ) ;
#45058=CARTESIAN_POINT ( 'NONE',  ( 2.500000000000002220, -69.66666666666667140, 4.330127018922192761 ) ) ;
#45060=CARTESIAN_POINT ( 'NONE',  ( -4.458734125000000326, -149.1250000013656063, 1.846868145590734089 ) ) ;
#45062=CARTESIAN_POINT ( 'NONE',  ( -5.000000000000000000, -14.08333333333333037, -2.886751345948128211 ) ) ;
#45063=CARTESIAN_POINT ( 'NONE',  ( 1.339745962155612702, -68.16965819600733312, -5.000000000000000000 ) ) ;
#45064=ORIENTED_EDGE ( 'NONE', *, *, #95, .T. ) ;
#45067=CYLINDRICAL_SURFACE ( 'NONE', #37062, 5.000000000000000000 ) ;
#45068=CARTESIAN_POINT ( 'NONE',  ( 2.499999999999998668, -1.333333333333332149, -4.330127018922193649 ) ) ;
#45069=CARTESIAN_POINT ( 'NONE',  ( 4.458734124999999437, -64.81249999863440792, -5.460374474430324690E-16 ) ) ;
#45071=CARTESIAN_POINT ( 'NONE',  ( 1.060575238724906964E-15, -9.624999997268814056, 5.773502691896257311 ) ) ;
#45072=CARTESIAN_POINT ( 'NONE',  ( 9.457646018065525792E-16, -34.06249999863440792, 5.148502694627439702 ) ) ;
#45074=CARTESIAN_POINT ( 'NONE',  ( -6.972266317189433020E-16, -78.24999999999998579, -5.000000000000000000 ) ) ;
#45076=ORIENTED_EDGE ( 'NONE', *, *, #47630, .F. ) ;
#45078=CARTESIAN_POINT ( 'NONE',  ( -2.500000000000000444, -48.16666666666666430, -4.330127018922193649 ) ) ;
#45079=CARTESIAN_POINT ( 'NONE',  ( 5.000000000000000000, -46.37499999726880873, -6.123233995736766282E-16 ) ) ;
#45081=AXIS2_PLACEMENT_3D ( 'NONE', #40563, #1041, #15811 ) ;
#45083=CARTESIAN_POINT ( 'NONE',  ( 2.229367062500001939, -75.97916666530106511, 3.861377020970579999 ) ) ;
#45084=CARTESIAN_POINT ( 'NONE',  ( -3.535533905932737309, -168.6250000000000284, -3.535533905932738197 ) ) ;
#45085=CARTESIAN_POINT ( 'NONE',  ( -4.458734124999999437, -79.39583333196773651, -2.574251347313719407 ) ) ;
#45086=EDGE_CURVE ( 'NONE', #176, #7443, #61427, .T. ) ;
#45088=CARTESIAN_POINT ( 'NONE',  ( -2.229367062499996610, -31.39583333196773651, 3.861377020970582219 ) ) ;
#45090=LINE ( 'NONE', #50233, #5325 ) ;
#45093=CARTESIAN_POINT ( 'NONE',  ( -4.999999999999998224, 22.20833333606451987, 2.886751345948131764 ) ) ;
#45096=CARTESIAN_POINT ( 'NONE',  ( -1.339745962155610925, -75.66965819600731891, 5.000000000000000000 ) ) ;
#45097=CARTESIAN_POINT ( 'NONE',  ( -4.458734124999998549, -64.47916666530106511, 2.574251347313722516 ) ) ;
#45099=VERTEX_POINT ( 'NONE', #42726 ) ;
#45100=CARTESIAN_POINT ( 'NONE',  ( 2.499999999999998668, -62.33333333333333570, -4.330127018922193649 ) ) ;
#45101=CYLINDRICAL_SURFACE ( 'NONE', #13042, 5.000000000000000000 ) ;
#45102=CARTESIAN_POINT ( 'NONE',  ( 2.229367062499998831, 15.35416666803225993, -3.861377020970580887 ) ) ;
#45105=CARTESIAN_POINT ( 'NONE',  ( 2.730187237215162345E-16, -162.1875000013655779, -4.458734124999999437 ) ) ;
#45106=( BOUNDED_CURVE ( )  B_SPLINE_CURVE ( 2, ( #54050, #63404, #3917, #28345, #47962, #13870, #9987, #38617, #29275 ),
 .UNSPECIFIED., .F., .F. ) 
 B_SPLINE_CURVE_WITH_KNOTS ( ( 3, 2, 2, 2, 3 ),
 ( 0.8479166666666666519, 0.8486111111111110938, 0.8499999999999999778, 0.8513888888888888618, 0.8520833333333333037 ),
 .UNSPECIFIED. ) 
 CURVE ( )  GEOMETRIC_REPRESENTATION_ITEM ( )  RATIONAL_B_SPLINE_CURVE ( ( 0.9330127018922194093, 0.9330127018922194093, 1.000000000000000000, 0.8660254037844387076, 1.000000000000000000, 0.8660254037844387076, 1.000000000000000000, 0.9330127018922194093, 0.9330127018922194093 ) ) 
 REPRESENTATION_ITEM ( '' )  );
#45107=CARTESIAN_POINT ( 'NONE',  ( -1.339745962155610925, 19.33034180399266688, 5.000000000000000000 ) ) ;
#45112=CARTESIAN_POINT ( 'NONE',  ( 1.339745962155612258, 25.41965820146970501, 5.000000000000000888 ) ) ;
#45113=CARTESIAN_POINT ( 'NONE',  ( 5.000000000000000888, -36.58333333333332149, 2.886751345948126879 ) ) ;
#45116=CARTESIAN_POINT ( 'NONE',  ( 1.975475456537005874E-15, -72.62499999726878741, 5.000000000000000000 ) ) ;
#45117=CARTESIAN_POINT ( 'NONE',  ( -5.000000000000000000, -82.87499999726881583, 0.000000000000000000 ) ) ;
#45118=CARTESIAN_POINT ( 'NONE',  ( 5.000000000000000888, -58.58333333333333570, 2.886751345948126879 ) ) ;
#45121=CARTESIAN_POINT ( 'NONE',  ( -3.152548672688508926E-16, 4.187500001365595637, -5.148502694627439702 ) ) ;
#45124=CARTESIAN_POINT ( 'NONE',  ( -2.071067811865475061, -143.8125000027312126, -5.000000000000000888 ) ) ;
#45125=LINE ( 'NONE', #39649, #24321 ) ;
#45133=CARTESIAN_POINT ( 'NONE',  ( 1.846868145590736310, -166.8750000013656063, 4.458734124999997661 ) ) ;
#45137=CARTESIAN_POINT ( 'NONE',  ( 4.458734124999999437, -140.4375000013656063, 0.000000000000000000 ) ) ;
#45138=ORIENTED_EDGE ( 'NONE', *, *, #5090, .F. ) ;
#45139=CARTESIAN_POINT ( 'NONE',  ( 9.457646018065525792E-16, 20.68750000136559564, 5.148502694627439702 ) ) ;
#45141=CARTESIAN_POINT ( 'NONE',  ( 2.229367062500001939, -62.22916666530106511, 3.861377020970579999 ) ) ;
#45145=CARTESIAN_POINT ( 'NONE',  ( -2.499999999999996447, 14.16666666666666785, 4.330127018922195425 ) ) ;
#45146=CARTESIAN_POINT ( 'NONE',  ( 9.457646018065525792E-16, -52.06249999863440792, 5.148502694627439702 ) ) ;
#45147=CARTESIAN_POINT ( 'NONE',  ( 2.229367062499998831, -9.645833331967738289, -3.861377020970580887 ) ) ;
#45148=CARTESIAN_POINT ( 'NONE',  ( 2.071067811865443975, -165.9375000027311557, -5.000000000000031974 ) ) ;
#45149=CARTESIAN_POINT ( 'NONE',  ( -4.999999999999998224, -63.79166666393547303, 2.886751345948131764 ) ) ;
#45155=CARTESIAN_POINT ( 'NONE',  ( -3.535533905932738641, -140.5000000027311842, 3.535533905932737309 ) ) ;
#45156=CARTESIAN_POINT ( 'NONE',  ( 9.457646018065525792E-16, -60.06249999863440792, 5.148502694627439702 ) ) ;
#45157=CARTESIAN_POINT ( 'NONE',  ( -4.458734125000000326, -156.2500000013656063, -1.846868145590735644 ) ) ;
#45158=ADVANCED_FACE ( 'NONE', ( #51766 ), #62371, .T. ) ;
#45159=CARTESIAN_POINT ( 'NONE',  ( 5.000000000000000888, -56.45833333060213732, 2.886751345948126879 ) ) ;
#45160=VERTEX_POINT ( 'NONE', #17671 ) ;
#45162=CARTESIAN_POINT ( 'NONE',  ( -4.458734124999999437, 1.437500001365592972, 0.000000000000000000 ) ) ;
#45163=ORIENTED_EDGE ( 'NONE', *, *, #9167, .F. ) ;
#45164=CYLINDRICAL_SURFACE ( 'NONE', #9130, 5.000000000000000000 ) ;
#45166=CARTESIAN_POINT ( 'NONE',  ( 2.730187237215162345E-16, -157.1875000013655779, -4.458734124999999437 ) ) ;
#45173=CARTESIAN_POINT ( 'NONE',  ( 4.458734125000001214, -49.14583333196772941, 2.574251347313718519 ) ) ;
#45174=VERTEX_POINT ( 'NONE', #48502 ) ;
#45175=CARTESIAN_POINT ( 'NONE',  ( 1.975475456537005874E-15, 10.37500000273118417, 5.000000000000000000 ) ) ;
#45176=EDGE_CURVE ( 'NONE', #26085, #11102, #34337, .T. ) ;
#45178=CARTESIAN_POINT ( 'NONE',  ( 4.458734124999999437, 29.18750000136559208, -5.460374474430324690E-16 ) ) ;
#45185=CARTESIAN_POINT ( 'NONE',  ( 1.975475456537005874E-15, -78.62499999726881583, 5.000000000000000000 ) ) ;
#45186=CARTESIAN_POINT ( 'NONE',  ( -2.499999999999996447, -26.83333333333333570, 4.330127018922195425 ) ) ;
#45189=CARTESIAN_POINT ( 'NONE',  ( 1.339745962155612702, -42.16965819600732601, -5.000000000000000000 ) ) ;
#45190=DIRECTION ( 'NONE',  ( 0.000000000000000000, 0.000000000000000000, 1.000000000000000000 ) ) ;
#45191=CARTESIAN_POINT ( 'NONE',  ( 4.458734125000001214, -89.14583333196775072, 2.574251347313718519 ) ) ;
#45192=DIRECTION ( 'NONE',  ( -0.000000000000000000, 1.000000000000000000, -0.000000000000000000 ) ) ;
#45197=CARTESIAN_POINT ( 'NONE',  ( 5.000000000000000000, -159.1875000027312410, 2.071067811865478614 ) ) ;
#45198=ORIENTED_EDGE ( 'NONE', *, *, #38048, .T. ) ;
#45200=CARTESIAN_POINT ( 'NONE',  ( 3.061616997868383141E-16, -162.8750000027311842, -5.000000000000000000 ) ) ;
#45210=CARTESIAN_POINT ( 'NONE',  ( 2.229367062499998831, -17.64583333196773651, -3.861377020970580887 ) ) ;
#45211=CARTESIAN_POINT ( 'NONE',  ( -6.972266317189433020E-16, 3.875000002731185500, -5.000000000000000000 ) ) ;
#45212=CARTESIAN_POINT ( 'NONE',  ( 3.061616997868383141E-16, -149.7500000000000284, -5.000000000000000000 ) ) ;
#45214=CARTESIAN_POINT ( 'NONE',  ( 4.458734125000000326, -156.3750000013655779, -1.846868145590734978 ) ) ;
#45215=ORIENTED_EDGE ( 'NONE', *, *, #20076, .T. ) ;
#45217=CARTESIAN_POINT ( 'NONE',  ( -4.458734124999997661, -44.47916666530106511, 2.574251347313722516 ) ) ;
#45220=CARTESIAN_POINT ( 'NONE',  ( -5.000000000000000000, 27.99999999999999645, 0.000000000000000000 ) ) ;
#45222=CARTESIAN_POINT ( 'NONE',  ( 4.458734124999999437, 2.187500001365593416, -5.460374474430324690E-16 ) ) ;
#45224=CARTESIAN_POINT ( 'NONE',  ( 5.000000000000000888, -82.58333333333334281, 2.886751345948126879 ) ) ;
#45225=CARTESIAN_POINT ( 'NONE',  ( 2.229367062500001939, 19.77083333469892779, 3.861377020970579999 ) ) ;
#45227=CARTESIAN_POINT ( 'NONE',  ( -2.499999999999996447, 8.291666669397852019, 4.330127018922195425 ) ) ;
#45229=CARTESIAN_POINT ( 'NONE',  ( 1.975475456537005874E-15, -30.74999999999999645, 5.000000000000000000 ) ) ;
#45232=CARTESIAN_POINT ( 'NONE',  ( 2.229367062499998831, -42.64583333196773651, -3.861377020970580887 ) ) ;
#45235=CARTESIAN_POINT ( 'NONE',  ( -3.535250795749689387E-16, -41.12499999726880162, -5.773502691896257311 ) ) ;
#45236=EDGE_CURVE ( 'NONE', #4902, #52130, #62340, .T. ) ;
#45238=CARTESIAN_POINT ( 'NONE',  ( 4.458734125000001214, -17.89583333196774007, 2.574251347313718519 ) ) ;
#45239=ORIENTED_EDGE ( 'NONE', *, *, #51539, .F. ) ;
#45240=CARTESIAN_POINT ( 'NONE',  ( -3.535250795749689387E-16, -81.25000000000001421, -5.773502691896257311 ) ) ;
#45241=CARTESIAN_POINT ( 'NONE',  ( 1.846868145590735200, -168.2500000013656063, -4.458734125000000326 ) ) ;
#45242=CARTESIAN_POINT ( 'NONE',  ( 5.000000000000000888, -86.45833333060213022, 2.886751345948126879 ) ) ;
#45244=VERTEX_POINT ( 'NONE', #53961 ) ;
#45246=CARTESIAN_POINT ( 'NONE',  ( -2.229367062500000163, -27.72916666530107221, -3.861377020970580443 ) ) ;
#45247=CARTESIAN_POINT ( 'NONE',  ( -6.972266317189433020E-16, -50.24999999999999289, -5.000000000000000000 ) ) ;
#45249=ORIENTED_EDGE ( 'NONE', *, *, #38099, .T. ) ;
#45251=CARTESIAN_POINT ( 'NONE',  ( -4.458734125000001214, -164.1250000013656063, 1.846868145590734089 ) ) ;
#45254=DIRECTION ( 'NONE',  ( 0.000000000000000000, 0.000000000000000000, 1.000000000000000000 ) ) ;
#45256=CARTESIAN_POINT ( 'NONE',  ( -4.999999999999998224, -25.91666666666666430, 2.886751345948131764 ) ) ;
#45258=CARTESIAN_POINT ( 'NONE',  ( -3.152548672688508926E-16, -73.81249999863440792, -5.148502694627439702 ) ) ;
#45261=CARTESIAN_POINT ( 'NONE',  ( -8.190561711645485556E-16, -141.9375000013656063, 4.458734124999999437 ) ) ;
#45263=AXIS2_PLACEMENT_3D ( 'NONE', #54405, #1352, #25447 ) ;
#45267=CARTESIAN_POINT ( 'NONE',  ( -1.846868145590737420, -142.0000000013655495, 4.458734124999999437 ) ) ;
#45270=CARTESIAN_POINT ( 'NONE',  ( 0.000000000000000000, -170.0000000000000000, 0.000000000000000000 ) ) ;
#45272=CARTESIAN_POINT ( 'NONE',  ( 4.458734124999999437, -75.06249999863440792, -5.460374474430324690E-16 ) ) ;
#45273=CARTESIAN_POINT ( 'NONE',  ( 6.123233995736766282E-16, -170.0000000000000000, -5.000000000000000000 ) ) ;
#45274=DIRECTION ( 'NONE',  ( -0.000000000000000000, 1.000000000000000000, -0.000000000000000000 ) ) ;
#45277=DIRECTION ( 'NONE',  ( -0.000000000000000000, 1.000000000000000000, -0.000000000000000000 ) ) ;
#45278=CARTESIAN_POINT ( 'NONE',  ( -5.000000000000000000, -60.08333333333333570, -2.886751345948128211 ) ) ;
#45283=CARTESIAN_POINT ( 'NONE',  ( 4.458734124999999437, 16.93750000136559564, -5.460374474430324690E-16 ) ) ;
#45284=CARTESIAN_POINT ( 'NONE',  ( 1.975475456537005874E-15, -42.62499999726880873, 5.000000000000000000 ) ) ;
#45289=( BOUNDED_CURVE ( )  B_SPLINE_CURVE ( 2, ( #47309, #17415, #3262, #11616, #27362, #7448, #2000, #62108, #46996 ),
 .UNSPECIFIED., .F., .F. ) 
 B_SPLINE_CURVE_WITH_KNOTS ( ( 3, 2, 2, 2, 3 ),
 ( 0.8249999999999997335, 0.8291666666666664964, 0.8333333333333331483, 0.8374999999999998002, 0.8416666666666664520 ),
 .UNSPECIFIED. ) 
 CURVE ( )  GEOMETRIC_REPRESENTATION_ITEM ( )  RATIONAL_B_SPLINE_CURVE ( ( 1.000000000000003997, 0.9238795325112826307, 1.000000000000000000, 0.9238795325112867385, 1.000000000000000000, 0.9238795325112867385, 1.000000000000000000, 0.9238795325112908463, 0.9999999999999958922 ) ) 
 REPRESENTATION_ITEM ( '' )  );
#45291=CARTESIAN_POINT ( 'NONE',  ( 4.458734124999999437, -84.81249999863439371, -5.460374474430324690E-16 ) ) ;
#45292=CARTESIAN_POINT ( 'NONE',  ( 4.458734124999999437, -5.812499998634403475, -5.460374474430324690E-16 ) ) ;
#45294=CARTESIAN_POINT ( 'NONE',  ( 4.458734124999998549, -27.97916666530107221, -2.574251347313721627 ) ) ;
#45298=CARTESIAN_POINT ( 'NONE',  ( -3.152548672688508926E-16, 19.43750000136559208, -5.148502694627439702 ) ) ;
#45301=CARTESIAN_POINT ( 'NONE',  ( -4.458734124999999437, -79.64583333196773651, -2.574251347313719407 ) ) ;
#45304=CARTESIAN_POINT ( 'NONE',  ( 5.000000000000000000, 26.70833333606451632, -2.886751345948129988 ) ) ;
#45306=DIRECTION ( 'NONE',  ( -0.000000000000000000, 1.000000000000000000, -0.000000000000000000 ) ) ;
#45309=CARTESIAN_POINT ( 'NONE',  ( 5.000000000000000888, -18.58333333333333215, 2.886751345948126879 ) ) ;
#45310=CARTESIAN_POINT ( 'NONE',  ( -4.458734124999999437, -20.31249999863440081, 0.000000000000000000 ) ) ;
#45312=CARTESIAN_POINT ( 'NONE',  ( -2.229367062499996610, -88.14583333196773651, 3.861377020970582219 ) ) ;
#45313=ADVANCED_FACE ( 'NONE', ( #14088 ), #19865, .T. ) ;
#45314=CARTESIAN_POINT ( 'NONE',  ( -2.500000000000000444, -25.04166666393547658, -4.330127018922193649 ) ) ;
#45315=CARTESIAN_POINT ( 'NONE',  ( 2.229367062500001939, -54.97916666530107221, 3.861377020970579999 ) ) ;
#45316=ORIENTED_EDGE ( 'NONE', *, *, #51601, .T. ) ;
#45318=DIRECTION ( 'NONE',  ( 0.000000000000000000, 0.000000000000000000, 1.000000000000000000 ) ) ;
#45319=CARTESIAN_POINT ( 'NONE',  ( -4.458734124999999437, -3.562499998634407916, 0.000000000000000000 ) ) ;
#45323=CARTESIAN_POINT ( 'NONE',  ( 2.499999999999998668, -65.33333333333332860, -4.330127018922193649 ) ) ;
#45324=CARTESIAN_POINT ( 'NONE',  ( -4.458734125000001214, -152.1250000013655779, 1.846868145590734089 ) ) ;
#45327=CARTESIAN_POINT ( 'NONE',  ( -2.071067811865475061, -157.6875000000000000, -5.000000000000000888 ) ) ;
#45330=CARTESIAN_POINT ( 'NONE',  ( 2.229367062499998831, -11.89583333196774007, -3.861377020970580887 ) ) ;
#45331=CARTESIAN_POINT ( 'NONE',  ( -4.458734124999998549, -51.47916666530106511, 2.574251347313722516 ) ) ;
#45333=CARTESIAN_POINT ( 'NONE',  ( -3.152801135295367096, -144.0625000013655779, -3.152801135295367541 ) ) ;
#45336=VERTEX_POINT ( 'NONE', #47866 ) ;
#45337=EDGE_CURVE ( 'NONE', #50505, #18747, #3825, .T. ) ;
#45338=DIRECTION ( 'NONE',  ( -0.000000000000000000, 1.000000000000000000, -0.000000000000000000 ) ) ;
#45339=CARTESIAN_POINT ( 'NONE',  ( 4.458734125000001214, 25.85416666803225638, 2.574251347313718519 ) ) ;
#45341=( BOUNDED_CURVE ( )  B_SPLINE_CURVE ( 2, ( #28985, #19341, #43465, #38338, #19022, #34131, #24810, #29293, #62794 ),
 .UNSPECIFIED., .F., .F. ) 
 B_SPLINE_CURVE_WITH_KNOTS ( ( 3, 2, 2, 2, 3 ),
 ( 0.2250000000000001998, 0.2291666666666668517, 0.2333333333333335313, 0.2375000000000001832, 0.2416666666666668628 ),
 .UNSPECIFIED. ) 
 CURVE ( )  GEOMETRIC_REPRESENTATION_ITEM ( )  RATIONAL_B_SPLINE_CURVE ( ( 0.9999999999999964473, 0.9238795325112902912, 1.000000000000000000, 0.9238795325112867385, 1.000000000000000000, 0.9238795325112867385, 1.000000000000000000, 0.9238795325112831858, 1.000000000000003553 ) ) 
 REPRESENTATION_ITEM ( '' )  );
#45343=CARTESIAN_POINT ( 'NONE',  ( -5.000000000000000000, -62.00000000000000000, 0.000000000000000000 ) ) ;
#45350=CARTESIAN_POINT ( 'NONE',  ( -4.458734124999998549, -7.229166665301073103, 2.574251347313722516 ) ) ;
#45351=CARTESIAN_POINT ( 'NONE',  ( 2.499999999999998668, 6.791666669397851130, -4.330127018922193649 ) ) ;
#45352=CARTESIAN_POINT ( 'NONE',  ( -1.846868145590737420, -150.7500000013656347, 4.458734124999997661 ) ) ;
#45354=ORIENTED_EDGE ( 'NONE', *, *, #43803, .F. ) ;
#45355=CARTESIAN_POINT ( 'NONE',  ( -5.000000000000000888, -148.4375000000000000, 2.071067811865474617 ) ) ;
#45365=FACE_OUTER_BOUND ( 'NONE', #42664, .T. ) ;
#45366=CARTESIAN_POINT ( 'NONE',  ( 9.457646018065525792E-16, 9.937500001365593860, 5.148502694627439702 ) ) ;
#45368=ORIENTED_EDGE ( 'NONE', *, *, #61823, .T. ) ;
#45369=CARTESIAN_POINT ( 'NONE',  ( 4.458734124999998549, -11.97916666530107044, -2.574251347313721627 ) ) ;
#45371=CARTESIAN_POINT ( 'NONE',  ( 3.152801135295366208, -165.5625000013656063, 3.152801135295367985 ) ) ;
#45372=CARTESIAN_POINT ( 'NONE',  ( -1.339745962155610925, -40.66965819600732601, 5.000000000000000000 ) ) ;
#45379=DIRECTION ( 'NONE',  ( 0.000000000000000000, 0.000000000000000000, 1.000000000000000000 ) ) ;
#45380=CARTESIAN_POINT ( 'NONE',  ( -4.458734124999999437, -149.2500000013656063, -1.846868145590735644 ) ) ;
#45382=CARTESIAN_POINT ( 'NONE',  ( -5.000000000000000000, -57.95833333060216574, -2.886751345948128211 ) ) ;
#45386=CARTESIAN_POINT ( 'NONE',  ( -2.499999999999996447, -8.708333330602144429, 4.330127018922195425 ) ) ;
#45387=CARTESIAN_POINT ( 'NONE',  ( -5.000000000000000000, -3.999999999999996447, 0.000000000000000000 ) ) ;
#45388=CARTESIAN_POINT ( 'NONE',  ( -4.458734124999997661, -64.22916666530106511, 2.574251347313722516 ) ) ;
#45389=EDGE_CURVE ( 'NONE', #7044, #61101, #7678, .T. ) ;
#45390=CARTESIAN_POINT ( 'NONE',  ( -4.999999999999998224, -16.91666666666666430, 2.886751345948131764 ) ) ;
#45391=CARTESIAN_POINT ( 'NONE',  ( 2.500000000000002220, -6.541666663935481019, 4.330127018922192761 ) ) ;
#45392=CARTESIAN_POINT ( 'NONE',  ( 9.457646018065525792E-16, -36.06249999863441502, 5.148502694627439702 ) ) ;
#45395=FACE_OUTER_BOUND ( 'NONE', #1529, .T. ) ;
#45396=CARTESIAN_POINT ( 'NONE',  ( 9.457646018065525792E-16, 10.68750000136559386, 5.148502694627439702 ) ) ;
#45397=ORIENTED_EDGE ( 'NONE', *, *, #35407, .F. ) ;
#45399=CARTESIAN_POINT ( 'NONE',  ( -2.499999999999996447, -52.83333333333332860, 4.330127018922195425 ) ) ;
#45402=CARTESIAN_POINT ( 'NONE',  ( -2.229367062500000163, -76.47916666530106511, -3.861377020970580443 ) ) ;
#45403=CARTESIAN_POINT ( 'NONE',  ( -4.458734125000001214, -140.1250000013655779, 1.846868145590734089 ) ) ;
#45404=CARTESIAN_POINT ( 'NONE',  ( 2.229367062499998831, -79.64583333196773651, -3.861377020970580887 ) ) ;
#45406=CARTESIAN_POINT ( 'NONE',  ( -2.229367062500000163, -35.72916666530107221, -3.861377020970580443 ) ) ;
#45409=ORIENTED_EDGE ( 'NONE', *, *, #34284, .T. ) ;
#45416=CARTESIAN_POINT ( 'NONE',  ( 4.458734124999999437, -64.06249999863440792, -5.460374474430324690E-16 ) ) ;
#45418=EDGE_LOOP ( 'NONE', ( #33462, #18008, #15496, #32950 ) ) ;
#45419=( BOUNDED_CURVE ( )  B_SPLINE_CURVE ( 2, ( #38583, #23500, #63056, #52768, #8697, #52462, #48557, #9320, #28309 ),
 .UNSPECIFIED., .F., .F. ) 
 B_SPLINE_CURVE_WITH_KNOTS ( ( 3, 2, 2, 2, 3 ),
 ( 0.05833333333333338283, 0.06250000000000005551, 0.06666666666666672125, 0.07083333333333338699, 0.07500000000000005274 ),
 .UNSPECIFIED. ) 
 CURVE ( )  GEOMETRIC_REPRESENTATION_ITEM ( )  RATIONAL_B_SPLINE_CURVE ( ( 0.9999999999999991118, 0.9238795325112876267, 1.000000000000000000, 0.9238795325112867385, 1.000000000000000000, 0.9238795325112867385, 1.000000000000000000, 0.9238795325112857393, 1.000000000000001110 ) ) 
 REPRESENTATION_ITEM ( '' )  );
#45420=CARTESIAN_POINT ( 'NONE',  ( -2.499999999999996447, 5.291666669397853795, 4.330127018922195425 ) ) ;
#45421=FACE_OUTER_BOUND ( 'NONE', #1995, .T. ) ;
#45422=CARTESIAN_POINT ( 'NONE',  ( -2.229367062500000163, 5.520833334698927786, -3.861377020970580443 ) ) ;
#45425=CARTESIAN_POINT ( 'NONE',  ( 4.458734124999997661, -161.5000000013656063, 1.846868145590737864 ) ) ;
#45427=VERTEX_POINT ( 'NONE', #49459 ) ;
#45429=CARTESIAN_POINT ( 'NONE',  ( 5.000000000000000888, -164.0625000027312410, -2.071067811865475505 ) ) ;
#45431=DIRECTION ( 'NONE',  ( -0.000000000000000000, 1.000000000000000000, -0.000000000000000000 ) ) ;
#45432=( BOUNDED_CURVE ( )  B_SPLINE_CURVE ( 2, ( #26727, #32491, #27042, #12557, #1985, #46659, #2604, #22543, #13192 ),
 .UNSPECIFIED., .F., .F. ) 
 B_SPLINE_CURVE_WITH_KNOTS ( ( 3, 2, 2, 2, 3 ),
 ( 0.8062500000000000222, 0.8069444444444444642, 0.8083333333333333481, 0.8097222222222222321, 0.8104166666666666741 ),
 .UNSPECIFIED. ) 
 CURVE ( )  GEOMETRIC_REPRESENTATION_ITEM ( )  RATIONAL_B_SPLINE_CURVE ( ( 0.9330127018922194093, 0.9330127018922194093, 1.000000000000000000, 0.8660254037844387076, 1.000000000000000000, 0.8660254037844387076, 1.000000000000000000, 0.9330127018922194093, 0.9330127018922194093 ) ) 
 REPRESENTATION_ITEM ( '' )  );
#45433=CARTESIAN_POINT ( 'NONE',  ( 1.975475456537005874E-15, 4.375000002731185056, 5.000000000000000000 ) ) ;
#45436=CARTESIAN_POINT ( 'NONE',  ( 6.123233995736766282E-16, -170.0000000000000000, -5.000000000000000000 ) ) ;
#45439=CARTESIAN_POINT ( 'NONE',  ( 4.458734125000000326, 28.10416666803225993, 2.574251347313718519 ) ) ;
#45442=CARTESIAN_POINT ( 'NONE',  ( -4.458734124999999437, 1.354166668032261933, -2.574251347313719407 ) ) ;
#45443=LINE ( 'NONE', #35482, #38109 ) ;
#45445=CARTESIAN_POINT ( 'NONE',  ( 3.535533905932736864, -144.2500000027311842, 3.535533905932738641 ) ) ;
#45446=DIRECTION ( 'NONE',  ( -0.000000000000000000, 1.000000000000000000, -0.000000000000000000 ) ) ;
#45450=CYLINDRICAL_SURFACE ( 'NONE', #51435, 5.000000000000000000 ) ;
#45453=CARTESIAN_POINT ( 'NONE',  ( -1.846868145590737420, -162.0000000013656063, 4.458734124999997661 ) ) ;
#45454=CARTESIAN_POINT ( 'NONE',  ( -2.499999999999996447, -32.83333333333332860, 4.330127018922195425 ) ) ;
#45455=CARTESIAN_POINT ( 'NONE',  ( 5.000000000000000000, 7.500000000000000000, -6.123233995736766282E-16 ) ) ;
#45457=CARTESIAN_POINT ( 'NONE',  ( 4.458734125000000326, -141.3750000013656063, -1.846868145590734978 ) ) ;
#45459=CARTESIAN_POINT ( 'NONE',  ( 4.458734124999998549, 22.02083333469892779, -2.574251347313721627 ) ) ;
#45460=ORIENTED_EDGE ( 'NONE', *, *, #24133, .T. ) ;
#45461=CARTESIAN_POINT ( 'NONE',  ( -2.229367062500000163, -60.72916666530106511, -3.861377020970580443 ) ) ;
#45463=CARTESIAN_POINT ( 'NONE',  ( -6.972266317189433020E-16, 2.750000000000000000, -5.000000000000000000 ) ) ;
#45464=CARTESIAN_POINT ( 'NONE',  ( 5.000000000000000000, 13.49999999999999822, -6.123233995736766282E-16 ) ) ;
#45465=CARTESIAN_POINT ( 'NONE',  ( 2.229367062499998831, -52.64583333196773651, -3.861377020970580887 ) ) ;
#45466=CARTESIAN_POINT ( 'NONE',  ( 4.458734124999998549, -9.729166665301068662, -2.574251347313721627 ) ) ;
#45467=DIRECTION ( 'NONE',  ( -0.000000000000000000, 1.000000000000000000, -0.000000000000000000 ) ) ;
#45469=CARTESIAN_POINT ( 'NONE',  ( -4.999999999999998224, -63.91666666666666430, 2.886751345948131764 ) ) ;
#45471=CARTESIAN_POINT ( 'NONE',  ( 1.060575238724906964E-15, -31.75000000000000000, 5.773502691896257311 ) ) ;
#45473=CARTESIAN_POINT ( 'NONE',  ( -6.972266317189433020E-16, -34.25000000000000000, -5.000000000000000000 ) ) ;
#45476=CARTESIAN_POINT ( 'NONE',  ( -4.458734124999999437, -58.39583333196774362, -2.574251347313719407 ) ) ;
#45477=CARTESIAN_POINT ( 'NONE',  ( -3.152801135295367985, -151.0625000013655779, 3.152801135295367096 ) ) ;
#45478=CARTESIAN_POINT ( 'NONE',  ( -4.458734124999999437, -63.39583333196772941, -2.574251347313719407 ) ) ;
#45479=CARTESIAN_POINT ( 'NONE',  ( 5.000000000000000000, -53.37499999726881583, -6.123233995736766282E-16 ) ) ;
#45482=CARTESIAN_POINT ( 'NONE',  ( -2.229367062499996610, -2.395833331967737845, 3.861377020970582219 ) ) ;
#45486=CARTESIAN_POINT ( 'NONE',  ( -3.152801135295367096, -158.0625000013656063, -3.152801135295367541 ) ) ;
#45487=ORIENTED_EDGE ( 'NONE', *, *, #47998, .F. ) ;
#45488=( BOUNDED_CURVE ( )  B_SPLINE_CURVE ( 2, ( #55624, #1284, #60449, #6093, #11220, #16374, #51107, #60765, #30844 ),
 .UNSPECIFIED., .F., .F. ) 
 B_SPLINE_CURVE_WITH_KNOTS ( ( 3, 2, 2, 2, 3 ),
 ( 0.6604166666666666519, 0.6611111111111110938, 0.6624999999999999778, 0.6638888888888888618, 0.6645833333333333037 ),
 .UNSPECIFIED. ) 
 CURVE ( )  GEOMETRIC_REPRESENTATION_ITEM ( )  RATIONAL_B_SPLINE_CURVE ( ( 0.9330127018922194093, 0.9330127018922194093, 1.000000000000000000, 0.8660254037844387076, 1.000000000000000000, 0.8660254037844387076, 1.000000000000000000, 0.9330127018922194093, 0.9330127018922194093 ) ) 
 REPRESENTATION_ITEM ( '' )  );
#45492=CARTESIAN_POINT ( 'NONE',  ( -4.458734124999999437, -46.64583333196774362, -2.574251347313719407 ) ) ;
#45494=CARTESIAN_POINT ( 'NONE',  ( -9.184850993605147944E-16, -145.2500000000000284, 5.000000000000000000 ) ) ;
#45496=CARTESIAN_POINT ( 'NONE',  ( -4.458734124999998549, 24.77083333469893134, 2.574251347313722516 ) ) ;
#45498=CARTESIAN_POINT ( 'NONE',  ( 3.061616997868383141E-16, -165.7500000000000000, -5.000000000000000000 ) ) ;
#45500=ORIENTED_EDGE ( 'NONE', *, *, #46782, .F. ) ;
#45502=CYLINDRICAL_SURFACE ( 'NONE', #42794, 5.000000000000000000 ) ;
#45504=CARTESIAN_POINT ( 'NONE',  ( -5.000000000000000000, 6.916666666666664298, -2.886751345948128211 ) ) ;
#45512=( BOUNDED_CURVE ( )  B_SPLINE_CURVE ( 2, ( #56793, #12398, #32327, #32966, #22374, #12071, #23009, #32644, #2443 ),
 .UNSPECIFIED., .F., .F. ) 
 B_SPLINE_CURVE_WITH_KNOTS ( ( 3, 2, 2, 2, 3 ),
 ( 0.6583333333333329929, 0.6624999999999996447, 0.6666666666666662966, 0.6708333333333328374, 0.6749999999999996003 ),
 .UNSPECIFIED. ) 
 CURVE ( )  GEOMETRIC_REPRESENTATION_ITEM ( )  RATIONAL_B_SPLINE_CURVE ( ( 1.000000000000005995, 0.9238795325112806323, 1.000000000000000000, 0.9238795325112867385, 1.000000000000000000, 0.9238795325112867385, 1.000000000000000000, 0.9238795325112948431, 0.9999999999999918954 ) ) 
 REPRESENTATION_ITEM ( '' )  );
#45514=ORIENTED_EDGE ( 'NONE', *, *, #62482, .T. ) ;
#45515=CARTESIAN_POINT ( 'NONE',  ( -5.000000000000000000, -163.6250000027311842, -6.123233995736766282E-16 ) ) ;
#45517=CARTESIAN_POINT ( 'NONE',  ( 5.000000000000000000, -158.1875000027312126, 2.071067811865478614 ) ) ;
#45520=EDGE_CURVE ( 'NONE', #33038, #25022, #62453, .T. ) ;
#45528=CARTESIAN_POINT ( 'NONE',  ( -3.152548672688508926E-16, -17.56249999863440792, -5.148502694627439702 ) ) ;
#45529=CARTESIAN_POINT ( 'NONE',  ( -1.339745962155610925, -79.66965819600731891, 5.000000000000000000 ) ) ;
#45530=CARTESIAN_POINT ( 'NONE',  ( 5.000000000000000888, -150.9375000000000284, -2.071067811865475505 ) ) ;
#45532=CARTESIAN_POINT ( 'NONE',  ( -4.458734124999999437, -152.9375000013655779, -5.460374474430324690E-16 ) ) ;
#45534=CARTESIAN_POINT ( 'NONE',  ( -3.152548672688508926E-16, -45.81249999863440081, -5.148502694627439702 ) ) ;
#45535=DIRECTION ( 'NONE',  ( 0.000000000000000000, 0.000000000000000000, 1.000000000000000000 ) ) ;
#45537=CARTESIAN_POINT ( 'NONE',  ( 5.000000000000000000, 27.50000000000000000, -6.123233995736766282E-16 ) ) ;
#45538=CARTESIAN_POINT ( 'NONE',  ( 9.457646018065525792E-16, 1.937500001365593416, 5.148502694627439702 ) ) ;
#45539=ADVANCED_FACE ( 'NONE', ( #50424 ), #10852, .T. ) ;
#45540=CARTESIAN_POINT ( 'NONE',  ( -1.339745962155610925, -73.66965819600733312, 5.000000000000000000 ) ) ;
#45542=CARTESIAN_POINT ( 'NONE',  ( 2.500000000000002220, -11.54166666393547835, 4.330127018922192761 ) ) ;
#45544=CARTESIAN_POINT ( 'NONE',  ( 2.229367062499998831, 15.10416666803225993, -3.861377020970580887 ) ) ;
#45546=CARTESIAN_POINT ( 'NONE',  ( -4.999999999999999112, 10.20833333606451987, 2.886751345948131764 ) ) ;
#45547=ORIENTED_EDGE ( 'NONE', *, *, #17654, .T. ) ;
#45548=CARTESIAN_POINT ( 'NONE',  ( -2.500000000000000444, 7.833333333333334814, -4.330127018922193649 ) ) ;
#45551=CARTESIAN_POINT ( 'NONE',  ( -4.458734124999999437, -44.39583333196773651, -2.574251347313719407 ) ) ;
#45552=CARTESIAN_POINT ( 'NONE',  ( -8.190561711645485556E-16, -164.9375000013655779, 4.458734124999999437 ) ) ;
#45554=CARTESIAN_POINT ( 'NONE',  ( 5.000000000000000000, -39.37499999726880162, -6.123233995736766282E-16 ) ) ;
#45556=CARTESIAN_POINT ( 'NONE',  ( -2.229367062500000163, -17.47916666530106866, -3.861377020970580443 ) ) ;
#45557=VERTEX_POINT ( 'NONE', #15044 ) ;
#45558=CARTESIAN_POINT ( 'NONE',  ( -2.500000000000000444, -86.16666666666667140, -4.330127018922193649 ) ) ;
#45559=CARTESIAN_POINT ( 'NONE',  ( -2.500000000000000444, 0.9583333360645186483, -4.330127018922193649 ) ) ;
#45560=CARTESIAN_POINT ( 'NONE',  ( -2.500000000000000444, -87.04166666393547303, -4.330127018922193649 ) ) ;
#45561=CARTESIAN_POINT ( 'NONE',  ( -1.339745962155613812, -35.08034179853028434, -5.000000000000000000 ) ) ;
#45562=ORIENTED_EDGE ( 'NONE', *, *, #46706, .F. ) ;
#45564=CARTESIAN_POINT ( 'NONE',  ( -3.152548672688508926E-16, -34.81249999863440792, -5.148502694627439702 ) ) ;
#45565=CARTESIAN_POINT ( 'NONE',  ( -6.972266317189433020E-16, -5.124999997268812280, -5.000000000000000000 ) ) ;
#45571=CARTESIAN_POINT ( 'NONE',  ( 1.975475456537005874E-15, -38.62499999726880873, 5.000000000000000000 ) ) ;
#45572=VERTEX_POINT ( 'NONE', #54926 ) ;
#45573=CARTESIAN_POINT ( 'NONE',  ( -2.071067811865559882, -161.6874999999999716, -4.999999999999914735 ) ) ;
#45575=CARTESIAN_POINT ( 'NONE',  ( 9.457646018065525792E-16, -81.31249999863440792, 5.148502694627439702 ) ) ;
#45578=CARTESIAN_POINT ( 'NONE',  ( -1.846868145590734756, -140.3750000013656063, -4.458734124999999437 ) ) ;
#45579=CARTESIAN_POINT ( 'NONE',  ( -4.999999999999998224, -57.91666666666665719, 2.886751345948131764 ) ) ;
#45581=CARTESIAN_POINT ( 'NONE',  ( -4.458734124999997661, -43.22916666530106511, 2.574251347313722516 ) ) ;
#45585=CARTESIAN_POINT ( 'NONE',  ( 3.152801135295367541, -140.5625000013655779, -3.152801135295367541 ) ) ;
#45590=CARTESIAN_POINT ( 'NONE',  ( 4.458734125000001214, -73.14583333196773651, 2.574251347313718519 ) ) ;
#45592=DIRECTION ( 'NONE',  ( -0.000000000000000000, 1.000000000000000000, -0.000000000000000000 ) ) ;
#45596=CARTESIAN_POINT ( 'NONE',  ( 2.500000000000002220, 23.45833333606451632, 4.330127018922192761 ) ) ;
#45599=CARTESIAN_POINT ( 'NONE',  ( -2.500000000000000444, -5.166666666666666963, -4.330127018922193649 ) ) ;
#45601=EDGE_CURVE ( 'NONE', #1992, #25522, #9334, .T. ) ;
#45602=CARTESIAN_POINT ( 'NONE',  ( -4.458734124999999437, 15.35416666803225993, -2.574251347313719407 ) ) ;
#45603=CARTESIAN_POINT ( 'NONE',  ( 0.000000000000000000, -170.0000000000000000, 0.000000000000000000 ) ) ;
#45604=AXIS2_PLACEMENT_3D ( 'NONE', #58779, #904, #40109 ) ;
#45606=EDGE_CURVE ( 'NONE', #48949, #33686, #11802, .T. ) ;
#45607=EDGE_CURVE ( 'NONE', #47078, #63425, #31417, .T. ) ;
#45611=FACE_OUTER_BOUND ( 'NONE', #56573, .T. ) ;
#45612=CARTESIAN_POINT ( 'NONE',  ( -2.229367062499996610, -86.14583333196773651, 3.861377020970582219 ) ) ;
#45613=CARTESIAN_POINT ( 'NONE',  ( 2.229367062500001939, -1.979166665301068662, 3.861377020970579999 ) ) ;
#45616=CARTESIAN_POINT ( 'NONE',  ( -3.152548672688508926E-16, -28.81249999863440792, -5.148502694627439702 ) ) ;
#45621=CARTESIAN_POINT ( 'NONE',  ( -4.458734124999999437, 22.60416666803225993, -2.574251347313719407 ) ) ;
#45623=EDGE_CURVE ( 'NONE', #51351, #2611, #2787, .T. ) ;
#45624=CARTESIAN_POINT ( 'NONE',  ( 2.499999999999998668, -66.33333333333332860, -4.330127018922193649 ) ) ;
#45625=CARTESIAN_POINT ( 'NONE',  ( 9.457646018065525792E-16, -78.31249999863440792, 5.148502694627439702 ) ) ;
#45628=CARTESIAN_POINT ( 'NONE',  ( -3.535250795749689387E-16, 22.87500000273118772, -5.773502691896257311 ) ) ;
#45631=FACE_OUTER_BOUND ( 'NONE', #40415, .T. ) ;
#45633=CARTESIAN_POINT ( 'NONE',  ( 5.000000000000000000, -23.41666666666667140, -2.886751345948129988 ) ) ;
#45634=CARTESIAN_POINT ( 'NONE',  ( 9.457646018065525792E-16, -26.06249999863440792, 5.148502694627439702 ) ) ;
#45635=CARTESIAN_POINT ( 'NONE',  ( -2.229367062499996610, -86.14583333196773651, 3.861377020970582219 ) ) ;
#45636=CARTESIAN_POINT ( 'NONE',  ( 1.060575238724906964E-15, -23.62499999726881228, 5.773502691896257311 ) ) ;
#45637=CARTESIAN_POINT ( 'NONE',  ( 2.229367062500001939, -52.97916666530107221, 3.861377020970579999 ) ) ;
#45638=ORIENTED_EDGE ( 'NONE', *, *, #55043, .F. ) ;
#45639=LINE ( 'NONE', #41117, #42791 ) ;
#45640=CARTESIAN_POINT ( 'NONE',  ( 1.339745962155612702, -74.16965819600731891, -5.000000000000000000 ) ) ;
#45641=CARTESIAN_POINT ( 'NONE',  ( -4.458734124999999437, -4.562499998634401699, 0.000000000000000000 ) ) ;
#45643=CARTESIAN_POINT ( 'NONE',  ( 5.000000000000000000, -69.49999999999998579, -6.123233995736766282E-16 ) ) ;
#45644=CARTESIAN_POINT ( 'NONE',  ( 3.152801135295366208, -152.8125000013656063, 3.152801135295367985 ) ) ;
#45647=CARTESIAN_POINT ( 'NONE',  ( 5.000000000000000000, -158.0625000000000284, 2.071067811865478614 ) ) ;
#45648=CARTESIAN_POINT ( 'NONE',  ( -1.127183054612291972E-14, 22.37500000273118417, 4.999999999999999112 ) ) ;
#45650=CARTESIAN_POINT ( 'NONE',  ( 4.458734125000001214, -19.14583333196774007, 2.574251347313718519 ) ) ;
#45651=CARTESIAN_POINT ( 'NONE',  ( 9.457646018065525792E-16, -53.31249999863441502, 5.148502694627439702 ) ) ;
#45654=CARTESIAN_POINT ( 'NONE',  ( 4.458734124999999437, -145.5000000013655779, 1.846868145590737864 ) ) ;
#45658=CARTESIAN_POINT ( 'NONE',  ( 3.061616997868383141E-16, -155.7500000000000000, -5.000000000000000000 ) ) ;
#45659=CARTESIAN_POINT ( 'NONE',  ( -4.458734124999999437, 25.43750000136559208, 0.000000000000000000 ) ) ;
#45661=CARTESIAN_POINT ( 'NONE',  ( 1.975475456537005874E-15, -50.75000000000000000, 5.000000000000000000 ) ) ;
#45665=( BOUNDED_CURVE ( )  B_SPLINE_CURVE ( 2, ( #8773, #9084, #58296, #19677, #9703, #28694, #48313, #34457, #29001 ),
 .UNSPECIFIED., .F., .F. ) 
 B_SPLINE_CURVE_WITH_KNOTS ( ( 3, 2, 2, 2, 3 ),
 ( 0.7854166666666666519, 0.7861111111111110938, 0.7874999999999999778, 0.7888888888888888618, 0.7895833333333333037 ),
 .UNSPECIFIED. ) 
 CURVE ( )  GEOMETRIC_REPRESENTATION_ITEM ( )  RATIONAL_B_SPLINE_CURVE ( ( 0.9330127018922194093, 0.9330127018922194093, 1.000000000000000000, 0.8660254037844387076, 1.000000000000000000, 0.8660254037844387076, 1.000000000000000000, 0.9330127018922194093, 0.9330127018922194093 ) ) 
 REPRESENTATION_ITEM ( '' )  );
#45666=CARTESIAN_POINT ( 'NONE',  ( 5.000000000000000000, 11.62500000273118594, -6.123233995736766282E-16 ) ) ;
#45667=CARTESIAN_POINT ( 'NONE',  ( -2.229367062499996610, -7.145833331967735624, 3.861377020970582219 ) ) ;
#45669=CARTESIAN_POINT ( 'NONE',  ( 3.152801135295366208, -148.5625000013655779, 3.152801135295367985 ) ) ;
#45670=( BOUNDED_CURVE ( )  B_SPLINE_CURVE ( 2, ( #35175, #59292, #1095, #49953, #59623, #35490, #14898, #60266, #16184 ),
 .UNSPECIFIED., .F., .F. ) 
 B_SPLINE_CURVE_WITH_KNOTS ( ( 3, 2, 2, 2, 3 ),
 ( 0.9249999999999998224, 0.9291666666666664742, 0.9333333333333331261, 0.9374999999999998890, 0.9416666666666665408 ),
 .UNSPECIFIED. ) 
 CURVE ( )  GEOMETRIC_REPRESENTATION_ITEM ( )  RATIONAL_B_SPLINE_CURVE ( ( 1.000000000000003997, 0.9238795325112826307, 1.000000000000000000, 0.9238795325112867385, 1.000000000000000000, 0.9238795325112867385, 1.000000000000000000, 0.9238795325112887369, 0.9999999999999980016 ) ) 
 REPRESENTATION_ITEM ( '' )  );
#45676=CARTESIAN_POINT ( 'NONE',  ( 1.975475456537005874E-15, -25.62499999726881228, 5.000000000000000000 ) ) ;
#45677=CARTESIAN_POINT ( 'NONE',  ( -6.972266317189433020E-16, -37.12499999726880873, -5.000000000000000000 ) ) ;
#45679=ADVANCED_FACE ( 'NONE', ( #46863 ), #52007, .T. ) ;
#45684=CARTESIAN_POINT ( 'NONE',  ( 0.000000000000000000, -170.0000000000000000, 0.000000000000000000 ) ) ;
#45686=EDGE_CURVE ( 'NONE', #39380, #36403, #44269, .T. ) ;
#45687=CARTESIAN_POINT ( 'NONE',  ( 2.229367062499998831, 12.35416666803226171, -3.861377020970580887 ) ) ;
#45689=CARTESIAN_POINT ( 'NONE',  ( -2.229367062500000163, -16.72916666530107577, -3.861377020970580443 ) ) ;
#45691=CARTESIAN_POINT ( 'NONE',  ( 4.458734124999999437, -163.4375000013655779, 0.000000000000000000 ) ) ;
#45696=ADVANCED_FACE ( 'NONE', ( #61349 ), #13078, .T. ) ;
#45697=CARTESIAN_POINT ( 'NONE',  ( -1.339745962155610925, -27.79465819873851729, 5.000000000000000000 ) ) ;
#45698=CARTESIAN_POINT ( 'NONE',  ( -2.499999999999996447, -35.83333333333332860, 4.330127018922195425 ) ) ;
#45699=CARTESIAN_POINT ( 'NONE',  ( -4.458734124999997661, -37.22916666530107221, 2.574251347313722516 ) ) ;
#45706=ORIENTED_EDGE ( 'NONE', *, *, #39080, .F. ) ;
#45710=ADVANCED_FACE ( 'NONE', ( #18538 ), #29418, .T. ) ;
#45711=CARTESIAN_POINT ( 'NONE',  ( -5.000000000000000000, -5.999999999999998224, 0.000000000000000000 ) ) ;
#45712=CARTESIAN_POINT ( 'NONE',  ( 9.457646018065525792E-16, -73.06249999863439371, 5.148502694627439702 ) ) ;
#45714=EDGE_CURVE ( 'NONE', #23096, #44027, #4674, .T. ) ;
#45715=CARTESIAN_POINT ( 'NONE',  ( -5.000000000000000000, -5.958333330602148870, -2.886751345948128211 ) ) ;
#45716=CARTESIAN_POINT ( 'NONE',  ( 4.458734124999998549, -37.72916666530107221, -2.574251347313721627 ) ) ;
#45719=CARTESIAN_POINT ( 'NONE',  ( 4.458734125000001214, 10.85416666803225993, 2.574251347313718519 ) ) ;
#45722=CARTESIAN_POINT ( 'NONE',  ( 5.000000000000000000, -49.50000000000000000, -6.123233995736766282E-16 ) ) ;
#45724=CARTESIAN_POINT ( 'NONE',  ( -5.000000000000000000, 14.04166666939785202, -2.886751345948128211 ) ) ;
#45725=CARTESIAN_POINT ( 'NONE',  ( 2.229367062500001939, -72.97916666530107932, 3.861377020970579999 ) ) ;
#45726=( BOUNDED_CURVE ( )  B_SPLINE_CURVE ( 2, ( #10643, #45063, #1029, #46339, #31858, #32488, #42448, #62090, #61464 ),
 .UNSPECIFIED., .F., .F. ) 
 B_SPLINE_CURVE_WITH_KNOTS ( ( 3, 2, 2, 2, 3 ),
 ( 0.8104166666666666741, 0.8111111111111111160, 0.8125000000000000000, 0.8138888888888888840, 0.8145833333333333259 ),
 .UNSPECIFIED. ) 
 CURVE ( )  GEOMETRIC_REPRESENTATION_ITEM ( )  RATIONAL_B_SPLINE_CURVE ( ( 0.9330127018922194093, 0.9330127018922194093, 1.000000000000000000, 0.8660254037844387076, 1.000000000000000000, 0.8660254037844387076, 1.000000000000000000, 0.9330127018922194093, 0.9330127018922194093 ) ) 
 REPRESENTATION_ITEM ( '' )  );
#45727=CARTESIAN_POINT ( 'NONE',  ( -9.184850993605147944E-16, -169.2500000000000000, 5.000000000000000000 ) ) ;
#45728=CARTESIAN_POINT ( 'NONE',  ( -4.458734124999999437, -85.39583333196773651, -2.574251347313719407 ) ) ;
#45730=CARTESIAN_POINT ( 'NONE',  ( -4.458734124999999437, -35.64583333196772941, -2.574251347313719407 ) ) ;
#45731=VERTEX_POINT ( 'NONE', #63232 ) ;
#45735=CARTESIAN_POINT ( 'NONE',  ( 5.000000000000000000, -21.41666666666666430, -2.886751345948130876 ) ) ;
#45736=ORIENTED_EDGE ( 'NONE', *, *, #31180, .F. ) ;
#45737=CARTESIAN_POINT ( 'NONE',  ( 1.062108568985190270E-13, -12.25000000000000000, -4.999999999999999112 ) ) ;
#45738=CARTESIAN_POINT ( 'NONE',  ( -6.972266317189433020E-16, -1.124999997268814278, -5.000000000000000000 ) ) ;
#45739=CARTESIAN_POINT ( 'NONE',  ( -4.458734124999999437, -64.64583333196772230, -2.574251347313719407 ) ) ;
#45744=VERTEX_POINT ( 'NONE', #58082 ) ;
#45746=CARTESIAN_POINT ( 'NONE',  ( -4.458734124999999437, 6.687500001365593860, 0.000000000000000000 ) ) ;
#45748=CARTESIAN_POINT ( 'NONE',  ( -1.846868145590734756, -161.1250000013656063, -4.458734124999999437 ) ) ;
#45749=CARTESIAN_POINT ( 'NONE',  ( -4.999999999999998224, 19.20833333606451632, 2.886751345948131764 ) ) ;
#45754=CARTESIAN_POINT ( 'NONE',  ( 1.339745962155612702, -71.16965819600731891, -5.000000000000000000 ) ) ;
#45755=FACE_OUTER_BOUND ( 'NONE', #35517, .T. ) ;
#45757=CARTESIAN_POINT ( 'NONE',  ( 1.339745962155612702, 12.83034180399266511, -5.000000000000000000 ) ) ;
#45762=CARTESIAN_POINT ( 'NONE',  ( 2.229367062499998831, 2.104166668032262599, -3.861377020970580887 ) ) ;
#45765=CARTESIAN_POINT ( 'NONE',  ( 5.000000000000000000, -146.1250000027312126, 0.000000000000000000 ) ) ;
#45766=CARTESIAN_POINT ( 'NONE',  ( -9.184850993605147944E-16, -159.2500000000000000, 5.000000000000000000 ) ) ;
#45770=CARTESIAN_POINT ( 'NONE',  ( 3.535533905932736864, -140.1250000000000000, 3.535533905932738641 ) ) ;
#45773=CARTESIAN_POINT ( 'NONE',  ( 4.458734124999997661, -160.7500000013655779, 1.846868145590737864 ) ) ;
#45776=CARTESIAN_POINT ( 'NONE',  ( 1.846868145590736310, -139.6250000013656347, 4.458734124999999437 ) ) ;
#45777=VERTEX_POINT ( 'NONE', #48731 ) ;
#45778=CARTESIAN_POINT ( 'NONE',  ( 4.458734125000001214, 24.85416666803225993, 2.574251347313718519 ) ) ;
#45779=ORIENTED_EDGE ( 'NONE', *, *, #16203, .T. ) ;
#45783=DIRECTION ( 'NONE',  ( -0.000000000000000000, 1.000000000000000000, -0.000000000000000000 ) ) ;
#45784=CARTESIAN_POINT ( 'NONE',  ( -5.000000000000000000, 15.00000000000000000, 0.000000000000000000 ) ) ;
#45785=CARTESIAN_POINT ( 'NONE',  ( -2.229367062499996610, -57.14583333196773651, 3.861377020970582219 ) ) ;
#45786=AXIS2_PLACEMENT_3D ( 'NONE', #51456, #22822, #7074 ) ;
#45787=CARTESIAN_POINT ( 'NONE',  ( -4.458734124999998549, -10.22916666530106866, 2.574251347313722516 ) ) ;
#45788=ADVANCED_FACE ( 'NONE', ( #49049 ), #24296, .T. ) ;
#45791=CARTESIAN_POINT ( 'NONE',  ( -5.000000000000000000, 0.04166666939785235169, -2.886751345948128211 ) ) ;
#45792=CARTESIAN_POINT ( 'NONE',  ( -2.499999999999996447, -36.83333333333332860, 4.330127018922195425 ) ) ;
#45793=CARTESIAN_POINT ( 'NONE',  ( -1.339745962155564296, -10.20534180126148271, -5.000000000000028422 ) ) ;
#45797=CARTESIAN_POINT ( 'NONE',  ( -3.152548672688508926E-16, -60.56249999863440792, -5.148502694627439702 ) ) ;
#45798=CARTESIAN_POINT ( 'NONE',  ( 4.458734125000000326, -151.6250000013656063, -1.846868145590734978 ) ) ;
#45799=CARTESIAN_POINT ( 'NONE',  ( 4.458734124999999437, -65.81249999863440792, -5.460374474430324690E-16 ) ) ;
#45802=CARTESIAN_POINT ( 'NONE',  ( -5.000000000000000000, -58.87499999726880873, 0.000000000000000000 ) ) ;
#45803=ORIENTED_EDGE ( 'NONE', *, *, #50325, .F. ) ;
#45804=CARTESIAN_POINT ( 'NONE',  ( 0.000000000000000000, -170.0000000000000000, 5.000000000000000000 ) ) ;
#45805=ORIENTED_EDGE ( 'NONE', *, *, #112, .T. ) ;
#45806=CARTESIAN_POINT ( 'NONE',  ( -3.535533905932738641, -157.5000000027312126, 3.535533905932737309 ) ) ;
#45808=CARTESIAN_POINT ( 'NONE',  ( 1.846868145590735200, -151.2500000013656063, -4.458734125000000326 ) ) ;
#45813=CARTESIAN_POINT ( 'NONE',  ( 4.458734124999998549, -49.97916666530106511, -2.574251347313721627 ) ) ;
#45815=( BOUNDED_CURVE ( )  B_SPLINE_CURVE ( 2, ( #34311, #27915, #3487, #29795, #30767, #35275, #45559, #39452, #49428 ),
 .UNSPECIFIED., .F., .F. ) 
 B_SPLINE_CURVE_WITH_KNOTS ( ( 3, 2, 2, 2, 3 ),
 ( 0.2312500000000000111, 0.2319444444444444531, 0.2333333333333333370, 0.2347222222222222210, 0.2354166666666666630 ),
 .UNSPECIFIED. ) 
 CURVE ( )  GEOMETRIC_REPRESENTATION_ITEM ( )  RATIONAL_B_SPLINE_CURVE ( ( 0.9330127018922194093, 0.9330127018922194093, 1.000000000000000000, 0.8660254037844387076, 1.000000000000000000, 0.8660254037844387076, 1.000000000000000000, 0.9330127018922194093, 0.9330127018922194093 ) ) 
 REPRESENTATION_ITEM ( '' )  );
#45818=CARTESIAN_POINT ( 'NONE',  ( -4.458734124999999437, 25.68750000136559208, 0.000000000000000000 ) ) ;
#45821=EDGE_LOOP ( 'NONE', ( #56461, #38591, #34614, #44211 ) ) ;
#45825=VECTOR ( 'NONE', #22840, 1000.000000000000000 ) ;
#45832=CARTESIAN_POINT ( 'NONE',  ( 0.000000000000000000, -170.0000000000000000, 0.000000000000000000 ) ) ;
#45838=CARTESIAN_POINT ( 'NONE',  ( -3.535533905932738641, -155.5000000027312126, 3.535533905932737309 ) ) ;
#45848=CARTESIAN_POINT ( 'NONE',  ( -4.458734124999999437, -17.39583333196773651, -2.574251347313719407 ) ) ;
#45850=CARTESIAN_POINT ( 'NONE',  ( -9.184850993605147944E-16, -149.2500000000000284, 5.000000000000000000 ) ) ;
#45852=CARTESIAN_POINT ( 'NONE',  ( 4.458734124999999437, -150.5000000013656347, 1.846868145590737864 ) ) ;
#45853=VERTEX_POINT ( 'NONE', #19146 ) ;
#45854=CARTESIAN_POINT ( 'NONE',  ( 2.229367062500001939, -54.22916666530107221, 3.861377020970579999 ) ) ;
#45855=CARTESIAN_POINT ( 'NONE',  ( -4.764381983412779477E-15, 26.25000000000000000, 5.000000000000000000 ) ) ;
#45856=CARTESIAN_POINT ( 'NONE',  ( -4.458734124999998549, -88.22916666530107932, 2.574251347313722516 ) ) ;
#45857=CARTESIAN_POINT ( 'NONE',  ( -4.458734124999999437, 3.687500001365594748, 0.000000000000000000 ) ) ;
#45858=DIRECTION ( 'NONE',  ( -0.000000000000000000, 1.000000000000000000, -0.000000000000000000 ) ) ;
#45859=CARTESIAN_POINT ( 'NONE',  ( -6.972266317189433020E-16, 6.750000000000000000, -5.000000000000000000 ) ) ;
#45861=CARTESIAN_POINT ( 'NONE',  ( 2.229367062499998831, 13.10416666803226171, -3.861377020970580887 ) ) ;
#45862=CARTESIAN_POINT ( 'NONE',  ( -2.500000000000000444, 3.958333336064518093, -4.330127018922193649 ) ) ;
#45863=ORIENTED_EDGE ( 'NONE', *, *, #24032, .F. ) ;
#45865=EDGE_LOOP ( 'NONE', ( #5376, #34425, #47707, #1273 ) ) ;
#45867=AXIS2_PLACEMENT_3D ( 'NONE', #13970, #53217, #9149 ) ;
#45868=CARTESIAN_POINT ( 'NONE',  ( 0.000000000000000000, -170.0000000000000000, 0.000000000000000000 ) ) ;
#45869=CARTESIAN_POINT ( 'NONE',  ( 2.229367062500001939, -43.97916666530106511, 3.861377020970579999 ) ) ;
#45870=CARTESIAN_POINT ( 'NONE',  ( -3.152801135295367985, -163.0625000013656063, 3.152801135295367096 ) ) ;
#45872=CARTESIAN_POINT ( 'NONE',  ( -5.000000000000000000, -37.95833333060214443, -2.886751345948128211 ) ) ;
#45874=CARTESIAN_POINT ( 'NONE',  ( -3.152548672688508926E-16, -17.56249999863440792, -5.148502694627439702 ) ) ;
#45876=CARTESIAN_POINT ( 'NONE',  ( -2.499999999999996447, -89.83333333333332860, 4.330127018922195425 ) ) ;
#45877=CARTESIAN_POINT ( 'NONE',  ( -3.152801135295367985, -164.8125000013656063, 3.152801135295367096 ) ) ;
#45878=CARTESIAN_POINT ( 'NONE',  ( 5.000000000000000000, -88.29166666393547303, -2.886751345948129988 ) ) ;
#45879=CARTESIAN_POINT ( 'NONE',  ( 1.975475456537005874E-15, -34.62499999726880873, 5.000000000000000000 ) ) ;
#45880=ORIENTED_EDGE ( 'NONE', *, *, #15336, .F. ) ;
#45882=ADVANCED_FACE ( 'NONE', ( #38453 ), #23053, .T. ) ;
#45883=CARTESIAN_POINT ( 'NONE',  ( 2.229367062500001939, -31.22916666530107221, 3.861377020970579999 ) ) ;
#45885=ORIENTED_EDGE ( 'NONE', *, *, #29867, .F. ) ;
#45888=CARTESIAN_POINT ( 'NONE',  ( -6.972266317189433020E-16, -29.12499999726880873, -5.000000000000000000 ) ) ;
#45892=CARTESIAN_POINT ( 'NONE',  ( -2.229367062500000163, -80.72916666530106511, -3.861377020970580443 ) ) ;
#45895=CARTESIAN_POINT ( 'NONE',  ( 4.458734124999999437, -141.6250000013656347, -1.846868145590734978 ) ) ;
#45897=LINE ( 'NONE', #50723, #30202 ) ;
#45899=CARTESIAN_POINT ( 'NONE',  ( 9.457646018065525792E-16, -46.06249999863440081, 5.148502694627439702 ) ) ;
#45902=EDGE_CURVE ( 'NONE', #1132, #1992, #9498, .T. ) ;
#45903=DIRECTION ( 'NONE',  ( -0.000000000000000000, 1.000000000000000000, -0.000000000000000000 ) ) ;
#45906=CARTESIAN_POINT ( 'NONE',  ( -2.500000000000000444, -40.04166666393548013, -4.330127018922193649 ) ) ;
#45908=CARTESIAN_POINT ( 'NONE',  ( -2.229367062500000163, -80.72916666530106511, -3.861377020970580443 ) ) ;
#45910=CYLINDRICAL_SURFACE ( 'NONE', #32606, 5.000000000000000000 ) ;
#45913=VECTOR ( 'NONE', #8363, 1000.000000000000000 ) ;
#45917=CARTESIAN_POINT ( 'NONE',  ( 5.000000000000000000, -168.1250000027312126, 0.000000000000000000 ) ) ;
#45919=CARTESIAN_POINT ( 'NONE',  ( 9.457646018065525792E-16, 10.68750000136559386, 5.148502694627439702 ) ) ;
#45920=CARTESIAN_POINT ( 'NONE',  ( 0.000000000000000000, -170.0000000000000000, 0.000000000000000000 ) ) ;
#45922=VECTOR ( 'NONE', #36353, 1000.000000000000000 ) ;
#45926=CARTESIAN_POINT ( 'NONE',  ( -2.500000000000000444, -14.04166666393548013, -4.330127018922193649 ) ) ;
#45927=CARTESIAN_POINT ( 'NONE',  ( 4.458734125000001214, -87.89583333196773651, 2.574251347313718519 ) ) ;
#45928=CARTESIAN_POINT ( 'NONE',  ( -4.458734124999999437, -5.312499998634402587, 0.000000000000000000 ) ) ;
#45929=ORIENTED_EDGE ( 'NONE', *, *, #60583, .F. ) ;
#45930=CARTESIAN_POINT ( 'NONE',  ( 2.229367062500001939, -30.22916666530107221, 3.861377020970579999 ) ) ;
#45934=CARTESIAN_POINT ( 'NONE',  ( -4.458734124999999437, 18.60416666803225993, -2.574251347313719407 ) ) ;
#45935=CARTESIAN_POINT ( 'NONE',  ( -5.000000000000000000, -43.87499999726880873, 0.000000000000000000 ) ) ;
#45937=CARTESIAN_POINT ( 'NONE',  ( 4.458734124999999437, -76.06249999863440792, -5.460374474430324690E-16 ) ) ;
#45940=CARTESIAN_POINT ( 'NONE',  ( 5.000000000000000000, 24.70833333606451987, -2.886751345948129988 ) ) ;
#45943=CARTESIAN_POINT ( 'NONE',  ( -2.071067811865477726, -168.8125000027312410, -4.999999999999996447 ) ) ;
#45944=CARTESIAN_POINT ( 'NONE',  ( 1.975475456537005874E-15, -0.7499999999999996669, 5.000000000000000000 ) ) ;
#45945=CARTESIAN_POINT ( 'NONE',  ( -5.000000000000000000, -26.00000000000000355, 0.000000000000000000 ) ) ;
#45946=CARTESIAN_POINT ( 'NONE',  ( 9.457646018065525792E-16, -29.06249999863440081, 5.148502694627439702 ) ) ;
#45947=CARTESIAN_POINT ( 'NONE',  ( 4.458734124999999437, -85.81249999863439371, -5.460374474430324690E-16 ) ) ;
#45948=CARTESIAN_POINT ( 'NONE',  ( -3.535250795749689387E-16, -23.12499999726881228, -5.773502691896257311 ) ) ;
#45949=CARTESIAN_POINT ( 'NONE',  ( -4.458734124999999437, -54.39583333196773651, -2.574251347313719407 ) ) ;
#45950=ORIENTED_EDGE ( 'NONE', *, *, #49954, .T. ) ;
#45951=CARTESIAN_POINT ( 'NONE',  ( 5.000000000000000888, -27.58333333333333570, 2.886751345948126879 ) ) ;
#45953=CARTESIAN_POINT ( 'NONE',  ( 9.457646018065525792E-16, -4.312499998634408804, 5.148502694627439702 ) ) ;
#45955=CARTESIAN_POINT ( 'NONE',  ( 2.499999999999998668, -73.33333333333332860, -4.330127018922193649 ) ) ;
#45959=AXIS2_PLACEMENT_3D ( 'NONE', #29506, #25336, #5722 ) ;
#45960=CARTESIAN_POINT ( 'NONE',  ( -3.535533905932737309, -158.6250000000000284, -3.535533905932738197 ) ) ;
#45961=CARTESIAN_POINT ( 'NONE',  ( 2.500000000000002220, -71.54166666393547303, 4.330127018922192761 ) ) ;
#45962=FACE_OUTER_BOUND ( 'NONE', #33234, .T. ) ;
#45964=EDGE_CURVE ( 'NONE', #41952, #53169, #57477, .T. ) ;
#45965=AXIS2_PLACEMENT_3D ( 'NONE', #22515, #61755, #35156 ) ;
#45966=CARTESIAN_POINT ( 'NONE',  ( 4.458734124999999437, -15.06249999863440436, -5.460374474430324690E-16 ) ) ;
#45967=AXIS2_PLACEMENT_3D ( 'NONE', #44432, #5849, #49896 ) ;
#45968=CARTESIAN_POINT ( 'NONE',  ( 4.458734124999998549, -53.97916666530107221, -2.574251347313721627 ) ) ;
#45970=CARTESIAN_POINT ( 'NONE',  ( 1.846868145590736310, -142.6250000013655779, 4.458734124999999437 ) ) ;
#45972=CARTESIAN_POINT ( 'NONE',  ( 2.071067811865348940, -157.8125000000000284, -5.000000000000127898 ) ) ;
#45973=ORIENTED_EDGE ( 'NONE', *, *, #31984, .T. ) ;
#45974=CARTESIAN_POINT ( 'NONE',  ( -2.071067811865308972, -155.3125000000000000, 5.000000000000169642 ) ) ;
#45975=CARTESIAN_POINT ( 'NONE',  ( 4.458734124999999437, 24.93750000136559208, -5.460374474430324690E-16 ) ) ;
#45977=EDGE_CURVE ( 'NONE', #55791, #27450, #42658, .T. ) ;
#45980=CARTESIAN_POINT ( 'NONE',  ( -4.458734124999999437, -147.1875000013656063, -5.460374474430324690E-16 ) ) ;
#45982=ADVANCED_FACE ( 'NONE', ( #34254 ), #29107, .T. ) ;
#45983=CARTESIAN_POINT ( 'NONE',  ( -2.229367062500000163, -63.72916666530106511, -3.861377020970580443 ) ) ;
#45985=CARTESIAN_POINT ( 'NONE',  ( -3.152548672688508926E-16, -6.562499998634404363, -5.148502694627439702 ) ) ;
#45986=CARTESIAN_POINT ( 'NONE',  ( -4.458734124999999437, -146.0000000013655779, -1.846868145590735644 ) ) ;
#45995=( BOUNDED_CURVE ( )  B_SPLINE_CURVE ( 2, ( #51523, #47007, #27068, #41848, #51829, #23510, #43112, #13543, #22885 ),
 .UNSPECIFIED., .F., .F. ) 
 B_SPLINE_CURVE_WITH_KNOTS ( ( 3, 2, 2, 2, 3 ),
 ( 0.9416666666666665408, 0.9458333333333331927, 0.9499999999999997335, 0.9541666666666664964, 0.9583333333333331483 ),
 .UNSPECIFIED. ) 
 CURVE ( )  GEOMETRIC_REPRESENTATION_ITEM ( )  RATIONAL_B_SPLINE_CURVE ( ( 1.000000000000001998, 0.9238795325112847401, 1.000000000000000000, 0.9238795325112867385, 1.000000000000000000, 0.9238795325112867385, 1.000000000000000000, 0.9238795325112908463, 0.9999999999999958922 ) ) 
 REPRESENTATION_ITEM ( '' )  );
#46000=CARTESIAN_POINT ( 'NONE',  ( 5.275681513340003914E-14, 11.74999999999999645, -5.000000000000000000 ) ) ;
#46001=CARTESIAN_POINT ( 'NONE',  ( -1.339745962155613812, -15.20534180126147916, -5.000000000000000000 ) ) ;
#46002=CARTESIAN_POINT ( 'NONE',  ( 2.229367062500001939, 13.02083333469892779, 3.861377020970579999 ) ) ;
#46004=CARTESIAN_POINT ( 'NONE',  ( -4.458734124999999437, -14.64583333196773474, -2.574251347313719407 ) ) ;
#46007=CARTESIAN_POINT ( 'NONE',  ( -3.152801135295367096, -162.0625000013656063, -3.152801135295367541 ) ) ;
#46008=CARTESIAN_POINT ( 'NONE',  ( -5.000000000000000000, -40.95833333060215153, -2.886751345948128211 ) ) ;
#46013=CARTESIAN_POINT ( 'NONE',  ( -2.499999999999996447, -27.83333333333333570, 4.330127018922195425 ) ) ;
#46014=CARTESIAN_POINT ( 'NONE',  ( -9.184850993605147944E-16, -139.3750000027312126, 5.000000000000000000 ) ) ;
#46015=CARTESIAN_POINT ( 'NONE',  ( 4.458734125000000326, -33.89583333196772941, 2.574251347313718519 ) ) ;
#46016=CARTESIAN_POINT ( 'NONE',  ( 1.339745962155612702, -60.29465819873851729, -5.000000000000000000 ) ) ;
#46019=CARTESIAN_POINT ( 'NONE',  ( 1.975475456537005874E-15, -50.75000000000000000, 5.000000000000000000 ) ) ;
#46023=DIRECTION ( 'NONE',  ( 0.000000000000000000, 0.000000000000000000, 1.000000000000000000 ) ) ;
#46024=CARTESIAN_POINT ( 'NONE',  ( 5.000000000000000000, -6.416666666666666963, -2.886751345948129988 ) ) ;
#46025=CARTESIAN_POINT ( 'NONE',  ( -4.458734124999997661, -73.22916666530106511, 2.574251347313722516 ) ) ;
#46027=CARTESIAN_POINT ( 'NONE',  ( 2.499999999999998668, -8.208333330602144429, -4.330127018922193649 ) ) ;
#46028=CARTESIAN_POINT ( 'NONE',  ( 2.229367062500001939, -39.97916666530107221, 3.861377020970579999 ) ) ;
#46029=EDGE_LOOP ( 'NONE', ( #23319, #18584, #18658, #31734 ) ) ;
#46031=CARTESIAN_POINT ( 'NONE',  ( -2.229367062500000163, 13.27083333469892779, -3.861377020970580443 ) ) ;
#46034=CARTESIAN_POINT ( 'NONE',  ( -5.000000000000000000, -53.99999999999999289, 0.000000000000000000 ) ) ;
#46037=CARTESIAN_POINT ( 'NONE',  ( -4.458734124999999437, -75.31249999863440792, 0.000000000000000000 ) ) ;
#46038=CARTESIAN_POINT ( 'NONE',  ( 2.730187237215162345E-16, -140.4375000013656063, -4.458734124999999437 ) ) ;
#46039=CARTESIAN_POINT ( 'NONE',  ( -4.458734124999999437, -86.39583333196772230, -2.574251347313719407 ) ) ;
#46041=CARTESIAN_POINT ( 'NONE',  ( 2.229367062500001939, -35.22916666530107221, 3.861377020970579999 ) ) ;
#46043=EDGE_CURVE ( 'NONE', #46757, #30862, #15920, .T. ) ;
#46047=( BOUNDED_CURVE ( )  B_SPLINE_CURVE ( 2, ( #9945, #30196, #25067, #29561, #49194, #44677, #49825, #50146, #10908 ),
 .UNSPECIFIED., .F., .F. ) 
 B_SPLINE_CURVE_WITH_KNOTS ( ( 3, 2, 2, 2, 3 ),
 ( 0.9145833333333333037, 0.9152777777777777457, 0.9166666666666666297, 0.9180555555555555136, 0.9187499999999999556 ),
 .UNSPECIFIED. ) 
 CURVE ( )  GEOMETRIC_REPRESENTATION_ITEM ( )  RATIONAL_B_SPLINE_CURVE ( ( 0.9330127018922194093, 0.9330127018922194093, 1.000000000000000000, 0.8660254037844387076, 1.000000000000000000, 0.8660254037844387076, 1.000000000000000000, 0.9330127018922194093, 0.9330127018922194093 ) ) 
 REPRESENTATION_ITEM ( '' )  );
#46053=CARTESIAN_POINT ( 'NONE',  ( -4.458734124999999437, -65.64583333196773651, -2.574251347313719407 ) ) ;
#46056=EDGE_CURVE ( 'NONE', #56335, #47300, #13491, .T. ) ;
#46058=CARTESIAN_POINT ( 'NONE',  ( 1.975475456537005874E-15, -62.74999999999998579, 5.000000000000000000 ) ) ;
#46062=CARTESIAN_POINT ( 'NONE',  ( 4.458734124999999437, 5.187500001365596525, -5.460374474430324690E-16 ) ) ;
#46064=CARTESIAN_POINT ( 'NONE',  ( -1.846868145590734756, -158.1250000013656063, -4.458734124999999437 ) ) ;
#46068=ADVANCED_FACE ( 'NONE', ( #11411 ), #25892, .T. ) ;
#46069=DIRECTION ( 'NONE',  ( -0.000000000000000000, 1.000000000000000000, -0.000000000000000000 ) ) ;
#46071=CARTESIAN_POINT ( 'NONE',  ( -6.972266317189433020E-16, -88.12499999726880162, -5.000000000000000000 ) ) ;
#46077=CARTESIAN_POINT ( 'NONE',  ( -4.458734124999999437, 29.60416666803225993, -2.574251347313719407 ) ) ;
#46080=CARTESIAN_POINT ( 'NONE',  ( 2.229367062500001939, 2.770833334698928674, 3.861377020970579999 ) ) ;
#46081=CARTESIAN_POINT ( 'NONE',  ( 3.535533905932736864, -160.2500000027312126, 3.535533905932738641 ) ) ;
#46083=CARTESIAN_POINT ( 'NONE',  ( 5.000000000000000000, -146.1875000027311842, 2.071067811865478614 ) ) ;
#46087=FACE_OUTER_BOUND ( 'NONE', #15446, .T. ) ;
#46090=CARTESIAN_POINT ( 'NONE',  ( -4.458734124999999437, -160.2500000013656063, -1.846868145590735644 ) ) ;
#46093=CARTESIAN_POINT ( 'NONE',  ( 1.846868145590736310, -141.6250000013656631, 4.458734124999999437 ) ) ;
#46095=CARTESIAN_POINT ( 'NONE',  ( 2.229367062500001939, 22.77083333469892423, 3.861377020970579999 ) ) ;
#46100=( BOUNDED_CURVE ( )  B_SPLINE_CURVE ( 2, ( #28575, #28889, #4448, #23767, #23452, #5086, #48510, #39487, #18619 ),
 .UNSPECIFIED., .F., .F. ) 
 B_SPLINE_CURVE_WITH_KNOTS ( ( 3, 2, 2, 2, 3 ),
 ( 0.8312500000000000444, 0.8319444444444444864, 0.8333333333333333703, 0.8347222222222222543, 0.8354166666666666963 ),
 .UNSPECIFIED. ) 
 CURVE ( )  GEOMETRIC_REPRESENTATION_ITEM ( )  RATIONAL_B_SPLINE_CURVE ( ( 0.9330127018922194093, 0.9330127018922194093, 1.000000000000000000, 0.8660254037844387076, 1.000000000000000000, 0.8660254037844387076, 1.000000000000000000, 0.9330127018922194093, 0.9330127018922194093 ) ) 
 REPRESENTATION_ITEM ( '' )  );
#46101=CARTESIAN_POINT ( 'NONE',  ( 2.499999999999998668, 2.666666666666667851, -4.330127018922193649 ) ) ;
#46102=CARTESIAN_POINT ( 'NONE',  ( 1.060575238724906964E-15, 9.250000000000001776, 5.773502691896257311 ) ) ;
#46104=CARTESIAN_POINT ( 'NONE',  ( -3.152548672688508926E-16, -55.56249999863440081, -5.148502694627439702 ) ) ;
#46105=CARTESIAN_POINT ( 'NONE',  ( -4.458734124999998549, -14.22916666530107221, 2.574251347313722516 ) ) ;
#46106=CARTESIAN_POINT ( 'NONE',  ( 5.000000000000000888, -6.583333333333329485, 2.886751345948126879 ) ) ;
#46108=CARTESIAN_POINT ( 'NONE',  ( 1.975475456537005874E-15, 0.3750000027311862216, 5.000000000000000000 ) ) ;
#46110=CARTESIAN_POINT ( 'NONE',  ( -2.500000000000000444, -40.16666666666667140, -4.330127018922193649 ) ) ;
#46111=DIRECTION ( 'NONE',  ( 0.000000000000000000, 0.000000000000000000, 1.000000000000000000 ) ) ;
#46112=CARTESIAN_POINT ( 'NONE',  ( 1.975475456537005874E-15, -44.74999999999999289, 5.000000000000000000 ) ) ;
#46115=CARTESIAN_POINT ( 'NONE',  ( -3.152548672688508926E-16, -59.56249999863440081, -5.148502694627439702 ) ) ;
#46116=CARTESIAN_POINT ( 'NONE',  ( -4.458734125000001214, -153.1250000013656063, 1.846868145590734089 ) ) ;
#46117=CARTESIAN_POINT ( 'NONE',  ( 9.457646018065525792E-16, -71.06249999863440792, 5.148502694627439702 ) ) ;
#46119=CARTESIAN_POINT ( 'NONE',  ( -4.458734124999999437, -20.64583333196774007, -2.574251347313719407 ) ) ;
#46120=CARTESIAN_POINT ( 'NONE',  ( -4.999999999999999112, -58.79166666393546592, 2.886751345948131764 ) ) ;
#46121=ADVANCED_FACE ( 'NONE', ( #1471 ), #30066, .T. ) ;
#46123=CARTESIAN_POINT ( 'NONE',  ( 1.339745962155612702, -31.16965819600732956, -5.000000000000000000 ) ) ;
#46128=CARTESIAN_POINT ( 'NONE',  ( 4.458734124999999437, -154.4375000013655779, 0.000000000000000000 ) ) ;
#46132=CARTESIAN_POINT ( 'NONE',  ( -2.229367062500000163, -47.72916666530106511, -3.861377020970580443 ) ) ;
#46136=EDGE_CURVE ( 'NONE', #62531, #2792, #33210, .T. ) ;
#46138=CARTESIAN_POINT ( 'NONE',  ( -3.152548672688508926E-16, 26.43750000136559208, -5.148502694627439702 ) ) ;
#46141=CARTESIAN_POINT ( 'NONE',  ( -1.339745962155610925, -35.66965819600732601, 5.000000000000000000 ) ) ;
#46142=VECTOR ( 'NONE', #47440, 1000.000000000000000 ) ;
#46143=ORIENTED_EDGE ( 'NONE', *, *, #112, .F. ) ;
#46161=CARTESIAN_POINT ( 'NONE',  ( -2.071067811865478170, -157.4375000027312410, 5.000000000000000000 ) ) ;
#46171=CARTESIAN_POINT ( 'NONE',  ( -4.458734124999999437, -27.39583333196774007, -2.574251347313719407 ) ) ;
#46173=CARTESIAN_POINT ( 'NONE',  ( 3.535533905932736864, -150.1250000000000000, 3.535533905932738641 ) ) ;
#46175=CARTESIAN_POINT ( 'NONE',  ( -3.152801135295367985, -151.8125000013655779, 3.152801135295367096 ) ) ;
#46177=CARTESIAN_POINT ( 'NONE',  ( 4.458734124999999437, -49.06249999863440792, -5.460374474430324690E-16 ) ) ;
#46180=CARTESIAN_POINT ( 'NONE',  ( -5.000000000000000000, 24.00000000000000000, 0.000000000000000000 ) ) ;
#46181=( BOUNDED_CURVE ( )  B_SPLINE_CURVE ( 2, ( #17323, #42700, #46276, #7995, #56887, #22793, #13127, #8310, #37568 ),
 .UNSPECIFIED., .F., .F. ) 
 B_SPLINE_CURVE_WITH_KNOTS ( ( 3, 2, 2, 2, 3 ),
 ( 0.7604166666666666297, 0.7611111111111110716, 0.7624999999999999556, 0.7638888888888888395, 0.7645833333333332815 ),
 .UNSPECIFIED. ) 
 CURVE ( )  GEOMETRIC_REPRESENTATION_ITEM ( )  RATIONAL_B_SPLINE_CURVE ( ( 0.9330127018922194093, 0.9330127018922194093, 1.000000000000000000, 0.8660254037844387076, 1.000000000000000000, 0.8660254037844387076, 1.000000000000000000, 0.9330127018922194093, 0.9330127018922194093 ) ) 
 REPRESENTATION_ITEM ( '' )  );
#46183=CARTESIAN_POINT ( 'NONE',  ( 9.457646018065525792E-16, 3.937500001365595192, 5.148502694627439702 ) ) ;
#46184=CARTESIAN_POINT ( 'NONE',  ( -3.535533905932738641, -160.5000000027312126, 3.535533905932737309 ) ) ;
#46185=DIRECTION ( 'NONE',  ( 0.000000000000000000, -1.000000000000000000, 0.000000000000000000 ) ) ;
#46186=CARTESIAN_POINT ( 'NONE',  ( 1.975475456537005874E-15, -7.750000000000000000, 5.000000000000000000 ) ) ;
#46187=CARTESIAN_POINT ( 'NONE',  ( 2.229367062500001939, 14.77083333469892779, 3.861377020970579999 ) ) ;
#46188=CARTESIAN_POINT ( 'NONE',  ( 5.000000000000000000, 4.625000002731187720, -6.123233995736766282E-16 ) ) ;
#46189=ORIENTED_EDGE ( 'NONE', *, *, #29867, .T. ) ;
#46193=CARTESIAN_POINT ( 'NONE',  ( 4.458734125000001214, -42.89583333196773651, 2.574251347313718519 ) ) ;
#46194=CARTESIAN_POINT ( 'NONE',  ( -4.458734125000000326, -164.2500000013656063, -1.846868145590735644 ) ) ;
#46196=CARTESIAN_POINT ( 'NONE',  ( -5.000000000000000000, -43.95833333060214443, -2.886751345948128211 ) ) ;
#46197=ORIENTED_EDGE ( 'NONE', *, *, #3851, .T. ) ;
#46198=CARTESIAN_POINT ( 'NONE',  ( -2.229367062499996610, -19.14583333196774007, 3.861377020970582219 ) ) ;
#46199=VERTEX_POINT ( 'NONE', #12917 ) ;
#46200=CARTESIAN_POINT ( 'NONE',  ( -4.999999999999999112, -85.91666666666667140, 2.886751345948131764 ) ) ;
#46201=CARTESIAN_POINT ( 'NONE',  ( 1.846868145590736310, -165.6250000013656063, 4.458734124999999437 ) ) ;
#46202=CARTESIAN_POINT ( 'NONE',  ( -6.972266317189433020E-16, -19.25000000000000000, -5.000000000000000000 ) ) ;
#46203=ORIENTED_EDGE ( 'NONE', *, *, #20853, .F. ) ;
#46205=CARTESIAN_POINT ( 'NONE',  ( 4.458734124999998549, -31.97916666530107577, -2.574251347313721627 ) ) ;
#46211=ORIENTED_EDGE ( 'NONE', *, *, #40175, .T. ) ;
#46214=CARTESIAN_POINT ( 'NONE',  ( -3.152548672688508926E-16, -82.81249999863442213, -5.148502694627439702 ) ) ;
#46217=CARTESIAN_POINT ( 'NONE',  ( -3.152801135295367985, -144.0625000013655779, 3.152801135295367096 ) ) ;
#46218=CARTESIAN_POINT ( 'NONE',  ( -6.972266317189433020E-16, 20.74999999999999645, -5.000000000000000000 ) ) ;
#46220=CARTESIAN_POINT ( 'NONE',  ( -4.458734124999999437, -46.31249999863440792, 0.000000000000000000 ) ) ;
#46223=CARTESIAN_POINT ( 'NONE',  ( 5.000000000000000000, -3.500000000000003109, -6.123233995736766282E-16 ) ) ;
#46226=CARTESIAN_POINT ( 'NONE',  ( -9.184850993605147944E-16, -153.3750000027311842, 5.000000000000000000 ) ) ;
#46228=CARTESIAN_POINT ( 'NONE',  ( -4.458734124999999437, -77.64583333196773651, -2.574251347313719407 ) ) ;
#46229=CARTESIAN_POINT ( 'NONE',  ( 5.000000000000000888, -34.58333333333332860, 2.886751345948126879 ) ) ;
#46232=VERTEX_POINT ( 'NONE', #22593 ) ;
#46234=CARTESIAN_POINT ( 'NONE',  ( 1.339745962155612702, -47.29465819873852439, -5.000000000000000000 ) ) ;
#46236=CARTESIAN_POINT ( 'NONE',  ( 3.535533905932738197, -169.0000000027312126, -3.535533905932738197 ) ) ;
#46239=CARTESIAN_POINT ( 'NONE',  ( -4.458734124999999437, 11.35416666803225993, -2.574251347313719407 ) ) ;
#46247=CARTESIAN_POINT ( 'NONE',  ( 4.458734124999998549, -86.72916666530107932, -2.574251347313721627 ) ) ;
#46248=CARTESIAN_POINT ( 'NONE',  ( -4.458734124999997661, -8.229166665301073991, 2.574251347313722516 ) ) ;
#46250=VERTEX_POINT ( 'NONE', #18059 ) ;
#46251=CARTESIAN_POINT ( 'NONE',  ( 4.458734124999999437, -38.06249999863440792, -5.460374474430324690E-16 ) ) ;
#46256=EDGE_CURVE ( 'NONE', #30690, #41008, #27714, .T. ) ;
#46257=CARTESIAN_POINT ( 'NONE',  ( 4.458734124999999437, 20.18750000136559208, -5.460374474430324690E-16 ) ) ;
#46259=CARTESIAN_POINT ( 'NONE',  ( 2.499999999999998668, 1.666666666666666963, -4.330127018922193649 ) ) ;
#46260=CARTESIAN_POINT ( 'NONE',  ( -3.152548672688508926E-16, -77.81249999863440792, -5.148502694627439702 ) ) ;
#46262=CARTESIAN_POINT ( 'NONE',  ( 5.000000000000000000, -72.29166666393548724, -2.886751345948130876 ) ) ;
#46263=CARTESIAN_POINT ( 'NONE',  ( 5.000000000000000000, 20.70833333606451632, -2.886751345948129988 ) ) ;
#46264=VERTEX_POINT ( 'NONE', #1793 ) ;
#46265=CARTESIAN_POINT ( 'NONE',  ( -2.499999999999996447, -65.83333333333332860, 4.330127018922195425 ) ) ;
#46268=CARTESIAN_POINT ( 'NONE',  ( -6.972266317189433020E-16, -14.12499999726881228, -5.000000000000000000 ) ) ;
#46269=CARTESIAN_POINT ( 'NONE',  ( -4.999999999999999112, -23.91666666666667140, 2.886751345948131764 ) ) ;
#46270=CARTESIAN_POINT ( 'NONE',  ( -4.458734124999998549, -28.22916666530106866, 2.574251347313722516 ) ) ;
#46271=CARTESIAN_POINT ( 'NONE',  ( -4.458734124999997661, -86.22916666530107932, 2.574251347313722516 ) ) ;
#46272=CARTESIAN_POINT ( 'NONE',  ( 1.060575238724906964E-15, -27.62499999726881228, 5.773502691896257311 ) ) ;
#46273=CARTESIAN_POINT ( 'NONE',  ( 4.458734124999998549, -56.72916666530107932, -2.574251347313721627 ) ) ;
#46275=CARTESIAN_POINT ( 'NONE',  ( 6.123233995736766282E-16, -170.0000000000000000, -5.000000000000000000 ) ) ;
#46276=CARTESIAN_POINT ( 'NONE',  ( 2.499999999999998668, -62.20833333060214443, -4.330127018922193649 ) ) ;
#46277=CARTESIAN_POINT ( 'NONE',  ( 4.458734124999998549, -5.979166665301073103, -2.574251347313721627 ) ) ;
#46278=ORIENTED_EDGE ( 'NONE', *, *, #19163, .F. ) ;
#46279=CARTESIAN_POINT ( 'NONE',  ( -2.500000000000000444, -72.16666666666667140, -4.330127018922193649 ) ) ;
#46283=( BOUNDED_CURVE ( )  B_SPLINE_CURVE ( 2, ( #21001, #44471, #10707, #25823, #755, #429, #20035, #40294, #59932 ),
 .UNSPECIFIED., .F., .F. ) 
 B_SPLINE_CURVE_WITH_KNOTS ( ( 3, 2, 2, 2, 3 ),
 ( 0.8937500000000000444, 0.8944444444444444864, 0.8958333333333333703, 0.8972222222222222543, 0.8979166666666666963 ),
 .UNSPECIFIED. ) 
 CURVE ( )  GEOMETRIC_REPRESENTATION_ITEM ( )  RATIONAL_B_SPLINE_CURVE ( ( 0.9330127018922194093, 0.9330127018922194093, 1.000000000000000000, 0.8660254037844387076, 1.000000000000000000, 0.8660254037844387076, 1.000000000000000000, 0.9330127018922194093, 0.9330127018922194093 ) ) 
 REPRESENTATION_ITEM ( '' )  );
#46284=CARTESIAN_POINT ( 'NONE',  ( 5.000000000000000000, -69.37499999726880162, -6.123233995736766282E-16 ) ) ;
#46288=CARTESIAN_POINT ( 'NONE',  ( -4.458734124999999437, -15.56249999863440436, 0.000000000000000000 ) ) ;
#46289=CARTESIAN_POINT ( 'NONE',  ( -3.152548672688508926E-16, -53.81249999863439371, -5.148502694627439702 ) ) ;
#46292=CARTESIAN_POINT ( 'NONE',  ( 4.458734124999999437, -140.5000000013656347, 1.846868145590737864 ) ) ;
#46294=FACE_OUTER_BOUND ( 'NONE', #21339, .T. ) ;
#46295=ORIENTED_EDGE ( 'NONE', *, *, #25268, .F. ) ;
#46296=CARTESIAN_POINT ( 'NONE',  ( -2.071067811865644259, -155.6875000000000000, -4.999999999999831246 ) ) ;
#46297=CARTESIAN_POINT ( 'NONE',  ( 9.457646018065525792E-16, 23.68750000136559564, 5.148502694627439702 ) ) ;
#46302=CARTESIAN_POINT ( 'NONE',  ( 1.846868145590735200, -148.5000000013656347, -4.458734125000000326 ) ) ;
#46305=DIRECTION ( 'NONE',  ( 0.000000000000000000, 0.000000000000000000, 1.000000000000000000 ) ) ;
#46306=CARTESIAN_POINT ( 'NONE',  ( 2.229367062500001939, -65.22916666530106511, 3.861377020970579999 ) ) ;
#46309=CARTESIAN_POINT ( 'NONE',  ( -1.846868145590737420, -145.7500000013656063, 4.458734124999997661 ) ) ;
#46311=ORIENTED_EDGE ( 'NONE', *, *, #22893, .F. ) ;
#46312=CARTESIAN_POINT ( 'NONE',  ( 1.975475456537005874E-15, -48.74999999999999289, 5.000000000000000000 ) ) ;
#46313=CARTESIAN_POINT ( 'NONE',  ( 1.339745962155612702, 16.70534180126147916, -5.000000000000000000 ) ) ;
#46316=CARTESIAN_POINT ( 'NONE',  ( 4.458734124999999437, 26.93750000136559564, -5.460374474430324690E-16 ) ) ;
#46317=CARTESIAN_POINT ( 'NONE',  ( 1.975475456537005874E-15, 1.375000002731185500, 5.000000000000000000 ) ) ;
#46322=CARTESIAN_POINT ( 'NONE',  ( 1.339745962155624914, 21.70534180126147561, -4.999999999999991118 ) ) ;
#46323=CARTESIAN_POINT ( 'NONE',  ( -4.458734124999999437, 10.60416666803225993, -2.574251347313719407 ) ) ;
#46325=CARTESIAN_POINT ( 'NONE',  ( -4.458734124999997661, -19.47916666530107221, 2.574251347313722516 ) ) ;
#46327=CARTESIAN_POINT ( 'NONE',  ( -3.152801135295367985, -161.8125000013656063, 3.152801135295367096 ) ) ;
#46328=CARTESIAN_POINT ( 'NONE',  ( -6.972266317189433020E-16, -58.24999999999999289, -5.000000000000000000 ) ) ;
#46333=CARTESIAN_POINT ( 'NONE',  ( 6.123233995736766282E-16, -170.0000000000000000, -5.000000000000000000 ) ) ;
#46334=CARTESIAN_POINT ( 'NONE',  ( -6.972266317189433020E-16, 4.875000002731184168, -5.000000000000000000 ) ) ;
#46335=CARTESIAN_POINT ( 'NONE',  ( 2.229367062499998831, -33.64583333196772941, -3.861377020970580887 ) ) ;
#46338=CARTESIAN_POINT ( 'NONE',  ( -1.339745962155610925, -13.79465819873852261, 5.000000000000000000 ) ) ;
#46339=CARTESIAN_POINT ( 'NONE',  ( 5.000000000000000000, -68.29166666393547303, -2.886751345948130876 ) ) ;
#46340=ORIENTED_EDGE ( 'NONE', *, *, #32613, .F. ) ;
#46344=CARTESIAN_POINT ( 'NONE',  ( -5.000000000000000000, -9.083333333333333925, -2.886751345948128211 ) ) ;
#46345=CARTESIAN_POINT ( 'NONE',  ( 4.458734125000000326, -72.89583333196775072, 2.574251347313718519 ) ) ;
#46348=CARTESIAN_POINT ( 'NONE',  ( -3.535250795749689387E-16, -7.124999997268813168, -5.773502691896257311 ) ) ;
#46349=CARTESIAN_POINT ( 'NONE',  ( -4.458734124999998549, -37.22916666530107221, 2.574251347313722516 ) ) ;
#46353=CARTESIAN_POINT ( 'NONE',  ( -4.458734124999999437, 14.43750000136559386, 0.000000000000000000 ) ) ;
#46356=CARTESIAN_POINT ( 'NONE',  ( -5.000000000000000000, -56.99999999999999289, 0.000000000000000000 ) ) ;
#46357=CARTESIAN_POINT ( 'NONE',  ( 3.152801135295367541, -161.5625000013656063, -3.152801135295367541 ) ) ;
#46359=LINE ( 'NONE', #2619, #50178 ) ;
#46360=CARTESIAN_POINT ( 'NONE',  ( -4.458734124999999437, -80.31249999863440792, 0.000000000000000000 ) ) ;
#46361=CARTESIAN_POINT ( 'NONE',  ( -4.458734125000001214, -141.1250000013655779, 1.846868145590734089 ) ) ;
#46362=CARTESIAN_POINT ( 'NONE',  ( -2.229367062500000163, -85.47916666530107932, -3.861377020970580443 ) ) ;
#46364=( BOUNDED_CURVE ( )  B_SPLINE_CURVE ( 2, ( #40672, #50651, #41615, #1465, #25886, #16872, #21067, #16557, #35864 ),
 .UNSPECIFIED., .F., .F. ) 
 B_SPLINE_CURVE_WITH_KNOTS ( ( 3, 2, 2, 2, 3 ),
 ( 0.4770833333333333592, 0.4777777777777778012, 0.4791666666666666852, 0.4805555555555555691, 0.4812500000000000111 ),
 .UNSPECIFIED. ) 
 CURVE ( )  GEOMETRIC_REPRESENTATION_ITEM ( )  RATIONAL_B_SPLINE_CURVE ( ( 0.9330127018922194093, 0.9330127018922220739, 1.000000000000000000, 0.8660254037844387076, 1.000000000000000000, 0.8660254037844387076, 1.000000000000000000, 0.9330127018922194093, 0.9330127018922194093 ) ) 
 REPRESENTATION_ITEM ( '' )  );
#46366=CARTESIAN_POINT ( 'NONE',  ( 9.457646018065525792E-16, -33.31249999863440792, 5.148502694627439702 ) ) ;
#46367=CARTESIAN_POINT ( 'NONE',  ( -5.000000000000000000, 24.12500000273118417, 0.000000000000000000 ) ) ;
#46368=EDGE_LOOP ( 'NONE', ( #55507, #28968, #10362, #38420 ) ) ;
#46370=CARTESIAN_POINT ( 'NONE',  ( -1.339745962155613812, 15.91965820146970501, -5.000000000000000000 ) ) ;
#46372=CARTESIAN_POINT ( 'NONE',  ( -4.999999999999998224, -3.791666663935478798, 2.886751345948131764 ) ) ;
#46373=LINE ( 'NONE', #42171, #6537 ) ;
#46375=CARTESIAN_POINT ( 'NONE',  ( -2.229367062499996610, -64.39583333196773651, 3.861377020970582219 ) ) ;
#46377=ORIENTED_EDGE ( 'NONE', *, *, #31726, .F. ) ;
#46378=CARTESIAN_POINT ( 'NONE',  ( 0.000000000000000000, -170.0000000000000000, 0.000000000000000000 ) ) ;
#46379=( BOUNDED_CURVE ( )  B_SPLINE_CURVE ( 2, ( #12066, #41969, #37471, #46803, #27495, #31691, #61292, #52270, #17214 ),
 .UNSPECIFIED., .F., .F. ) 
 B_SPLINE_CURVE_WITH_KNOTS ( ( 3, 2, 2, 2, 3 ),
 ( 0.1270833333333333259, 0.1277777777777777679, 0.1291666666666666796, 0.1305555555555555636, 0.1312500000000000056 ),
 .UNSPECIFIED. ) 
 CURVE ( )  GEOMETRIC_REPRESENTATION_ITEM ( )  RATIONAL_B_SPLINE_CURVE ( ( 0.9330127018922194093, 0.9330127018922194093, 1.000000000000000000, 0.8660254037844387076, 1.000000000000000000, 0.8660254037844387076, 1.000000000000000000, 0.9330127018922194093, 0.9330127018922194093 ) ) 
 REPRESENTATION_ITEM ( '' )  );
#46384=CARTESIAN_POINT ( 'NONE',  ( -3.152548672688508926E-16, 10.43750000136559386, -5.148502694627439702 ) ) ;
#46385=CARTESIAN_POINT ( 'NONE',  ( -1.339745962155610925, -32.66965819600733312, 5.000000000000000000 ) ) ;
#46386=CARTESIAN_POINT ( 'NONE',  ( -3.152801135295367985, -156.8125000013656063, 3.152801135295367096 ) ) ;
#46387=CARTESIAN_POINT ( 'NONE',  ( 3.061616997868383141E-16, -145.7500000000000284, -5.000000000000000000 ) ) ;
#46388=ORIENTED_EDGE ( 'NONE', *, *, #53014, .T. ) ;
#46390=LINE ( 'NONE', #39952, #49019 ) ;
#46394=CARTESIAN_POINT ( 'NONE',  ( 2.500000000000002220, -78.66666666666665719, 4.330127018922192761 ) ) ;
#46396=CARTESIAN_POINT ( 'NONE',  ( -4.458734124999999437, 28.60416666803226349, -2.574251347313719407 ) ) ;
#46399=CARTESIAN_POINT ( 'NONE',  ( 9.457646018065525792E-16, -0.3124999986344051961, 5.148502694627439702 ) ) ;
#46402=CARTESIAN_POINT ( 'NONE',  ( -5.000000000000000888, -144.6875000027311842, -2.071067811865475949 ) ) ;
#46403=FACE_OUTER_BOUND ( 'NONE', #60051, .T. ) ;
#46406=EDGE_CURVE ( 'NONE', #39890, #1596, #13967, .T. ) ;
#46409=EDGE_CURVE ( 'NONE', #30399, #58407, #20047, .T. ) ;
#46410=EDGE_CURVE ( 'NONE', #12181, #18978, #24464, .T. ) ;
#46412=CARTESIAN_POINT ( 'NONE',  ( 4.458734124999997661, -161.7500000013655779, 1.846868145590737864 ) ) ;
#46416=VERTEX_POINT ( 'NONE', #44707 ) ;
#46417=CARTESIAN_POINT ( 'NONE',  ( 2.229367062499998831, 21.10416666803226349, -3.861377020970580887 ) ) ;
#46418=ORIENTED_EDGE ( 'NONE', *, *, #33149, .F. ) ;
#46423=CARTESIAN_POINT ( 'NONE',  ( 2.499999999999998668, 6.666666666666667851, -4.330127018922193649 ) ) ;
#46424=EDGE_CURVE ( 'NONE', #42274, #28232, #4829, .T. ) ;
#46425=CARTESIAN_POINT ( 'NONE',  ( 4.458734124999998549, -55.72916666530107221, -2.574251347313721627 ) ) ;
#46426=CARTESIAN_POINT ( 'NONE',  ( 5.000000000000000000, -6.416666666666667851, -2.886751345948130876 ) ) ;
#46430=ADVANCED_FACE ( 'NONE', ( #9043 ), #23840, .T. ) ;
#46432=CARTESIAN_POINT ( 'NONE',  ( 2.499999999999998668, -42.33333333333333570, -4.330127018922193649 ) ) ;
#46433=CARTESIAN_POINT ( 'NONE',  ( 1.975475456537005874E-15, -50.62499999726881583, 5.000000000000000000 ) ) ;
#46435=( BOUNDED_CURVE ( )  B_SPLINE_CURVE ( 2, ( #57888, #19260, #15080, #62719, #58191, #43391, #10257, #29858, #4174 ),
 .UNSPECIFIED., .F., .F. ) 
 B_SPLINE_CURVE_WITH_KNOTS ( ( 3, 2, 2, 2, 3 ),
 ( 0.7895833333333333037, 0.7902777777777777457, 0.7916666666666666297, 0.7930555555555555136, 0.7937499999999999556 ),
 .UNSPECIFIED. ) 
 CURVE ( )  GEOMETRIC_REPRESENTATION_ITEM ( )  RATIONAL_B_SPLINE_CURVE ( ( 0.9330127018922194093, 0.9330127018922194093, 1.000000000000000000, 0.8660254037844387076, 1.000000000000000000, 0.8660254037844387076, 1.000000000000000000, 0.9330127018922194093, 0.9330127018922194093 ) ) 
 REPRESENTATION_ITEM ( '' )  );
#46438=CARTESIAN_POINT ( 'NONE',  ( -4.458734124999999437, -57.31249999863440081, 0.000000000000000000 ) ) ;
#46439=CARTESIAN_POINT ( 'NONE',  ( -8.190561711645485556E-16, -153.9375000013655779, 4.458734124999999437 ) ) ;
#46440=CARTESIAN_POINT ( 'NONE',  ( 9.457646018065525792E-16, -73.06249999863440792, 5.148502694627439702 ) ) ;
#46442=CARTESIAN_POINT ( 'NONE',  ( 4.458734125000001214, -21.14583333196774362, 2.574251347313718519 ) ) ;
#46443=CARTESIAN_POINT ( 'NONE',  ( 5.000000000000000000, -58.37499999726880873, -6.123233995736766282E-16 ) ) ;
#46444=ORIENTED_EDGE ( 'NONE', *, *, #19304, .T. ) ;
#46445=LINE ( 'NONE', #56097, #57999 ) ;
#46450=CARTESIAN_POINT ( 'NONE',  ( 3.152801135295367541, -152.3125000013655779, -3.152801135295367541 ) ) ;
#46451=VERTEX_POINT ( 'NONE', #44070 ) ;
#46452=CARTESIAN_POINT ( 'NONE',  ( 6.123233995736766282E-16, -170.0000000000000000, -5.000000000000000000 ) ) ;
#46454=CARTESIAN_POINT ( 'NONE',  ( 1.975475456537005874E-15, -77.62499999726881583, 5.000000000000000000 ) ) ;
#46455=CARTESIAN_POINT ( 'NONE',  ( -2.229367062499996610, -47.39583333196774362, 3.861377020970582219 ) ) ;
#46459=CARTESIAN_POINT ( 'NONE',  ( 4.458734124999998549, 26.27083333469893134, -2.574251347313721627 ) ) ;
#46462=CARTESIAN_POINT ( 'NONE',  ( 2.730187237215162345E-16, -167.1875000013655779, -4.458734124999999437 ) ) ;
#46463=ORIENTED_EDGE ( 'NONE', *, *, #35884, .F. ) ;
#46471=CARTESIAN_POINT ( 'NONE',  ( 3.061616997868383141E-16, -160.7500000000000000, -5.000000000000000000 ) ) ;
#46475=( BOUNDED_CURVE ( )  B_SPLINE_CURVE ( 2, ( #57430, #58669, #47754, #32973, #29374, #49006, #52903, #33596, #33284 ),
 .UNSPECIFIED., .F., .F. ) 
 B_SPLINE_CURVE_WITH_KNOTS ( ( 3, 2, 2, 2, 3 ),
 ( 0.9895833333333333703, 0.9902777777777778123, 0.9916666666666666963, 0.9930555555555555802, 0.9937500000000000222 ),
 .UNSPECIFIED. ) 
 CURVE ( )  GEOMETRIC_REPRESENTATION_ITEM ( )  RATIONAL_B_SPLINE_CURVE ( ( 0.9330127018922194093, 0.9330127018922194093, 1.000000000000000000, 0.8660254037844387076, 1.000000000000000000, 0.8660254037844387076, 1.000000000000000000, 0.9330127018922194093, 0.9330127018922194093 ) ) 
 REPRESENTATION_ITEM ( '' )  );
#46478=CARTESIAN_POINT ( 'NONE',  ( 2.071067811865475505, -157.9375000027312410, -5.000000000000000888 ) ) ;
#46479=ORIENTED_EDGE ( 'NONE', *, *, #49152, .T. ) ;
#46484=CARTESIAN_POINT ( 'NONE',  ( -9.184850993605147944E-16, -147.2500000000000284, 5.000000000000000000 ) ) ;
#46489=CARTESIAN_POINT ( 'NONE',  ( 4.458734124999998549, -22.72916666530107221, -2.574251347313721627 ) ) ;
#46491=CARTESIAN_POINT ( 'NONE',  ( -3.535533905932738641, -152.3750000000000000, 3.535533905932737309 ) ) ;
#46493=CARTESIAN_POINT ( 'NONE',  ( -8.190561711645485556E-16, -151.6875000013656063, 4.458734124999999437 ) ) ;
#46494=EDGE_LOOP ( 'NONE', ( #53162, #20813, #18509, #35313 ) ) ;
#46496=CARTESIAN_POINT ( 'NONE',  ( -4.458734124999999437, -49.56249999863440792, 0.000000000000000000 ) ) ;
#46500=CARTESIAN_POINT ( 'NONE',  ( -3.535250795749689387E-16, 23.75000000000000000, -5.773502691896257311 ) ) ;
#46504=CARTESIAN_POINT ( 'NONE',  ( -2.229367062499996610, 6.854166668032259935, 3.861377020970582219 ) ) ;
#46505=CARTESIAN_POINT ( 'NONE',  ( -2.071067811865562991, -142.3125000000000000, 4.999999999999913847 ) ) ;
#46507=CARTESIAN_POINT ( 'NONE',  ( -2.500000000000000444, -74.16666666666665719, -4.330127018922193649 ) ) ;
#46508=CARTESIAN_POINT ( 'NONE',  ( 4.458734124999998549, 18.02083333469892779, -2.574251347313721627 ) ) ;
#46509=CARTESIAN_POINT ( 'NONE',  ( -2.499999999999996447, 5.291666669397853795, 4.330127018922195425 ) ) ;
#46512=CARTESIAN_POINT ( 'NONE',  ( -4.764381983412779477E-15, 26.25000000000000000, 5.000000000000000000 ) ) ;
#46513=EDGE_LOOP ( 'NONE', ( #61570, #44372, #9717, #5420 ) ) ;
#46514=CARTESIAN_POINT ( 'NONE',  ( -1.339745962155613812, -71.20534180126148271, -5.000000000000000000 ) ) ;
#46515=CARTESIAN_POINT ( 'NONE',  ( -4.458734124999999437, -45.31249999863440081, 0.000000000000000000 ) ) ;
#46516=EDGE_CURVE ( 'NONE', #53481, #40578, #31639, .T. ) ;
#46517=CARTESIAN_POINT ( 'NONE',  ( 4.458734125000000326, -165.6250000013656063, -1.846868145590734978 ) ) ;
#46518=EDGE_CURVE ( 'NONE', #44762, #45336, #57936, .T. ) ;
#46519=CARTESIAN_POINT ( 'NONE',  ( -2.499999999999996447, -43.70833333060214443, 4.330127018922195425 ) ) ;
#46520=VERTEX_POINT ( 'NONE', #55664 ) ;
#46521=CARTESIAN_POINT ( 'NONE',  ( -2.229367062499996610, -17.14583333196773651, 3.861377020970582219 ) ) ;
#46522=ORIENTED_EDGE ( 'NONE', *, *, #26024, .T. ) ;
#46523=CARTESIAN_POINT ( 'NONE',  ( 5.000000000000000000, -85.49999999999998579, -6.123233995736766282E-16 ) ) ;
#46524=CARTESIAN_POINT ( 'NONE',  ( 1.846868145590735200, -165.2500000013655779, -4.458734125000000326 ) ) ;
#46525=CARTESIAN_POINT ( 'NONE',  ( 5.000000000000000888, -20.45833333060214798, 2.886751345948126879 ) ) ;
#46526=ORIENTED_EDGE ( 'NONE', *, *, #45389, .T. ) ;
#46528=CARTESIAN_POINT ( 'NONE',  ( 4.458734125000001214, -32.14583333196773651, 2.574251347313718519 ) ) ;
#46530=ORIENTED_EDGE ( 'NONE', *, *, #11135, .F. ) ;
#46533=CARTESIAN_POINT ( 'NONE',  ( 5.000000000000000000, 24.70833333606452342, -2.886751345948130876 ) ) ;
#46537=CARTESIAN_POINT ( 'NONE',  ( -4.458734124999999437, -82.64583333196772230, -2.574251347313719407 ) ) ;
#46539=CARTESIAN_POINT ( 'NONE',  ( 5.000000000000000000, 22.58333333333333215, -2.886751345948130876 ) ) ;
#46541=CARTESIAN_POINT ( 'NONE',  ( 1.975475456537005874E-15, -84.62499999726880162, 5.000000000000000000 ) ) ;
#46543=CARTESIAN_POINT ( 'NONE',  ( -2.229367062500000163, -47.47916666530106511, -3.861377020970580443 ) ) ;
#46546=CARTESIAN_POINT ( 'NONE',  ( 0.000000000000000000, -170.0000000000000000, 0.000000000000000000 ) ) ;
#46551=CARTESIAN_POINT ( 'NONE',  ( -2.229367062500000163, -77.72916666530106511, -3.861377020970580443 ) ) ;
#46559=CARTESIAN_POINT ( 'NONE',  ( -3.535533905932738641, -167.5000000027312126, 3.535533905932737309 ) ) ;
#46561=CARTESIAN_POINT ( 'NONE',  ( 2.229367062500001939, 11.77083333469892601, 3.861377020970579999 ) ) ;
#46563=( BOUNDED_CURVE ( )  B_SPLINE_CURVE ( 2, ( #21464, #32688, #47476, #18529, #33316, #38445, #22735, #2799, #12751 ),
 .UNSPECIFIED., .F., .F. ) 
 B_SPLINE_CURVE_WITH_KNOTS ( ( 3, 2, 2, 2, 3 ),
 ( 0.7916666666666664076, 0.7958333333333330595, 0.7999999999999998224, 0.8041666666666664742, 0.8083333333333331261 ),
 .UNSPECIFIED. ) 
 CURVE ( )  GEOMETRIC_REPRESENTATION_ITEM ( )  RATIONAL_B_SPLINE_CURVE ( ( 1.000000000000003997, 0.9238795325112826307, 1.000000000000000000, 0.9238795325112867385, 1.000000000000000000, 0.9238795325112867385, 1.000000000000000000, 0.9238795325112908463, 0.9999999999999958922 ) ) 
 REPRESENTATION_ITEM ( '' )  );
#46568=CARTESIAN_POINT ( 'NONE',  ( -5.000000000000000000, -13.95833333060214976, -2.886751345948128211 ) ) ;
#46569=CARTESIAN_POINT ( 'NONE',  ( 5.000000000000000000, 17.50000000000000000, -6.123233995736766282E-16 ) ) ;
#46570=CARTESIAN_POINT ( 'NONE',  ( -3.152548672688508926E-16, -8.562499998634406140, -5.148502694627439702 ) ) ;
#46571=DIRECTION ( 'NONE',  ( -0.000000000000000000, 1.000000000000000000, -0.000000000000000000 ) ) ;
#46573=CARTESIAN_POINT ( 'NONE',  ( -2.229367062500000163, -34.72916666530107221, -3.861377020970580443 ) ) ;
#46577=CARTESIAN_POINT ( 'NONE',  ( 2.730187237215162345E-16, -148.4375000013656063, -4.458734124999999437 ) ) ;
#46578=VECTOR ( 'NONE', #51524, 1000.000000000000000 ) ;
#46579=CARTESIAN_POINT ( 'NONE',  ( 2.229367062500001939, 23.02083333469892423, 3.861377020970579999 ) ) ;
#46580=CARTESIAN_POINT ( 'NONE',  ( -1.339745962155613812, -44.08034179853027723, -5.000000000000000000 ) ) ;
#46582=CARTESIAN_POINT ( 'NONE',  ( -2.229367062500000163, -84.72916666530107932, -3.861377020970580443 ) ) ;
#46584=CARTESIAN_POINT ( 'NONE',  ( -5.000000000000000000, 21.04166666939785202, -2.886751345948128211 ) ) ;
#46585=ORIENTED_EDGE ( 'NONE', *, *, #44001, .F. ) ;
#46586=CARTESIAN_POINT ( 'NONE',  ( 2.500000000000002220, -25.66666666666666430, 4.330127018922192761 ) ) ;
#46588=CYLINDRICAL_SURFACE ( 'NONE', #42927, 5.000000000000000000 ) ;
#46589=CARTESIAN_POINT ( 'NONE',  ( 5.000000000000000000, -23.50000000000000000, -6.123233995736766282E-16 ) ) ;
#46590=CARTESIAN_POINT ( 'NONE',  ( -2.229367062499996610, -25.14583333196773651, 3.861377020970582219 ) ) ;
#46591=CARTESIAN_POINT ( 'NONE',  ( -4.458734124999999437, -89.39583333196773651, -2.574251347313719407 ) ) ;
#46592=CARTESIAN_POINT ( 'NONE',  ( -3.535250795749689387E-16, -31.12499999726881228, -5.773502691896257311 ) ) ;
#46593=CARTESIAN_POINT ( 'NONE',  ( 9.457646018065525792E-16, -54.06249999863440081, 5.148502694627439702 ) ) ;
#46596=CARTESIAN_POINT ( 'NONE',  ( -2.229367062500000163, -9.729166665301068662, -3.861377020970580443 ) ) ;
#46598=CARTESIAN_POINT ( 'NONE',  ( -2.499999999999996447, -71.83333333333332860, 4.330127018922195425 ) ) ;
#46602=CARTESIAN_POINT ( 'NONE',  ( 2.500000000000002220, -75.54166666393547303, 4.330127018922192761 ) ) ;
#46603=CARTESIAN_POINT ( 'NONE',  ( -2.499999999999996447, -53.70833333060213732, 4.330127018922195425 ) ) ;
#46605=CARTESIAN_POINT ( 'NONE',  ( 2.229367062500001939, -15.22916666530107399, 3.861377020970579999 ) ) ;
#46606=CARTESIAN_POINT ( 'NONE',  ( 2.229367062499998831, -50.89583333196772941, -3.861377020970580887 ) ) ;
#46607=CARTESIAN_POINT ( 'NONE',  ( -2.499999999999996447, -29.70833333060215153, 4.330127018922195425 ) ) ;
#46608=CARTESIAN_POINT ( 'NONE',  ( -3.152801135295367096, -140.0625000013655779, -3.152801135295367541 ) ) ;
#46614=CARTESIAN_POINT ( 'NONE',  ( 2.499999999999998668, 18.66666666666666430, -4.330127018922193649 ) ) ;
#46617=VECTOR ( 'NONE', #31574, 1000.000000000000000 ) ;
#46618=CARTESIAN_POINT ( 'NONE',  ( 4.458734124999999437, -146.7500000013656063, 1.846868145590737864 ) ) ;
#46621=CARTESIAN_POINT ( 'NONE',  ( 2.229367062500001939, -61.22916666530106511, 3.861377020970579999 ) ) ;
#46622=CARTESIAN_POINT ( 'NONE',  ( -9.184850993605147944E-16, -154.3750000027311842, 5.000000000000000000 ) ) ;
#46624=CARTESIAN_POINT ( 'NONE',  ( 4.458734124999997661, -145.5000000013656063, 1.846868145590737864 ) ) ;
#46629=CARTESIAN_POINT ( 'NONE',  ( 5.000000000000000000, 16.58333333333333215, -2.886751345948130876 ) ) ;
#46633=CARTESIAN_POINT ( 'NONE',  ( -2.229367062500000163, 28.27083333469892779, -3.861377020970580443 ) ) ;
#46634=CARTESIAN_POINT ( 'NONE',  ( -2.500000000000000444, -18.04166666393547658, -4.330127018922193649 ) ) ;
#46641=CARTESIAN_POINT ( 'NONE',  ( 4.458734124999998549, 8.270833334698926009, -2.574251347313721627 ) ) ;
#46643=CARTESIAN_POINT ( 'NONE',  ( 9.457646018065525792E-16, -18.31249999863440792, 5.148502694627439702 ) ) ;
#46645=CARTESIAN_POINT ( 'NONE',  ( 3.152801135295366208, -161.5625000013656063, 3.152801135295367985 ) ) ;
#46646=CARTESIAN_POINT ( 'NONE',  ( 5.000000000000000000, 15.62500000273118417, -6.123233995736766282E-16 ) ) ;
#46649=CARTESIAN_POINT ( 'NONE',  ( -2.500000000000000444, -89.04166666393547303, -4.330127018922193649 ) ) ;
#46650=CARTESIAN_POINT ( 'NONE',  ( 4.458734124999999437, -41.81249999863440081, -5.460374474430324690E-16 ) ) ;
#46651=CARTESIAN_POINT ( 'NONE',  ( 5.000000000000000888, 19.54166666939785202, 2.886751345948126879 ) ) ;
#46652=CARTESIAN_POINT ( 'NONE',  ( 4.458734125000000326, -66.14583333196773651, 2.574251347313718519 ) ) ;
#46655=ORIENTED_EDGE ( 'NONE', *, *, #3660, .T. ) ;
#46656=CARTESIAN_POINT ( 'NONE',  ( -5.000000000000000000, -84.99999999999998579, 0.000000000000000000 ) ) ;
#46659=CARTESIAN_POINT ( 'NONE',  ( -5.000000000000000000, -67.95833333060214443, -2.886751345948128211 ) ) ;
#46660=CARTESIAN_POINT ( 'NONE',  ( 2.499999999999998668, -7.333333333333330373, -4.330127018922193649 ) ) ;
#46661=CARTESIAN_POINT ( 'NONE',  ( -4.458734124999999437, -71.31249999863439371, 0.000000000000000000 ) ) ;
#46664=CARTESIAN_POINT ( 'NONE',  ( -4.999999999999999112, -14.79166666393548368, 2.886751345948131764 ) ) ;
#46665=CARTESIAN_POINT ( 'NONE',  ( -2.229367062499996610, -40.14583333196773651, 3.861377020970582219 ) ) ;
#46666=ORIENTED_EDGE ( 'NONE', *, *, #2429, .F. ) ;
#46668=CARTESIAN_POINT ( 'NONE',  ( 4.458734124999998549, 10.02083333469892779, -2.574251347313721627 ) ) ;
#46669=ORIENTED_EDGE ( 'NONE', *, *, #37851, .T. ) ;
#46670=CARTESIAN_POINT ( 'NONE',  ( 5.000000000000000000, -81.37499999726881583, -6.123233995736766282E-16 ) ) ;
#46671=CARTESIAN_POINT ( 'NONE',  ( -4.999999999999999112, -56.91666666666667140, 2.886751345948131764 ) ) ;
#46672=CARTESIAN_POINT ( 'NONE',  ( 4.458734125000000326, -160.6250000013655779, -1.846868145590734978 ) ) ;
#46675=CARTESIAN_POINT ( 'NONE',  ( 2.229367062500001939, -79.97916666530106511, 3.861377020970579999 ) ) ;
#46676=CARTESIAN_POINT ( 'NONE',  ( 5.000000000000000000, -168.0625000000000000, 2.071067811865478614 ) ) ;
#46677=CARTESIAN_POINT ( 'NONE',  ( 4.458734124999999437, -87.81249999863439371, -5.460374474430324690E-16 ) ) ;
#46679=CARTESIAN_POINT ( 'NONE',  ( 4.458734124999999437, -1.062499998634405696, -5.460374474430324690E-16 ) ) ;
#46680=CARTESIAN_POINT ( 'NONE',  ( -2.229367062499996610, -36.39583333196773651, 3.861377020970582219 ) ) ;
#46682=CYLINDRICAL_SURFACE ( 'NONE', #37931, 5.000000000000000000 ) ;
#46684=CARTESIAN_POINT ( 'NONE',  ( -9.184850993605147944E-16, -148.3750000027312126, 5.000000000000000000 ) ) ;
#46686=CARTESIAN_POINT ( 'NONE',  ( 2.229367062500001939, -70.22916666530107932, 3.861377020970579999 ) ) ;
#46689=VERTEX_POINT ( 'NONE', #45677 ) ;
#46690=FACE_OUTER_BOUND ( 'NONE', #22188, .T. ) ;
#46691=CARTESIAN_POINT ( 'NONE',  ( 2.500000000000002220, -3.541666663935478354, 4.330127018922192761 ) ) ;
#46694=CARTESIAN_POINT ( 'NONE',  ( 2.229367062500001939, 0.02083333469892964529, 3.861377020970579999 ) ) ;
#46695=CARTESIAN_POINT ( 'NONE',  ( 4.458734124999999437, -155.4375000013655779, 0.000000000000000000 ) ) ;
#46697=ORIENTED_EDGE ( 'NONE', *, *, #20051, .F. ) ;
#46702=AXIS2_PLACEMENT_3D ( 'NONE', #9698, #29305, #48935 ) ;
#46704=CARTESIAN_POINT ( 'NONE',  ( 3.061616997868383141E-16, -160.7500000000000000, -5.000000000000000000 ) ) ;
#46706=EDGE_CURVE ( 'NONE', #45160, #31680, #37715, .T. ) ;
#46707=FACE_OUTER_BOUND ( 'NONE', #6905, .T. ) ;
#46710=CARTESIAN_POINT ( 'NONE',  ( -4.458734124999999437, 25.60416666803225638, -2.574251347313719407 ) ) ;
#46712=CARTESIAN_POINT ( 'NONE',  ( -3.152548672688508926E-16, -4.812499998634402587, -5.148502694627439702 ) ) ;
#46713=CARTESIAN_POINT ( 'NONE',  ( 5.000000000000000888, -0.4583333306021481479, 2.886751345948126879 ) ) ;
#46715=CARTESIAN_POINT ( 'NONE',  ( -5.000000000000000000, -142.6250000027312126, -6.123233995736766282E-16 ) ) ;
#46720=CARTESIAN_POINT ( 'NONE',  ( -2.499999999999996447, -86.83333333333332860, 4.330127018922195425 ) ) ;
#46723=CARTESIAN_POINT ( 'NONE',  ( 3.152801135295367541, -163.5625000013656063, -3.152801135295367541 ) ) ;
#46726=EDGE_LOOP ( 'NONE', ( #43083, #41214, #41531, #1136 ) ) ;
#46727=CARTESIAN_POINT ( 'NONE',  ( 2.229367062499998831, 16.10416666803225993, -3.861377020970580887 ) ) ;
#46733=CARTESIAN_POINT ( 'NONE',  ( 5.000000000000000000, 7.583333333333333925, -2.886751345948129988 ) ) ;
#46734=( BOUNDED_CURVE ( )  B_SPLINE_CURVE ( 2, ( #20470, #40072, #12720, #32340, #47140, #22385, #46507, #17862, #3087 ),
 .UNSPECIFIED., .F., .F. ) 
 B_SPLINE_CURVE_WITH_KNOTS ( ( 3, 2, 2, 2, 3 ),
 ( 0.8645833333333333703, 0.8652777777777778123, 0.8666666666666666963, 0.8680555555555555802, 0.8687500000000000222 ),
 .UNSPECIFIED. ) 
 CURVE ( )  GEOMETRIC_REPRESENTATION_ITEM ( )  RATIONAL_B_SPLINE_CURVE ( ( 0.9330127018922194093, 0.9330127018922194093, 1.000000000000000000, 0.8660254037844387076, 1.000000000000000000, 0.8660254037844387076, 1.000000000000000000, 0.9330127018922194093, 0.9330127018922194093 ) ) 
 REPRESENTATION_ITEM ( '' )  );
#46735=CARTESIAN_POINT ( 'NONE',  ( -4.458734124999999437, -55.39583333196773651, -2.574251347313719407 ) ) ;
#46742=CARTESIAN_POINT ( 'NONE',  ( -6.972266317189433020E-16, -25.12499999726881228, -5.000000000000000000 ) ) ;
#46743=CARTESIAN_POINT ( 'NONE',  ( -5.000000000000000000, -40.99999999999999289, 0.000000000000000000 ) ) ;
#46744=CYLINDRICAL_SURFACE ( 'NONE', #8909, 5.000000000000000000 ) ;
#46745=CARTESIAN_POINT ( 'NONE',  ( -2.499999999999996447, -47.83333333333332149, 4.330127018922195425 ) ) ;
#46747=CARTESIAN_POINT ( 'NONE',  ( -1.339745962155613812, 12.79465819873851906, -5.000000000000000000 ) ) ;
#46748=CARTESIAN_POINT ( 'NONE',  ( 4.458734124999998549, -63.72916666530107221, -2.574251347313721627 ) ) ;
#46749=CARTESIAN_POINT ( 'NONE',  ( -1.846868145590734756, -151.3750000013656063, -4.458734125000000326 ) ) ;
#46750=CARTESIAN_POINT ( 'NONE',  ( 4.458734124999999437, -71.81249999863439371, -5.460374474430324690E-16 ) ) ;
#46752=CARTESIAN_POINT ( 'NONE',  ( 2.229367062500001939, -20.22916666530107221, 3.861377020970579999 ) ) ;
#46754=CARTESIAN_POINT ( 'NONE',  ( 2.499999999999998668, -59.20833333060214443, -4.330127018922193649 ) ) ;
#46756=CARTESIAN_POINT ( 'NONE',  ( 5.000000000000000000, -31.37499999726880873, -6.123233995736766282E-16 ) ) ;
#46757=VERTEX_POINT ( 'NONE', #1636 ) ;
#46761=CARTESIAN_POINT ( 'NONE',  ( 1.846868145590736310, -151.6250000013656063, 4.458734124999999437 ) ) ;
#46762=ORIENTED_EDGE ( 'NONE', *, *, #60157, .T. ) ;
#46763=CARTESIAN_POINT ( 'NONE',  ( 3.535533905932738197, -155.0000000027312126, -3.535533905932738197 ) ) ;
#46765=CARTESIAN_POINT ( 'NONE',  ( 1.339745962155615144, -8.705341801261482715, 4.999999999999999112 ) ) ;
#46766=CARTESIAN_POINT ( 'NONE',  ( 2.229367062499998831, -51.89583333196773651, -3.861377020970580887 ) ) ;
#46767=EDGE_CURVE ( 'NONE', #44335, #45731, #8972, .T. ) ;
#46769=CARTESIAN_POINT ( 'NONE',  ( 0.000000000000000000, -170.0000000000000000, 0.000000000000000000 ) ) ;
#46771=CARTESIAN_POINT ( 'NONE',  ( 4.458734125000001214, 25.10416666803225638, 2.574251347313718519 ) ) ;
#46773=CARTESIAN_POINT ( 'NONE',  ( 5.000000000000000000, -13.29166666393548191, -2.886751345948130876 ) ) ;
#46774=CARTESIAN_POINT ( 'NONE',  ( -9.184850993605147944E-16, -165.2500000000000000, 5.000000000000000000 ) ) ;
#46782=EDGE_CURVE ( 'NONE', #19199, #56488, #36031, .T. ) ;
#46787=ADVANCED_FACE ( 'NONE', ( #40842 ), #59849, .T. ) ;
#46792=CARTESIAN_POINT ( 'NONE',  ( 2.071067811865475505, -153.9375000027312126, -5.000000000000000888 ) ) ;
#46793=ORIENTED_EDGE ( 'NONE', *, *, #23973, .T. ) ;
#46798=CARTESIAN_POINT ( 'NONE',  ( 5.000000000000000000, -147.0000000000000284, 0.000000000000000000 ) ) ;
#46802=CARTESIAN_POINT ( 'NONE',  ( -4.458734124999999437, -23.39583333196773651, -2.574251347313719407 ) ) ;
#46803=CARTESIAN_POINT ( 'NONE',  ( 5.000000000000000000, 14.58333333333333215, -2.886751345948130876 ) ) ;
#46804=CARTESIAN_POINT ( 'NONE',  ( -1.339745962155613812, 8.919658201469705006, -5.000000000000000000 ) ) ;
#46806=CARTESIAN_POINT ( 'NONE',  ( -1.846868145590734756, -152.1250000013655779, -4.458734125000000326 ) ) ;
#46809=CARTESIAN_POINT ( 'NONE',  ( -2.229367062500000163, -53.72916666530107221, -3.861377020970580443 ) ) ;
#46810=( BOUNDED_CURVE ( )  B_SPLINE_CURVE ( 2, ( #21897, #46338, #15485, #1658, #31218, #45062, #25770, #40551, #1028 ),
 .UNSPECIFIED., .F., .F. ) 
 B_SPLINE_CURVE_WITH_KNOTS ( ( 3, 2, 2, 2, 3 ),
 ( 0.3645833333333333148, 0.3652777777777777568, 0.3666666666666666408, 0.3680555555555555802, 0.3687500000000000222 ),
 .UNSPECIFIED. ) 
 CURVE ( )  GEOMETRIC_REPRESENTATION_ITEM ( )  RATIONAL_B_SPLINE_CURVE ( ( 0.9330127018922194093, 0.9330127018922194093, 1.000000000000000000, 0.8660254037844387076, 1.000000000000000000, 0.8660254037844387076, 1.000000000000000000, 0.9330127018922194093, 0.9330127018922194093 ) ) 
 REPRESENTATION_ITEM ( '' )  );
#46813=CARTESIAN_POINT ( 'NONE',  ( 5.000000000000000000, 25.58333333333333215, -2.886751345948129988 ) ) ;
#46815=DIRECTION ( 'NONE',  ( -0.000000000000000000, 1.000000000000000000, -0.000000000000000000 ) ) ;
#46816=CARTESIAN_POINT ( 'NONE',  ( -3.152548672688508926E-16, 0.4375000013655955255, -5.148502694627439702 ) ) ;
#46817=CARTESIAN_POINT ( 'NONE',  ( -2.500000000000000444, -74.04166666393547303, -4.330127018922193649 ) ) ;
#46820=CARTESIAN_POINT ( 'NONE',  ( -4.458734124999999437, 16.35416666803225993, -2.574251347313719407 ) ) ;
#46821=CARTESIAN_POINT ( 'NONE',  ( -2.499999999999996447, 4.291666669397852907, 4.330127018922195425 ) ) ;
#46822=VERTEX_POINT ( 'NONE', #42743 ) ;
#46825=CARTESIAN_POINT ( 'NONE',  ( 1.975475456537005874E-15, -7.624999997268812280, 5.000000000000000000 ) ) ;
#46826=CARTESIAN_POINT ( 'NONE',  ( -2.229367062499996610, -48.14583333196772941, 3.861377020970582219 ) ) ;
#46827=CARTESIAN_POINT ( 'NONE',  ( -3.152801135295367096, -163.3125000013656063, -3.152801135295367541 ) ) ;
#46828=CARTESIAN_POINT ( 'NONE',  ( -5.000000000000000000, -45.87499999726880873, 0.000000000000000000 ) ) ;
#46829=ORIENTED_EDGE ( 'NONE', *, *, #43719, .T. ) ;
#46830=CARTESIAN_POINT ( 'NONE',  ( 9.457646018065525792E-16, -25.06249999863440792, 5.148502694627439702 ) ) ;
#46832=CARTESIAN_POINT ( 'NONE',  ( -4.999999999999999112, -87.91666666666667140, 2.886751345948131764 ) ) ;
#46833=CARTESIAN_POINT ( 'NONE',  ( 2.730187237215162345E-16, -163.1875000013655779, -4.458734124999999437 ) ) ;
#46836=CARTESIAN_POINT ( 'NONE',  ( -4.458734124999999437, -34.56249999863440792, 0.000000000000000000 ) ) ;
#46838=ORIENTED_EDGE ( 'NONE', *, *, #60078, .T. ) ;
#46841=ADVANCED_FACE ( 'NONE', ( #41797 ), #52098, .T. ) ;
#46844=EDGE_CURVE ( 'NONE', #42676, #25930, #61962, .T. ) ;
#46845=VERTEX_POINT ( 'NONE', #27328 ) ;
#46848=CARTESIAN_POINT ( 'NONE',  ( 2.229367062500001939, -79.22916666530106511, 3.861377020970579999 ) ) ;
#46851=CARTESIAN_POINT ( 'NONE',  ( 1.975475456537005874E-15, -23.62499999726880873, 5.000000000000000000 ) ) ;
#46852=( BOUNDED_CURVE ( )  B_SPLINE_CURVE ( 2, ( #63155, #34176, #5239, #58007, #48967, #4919, #24538, #38683, #19389 ),
 .UNSPECIFIED., .F., .F. ) 
 B_SPLINE_CURVE_WITH_KNOTS ( ( 3, 2, 2, 2, 3 ),
 ( 0.5416666666666671848, 0.5458333333333338366, 0.5500000000000004885, 0.5541666666666671404, 0.5583333333333337922 ),
 .UNSPECIFIED. ) 
 CURVE ( )  GEOMETRIC_REPRESENTATION_ITEM ( )  RATIONAL_B_SPLINE_CURVE ( ( 0.9999999999999898970, 0.9238795325112968415, 1.000000000000000000, 0.9238795325112867385, 1.000000000000000000, 0.9238795325112867385, 1.000000000000000000, 0.9238795325112786339, 1.000000000000008216 ) ) 
 REPRESENTATION_ITEM ( '' )  );
#46855=CARTESIAN_POINT ( 'NONE',  ( 4.458734124999999437, -44.81249999863440081, -5.460374474430324690E-16 ) ) ;
#46858=EDGE_CURVE ( 'NONE', #20760, #44027, #48775, .T. ) ;
#46863=FACE_OUTER_BOUND ( 'NONE', #61003, .T. ) ;
#46864=ADVANCED_FACE ( 'NONE', ( #47575 ), #27644, .T. ) ;
#46866=CARTESIAN_POINT ( 'NONE',  ( 4.458734125000001214, -80.14583333196773651, 2.574251347313718519 ) ) ;
#46875=CARTESIAN_POINT ( 'NONE',  ( 2.071067811865476394, -164.3125000027312410, 5.000000000000000000 ) ) ;
#46877=CARTESIAN_POINT ( 'NONE',  ( 4.458734124999999437, 12.93750000136559208, -5.460374474430324690E-16 ) ) ;
#46878=CARTESIAN_POINT ( 'NONE',  ( -1.339745962155613812, -16.20534180126148271, -5.000000000000000000 ) ) ;
#46883=CARTESIAN_POINT ( 'NONE',  ( -6.972266317189433020E-16, -14.12499999726881228, -5.000000000000000000 ) ) ;
#46884=CARTESIAN_POINT ( 'NONE',  ( -2.071067811865308972, -152.3125000000000000, 5.000000000000169642 ) ) ;
#46885=CARTESIAN_POINT ( 'NONE',  ( 4.458734124999999437, -7.812499998634405252, -5.460374474430324690E-16 ) ) ;
#46888=CARTESIAN_POINT ( 'NONE',  ( 9.457646018065525792E-16, -34.31249999863440792, 5.148502694627439702 ) ) ;
#46889=AXIS2_PLACEMENT_3D ( 'NONE', #10805, #25917, #45535 ) ;
#46895=VECTOR ( 'NONE', #33951, 1000.000000000000000 ) ;
#46896=CARTESIAN_POINT ( 'NONE',  ( -4.458734124999999437, -151.1875000013656063, -5.460374474430324690E-16 ) ) ;
#46897=CARTESIAN_POINT ( 'NONE',  ( -4.458734124999999437, 13.60416666803226349, -2.574251347313719407 ) ) ;
#46898=CARTESIAN_POINT ( 'NONE',  ( 2.499999999999998668, -53.33333333333332860, -4.330127018922193649 ) ) ;
#46900=CARTESIAN_POINT ( 'NONE',  ( -2.229367062500000163, -85.72916666530107932, -3.861377020970580443 ) ) ;
#46903=CARTESIAN_POINT ( 'NONE',  ( -3.535250795749689387E-16, 16.87500000273118417, -5.773502691896257311 ) ) ;
#46905=CARTESIAN_POINT ( 'NONE',  ( 3.535533905932736864, -147.2500000027311842, 3.535533905932738641 ) ) ;
#46908=CARTESIAN_POINT ( 'NONE',  ( -5.000000000000000000, -22.00000000000000000, 0.000000000000000000 ) ) ;
#46909=CARTESIAN_POINT ( 'NONE',  ( 4.458734124999998549, -25.72916666530107221, -2.574251347313721627 ) ) ;
#46910=DIRECTION ( 'NONE',  ( -0.000000000000000000, 1.000000000000000000, -0.000000000000000000 ) ) ;
#46911=CARTESIAN_POINT ( 'NONE',  ( 2.499999999999998668, -27.20833333060214798, -4.330127018922193649 ) ) ;
#46912=CARTESIAN_POINT ( 'NONE',  ( -4.458734124999999437, -60.31249999863440081, 0.000000000000000000 ) ) ;
#46915=CARTESIAN_POINT ( 'NONE',  ( -2.229367062500000163, -10.72916666530106866, -3.861377020970580443 ) ) ;
#46916=VERTEX_POINT ( 'NONE', #13490 ) ;
#46917=CARTESIAN_POINT ( 'NONE',  ( 2.499999999999998668, -74.33333333333332860, -4.330127018922193649 ) ) ;
#46920=CARTESIAN_POINT ( 'NONE',  ( 5.000000000000000000, -77.37499999726881583, -6.123233995736766282E-16 ) ) ;
#46921=CYLINDRICAL_SURFACE ( 'NONE', #22103, 5.000000000000000000 ) ;
#46922=ORIENTED_EDGE ( 'NONE', *, *, #12734, .F. ) ;
#46924=CARTESIAN_POINT ( 'NONE',  ( 4.458734125000001214, -17.14583333196773651, 2.574251347313718519 ) ) ;
#46925=CARTESIAN_POINT ( 'NONE',  ( 4.458734125000001214, -58.14583333196773651, 2.574251347313718519 ) ) ;
#46926=CARTESIAN_POINT ( 'NONE',  ( 0.000000000000000000, -170.0000000000000000, 5.000000000000000000 ) ) ;
#46927=CARTESIAN_POINT ( 'NONE',  ( 3.152801135295367541, -140.3125000013655779, -3.152801135295367541 ) ) ;
#46930=ORIENTED_EDGE ( 'NONE', *, *, #28742, .T. ) ;
#46933=AXIS2_PLACEMENT_3D ( 'NONE', #59617, #45446, #55102 ) ;
#46936=AXIS2_PLACEMENT_3D ( 'NONE', #45603, #6691, #36278 ) ;
#46939=CARTESIAN_POINT ( 'NONE',  ( 4.458734125000000326, -146.6250000013655779, -1.846868145590734978 ) ) ;
#46944=CARTESIAN_POINT ( 'NONE',  ( -4.458734124999999437, -63.56249999863440792, 0.000000000000000000 ) ) ;
#46945=EDGE_CURVE ( 'NONE', #40725, #2367, #11901, .T. ) ;
#46948=CARTESIAN_POINT ( 'NONE',  ( -8.190561711645485556E-16, -145.6875000013656063, 4.458734124999999437 ) ) ;
#46950=ORIENTED_EDGE ( 'NONE', *, *, #32424, .T. ) ;
#46952=CARTESIAN_POINT ( 'NONE',  ( -3.535533905932737309, -144.6250000000000000, -3.535533905932738197 ) ) ;
#46955=CARTESIAN_POINT ( 'NONE',  ( 5.000000000000000000, -36.41666666666666430, -2.886751345948130876 ) ) ;
#46957=DIRECTION ( 'NONE',  ( 0.000000000000000000, 0.000000000000000000, 1.000000000000000000 ) ) ;
#46960=EDGE_CURVE ( 'NONE', #7305, #60372, #60007, .T. ) ;
#46961=CARTESIAN_POINT ( 'NONE',  ( 2.071067811865349828, -150.3125000027311842, 5.000000000000126121 ) ) ;
#46964=CARTESIAN_POINT ( 'NONE',  ( 1.975475456537005874E-15, -62.74999999999998579, 5.000000000000000000 ) ) ;
#46965=CARTESIAN_POINT ( 'NONE',  ( 4.458734125000000326, 7.104166668032259935, 2.574251347313718519 ) ) ;
#46967=CARTESIAN_POINT ( 'NONE',  ( -4.458734124999999437, -17.64583333196773651, -2.574251347313719407 ) ) ;
#46969=CARTESIAN_POINT ( 'NONE',  ( -8.190561711645485556E-16, -158.6875000013655779, 4.458734124999999437 ) ) ;
#46973=CARTESIAN_POINT ( 'NONE',  ( 4.458734124999999437, -40.81249999863440081, -5.460374474430324690E-16 ) ) ;
#46975=CARTESIAN_POINT ( 'NONE',  ( -4.458734124999997661, -65.47916666530106511, 2.574251347313722516 ) ) ;
#46982=CARTESIAN_POINT ( 'NONE',  ( -6.972266317189433020E-16, -89.12499999726880162, -5.000000000000000000 ) ) ;
#46983=CARTESIAN_POINT ( 'NONE',  ( 5.000000000000000000, -9.500000000000001776, -6.123233995736766282E-16 ) ) ;
#46984=CARTESIAN_POINT ( 'NONE',  ( -2.229367062499996610, -70.14583333196773651, 3.861377020970582219 ) ) ;
#46985=CARTESIAN_POINT ( 'NONE',  ( 1.060575238724906964E-15, -14.62499999726881228, 5.773502691896257311 ) ) ;
#46986=CARTESIAN_POINT ( 'NONE',  ( -4.458734124999998549, -46.22916666530106511, 2.574251347313722516 ) ) ;
#46988=CARTESIAN_POINT ( 'NONE',  ( 0.000000000000000000, -170.0000000000000000, 0.000000000000000000 ) ) ;
#46989=CARTESIAN_POINT ( 'NONE',  ( 4.458734125000001214, 8.854166668032261711, 2.574251347313718519 ) ) ;
#46991=( BOUNDED_CURVE ( )  B_SPLINE_CURVE ( 2, ( #47779, #13998, #19132, #52312, #58388, #13689, #37507, #23971, #23357 ),
 .UNSPECIFIED., .F., .F. ) 
 B_SPLINE_CURVE_WITH_KNOTS ( ( 3, 2, 2, 2, 3 ),
 ( 0.4437499999999999778, 0.4444444444444444198, 0.4458333333333333592, 0.4472222222222222432, 0.4479166666666666852 ),
 .UNSPECIFIED. ) 
 CURVE ( )  GEOMETRIC_REPRESENTATION_ITEM ( )  RATIONAL_B_SPLINE_CURVE ( ( 0.9330127018922194093, 0.9330127018922194093, 1.000000000000000000, 0.8660254037844387076, 1.000000000000000000, 0.8660254037844387076, 1.000000000000000000, 0.9330127018922194093, 0.9330127018922194093 ) ) 
 REPRESENTATION_ITEM ( '' )  );
#46992=CARTESIAN_POINT ( 'NONE',  ( -3.535533905932738641, -151.3750000000000000, 3.535533905932737309 ) ) ;
#46993=CARTESIAN_POINT ( 'NONE',  ( -5.000000000000000000, -53.08333333333332860, -2.886751345948128211 ) ) ;
#46994=CARTESIAN_POINT ( 'NONE',  ( -3.152801135295367985, -159.0625000013656063, 3.152801135295367096 ) ) ;
#46996=CARTESIAN_POINT ( 'NONE',  ( 3.061616997868383141E-16, -144.7500000000000284, -5.000000000000000000 ) ) ;
#46997=CARTESIAN_POINT ( 'NONE',  ( -4.458734124999998549, -82.22916666530107932, 2.574251347313722516 ) ) ;
#46998=CARTESIAN_POINT ( 'NONE',  ( -5.000000000000000888, -167.5625000000000568, -2.071067811865475949 ) ) ;
#46999=CARTESIAN_POINT ( 'NONE',  ( -3.152548672688508926E-16, -89.56249999863439371, -5.148502694627439702 ) ) ;
#47001=CARTESIAN_POINT ( 'NONE',  ( -3.152548672688508926E-16, 1.187500001365596081, -5.148502694627439702 ) ) ;
#47002=CARTESIAN_POINT ( 'NONE',  ( -3.152548672688508926E-16, -41.81249999863440081, -5.148502694627439702 ) ) ;
#47003=CARTESIAN_POINT ( 'NONE',  ( 2.499999999999998668, -72.33333333333332860, -4.330127018922193649 ) ) ;
#47005=CARTESIAN_POINT ( 'NONE',  ( 5.000000000000000000, -86.50000000000000000, -6.123233995736766282E-16 ) ) ;
#47007=CARTESIAN_POINT ( 'NONE',  ( -2.071067811865432873, -141.6875000000000284, -5.000000000000041744 ) ) ;
#47009=CARTESIAN_POINT ( 'NONE',  ( 2.229367062500001939, -72.22916666530107932, 3.861377020970579999 ) ) ;
#47013=CARTESIAN_POINT ( 'NONE',  ( 6.123233995736766282E-16, -170.0000000000000000, -5.000000000000000000 ) ) ;
#47017=CARTESIAN_POINT ( 'NONE',  ( -4.458734124999999437, 1.687500001365593194, 0.000000000000000000 ) ) ;
#47018=CARTESIAN_POINT ( 'NONE',  ( 0.000000000000000000, -170.0000000000000000, 5.000000000000000000 ) ) ;
#47019=CARTESIAN_POINT ( 'NONE',  ( -4.458734125000000326, -155.8750000013655779, 1.846868145590734089 ) ) ;
#47020=AXIS2_PLACEMENT_3D ( 'NONE', #58159, #33404, #28257 ) ;
#47022=ORIENTED_EDGE ( 'NONE', *, *, #23348, .F. ) ;
#47024=CARTESIAN_POINT ( 'NONE',  ( -1.339745962155610925, -46.79465819873852439, 5.000000000000000000 ) ) ;
#47026=CARTESIAN_POINT ( 'NONE',  ( 6.123233995736766282E-16, -170.0000000000000000, -5.000000000000000000 ) ) ;
#47029=CARTESIAN_POINT ( 'NONE',  ( -6.972266317189433020E-16, -78.24999999999998579, -5.000000000000000000 ) ) ;
#47032=CARTESIAN_POINT ( 'NONE',  ( 2.229367062499998831, 25.35416666803225993, -3.861377020970580887 ) ) ;
#47034=CARTESIAN_POINT ( 'NONE',  ( -4.458734124999999437, -5.645833331967740953, -2.574251347313719407 ) ) ;
#47035=( BOUNDED_CURVE ( )  B_SPLINE_CURVE ( 2, ( #27157, #42258, #22017, #46773, #50968, #26200, #21382, #7859, #16553 ),
 .UNSPECIFIED., .F., .F. ) 
 B_SPLINE_CURVE_WITH_KNOTS ( ( 3, 2, 2, 2, 3 ),
 ( 0.3520833333333333592, 0.3527777777777778012, 0.3541666666666666852, 0.3555555555555555691, 0.3562500000000000111 ),
 .UNSPECIFIED. ) 
 CURVE ( )  GEOMETRIC_REPRESENTATION_ITEM ( )  RATIONAL_B_SPLINE_CURVE ( ( 0.9330127018922194093, 0.9330127018922220739, 1.000000000000000000, 0.8660254037844387076, 1.000000000000000000, 0.8660254037844387076, 1.000000000000000000, 0.9330127018922194093, 0.9330127018922194093 ) ) 
 REPRESENTATION_ITEM ( '' )  );
#47038=CARTESIAN_POINT ( 'NONE',  ( 2.071067811865476394, -140.3125000027312126, 5.000000000000000000 ) ) ;
#47046=CARTESIAN_POINT ( 'NONE',  ( -8.190561711645485556E-16, -155.9375000013655779, 4.458734124999999437 ) ) ;
#47049=ORIENTED_EDGE ( 'NONE', *, *, #6767, .F. ) ;
#47050=CARTESIAN_POINT ( 'NONE',  ( -4.458734124999999437, 15.43750000136559386, 0.000000000000000000 ) ) ;
#47051=ORIENTED_EDGE ( 'NONE', *, *, #40483, .T. ) ;
#47056=CARTESIAN_POINT ( 'NONE',  ( -2.500000000000000444, 5.833333333333333037, -4.330127018922193649 ) ) ;
#47057=ADVANCED_FACE ( 'NONE', ( #48203 ), #14418, .T. ) ;
#47058=CARTESIAN_POINT ( 'NONE',  ( 4.458734125000000326, -57.89583333196773651, 2.574251347313718519 ) ) ;
#47061=FACE_OUTER_BOUND ( 'NONE', #8939, .T. ) ;
#47062=CARTESIAN_POINT ( 'NONE',  ( 1.975475456537005874E-15, -37.62499999726880873, 5.000000000000000000 ) ) ;
#47065=CARTESIAN_POINT ( 'NONE',  ( 5.000000000000000888, -41.58333333333332860, 2.886751345948126879 ) ) ;
#47066=CARTESIAN_POINT ( 'NONE',  ( -9.184850993605147944E-16, -149.2500000000000284, 5.000000000000000000 ) ) ;
#47071=CARTESIAN_POINT ( 'NONE',  ( 2.229367062499998831, -66.64583333196773651, -3.861377020970580887 ) ) ;
#47072=CARTESIAN_POINT ( 'NONE',  ( -4.458734125000001214, -147.1250000013656063, 1.846868145590734089 ) ) ;
#47073=CARTESIAN_POINT ( 'NONE',  ( 2.229367062500001939, -70.97916666530107932, 3.861377020970579999 ) ) ;
#47074=AXIS2_PLACEMENT_3D ( 'NONE', #57822, #57201, #33365 ) ;
#47076=CARTESIAN_POINT ( 'NONE',  ( -4.458734124999999437, -20.56249999863440081, 0.000000000000000000 ) ) ;
#47077=CARTESIAN_POINT ( 'NONE',  ( 2.500000000000002220, -59.54166666393546592, 4.330127018922192761 ) ) ;
#47078=VERTEX_POINT ( 'NONE', #34041 ) ;
#47080=ORIENTED_EDGE ( 'NONE', *, *, #57391, .F. ) ;
#47082=CARTESIAN_POINT ( 'NONE',  ( -6.972266317189433020E-16, -81.12499999726881583, -5.000000000000000000 ) ) ;
#47083=CARTESIAN_POINT ( 'NONE',  ( 0.000000000000000000, -170.0000000000000000, 0.000000000000000000 ) ) ;
#47084=EDGE_LOOP ( 'NONE', ( #27457, #41707, #17873, #61465 ) ) ;
#47087=CARTESIAN_POINT ( 'NONE',  ( -2.229367062499996610, -53.39583333196773651, 3.861377020970582219 ) ) ;
#47089=VECTOR ( 'NONE', #21717, 1000.000000000000000 ) ;
#47090=CARTESIAN_POINT ( 'NONE',  ( -2.498395430326213474E-14, 14.37500000273118417, 5.000000000000000000 ) ) ;
#47092=CARTESIAN_POINT ( 'NONE',  ( -4.458734124999999437, 17.60416666803225993, -2.574251347313719407 ) ) ;
#47105=CARTESIAN_POINT ( 'NONE',  ( -1.339745962155610925, 19.20534180126147916, 5.000000000000000000 ) ) ;
#47110=DIRECTION ( 'NONE',  ( -0.000000000000000000, 1.000000000000000000, -0.000000000000000000 ) ) ;
#47112=CARTESIAN_POINT ( 'NONE',  ( 3.535533905932736864, -153.2500000027312126, 3.535533905932738641 ) ) ;
#47117=( BOUNDED_CURVE ( )  B_SPLINE_CURVE ( 2, ( #36479, #40340, #56104, #12025, #15592, #2397, #22007, #59660, #54827 ),
 .UNSPECIFIED., .F., .F. ) 
 B_SPLINE_CURVE_WITH_KNOTS ( ( 3, 2, 2, 2, 3 ),
 ( 0.03541666666666666574, 0.03611111111111110772, 0.03749999999999999861, 0.03888888888888888951, 0.03958333333333333842 ),
 .UNSPECIFIED. ) 
 CURVE ( )  GEOMETRIC_REPRESENTATION_ITEM ( )  RATIONAL_B_SPLINE_CURVE ( ( 0.9330127018922194093, 0.9330127018922194093, 1.000000000000000000, 0.8660254037844387076, 1.000000000000000000, 0.8660254037844387076, 1.000000000000000000, 0.9330127018922189652, 0.9330127018922192983 ) ) 
 REPRESENTATION_ITEM ( '' )  );
#47119=CARTESIAN_POINT ( 'NONE',  ( -3.535533905932737309, -147.6250000000000000, -3.535533905932738197 ) ) ;
#47122=CARTESIAN_POINT ( 'NONE',  ( 5.000000000000000000, 22.70833333606451632, -2.886751345948130876 ) ) ;
#47123=CARTESIAN_POINT ( 'NONE',  ( 2.229367062500001939, -23.97916666530107577, 3.861377020970579999 ) ) ;
#47124=CARTESIAN_POINT ( 'NONE',  ( 1.975475456537005874E-15, -45.74999999999999289, 5.000000000000000000 ) ) ;
#47125=CARTESIAN_POINT ( 'NONE',  ( 1.339745962155615144, 18.41965820146970856, 4.999999999999999112 ) ) ;
#47127=CARTESIAN_POINT ( 'NONE',  ( 3.152801135295366208, -147.5625000013655779, 3.152801135295367985 ) ) ;
#47130=CARTESIAN_POINT ( 'NONE',  ( 2.229367062499998831, -49.89583333196772941, -3.861377020970580887 ) ) ;
#47132=CYLINDRICAL_SURFACE ( 'NONE', #14442, 5.000000000000000000 ) ;
#47133=CARTESIAN_POINT ( 'NONE',  ( 1.060575238724906964E-15, 23.25000000000000000, 5.773502691896257311 ) ) ;
#47137=CARTESIAN_POINT ( 'NONE',  ( -2.229367062499996610, -0.1458333319677394824, 3.861377020970582219 ) ) ;
#47140=CARTESIAN_POINT ( 'NONE',  ( -5.000000000000000000, -74.00000000000000000, 0.000000000000000000 ) ) ;
#47141=CARTESIAN_POINT ( 'NONE',  ( -4.458734124999998549, 11.52083333469892779, 2.574251347313722516 ) ) ;
#47142=ORIENTED_EDGE ( 'NONE', *, *, #56322, .F. ) ;
#47144=ORIENTED_EDGE ( 'NONE', *, *, #20940, .F. ) ;
#47146=CARTESIAN_POINT ( 'NONE',  ( -2.229367062499996610, -50.14583333196772941, 3.861377020970582219 ) ) ;
#47147=CARTESIAN_POINT ( 'NONE',  ( 4.458734124999999437, -159.6875000013655779, 0.000000000000000000 ) ) ;
#47149=CARTESIAN_POINT ( 'NONE',  ( -5.000000000000000000, -42.87499999726880873, 0.000000000000000000 ) ) ;
#47151=CARTESIAN_POINT ( 'NONE',  ( -4.458734124999998549, -21.22916666530107221, 2.574251347313722516 ) ) ;
#47153=ORIENTED_EDGE ( 'NONE', *, *, #24714, .T. ) ;
#47155=CARTESIAN_POINT ( 'NONE',  ( 2.730187237215162345E-16, -166.1875000013655779, -4.458734124999999437 ) ) ;
#47157=CARTESIAN_POINT ( 'NONE',  ( 1.339745962155615144, -39.58034179853028434, 4.999999999999999112 ) ) ;
#47159=VECTOR ( 'NONE', #14626, 1000.000000000000000 ) ;
#47160=CARTESIAN_POINT ( 'NONE',  ( 4.458734124999998549, -39.97916666530107221, -2.574251347313721627 ) ) ;
#47161=CARTESIAN_POINT ( 'NONE',  ( 1.975475456537005874E-15, -38.75000000000000000, 5.000000000000000000 ) ) ;
#47163=ADVANCED_FACE ( 'NONE', ( #58172 ), #33728, .T. ) ;
#47166=CARTESIAN_POINT ( 'NONE',  ( 1.975475456537005874E-15, -28.62499999726881583, 5.000000000000000000 ) ) ;
#47170=CARTESIAN_POINT ( 'NONE',  ( 9.457646018065525792E-16, -83.31249999863440792, 5.148502694627439702 ) ) ;
#47173=CARTESIAN_POINT ( 'NONE',  ( 0.000000000000000000, -170.0000000000000000, 5.000000000000000000 ) ) ;
#47178=CARTESIAN_POINT ( 'NONE',  ( 5.000000000000000888, -159.0625000027312126, -2.071067811865475505 ) ) ;
#47182=CARTESIAN_POINT ( 'NONE',  ( -2.071067811865644259, -153.8125000027311273, -4.999999999999831246 ) ) ;
#47184=CARTESIAN_POINT ( 'NONE',  ( -4.458734124999999437, -81.56249999863440792, 0.000000000000000000 ) ) ;
#47191=CARTESIAN_POINT ( 'NONE',  ( -2.071067811865478170, -167.4375000027311842, 5.000000000000000000 ) ) ;
#47193=CARTESIAN_POINT ( 'NONE',  ( 9.457646018065525792E-16, 14.68750000136559564, 5.148502694627439702 ) ) ;
#47200=CARTESIAN_POINT ( 'NONE',  ( -2.071067811865686448, -152.6875000000000284, -4.999999999999789502 ) ) ;
#47201=CARTESIAN_POINT ( 'NONE',  ( -4.458734124999999437, -9.395833331967736513, -2.574251347313719407 ) ) ;
#47204=CARTESIAN_POINT ( 'NONE',  ( -4.458734124999997661, -33.47916666530107221, 2.574251347313722516 ) ) ;
#47210=CARTESIAN_POINT ( 'NONE',  ( 4.458734125000001214, 14.10416666803225993, 2.574251347313718519 ) ) ;
#47211=EDGE_CURVE ( 'NONE', #18516, #10357, #44768, .T. ) ;
#47212=ADVANCED_FACE ( 'NONE', ( #50107 ), #20537, .T. ) ;
#47213=DIRECTION ( 'NONE',  ( 0.000000000000000000, 0.000000000000000000, 1.000000000000000000 ) ) ;
#47214=DIRECTION ( 'NONE',  ( -0.000000000000000000, 1.000000000000000000, -0.000000000000000000 ) ) ;
#47215=CARTESIAN_POINT ( 'NONE',  ( 2.229367062500001939, -86.22916666530107932, 3.861377020970579999 ) ) ;
#47218=CARTESIAN_POINT ( 'NONE',  ( -5.000000000000000000, 20.04166666939785202, -2.886751345948128211 ) ) ;
#47223=CARTESIAN_POINT ( 'NONE',  ( 1.060575238724906964E-15, -26.74999999999999645, 5.773502691896257311 ) ) ;
#47224=CARTESIAN_POINT ( 'NONE',  ( 2.229367062499998831, -32.64583333196773651, -3.861377020970580887 ) ) ;
#47227=CARTESIAN_POINT ( 'NONE',  ( 5.000000000000000888, -29.45833333060214798, 2.886751345948126879 ) ) ;
#47228=CARTESIAN_POINT ( 'NONE',  ( -2.229367062499996610, -60.14583333196774362, 3.861377020970582219 ) ) ;
#47231=ADVANCED_FACE ( 'NONE', ( #30810 ), #60416, .T. ) ;
#47232=CARTESIAN_POINT ( 'NONE',  ( -2.229367062499996610, -8.395833331967736513, 3.861377020970582219 ) ) ;
#47234=CARTESIAN_POINT ( 'NONE',  ( -2.499999999999996447, -77.83333333333334281, 4.330127018922195425 ) ) ;
#47237=CARTESIAN_POINT ( 'NONE',  ( -3.535250795749689387E-16, -79.12499999726881583, -5.773502691896257311 ) ) ;
#47238=CARTESIAN_POINT ( 'NONE',  ( 1.339745962155615144, -65.58034179853029855, 4.999999999999999112 ) ) ;
#47239=ORIENTED_EDGE ( 'NONE', *, *, #57391, .T. ) ;
#47241=CARTESIAN_POINT ( 'NONE',  ( -3.152548672688508926E-16, -19.81249999863440436, -5.148502694627439702 ) ) ;
#47242=CARTESIAN_POINT ( 'NONE',  ( -4.458734124999998549, -54.47916666530107932, 2.574251347313722516 ) ) ;
#47243=CARTESIAN_POINT ( 'NONE',  ( -2.500000000000000444, -30.04166666393548013, -4.330127018922193649 ) ) ;
#47244=SURFACE_SIDE_STYLE ('',( #51441 ) ) ;
#47245=CARTESIAN_POINT ( 'NONE',  ( -4.458734125000001214, -141.8750000013656063, 1.846868145590734089 ) ) ;
#47247=DIRECTION ( 'NONE',  ( -0.000000000000000000, 1.000000000000000000, -0.000000000000000000 ) ) ;
#47255=CARTESIAN_POINT ( 'NONE',  ( 3.152801135295366208, -149.8125000013655779, 3.152801135295367985 ) ) ;
#47259=CARTESIAN_POINT ( 'NONE',  ( 9.457646018065525792E-16, -65.31249999863440792, 5.148502694627439702 ) ) ;
#47260=PLANE ( 'NONE',  #16861 ) ;
#47261=CARTESIAN_POINT ( 'NONE',  ( -5.000000000000000000, -42.87499999726880873, 0.000000000000000000 ) ) ;
#47262=CARTESIAN_POINT ( 'NONE',  ( -4.458734124999999437, -145.9375000013656063, -5.460374474430324690E-16 ) ) ;
#47270=CARTESIAN_POINT ( 'NONE',  ( 4.458734125000000326, 27.85416666803225993, 2.574251347313718519 ) ) ;
#47271=CARTESIAN_POINT ( 'NONE',  ( -6.972266317189433020E-16, -18.12499999726881228, -5.000000000000000000 ) ) ;
#47274=DIRECTION ( 'NONE',  ( -0.000000000000000000, 1.000000000000000000, -0.000000000000000000 ) ) ;
#47275=CARTESIAN_POINT ( 'NONE',  ( 5.000000000000000000, 21.50000000000000000, -6.123233995736766282E-16 ) ) ;
#47276=CARTESIAN_POINT ( 'NONE',  ( -3.152548672688508926E-16, 7.437500001365594748, -5.148502694627439702 ) ) ;
#47278=CARTESIAN_POINT ( 'NONE',  ( -4.458734124999999437, -18.56249999863440792, 0.000000000000000000 ) ) ;
#47280=CARTESIAN_POINT ( 'NONE',  ( 4.458734124999999437, -160.4375000013655779, 0.000000000000000000 ) ) ;
#47281=CYLINDRICAL_SURFACE ( 'NONE', #12024, 5.000000000000000000 ) ;
#47284=CARTESIAN_POINT ( 'NONE',  ( 0.000000000000000000, -170.0000000000000000, 5.000000000000000000 ) ) ;
#47285=CARTESIAN_POINT ( 'NONE',  ( 4.458734124999999437, -38.81249999863440081, -5.460374474430324690E-16 ) ) ;
#47288=CARTESIAN_POINT ( 'NONE',  ( 4.458734124999999437, -65.06249999863440792, -5.460374474430324690E-16 ) ) ;
#47290=LINE ( 'NONE', #27037, #24372 ) ;
#47291=CARTESIAN_POINT ( 'NONE',  ( -9.184850993605147944E-16, -152.3750000027311842, 5.000000000000000000 ) ) ;
#47293=CARTESIAN_POINT ( 'NONE',  ( -4.999999999999998224, -84.91666666666667140, 2.886751345948131764 ) ) ;
#47294=CARTESIAN_POINT ( 'NONE',  ( 0.000000000000000000, -170.0000000000000000, 0.000000000000000000 ) ) ;
#47295=CARTESIAN_POINT ( 'NONE',  ( 2.499999999999998668, -12.33333333333333570, -4.330127018922193649 ) ) ;
#47296=CARTESIAN_POINT ( 'NONE',  ( -2.229367062500000163, -18.47916666530106866, -3.861377020970580443 ) ) ;
#47297=CARTESIAN_POINT ( 'NONE',  ( -4.458734124999997661, -76.22916666530107932, 2.574251347313722516 ) ) ;
#47298=CARTESIAN_POINT ( 'NONE',  ( 5.000000000000000000, -12.29166666393547835, -2.886751345948129988 ) ) ;
#47299=CARTESIAN_POINT ( 'NONE',  ( -4.458734124999999437, -43.39583333196774362, -2.574251347313719407 ) ) ;
#47300=VERTEX_POINT ( 'NONE', #45284 ) ;
#47301=CARTESIAN_POINT ( 'NONE',  ( 1.339745962155612702, -41.29465819873852439, -5.000000000000000000 ) ) ;
#47302=CARTESIAN_POINT ( 'NONE',  ( 2.229367062500001939, 5.770833334698927786, 3.861377020970579999 ) ) ;
#47305=CARTESIAN_POINT ( 'NONE',  ( 2.499999999999998668, -55.33333333333332860, -4.330127018922193649 ) ) ;
#47307=CARTESIAN_POINT ( 'NONE',  ( -1.846868145590734756, -158.3750000013655779, -4.458734125000000326 ) ) ;
#47309=CARTESIAN_POINT ( 'NONE',  ( -9.184850993605147944E-16, -145.2500000000000284, 5.000000000000000000 ) ) ;
#47310=CARTESIAN_POINT ( 'NONE',  ( 2.229367062499998831, -81.64583333196773651, -3.861377020970580887 ) ) ;
#47311=CARTESIAN_POINT ( 'NONE',  ( -3.535533905932737309, -165.6250000000000284, -3.535533905932738197 ) ) ;
#47312=EDGE_CURVE ( 'NONE', #57843, #50566, #11406, .T. ) ;
#47315=CARTESIAN_POINT ( 'NONE',  ( 2.229367062500001939, 0.7708333346989268975, 3.861377020970579999 ) ) ;
#47316=CARTESIAN_POINT ( 'NONE',  ( 4.458734125000001214, -41.14583333196774362, 2.574251347313718519 ) ) ;
#47318=EDGE_CURVE ( 'NONE', #33853, #15348, #11813, .T. ) ;
#47321=CARTESIAN_POINT ( 'NONE',  ( 1.339745962155615144, -86.70534180126148271, 4.999999999999999112 ) ) ;
#47322=ORIENTED_EDGE ( 'NONE', *, *, #16497, .F. ) ;
#47323=CARTESIAN_POINT ( 'NONE',  ( -2.071067811865306307, -148.8125000027312126, -5.000000000000171418 ) ) ;
#47325=CARTESIAN_POINT ( 'NONE',  ( -4.458734124999999437, -70.56249999863439371, 0.000000000000000000 ) ) ;
#47332=CARTESIAN_POINT ( 'NONE',  ( 2.229367062499998831, 3.354166668032259935, -3.861377020970580887 ) ) ;
#47334=CARTESIAN_POINT ( 'NONE',  ( -1.846868145590737420, -157.7500000013656063, 4.458734124999997661 ) ) ;
#47336=ORIENTED_EDGE ( 'NONE', *, *, #42129, .F. ) ;
#47340=AXIS2_PLACEMENT_3D ( 'NONE', #60441, #15724, #54645 ) ;
#47347=CARTESIAN_POINT ( 'NONE',  ( -4.458734124999999437, 20.68750000136559208, 0.000000000000000000 ) ) ;
#47349=CARTESIAN_POINT ( 'NONE',  ( -4.458734124999999437, -3.645833331967739177, -2.574251347313719407 ) ) ;
#47352=CARTESIAN_POINT ( 'NONE',  ( 2.071067811865475505, -141.9375000027312126, -5.000000000000000888 ) ) ;
#47353=CARTESIAN_POINT ( 'NONE',  ( -1.339745962155610925, -51.79465819873851729, 5.000000000000000000 ) ) ;
#47357=FACE_OUTER_BOUND ( 'NONE', #44202, .T. ) ;
#47361=CARTESIAN_POINT ( 'NONE',  ( 3.152801135295367541, -158.5625000013656063, -3.152801135295367541 ) ) ;
#47362=( BOUNDED_CURVE ( )  B_SPLINE_CURVE ( 2, ( #49958, #10725, #6862, #60269, #50920, #16187, #54797, #50600, #30332 ),
 .UNSPECIFIED., .F., .F. ) 
 B_SPLINE_CURVE_WITH_KNOTS ( ( 3, 2, 2, 2, 3 ),
 ( 0.3083333333333336257, 0.3125000000000002776, 0.3166666666666669294, 0.3208333333333336368, 0.3250000000000002887 ),
 .UNSPECIFIED. ) 
 CURVE ( )  GEOMETRIC_REPRESENTATION_ITEM ( )  RATIONAL_B_SPLINE_CURVE ( ( 0.9999999999999948930, 0.9238795325112918455, 1.000000000000000000, 0.9238795325112867385, 1.000000000000000000, 0.9238795325112867385, 1.000000000000000000, 0.9238795325112816315, 1.000000000000005107 ) ) 
 REPRESENTATION_ITEM ( '' )  );
#47364=CARTESIAN_POINT ( 'NONE',  ( -2.071067811865391128, -147.6875000000000568, -5.000000000000086153 ) ) ;
#47365=ORIENTED_EDGE ( 'NONE', *, *, #29384, .F. ) ;
#47366=CARTESIAN_POINT ( 'NONE',  ( 2.229367062499998831, 15.10416666803225993, -3.861377020970580887 ) ) ;
#47372=CARTESIAN_POINT ( 'NONE',  ( 2.499999999999998668, 8.666666666666666075, -4.330127018922193649 ) ) ;
#47373=CARTESIAN_POINT ( 'NONE',  ( 4.458734125000000326, -58.89583333196773651, 2.574251347313718519 ) ) ;
#47374=CARTESIAN_POINT ( 'NONE',  ( 0.000000000000000000, -170.0000000000000000, 0.000000000000000000 ) ) ;
#47376=CARTESIAN_POINT ( 'NONE',  ( -2.229367062499996610, -31.14583333196773651, 3.861377020970582219 ) ) ;
#47379=CARTESIAN_POINT ( 'NONE',  ( -2.500000000000000444, -42.16666666666667140, -4.330127018922193649 ) ) ;
#47380=CARTESIAN_POINT ( 'NONE',  ( -4.999999999999998224, 13.20833333606451987, 2.886751345948131764 ) ) ;
#47381=CARTESIAN_POINT ( 'NONE',  ( -1.339745962155613812, -48.20534180126148271, -5.000000000000000000 ) ) ;
#47384=CARTESIAN_POINT ( 'NONE',  ( -4.458734124999999437, -62.39583333196774362, -2.574251347313719407 ) ) ;
#47385=CARTESIAN_POINT ( 'NONE',  ( 4.458734124999999437, -147.6875000013656063, 0.000000000000000000 ) ) ;
#47386=CARTESIAN_POINT ( 'NONE',  ( 4.458734124999999437, -68.81249999863439371, -5.460374474430324690E-16 ) ) ;
#47388=CARTESIAN_POINT ( 'NONE',  ( 4.458734124999999437, -26.06249999863440792, -5.460374474430324690E-16 ) ) ;
#47389=CARTESIAN_POINT ( 'NONE',  ( -5.000000000000000000, -63.87499999726880873, 0.000000000000000000 ) ) ;
#47391=CARTESIAN_POINT ( 'NONE',  ( 5.000000000000000888, -1.583333333333332371, 2.886751345948126879 ) ) ;
#47392=ORIENTED_EDGE ( 'NONE', *, *, #39262, .F. ) ;
#47395=ORIENTED_EDGE ( 'NONE', *, *, #43342, .T. ) ;
#47397=CARTESIAN_POINT ( 'NONE',  ( 1.975475456537005874E-15, -74.62499999726880162, 5.000000000000000000 ) ) ;
#47398=CARTESIAN_POINT ( 'NONE',  ( 2.229367062500001939, -54.22916666530107221, 3.861377020970579999 ) ) ;
#47399=ORIENTED_EDGE ( 'NONE', *, *, #893, .F. ) ;
#47402=CARTESIAN_POINT ( 'NONE',  ( -4.458734124999999437, 19.68750000136559208, 0.000000000000000000 ) ) ;
#47405=CARTESIAN_POINT ( 'NONE',  ( 1.846868145590735200, -168.2500000013656063, -4.458734124999999437 ) ) ;
#47409=DIRECTION ( 'NONE',  ( -0.000000000000000000, 1.000000000000000000, -0.000000000000000000 ) ) ;
#47411=CARTESIAN_POINT ( 'NONE',  ( 3.535533905932738197, -140.0000000027311842, -3.535533905932738197 ) ) ;
#47421=CARTESIAN_POINT ( 'NONE',  ( 5.000000000000000000, 11.50000000000000000, -6.123233995736766282E-16 ) ) ;
#47423=CARTESIAN_POINT ( 'NONE',  ( -2.071067811865478170, -153.4375000027312410, 5.000000000000000000 ) ) ;
#47430=CARTESIAN_POINT ( 'NONE',  ( 5.000000000000000888, -145.9375000000000000, -2.071067811865475505 ) ) ;
#47433=CARTESIAN_POINT ( 'NONE',  ( 3.152801135295367541, -168.5625000013656063, -3.152801135295367541 ) ) ;
#47434=CARTESIAN_POINT ( 'NONE',  ( 4.458734125000000326, -25.89583333196773651, 2.574251347313718519 ) ) ;
#47435=CARTESIAN_POINT ( 'NONE',  ( 3.061616997868383141E-16, -146.7500000000000284, -5.000000000000000000 ) ) ;
#47438=CARTESIAN_POINT ( 'NONE',  ( 3.152801135295366208, -146.5625000013655779, 3.152801135295367985 ) ) ;
#47440=DIRECTION ( 'NONE',  ( -0.000000000000000000, 1.000000000000000000, -0.000000000000000000 ) ) ;
#47441=CARTESIAN_POINT ( 'NONE',  ( 4.458734124999999437, -57.06249999863440081, -5.460374474430324690E-16 ) ) ;
#47445=CARTESIAN_POINT ( 'NONE',  ( -2.500000000000000444, 21.83333333333333215, -4.330127018922193649 ) ) ;
#47446=CARTESIAN_POINT ( 'NONE',  ( -3.152548672688508926E-16, -3.562499998634408360, -5.148502694627439702 ) ) ;
#47447=CARTESIAN_POINT ( 'NONE',  ( -1.339745962155610925, -10.79465819873852261, 5.000000000000000000 ) ) ;
#47448=CARTESIAN_POINT ( 'NONE',  ( -3.535533905932737309, -164.6250000000000284, -3.535533905932738197 ) ) ;
#47449=CARTESIAN_POINT ( 'NONE',  ( 2.229367062500001939, 11.77083333469892601, 3.861377020970579999 ) ) ;
#47450=ORIENTED_EDGE ( 'NONE', *, *, #61024, .F. ) ;
#47453=CARTESIAN_POINT ( 'NONE',  ( -1.339745962155613812, -24.08034179853029499, -5.000000000000000000 ) ) ;
#47454=CARTESIAN_POINT ( 'NONE',  ( 2.229367062499998831, -50.64583333196772941, -3.861377020970580887 ) ) ;
#47455=CARTESIAN_POINT ( 'NONE',  ( 3.152801135295366208, -160.8125000013656063, 3.152801135295367985 ) ) ;
#47456=CARTESIAN_POINT ( 'NONE',  ( 1.060575238724906964E-15, -45.62499999726880873, 5.773502691896257311 ) ) ;
#47458=CARTESIAN_POINT ( 'NONE',  ( 4.458734124999998549, -25.72916666530107221, -2.574251347313721627 ) ) ;
#47461=CARTESIAN_POINT ( 'NONE',  ( -4.458734124999999437, -161.9375000013655779, -5.460374474430324690E-16 ) ) ;
#47464=CARTESIAN_POINT ( 'NONE',  ( -2.229367062499996610, -40.39583333196773651, 3.861377020970582219 ) ) ;
#47465=VERTEX_POINT ( 'NONE', #16653 ) ;
#47468=DIRECTION ( 'NONE',  ( -0.000000000000000000, 1.000000000000000000, -0.000000000000000000 ) ) ;
#47469=VERTEX_POINT ( 'NONE', #599 ) ;
#47472=CARTESIAN_POINT ( 'NONE',  ( -4.458734124999999437, -84.56249999863439371, 0.000000000000000000 ) ) ;
#47475=CARTESIAN_POINT ( 'NONE',  ( -3.152801135295367985, -140.0625000013655779, 3.152801135295367096 ) ) ;
#47476=CARTESIAN_POINT ( 'NONE',  ( 3.535533905932736864, -145.2500000027311842, 3.535533905932738641 ) ) ;
#47479=ADVANCED_FACE ( 'NONE', ( #59453 ), #15384, .T. ) ;
#47481=CYLINDRICAL_SURFACE ( 'NONE', #55335, 5.000000000000000000 ) ;
#47485=CARTESIAN_POINT ( 'NONE',  ( -5.000000000000000000, -73.08333333333332860, -2.886751345948128211 ) ) ;
#47487=CARTESIAN_POINT ( 'NONE',  ( -4.458734124999999437, -86.64583333196773651, -2.574251347313719407 ) ) ;
#47490=VERTEX_POINT ( 'NONE', #44969 ) ;
#47491=CARTESIAN_POINT ( 'NONE',  ( 5.000000000000000888, -47.58333333333333570, 2.886751345948126879 ) ) ;
#47493=CARTESIAN_POINT ( 'NONE',  ( -2.071067811865478170, -164.4375000027311842, 5.000000000000000000 ) ) ;
#47495=CARTESIAN_POINT ( 'NONE',  ( -2.229367062500000163, 9.270833334698927786, -3.861377020970580443 ) ) ;
#47498=( BOUNDED_CURVE ( )  B_SPLINE_CURVE ( 2, ( #58595, #28367, #47988, #48613, #14514, #3942, #62799, #35420, #31222 ),
 .UNSPECIFIED., .F., .F. ) 
 B_SPLINE_CURVE_WITH_KNOTS ( ( 3, 2, 2, 2, 3 ),
 ( 0.1437499999999999889, 0.1444444444444444309, 0.1458333333333333426, 0.1472222222222222265, 0.1479166666666666685 ),
 .UNSPECIFIED. ) 
 CURVE ( )  GEOMETRIC_REPRESENTATION_ITEM ( )  RATIONAL_B_SPLINE_CURVE ( ( 0.9330127018922194093, 0.9330127018922194093, 1.000000000000000000, 0.8660254037844387076, 1.000000000000000000, 0.8660254037844387076, 1.000000000000000000, 0.9330127018922194093, 0.9330127018922194093 ) ) 
 REPRESENTATION_ITEM ( '' )  );
#47506=CARTESIAN_POINT ( 'NONE',  ( -4.458734124999997661, -10.22916666530106866, 2.574251347313722516 ) ) ;
#47508=ORIENTED_EDGE ( 'NONE', *, *, #5090, .T. ) ;
#47509=CARTESIAN_POINT ( 'NONE',  ( -4.458734124999999437, -37.56249999863440792, 0.000000000000000000 ) ) ;
#47512=CARTESIAN_POINT ( 'NONE',  ( -5.000000000000000000, -28.08333333333333925, -2.886751345948128211 ) ) ;
#47516=CARTESIAN_POINT ( 'NONE',  ( -2.229367062499996610, 15.85416666803226171, 3.861377020970582219 ) ) ;
#47519=CARTESIAN_POINT ( 'NONE',  ( 4.458734124999999437, -84.06249999863439371, -5.460374474430324690E-16 ) ) ;
#47521=CARTESIAN_POINT ( 'NONE',  ( -5.000000000000000000, 18.12500000273118417, 0.000000000000000000 ) ) ;
#47525=CARTESIAN_POINT ( 'NONE',  ( 5.000000000000000000, -52.41666666666666430, -2.886751345948130876 ) ) ;
#47526=CARTESIAN_POINT ( 'NONE',  ( -3.535250795749689387E-16, -31.25000000000000000, -5.773502691896257311 ) ) ;
#47527=CARTESIAN_POINT ( 'NONE',  ( -2.229367062500000163, -35.47916666530107221, -3.861377020970580443 ) ) ;
#47529=CARTESIAN_POINT ( 'NONE',  ( 1.060575238724906964E-15, -30.62499999726881228, 5.773502691896257311 ) ) ;
#47531=CARTESIAN_POINT ( 'NONE',  ( -2.229367062500000163, -58.47916666530106511, -3.861377020970580443 ) ) ;
#47533=DIRECTION ( 'NONE',  ( -0.000000000000000000, 1.000000000000000000, -0.000000000000000000 ) ) ;
#47534=CARTESIAN_POINT ( 'NONE',  ( -4.458734124999998549, -7.479166665301073991, 2.574251347313722516 ) ) ;
#47535=ORIENTED_EDGE ( 'NONE', *, *, #15415, .T. ) ;
#47536=CARTESIAN_POINT ( 'NONE',  ( -5.000000000000000000, -78.08333333333332860, -2.886751345948128211 ) ) ;
#47539=CARTESIAN_POINT ( 'NONE',  ( -5.000000000000000000, -77.87499999726881583, 0.000000000000000000 ) ) ;
#47541=VERTEX_POINT ( 'NONE', #56218 ) ;
#47543=CARTESIAN_POINT ( 'NONE',  ( -4.458734124999998549, -20.47916666530107577, 2.574251347313722516 ) ) ;
#47544=CARTESIAN_POINT ( 'NONE',  ( 2.229367062500001939, -57.22916666530107932, 3.861377020970579999 ) ) ;
#47547=CARTESIAN_POINT ( 'NONE',  ( 4.458734125000000326, -140.3750000013656063, -1.846868145590734978 ) ) ;
#47549=CARTESIAN_POINT ( 'NONE',  ( -5.000000000000000000, 18.00000000000000000, 0.000000000000000000 ) ) ;
#47550=ORIENTED_EDGE ( 'NONE', *, *, #63552, .T. ) ;
#47553=( BOUNDED_CURVE ( )  B_SPLINE_CURVE ( 2, ( #28916, #19583, #48539, #58194, #58822, #49494, #29538, #19263, #63039 ),
 .UNSPECIFIED., .F., .F. ) 
 B_SPLINE_CURVE_WITH_KNOTS ( ( 3, 2, 2, 2, 3 ),
 ( 0.9749999999999998668, 0.9791666666666665186, 0.9833333333333331705, 0.9874999999999999334, 0.9916666666666665853 ),
 .UNSPECIFIED. ) 
 CURVE ( )  GEOMETRIC_REPRESENTATION_ITEM ( )  RATIONAL_B_SPLINE_CURVE ( ( 1.000000000000001998, 0.9238795325112847401, 1.000000000000000000, 0.9238795325112867385, 1.000000000000000000, 0.9238795325112867385, 1.000000000000000000, 0.9238795325112887369, 0.9999999999999980016 ) ) 
 REPRESENTATION_ITEM ( '' )  );
#47558=ADVANCED_FACE ( 'NONE', ( #2202 ), #27877, .T. ) ;
#47559=CARTESIAN_POINT ( 'NONE',  ( -4.458734125000001214, -144.1250000013655779, 1.846868145590734089 ) ) ;
#47563=CARTESIAN_POINT ( 'NONE',  ( -3.152548672688508926E-16, -66.81249999863442213, -5.148502694627439702 ) ) ;
#47565=CARTESIAN_POINT ( 'NONE',  ( -1.846868145590737420, -139.7500000013655779, 4.458734124999997661 ) ) ;
#47568=CARTESIAN_POINT ( 'NONE',  ( -4.999999999999998224, -49.79166666393547303, 2.886751345948131764 ) ) ;
#47574=CARTESIAN_POINT ( 'NONE',  ( -4.458734124999997661, 26.52083333469892779, 2.574251347313722516 ) ) ;
#47575=FACE_OUTER_BOUND ( 'NONE', #18595, .T. ) ;
#47581=CARTESIAN_POINT ( 'NONE',  ( 2.500000000000002220, -43.54166666393548013, 4.330127018922192761 ) ) ;
#47582=CARTESIAN_POINT ( 'NONE',  ( 9.457646018065525792E-16, 7.937500001365596525, 5.148502694627439702 ) ) ;
#47584=CARTESIAN_POINT ( 'NONE',  ( -3.152548672688508926E-16, -20.81249999863440081, -5.148502694627439702 ) ) ;
#47586=CARTESIAN_POINT ( 'NONE',  ( -4.458734125000001214, -157.8750000013656063, 1.846868145590734089 ) ) ;
#47587=CARTESIAN_POINT ( 'NONE',  ( -5.000000000000000888, -158.4375000000000568, 2.071067811865474617 ) ) ;
#47590=CARTESIAN_POINT ( 'NONE',  ( 5.000000000000000000, 15.50000000000000000, -6.123233995736766282E-16 ) ) ;
#47591=CARTESIAN_POINT ( 'NONE',  ( -3.152548672688508926E-16, -39.56249999863440081, -5.148502694627439702 ) ) ;
#47592=CARTESIAN_POINT ( 'NONE',  ( -2.500000000000000444, -84.16666666666667140, -4.330127018922193649 ) ) ;
#47594=CARTESIAN_POINT ( 'NONE',  ( 4.458734124999999437, -66.06249999863440792, -5.460374474430324690E-16 ) ) ;
#47598=CARTESIAN_POINT ( 'NONE',  ( -5.000000000000000000, 15.04166666939785202, -2.886751345948128211 ) ) ;
#47599=CARTESIAN_POINT ( 'NONE',  ( 1.975475456537005874E-15, 12.37500000273118417, 5.000000000000000000 ) ) ;
#47600=CARTESIAN_POINT ( 'NONE',  ( -4.999999999999999112, -12.91666666666666785, 2.886751345948131764 ) ) ;
#47601=CARTESIAN_POINT ( 'NONE',  ( 4.458734125000001214, -16.89583333196773651, 2.574251347313718519 ) ) ;
#47602=CARTESIAN_POINT ( 'NONE',  ( 4.458734124999998549, -76.72916666530106511, -2.574251347313721627 ) ) ;
#47604=CARTESIAN_POINT ( 'NONE',  ( -2.500000000000000444, -11.04166666393547835, -4.330127018922193649 ) ) ;
#47605=CARTESIAN_POINT ( 'NONE',  ( 4.458734124999999437, -44.81249999863440081, -5.460374474430324690E-16 ) ) ;
#47606=ORIENTED_EDGE ( 'NONE', *, *, #44521, .F. ) ;
#47607=CARTESIAN_POINT ( 'NONE',  ( 5.000000000000000000, -41.41666666666667140, -2.886751345948130876 ) ) ;
#47608=CARTESIAN_POINT ( 'NONE',  ( 2.229367062499998831, 5.104166668032261711, -3.861377020970580887 ) ) ;
#47610=CARTESIAN_POINT ( 'NONE',  ( 1.975475456537005874E-15, -81.62499999726881583, 5.000000000000000000 ) ) ;
#47611=CARTESIAN_POINT ( 'NONE',  ( 2.500000000000002220, -59.66666666666665719, 4.330127018922192761 ) ) ;
#47612=CARTESIAN_POINT ( 'NONE',  ( 2.730187237215162345E-16, -161.4375000013655779, -4.458734124999999437 ) ) ;
#47615=CARTESIAN_POINT ( 'NONE',  ( 5.000000000000000888, -14.58333333333333215, 2.886751345948126879 ) ) ;
#47616=CARTESIAN_POINT ( 'NONE',  ( 2.071067811865475505, -167.8125000000000284, -5.000000000000000888 ) ) ;
#47617=CARTESIAN_POINT ( 'NONE',  ( -6.972266317189433020E-16, -11.25000000000000178, -5.000000000000000000 ) ) ;
#47619=CARTESIAN_POINT ( 'NONE',  ( -2.229367062499996610, -6.395833331967741842, 3.861377020970582219 ) ) ;
#47620=CARTESIAN_POINT ( 'NONE',  ( 4.458734124999998549, -40.97916666530107932, -2.574251347313721627 ) ) ;
#47623=CARTESIAN_POINT ( 'NONE',  ( -6.972266317189433020E-16, -84.24999999999998579, -5.000000000000000000 ) ) ;
#47624=ORIENTED_EDGE ( 'NONE', *, *, #42564, .F. ) ;
#47627=CARTESIAN_POINT ( 'NONE',  ( 9.457646018065525792E-16, -67.31249999863440792, 5.148502694627439702 ) ) ;
#47628=CARTESIAN_POINT ( 'NONE',  ( -1.846868145590737420, -147.0000000013656063, 4.458734124999997661 ) ) ;
#47629=EDGE_LOOP ( 'NONE', ( #55502, #54758, #42813, #6546 ) ) ;
#47630=EDGE_CURVE ( 'NONE', #1769, #21623, #37227, .T. ) ;
#47632=CARTESIAN_POINT ( 'NONE',  ( 5.000000000000000000, -3.291666663935478354, -2.886751345948130876 ) ) ;
#47634=ADVANCED_FACE ( 'NONE', ( #32393 ), #27251, .T. ) ;
#47636=CARTESIAN_POINT ( 'NONE',  ( -4.458734124999998549, 2.770833334698928674, 2.574251347313722516 ) ) ;
#47638=CARTESIAN_POINT ( 'NONE',  ( 1.846868145590736310, -154.6250000013655779, 4.458734124999997661 ) ) ;
#47647=EDGE_CURVE ( 'NONE', #56674, #5292, #7416, .T. ) ;
#47652=CARTESIAN_POINT ( 'NONE',  ( -3.152548672688508926E-16, 24.43750000136559564, -5.148502694627439702 ) ) ;
#47653=EDGE_CURVE ( 'NONE', #36379, #11571, #20559, .T. ) ;
#47655=CARTESIAN_POINT ( 'NONE',  ( 4.458734124999999437, -4.062499998634408804, -5.460374474430324690E-16 ) ) ;
#47656=CARTESIAN_POINT ( 'NONE',  ( 1.975475456537005874E-15, -63.74999999999998579, 5.000000000000000000 ) ) ;
#47659=CARTESIAN_POINT ( 'NONE',  ( -2.071067811865475061, -139.8125000027312126, -5.000000000000000888 ) ) ;
#47660=CARTESIAN_POINT ( 'NONE',  ( -2.500000000000000444, -52.16666666666666430, -4.330127018922193649 ) ) ;
#47668=CARTESIAN_POINT ( 'NONE',  ( 4.458734124999997661, -156.7500000013656063, 1.846868145590737864 ) ) ;
#47672=CARTESIAN_POINT ( 'NONE',  ( 4.458734124999999437, 15.93750000136559564, -5.460374474430324690E-16 ) ) ;
#47677=DIRECTION ( 'NONE',  ( -0.000000000000000000, 1.000000000000000000, -0.000000000000000000 ) ) ;
#47678=CARTESIAN_POINT ( 'NONE',  ( 5.000000000000000888, 1.416666666666666741, 2.886751345948126879 ) ) ;
#47679=CARTESIAN_POINT ( 'NONE',  ( -4.458734124999999437, -63.39583333196772941, -2.574251347313719407 ) ) ;
#47682=CARTESIAN_POINT ( 'NONE',  ( -2.229367062499996610, -29.14583333196774007, 3.861377020970582219 ) ) ;
#47683=DIRECTION ( 'NONE',  ( -0.000000000000000000, 1.000000000000000000, -0.000000000000000000 ) ) ;
#47684=FACE_OUTER_BOUND ( 'NONE', #51036, .T. ) ;
#47686=CARTESIAN_POINT ( 'NONE',  ( 5.000000000000000000, -47.41666666666666430, -2.886751345948129988 ) ) ;
#47687=LINE ( 'NONE', #32904, #24328 ) ;
#47688=CARTESIAN_POINT ( 'NONE',  ( 5.000000000000000000, -26.29166666393547658, -2.886751345948130876 ) ) ;
#47691=CARTESIAN_POINT ( 'NONE',  ( 2.229367062499998831, -63.64583333196772941, -3.861377020970580887 ) ) ;
#47692=CARTESIAN_POINT ( 'NONE',  ( 1.846868145590735200, -148.5000000013656347, -4.458734125000000326 ) ) ;
#47693=CARTESIAN_POINT ( 'NONE',  ( 4.458734124999998549, -74.72916666530106511, -2.574251347313721627 ) ) ;
#47695=CARTESIAN_POINT ( 'NONE',  ( 4.458734124999999437, -27.06249999863440081, -5.460374474430324690E-16 ) ) ;
#47696=CARTESIAN_POINT ( 'NONE',  ( -5.000000000000000000, -68.87499999726880162, 0.000000000000000000 ) ) ;
#47698=CARTESIAN_POINT ( 'NONE',  ( 2.499999999999998668, -1.333333333333332149, -4.330127018922193649 ) ) ;
#47701=CARTESIAN_POINT ( 'NONE',  ( 1.339745962155615144, -21.58034179853029855, 4.999999999999999112 ) ) ;
#47703=VERTEX_POINT ( 'NONE', #14023 ) ;
#47704=CARTESIAN_POINT ( 'NONE',  ( 0.000000000000000000, -170.0000000000000000, 0.000000000000000000 ) ) ;
#47705=CARTESIAN_POINT ( 'NONE',  ( -4.458734124999999437, -55.56249999863440081, 0.000000000000000000 ) ) ;
#47707=ORIENTED_EDGE ( 'NONE', *, *, #42491, .T. ) ;
#47711=CARTESIAN_POINT ( 'NONE',  ( -4.458734124999998549, 20.77083333469892779, 2.574251347313722516 ) ) ;
#47713=CARTESIAN_POINT ( 'NONE',  ( 1.339745962155624914, 20.83034180399265978, -4.999999999999991118 ) ) ;
#47714=CARTESIAN_POINT ( 'NONE',  ( -3.152801135295367096, -168.0625000013656063, -3.152801135295367541 ) ) ;
#47715=VERTEX_POINT ( 'NONE', #62932 ) ;
#47725=CARTESIAN_POINT ( 'NONE',  ( -5.000000000000000888, -156.5625000000000284, -2.071067811865475949 ) ) ;
#47732=CARTESIAN_POINT ( 'NONE',  ( -2.071067811865478170, -155.4375000027312694, 5.000000000000000000 ) ) ;
#47738=CARTESIAN_POINT ( 'NONE',  ( 3.535533905932738197, -147.8750000000000000, -3.535533905932738197 ) ) ;
#47742=CARTESIAN_POINT ( 'NONE',  ( 4.458734124999997661, -167.7500000013655779, 1.846868145590737864 ) ) ;
#47743=CARTESIAN_POINT ( 'NONE',  ( 4.458734124999999437, -27.81249999863440081, -5.460374474430324690E-16 ) ) ;
#47745=LINE ( 'NONE', #62564, #38960 ) ;
#47747=CARTESIAN_POINT ( 'NONE',  ( 3.152801135295367541, -149.3125000013655779, -3.152801135295367541 ) ) ;
#47748=VERTEX_POINT ( 'NONE', #43914 ) ;
#47750=CARTESIAN_POINT ( 'NONE',  ( 4.458734124999998549, -58.97916666530106511, -2.574251347313721627 ) ) ;
#47752=FACE_OUTER_BOUND ( 'NONE', #39859, .T. ) ;
#47753=CARTESIAN_POINT ( 'NONE',  ( -5.000000000000000000, 18.91666666666666430, -2.886751345948128211 ) ) ;
#47754=CARTESIAN_POINT ( 'NONE',  ( -2.499999999999996447, -88.83333333333332860, 4.330127018922195425 ) ) ;
#47756=CARTESIAN_POINT ( 'NONE',  ( -4.458734124999999437, -0.3958333319677397322, -2.574251347313719407 ) ) ;
#47757=DIRECTION ( 'NONE',  ( 0.000000000000000000, 0.000000000000000000, 1.000000000000000000 ) ) ;
#47758=CARTESIAN_POINT ( 'NONE',  ( -4.458734124999999437, 9.437500001365593860, 0.000000000000000000 ) ) ;
#47761=ORIENTED_EDGE ( 'NONE', *, *, #8728, .T. ) ;
#47762=CARTESIAN_POINT ( 'NONE',  ( 3.061616997868383141E-16, -167.8750000027312126, -5.000000000000000000 ) ) ;
#47763=CARTESIAN_POINT ( 'NONE',  ( -4.458734124999999437, -50.31249999863440792, 0.000000000000000000 ) ) ;
#47764=CARTESIAN_POINT ( 'NONE',  ( 1.846868145590735200, -158.5000000013656631, -4.458734125000000326 ) ) ;
#47765=CARTESIAN_POINT ( 'NONE',  ( -2.499999999999996447, -51.70833333060213732, 4.330127018922195425 ) ) ;
#47767=CARTESIAN_POINT ( 'NONE',  ( -3.152548672688508926E-16, -22.56249999863440081, -5.148502694627439702 ) ) ;
#47771=CARTESIAN_POINT ( 'NONE',  ( -4.458734125000000326, -161.0000000013656063, -1.846868145590735644 ) ) ;
#47772=( BOUNDED_CURVE ( )  B_SPLINE_CURVE ( 2, ( #41024, #27194, #26883, #51648, #7897, #56795, #12400, #32014, #51333 ),
 .UNSPECIFIED., .F., .F. ) 
 B_SPLINE_CURVE_WITH_KNOTS ( ( 3, 2, 2, 2, 3 ),
 ( 0.7270833333333333037, 0.7277777777777777457, 0.7291666666666666297, 0.7305555555555555136, 0.7312499999999999556 ),
 .UNSPECIFIED. ) 
 CURVE ( )  GEOMETRIC_REPRESENTATION_ITEM ( )  RATIONAL_B_SPLINE_CURVE ( ( 0.9330127018922194093, 0.9330127018922194093, 1.000000000000000000, 0.8660254037844387076, 1.000000000000000000, 0.8660254037844387076, 1.000000000000000000, 0.9330127018922194093, 0.9330127018922194093 ) ) 
 REPRESENTATION_ITEM ( '' )  );
#47773=FACE_OUTER_BOUND ( 'NONE', #18, .T. ) ;
#47775=CARTESIAN_POINT ( 'NONE',  ( 2.229367062499998831, -38.89583333196773651, -3.861377020970580887 ) ) ;
#47779=CARTESIAN_POINT ( 'NONE',  ( -6.972266317189433020E-16, -24.12499999726881228, -5.000000000000000000 ) ) ;
#47782=CARTESIAN_POINT ( 'NONE',  ( -3.152548672688508926E-16, -84.81249999863439371, -5.148502694627439702 ) ) ;
#47785=CARTESIAN_POINT ( 'NONE',  ( 3.061616997868383141E-16, -158.8750000027311842, -5.000000000000000000 ) ) ;
#47787=CARTESIAN_POINT ( 'NONE',  ( 5.000000000000000000, -37.50000000000000711, -6.123233995736766282E-16 ) ) ;
#47796=CARTESIAN_POINT ( 'NONE',  ( 2.229367062500001939, -87.22916666530107932, 3.861377020970579999 ) ) ;
#47802=CARTESIAN_POINT ( 'NONE',  ( 3.535533905932736864, -165.2500000027312126, 3.535533905932738641 ) ) ;
#47812=CARTESIAN_POINT ( 'NONE',  ( -4.458734124999999437, -13.39583333196774007, -2.574251347313719407 ) ) ;
#47815=CARTESIAN_POINT ( 'NONE',  ( -3.152548672688508926E-16, -39.81249999863440081, -5.148502694627439702 ) ) ;
#47821=CARTESIAN_POINT ( 'NONE',  ( 2.229367062500001939, 17.02083333469892779, 3.861377020970579999 ) ) ;
#47823=CARTESIAN_POINT ( 'NONE',  ( 1.975475456537005874E-15, -55.74999999999999289, 5.000000000000000000 ) ) ;
#47824=CARTESIAN_POINT ( 'NONE',  ( 2.229367062499998831, -86.89583333196773651, -3.861377020970580887 ) ) ;
#47826=CARTESIAN_POINT ( 'NONE',  ( -2.499999999999996447, 12.29166666939785202, 4.330127018922195425 ) ) ;
#47829=CARTESIAN_POINT ( 'NONE',  ( -1.339745962155623360, 16.20534180126147916, 4.999999999999991118 ) ) ;
#47831=CARTESIAN_POINT ( 'NONE',  ( -2.500000000000000444, -29.16666666666666785, -4.330127018922193649 ) ) ;
#47832=CARTESIAN_POINT ( 'NONE',  ( -3.152548672688508926E-16, -35.56249999863440792, -5.148502694627439702 ) ) ;
#47836=CARTESIAN_POINT ( 'NONE',  ( -2.499999999999996447, -34.70833333060213732, 4.330127018922195425 ) ) ;
#47837=CARTESIAN_POINT ( 'NONE',  ( 2.229367062500001939, -61.97916666530106511, 3.861377020970579999 ) ) ;
#47840=CARTESIAN_POINT ( 'NONE',  ( 2.229367062499998831, -8.895833331967736513, -3.861377020970580887 ) ) ;
#47841=ORIENTED_EDGE ( 'NONE', *, *, #15023, .T. ) ;
#47842=CARTESIAN_POINT ( 'NONE',  ( 5.000000000000000000, -77.50000000000000000, -6.123233995736766282E-16 ) ) ;
#47845=CARTESIAN_POINT ( 'NONE',  ( -5.000000000000000000, -75.87499999726880162, 0.000000000000000000 ) ) ;
#47846=CARTESIAN_POINT ( 'NONE',  ( 5.000000000000000000, -13.41666666666666785, -2.886751345948130876 ) ) ;
#47847=ORIENTED_EDGE ( 'NONE', *, *, #27823, .T. ) ;
#47849=CARTESIAN_POINT ( 'NONE',  ( 2.229367062499998831, -19.89583333196774007, -3.861377020970580887 ) ) ;
#47850=CARTESIAN_POINT ( 'NONE',  ( 4.458734125000001214, -55.14583333196772941, 2.574251347313718519 ) ) ;
#47852=( BOUNDED_CURVE ( )  B_SPLINE_CURVE ( 2, ( #33229, #18739, #18114, #23890, #4272, #3342, #62516, #3652, #42869 ),
 .UNSPECIFIED., .F., .F. ) 
 B_SPLINE_CURVE_WITH_KNOTS ( ( 3, 2, 2, 2, 3 ),
 ( 0.4312500000000000222, 0.4319444444444444642, 0.4333333333333333481, 0.4347222222222222321, 0.4354166666666666741 ),
 .UNSPECIFIED. ) 
 CURVE ( )  GEOMETRIC_REPRESENTATION_ITEM ( )  RATIONAL_B_SPLINE_CURVE ( ( 0.9330127018922194093, 0.9330127018922194093, 1.000000000000000000, 0.8660254037844387076, 1.000000000000000000, 0.8660254037844387076, 1.000000000000000000, 0.9330127018922194093, 0.9330127018922194093 ) ) 
 REPRESENTATION_ITEM ( '' )  );
#47854=CARTESIAN_POINT ( 'NONE',  ( -3.152801135295367985, -166.0625000013656063, 3.152801135295367096 ) ) ;
#47857=ORIENTED_EDGE ( 'NONE', *, *, #48885, .T. ) ;
#47864=CARTESIAN_POINT ( 'NONE',  ( -1.846868145590737420, -145.0000000013656063, 4.458734124999999437 ) ) ;
#47866=CARTESIAN_POINT ( 'NONE',  ( 1.975475456537005874E-15, -88.62499999726880162, 5.000000000000000000 ) ) ;
#47868=CARTESIAN_POINT ( 'NONE',  ( 4.458734124999998549, -70.97916666530107932, -2.574251347313721627 ) ) ;
#47870=CARTESIAN_POINT ( 'NONE',  ( -3.152801135295367985, -142.8125000013655779, 3.152801135295367096 ) ) ;
#47873=VECTOR ( 'NONE', #48662, 1000.000000000000000 ) ;
#47874=DIRECTION ( 'NONE',  ( 0.000000000000000000, 0.000000000000000000, 1.000000000000000000 ) ) ;
#47881=CARTESIAN_POINT ( 'NONE',  ( 4.458734124999998549, 22.02083333469892779, -2.574251347313721627 ) ) ;
#47889=CARTESIAN_POINT ( 'NONE',  ( 2.229367062499998831, 4.354166668032260823, -3.861377020970580887 ) ) ;
#47891=CARTESIAN_POINT ( 'NONE',  ( 2.229367062499998831, -23.89583333196773651, -3.861377020970580887 ) ) ;
#47892=CARTESIAN_POINT ( 'NONE',  ( 4.458734124999999437, -156.4375000013655779, 0.000000000000000000 ) ) ;
#47895=CARTESIAN_POINT ( 'NONE',  ( 2.626220312808019583E-14, 15.74999999999999645, -5.000000000000000000 ) ) ;
#47896=CARTESIAN_POINT ( 'NONE',  ( 9.457646018065525792E-16, -42.06249999863440081, 5.148502694627439702 ) ) ;
#47897=CARTESIAN_POINT ( 'NONE',  ( -5.000000000000000000, -84.08333333333332860, -2.886751345948128211 ) ) ;
#47899=CARTESIAN_POINT ( 'NONE',  ( -4.458734124999999437, -67.56249999863440792, 0.000000000000000000 ) ) ;
#47902=CARTESIAN_POINT ( 'NONE',  ( 5.000000000000000000, 28.70833333606451987, -2.886751345948129988 ) ) ;
#47903=ORIENTED_EDGE ( 'NONE', *, *, #55953, .F. ) ;
#47904=DIRECTION ( 'NONE',  ( -0.000000000000000000, 1.000000000000000000, -0.000000000000000000 ) ) ;
#47905=CARTESIAN_POINT ( 'NONE',  ( 2.499999999999998668, 2.791666669397851130, -4.330127018922193649 ) ) ;
#47906=CARTESIAN_POINT ( 'NONE',  ( -5.000000000000000000, -11.00000000000000355, 0.000000000000000000 ) ) ;
#47907=CARTESIAN_POINT ( 'NONE',  ( -2.229367062499996610, -19.14583333196774007, 3.861377020970582219 ) ) ;
#47908=ADVANCED_FACE ( 'NONE', ( #49064 ), #53270, .T. ) ;
#47909=CARTESIAN_POINT ( 'NONE',  ( -4.458734124999999437, -76.39583333196773651, -2.574251347313719407 ) ) ;
#47910=CARTESIAN_POINT ( 'NONE',  ( 5.000000000000000888, -59.45833333060214443, 2.886751345948126879 ) ) ;
#47911=CARTESIAN_POINT ( 'NONE',  ( 5.000000000000000000, -15.29166666393548368, -2.886751345948129988 ) ) ;
#47912=CARTESIAN_POINT ( 'NONE',  ( -4.458734124999998549, -44.22916666530106511, 2.574251347313722516 ) ) ;
#47914=CARTESIAN_POINT ( 'NONE',  ( 6.972266317189433020E-16, 29.74999999999999645, -5.000000000000000000 ) ) ;
#47915=CARTESIAN_POINT ( 'NONE',  ( 4.458734124999999437, 8.937500001365592084, -5.460374474430324690E-16 ) ) ;
#47916=ORIENTED_EDGE ( 'NONE', *, *, #58903, .F. ) ;
#47917=CARTESIAN_POINT ( 'NONE',  ( -1.339745962155613812, -87.08034179853028434, -5.000000000000000000 ) ) ;
#47918=CARTESIAN_POINT ( 'NONE',  ( -5.000000000000000000, -60.00000000000000000, 0.000000000000000000 ) ) ;
#47919=CARTESIAN_POINT ( 'NONE',  ( 4.458734124999999437, -155.6875000013655779, 0.000000000000000000 ) ) ;
#47921=CARTESIAN_POINT ( 'NONE',  ( -2.500000000000000444, -56.16666666666667140, -4.330127018922193649 ) ) ;
#47922=( BOUNDED_CURVE ( )  B_SPLINE_CURVE ( 2, ( #52048, #56878, #32417, #63588, #13742, #38800, #38195, #9544, #18574 ),
 .UNSPECIFIED., .F., .F. ) 
 B_SPLINE_CURVE_WITH_KNOTS ( ( 3, 2, 2, 2, 3 ),
 ( 0.9104166666666666519, 0.9111111111111110938, 0.9124999999999999778, 0.9138888888888888618, 0.9145833333333333037 ),
 .UNSPECIFIED. ) 
 CURVE ( )  GEOMETRIC_REPRESENTATION_ITEM ( )  RATIONAL_B_SPLINE_CURVE ( ( 0.9330127018922194093, 0.9330127018922194093, 1.000000000000000000, 0.8660254037844387076, 1.000000000000000000, 0.8660254037844387076, 1.000000000000000000, 0.9330127018922194093, 0.9330127018922194093 ) ) 
 REPRESENTATION_ITEM ( '' )  );
#47924=CARTESIAN_POINT ( 'NONE',  ( 2.071067811865476394, -166.1875000000000000, 5.000000000000000000 ) ) ;
#47926=CARTESIAN_POINT ( 'NONE',  ( 2.499999999999998668, -11.33333333333333393, -4.330127018922193649 ) ) ;
#47928=CARTESIAN_POINT ( 'NONE',  ( -3.152548672688508926E-16, -6.812499998634404363, -5.148502694627439702 ) ) ;
#47929=AXIS2_PLACEMENT_3D ( 'NONE', #53346, #43680, #39494 ) ;
#47930=CARTESIAN_POINT ( 'NONE',  ( 4.458734124999998549, -39.97916666530107221, -2.574251347313721627 ) ) ;
#47932=CARTESIAN_POINT ( 'NONE',  ( -1.846868145590737420, -147.7500000013655779, 4.458734124999999437 ) ) ;
#47936=CARTESIAN_POINT ( 'NONE',  ( 3.535533905932738197, -167.0000000027312126, -3.535533905932738197 ) ) ;
#47940=CARTESIAN_POINT ( 'NONE',  ( 4.458734124999998549, -68.97916666530106511, -2.574251347313721627 ) ) ;
#47941=CARTESIAN_POINT ( 'NONE',  ( 1.846868145590736310, -144.8750000013656063, 4.458734124999997661 ) ) ;
#47945=CARTESIAN_POINT ( 'NONE',  ( 1.339745962155612702, -79.16965819600730470, -5.000000000000000000 ) ) ;
#47946=CARTESIAN_POINT ( 'NONE',  ( 9.457646018065525792E-16, 2.937500001365594304, 5.148502694627439702 ) ) ;
#47947=CARTESIAN_POINT ( 'NONE',  ( -6.972266317189433020E-16, -43.25000000000000000, -5.000000000000000000 ) ) ;
#47948=CARTESIAN_POINT ( 'NONE',  ( -1.846868145590737420, -153.7500000013656063, 4.458734124999997661 ) ) ;
#47949=( BOUNDED_CURVE ( )  B_SPLINE_CURVE ( 2, ( #8914, #52042, #8599, #38190, #28209, #43004, #57815, #13737, #52973 ),
 .UNSPECIFIED., .F., .F. ) 
 B_SPLINE_CURVE_WITH_KNOTS ( ( 3, 2, 2, 2, 3 ),
 ( 0.7812500000000000000, 0.7819444444444444420, 0.7833333333333333259, 0.7847222222222222099, 0.7854166666666666519 ),
 .UNSPECIFIED. ) 
 CURVE ( )  GEOMETRIC_REPRESENTATION_ITEM ( )  RATIONAL_B_SPLINE_CURVE ( ( 0.9330127018922194093, 0.9330127018922194093, 1.000000000000000000, 0.8660254037844387076, 1.000000000000000000, 0.8660254037844387076, 1.000000000000000000, 0.9330127018922194093, 0.9330127018922194093 ) ) 
 REPRESENTATION_ITEM ( '' )  );
#47951=ORIENTED_EDGE ( 'NONE', *, *, #46406, .T. ) ;
#47960=CARTESIAN_POINT ( 'NONE',  ( -6.972266317189433020E-16, -48.12499999726880873, -5.000000000000000000 ) ) ;
#47962=CARTESIAN_POINT ( 'NONE',  ( -5.000000000000000000, -72.00000000000000000, 0.000000000000000000 ) ) ;
#47963=CARTESIAN_POINT ( 'NONE',  ( -4.458734124999997661, 24.77083333469893134, 2.574251347313722516 ) ) ;
#47965=CARTESIAN_POINT ( 'NONE',  ( 9.457646018065525792E-16, -1.312499998634406140, 5.148502694627439702 ) ) ;
#47966=CARTESIAN_POINT ( 'NONE',  ( -6.972266317189433020E-16, -63.25000000000000000, -5.000000000000000000 ) ) ;
#47968=CARTESIAN_POINT ( 'NONE',  ( -1.846868145590734756, -168.1250000013656063, -4.458734125000000326 ) ) ;
#47972=AXIS2_PLACEMENT_3D ( 'NONE', #12531, #51777, #17980 ) ;
#47979=CARTESIAN_POINT ( 'NONE',  ( 4.458734124999999437, -158.6250000013655779, -1.846868145590734978 ) ) ;
#47981=CYLINDRICAL_SURFACE ( 'NONE', #19221, 5.000000000000000000 ) ;
#47983=CARTESIAN_POINT ( 'NONE',  ( -3.152548672688508926E-16, 19.18750000136559208, -5.148502694627439702 ) ) ;
#47984=VERTEX_POINT ( 'NONE', #3762 ) ;
#47988=CARTESIAN_POINT ( 'NONE',  ( 2.499999999999998668, 12.66666666666666607, -4.330127018922193649 ) ) ;
#47989=CARTESIAN_POINT ( 'NONE',  ( -5.000000000000000000, 2.999999999999999112, 0.000000000000000000 ) ) ;
#47990=CARTESIAN_POINT ( 'NONE',  ( 4.458734124999998549, -61.72916666530106511, -2.574251347313721627 ) ) ;
#47994=CARTESIAN_POINT ( 'NONE',  ( 2.500000000000002220, 5.458333336064518981, 4.330127018922192761 ) ) ;
#47995=CARTESIAN_POINT ( 'NONE',  ( 4.458734125000001214, -27.89583333196774007, 2.574251347313718519 ) ) ;
#47996=CARTESIAN_POINT ( 'NONE',  ( 3.535533905932738197, -153.0000000027312126, -3.535533905932738197 ) ) ;
#47997=CARTESIAN_POINT ( 'NONE',  ( -5.000000000000000000, 26.04166666939784847, -2.886751345948128211 ) ) ;
#47998=EDGE_CURVE ( 'NONE', #53339, #21155, #36153, .T. ) ;
#47999=CYLINDRICAL_SURFACE ( 'NONE', #49433, 5.000000000000000000 ) ;
#48000=CARTESIAN_POINT ( 'NONE',  ( -2.500000000000000444, -44.16666666666665719, -4.330127018922193649 ) ) ;
#48003=CARTESIAN_POINT ( 'NONE',  ( 2.229367062500001939, -66.97916666530106511, 3.861377020970579999 ) ) ;
#48004=CARTESIAN_POINT ( 'NONE',  ( -3.152801135295367096, -147.3125000013655779, -3.152801135295367541 ) ) ;
#48005=CARTESIAN_POINT ( 'NONE',  ( -2.229367062499996610, -76.14583333196773651, 3.861377020970582219 ) ) ;
#48008=CARTESIAN_POINT ( 'NONE',  ( -2.229367062499996610, -27.39583333196774007, 3.861377020970582219 ) ) ;
#48009=CARTESIAN_POINT ( 'NONE',  ( 1.060575238724906964E-15, -63.62499999726881583, 5.773502691896257311 ) ) ;
#48010=VERTEX_POINT ( 'NONE', #10151 ) ;
#48014=CARTESIAN_POINT ( 'NONE',  ( 2.500000000000002220, 28.33333333333333215, 4.330127018922192761 ) ) ;
#48015=CARTESIAN_POINT ( 'NONE',  ( -6.972266317189433020E-16, -56.12499999726880162, -5.000000000000000000 ) ) ;
#48016=VECTOR ( 'NONE', #9789, 1000.000000000000000 ) ;
#48018=AXIS2_PLACEMENT_3D ( 'NONE', #53872, #3428, #9799 ) ;
#48019=EDGE_CURVE ( 'NONE', #24978, #45572, #27133, .T. ) ;
#48020=CARTESIAN_POINT ( 'NONE',  ( -5.000000000000000000, -82.99999999999998579, 0.000000000000000000 ) ) ;
#48021=CARTESIAN_POINT ( 'NONE',  ( -4.458734124999999437, -54.56249999863440081, 0.000000000000000000 ) ) ;
#48025=CARTESIAN_POINT ( 'NONE',  ( 6.123233995736766282E-16, -170.0000000000000000, -5.000000000000000000 ) ) ;
#48026=CARTESIAN_POINT ( 'NONE',  ( 4.458734125000001214, 16.10416666803225993, 2.574251347313718519 ) ) ;
#48028=CARTESIAN_POINT ( 'NONE',  ( -4.999999999999998224, -1.916666666666663854, 2.886751345948131764 ) ) ;
#48029=CARTESIAN_POINT ( 'NONE',  ( -4.458734124999999437, -163.9375000013655779, -5.460374474430324690E-16 ) ) ;
#48032=DIRECTION ( 'NONE',  ( 0.000000000000000000, 0.000000000000000000, 1.000000000000000000 ) ) ;
#48038=CARTESIAN_POINT ( 'NONE',  ( 0.000000000000000000, -170.0000000000000000, 0.000000000000000000 ) ) ;
#48040=CARTESIAN_POINT ( 'NONE',  ( 0.000000000000000000, -170.0000000000000000, 0.000000000000000000 ) ) ;
#48045=CARTESIAN_POINT ( 'NONE',  ( -5.000000000000000000, -151.6250000027312126, -6.123233995736766282E-16 ) ) ;
#48046=VERTEX_POINT ( 'NONE', #9188 ) ;
#48051=( BOUNDED_CURVE ( )  B_SPLINE_CURVE ( 2, ( #20034, #45757, #54123, #20687, #16169, #29993, #30313, #50261, #60250 ),
 .UNSPECIFIED., .F., .F. ) 
 B_SPLINE_CURVE_WITH_KNOTS ( ( 3, 2, 2, 2, 3 ),
 ( 0.1354166666666666574, 0.1361111111111110994, 0.1375000000000000111, 0.1388888888888888951, 0.1395833333333333370 ),
 .UNSPECIFIED. ) 
 CURVE ( )  GEOMETRIC_REPRESENTATION_ITEM ( )  RATIONAL_B_SPLINE_CURVE ( ( 0.9330127018922194093, 0.9330127018922194093, 1.000000000000000000, 0.8660254037844387076, 1.000000000000000000, 0.8660254037844387076, 1.000000000000000000, 0.9330127018922194093, 0.9330127018922194093 ) ) 
 REPRESENTATION_ITEM ( '' )  );
#48052=CARTESIAN_POINT ( 'NONE',  ( -3.535533905932737309, -142.6250000000000000, -3.535533905932738197 ) ) ;
#48055=CARTESIAN_POINT ( 'NONE',  ( 4.458734124999999437, -169.6875000013656063, 0.000000000000000000 ) ) ;
#48056=CARTESIAN_POINT ( 'NONE',  ( -3.152548672688508926E-16, -32.56249999863440792, -5.148502694627439702 ) ) ;
#48060=CARTESIAN_POINT ( 'NONE',  ( 4.458734125000000326, -149.3750000013656347, -1.846868145590734978 ) ) ;
#48063=CARTESIAN_POINT ( 'NONE',  ( 9.457646018065525792E-16, -55.31249999863439371, 5.148502694627439702 ) ) ;
#48065=DIRECTION ( 'NONE',  ( -0.000000000000000000, 1.000000000000000000, -0.000000000000000000 ) ) ;
#48066=CARTESIAN_POINT ( 'NONE',  ( 2.500000000000002220, 18.33333333333333215, 4.330127018922192761 ) ) ;
#48067=LINE ( 'NONE', #28137, #6952 ) ;
#48068=CARTESIAN_POINT ( 'NONE',  ( -4.458734124999998549, 0.7708333346989267865, 2.574251347313722516 ) ) ;
#48069=CARTESIAN_POINT ( 'NONE',  ( -5.000000000000000888, -154.4375000000000000, 2.071067811865474617 ) ) ;
#48070=EDGE_CURVE ( 'NONE', #53780, #26245, #57453, .T. ) ;
#48071=CARTESIAN_POINT ( 'NONE',  ( -9.184850993605147944E-16, -164.3750000027311842, 5.000000000000000000 ) ) ;
#48072=CARTESIAN_POINT ( 'NONE',  ( -4.458734124999999437, 10.35416666803225816, -2.574251347313719407 ) ) ;
#48073=CARTESIAN_POINT ( 'NONE',  ( -6.972266317189433020E-16, -53.12499999726880162, -5.000000000000000000 ) ) ;
#48076=CARTESIAN_POINT ( 'NONE',  ( -3.152548672688508926E-16, -48.56249999863440792, -5.148502694627439702 ) ) ;
#48077=CARTESIAN_POINT ( 'NONE',  ( -3.152801135295367096, -161.3125000013656063, -3.152801135295367541 ) ) ;
#48078=AXIS2_PLACEMENT_3D ( 'NONE', #30615, #59911, #35447 ) ;
#48079=CARTESIAN_POINT ( 'NONE',  ( 5.000000000000000000, -52.37499999726881583, -6.123233995736766282E-16 ) ) ;
#48081=CARTESIAN_POINT ( 'NONE',  ( -4.458734124999998549, -23.22916666530107221, 2.574251347313722516 ) ) ;
#48082=ORIENTED_EDGE ( 'NONE', *, *, #411, .T. ) ;
#48084=CARTESIAN_POINT ( 'NONE',  ( 3.152801135295367541, -159.3125000013656063, -3.152801135295367541 ) ) ;
#48085=EDGE_CURVE ( 'NONE', #11953, #14479, #57776, .T. ) ;
#48090=CARTESIAN_POINT ( 'NONE',  ( -4.458734124999999437, -37.64583333196773651, -2.574251347313719407 ) ) ;
#48096=( BOUNDED_CURVE ( )  B_SPLINE_CURVE ( 2, ( #55702, #20323, #24828, #25141, #10662, #34798, #40258, #29639, #40885 ),
 .UNSPECIFIED., .F., .F. ) 
 B_SPLINE_CURVE_WITH_KNOTS ( ( 3, 2, 2, 2, 3 ),
 ( 0.5104166666666666297, 0.5111111111111110716, 0.5124999999999999556, 0.5138888888888888395, 0.5145833333333332815 ),
 .UNSPECIFIED. ) 
 CURVE ( )  GEOMETRIC_REPRESENTATION_ITEM ( )  RATIONAL_B_SPLINE_CURVE ( ( 0.9330127018922194093, 0.9330127018922194093, 1.000000000000000000, 0.8660254037844387076, 1.000000000000000000, 0.8660254037844387076, 1.000000000000000000, 0.9330127018922194093, 0.9330127018922194093 ) ) 
 REPRESENTATION_ITEM ( '' )  );
#48099=CARTESIAN_POINT ( 'NONE',  ( 4.458734125000001214, -85.14583333196773651, 2.574251347313718519 ) ) ;
#48101=CARTESIAN_POINT ( 'NONE',  ( 2.500000000000002220, -35.54166666393547303, 4.330127018922192761 ) ) ;
#48102=CARTESIAN_POINT ( 'NONE',  ( 1.975475456537005874E-15, 0.3750000027311862216, 5.000000000000000000 ) ) ;
#48104=AXIS2_PLACEMENT_3D ( 'NONE', #20869, #51409, #36930 ) ;
#48106=CARTESIAN_POINT ( 'NONE',  ( 1.975475456537005874E-15, -84.62499999726880162, 5.000000000000000000 ) ) ;
#48114=CARTESIAN_POINT ( 'NONE',  ( -6.972266317189433020E-16, -46.12499999726880873, -5.000000000000000000 ) ) ;
#48115=CARTESIAN_POINT ( 'NONE',  ( 4.458734125000001214, -82.14583333196772230, 2.574251347313718519 ) ) ;
#48119=CARTESIAN_POINT ( 'NONE',  ( 1.975475456537005874E-15, -9.624999997268814056, 5.000000000000000000 ) ) ;
#48121=CARTESIAN_POINT ( 'NONE',  ( -3.535533905932738641, -166.5000000027312126, 3.535533905932737309 ) ) ;
#48124=CARTESIAN_POINT ( 'NONE',  ( -1.339745962155613812, -30.20534180126148271, -5.000000000000000000 ) ) ;
#48125=AXIS2_PLACEMENT_3D ( 'NONE', #36821, #32940, #61591 ) ;
#48133=CARTESIAN_POINT ( 'NONE',  ( 4.458734124999998549, -11.72916666530107044, -2.574251347313721627 ) ) ;
#48135=ORIENTED_EDGE ( 'NONE', *, *, #54784, .T. ) ;
#48136=CARTESIAN_POINT ( 'NONE',  ( -2.229367062500000163, -38.72916666530107221, -3.861377020970580443 ) ) ;
#48137=DIRECTION ( 'NONE',  ( -0.000000000000000000, 1.000000000000000000, -0.000000000000000000 ) ) ;
#48139=CARTESIAN_POINT ( 'NONE',  ( -5.000000000000000000, 27.12500000273118772, 0.000000000000000000 ) ) ;
#48142=CARTESIAN_POINT ( 'NONE',  ( 4.458734125000001214, 13.10416666803226171, 2.574251347313718519 ) ) ;
#48146=CARTESIAN_POINT ( 'NONE',  ( -2.229367062499996610, -86.39583333196773651, 3.861377020970582219 ) ) ;
#48148=CARTESIAN_POINT ( 'NONE',  ( 1.060575238724906964E-15, 14.37500000273118594, 5.773502691896257311 ) ) ;
#48149=ORIENTED_EDGE ( 'NONE', *, *, #17654, .F. ) ;
#48151=VECTOR ( 'NONE', #54156, 1000.000000000000000 ) ;
#48152=CARTESIAN_POINT ( 'NONE',  ( 3.535533905932736864, -167.1250000000000284, 3.535533905932738641 ) ) ;
#48153=( BOUNDED_CURVE ( )  B_SPLINE_CURVE ( 2, ( #154, #52053, #49012, #27907, #39361, #58992, #4961, #7677, #27591 ),
 .UNSPECIFIED., .F., .F. ) 
 B_SPLINE_CURVE_WITH_KNOTS ( ( 3, 2, 2, 2, 3 ),
 ( 0.2437499999999999944, 0.2444444444444444364, 0.2458333333333333204, 0.2472222222222222321, 0.2479166666666666741 ),
 .UNSPECIFIED. ) 
 CURVE ( )  GEOMETRIC_REPRESENTATION_ITEM ( )  RATIONAL_B_SPLINE_CURVE ( ( 0.9330127018922194093, 0.9330127018922194093, 1.000000000000000000, 0.8660254037844387076, 1.000000000000000000, 0.8660254037844387076, 1.000000000000000000, 0.9330127018922194093, 0.9330127018922194093 ) ) 
 REPRESENTATION_ITEM ( '' )  );
#48154=CARTESIAN_POINT ( 'NONE',  ( 1.975475456537005874E-15, 2.249999999999999556, 5.000000000000000000 ) ) ;
#48155=CARTESIAN_POINT ( 'NONE',  ( -4.999999999999999112, -28.91666666666666430, 2.886751345948131764 ) ) ;
#48156=CARTESIAN_POINT ( 'NONE',  ( -4.458734124999998549, -32.22916666530106511, 2.574251347313722516 ) ) ;
#48157=CARTESIAN_POINT ( 'NONE',  ( -2.500000000000000444, -36.04166666393547303, -4.330127018922193649 ) ) ;
#48158=CARTESIAN_POINT ( 'NONE',  ( 2.229367062500001939, -62.97916666530106511, 3.861377020970579999 ) ) ;
#48159=ORIENTED_EDGE ( 'NONE', *, *, #45623, .T. ) ;
#48161=CARTESIAN_POINT ( 'NONE',  ( 4.458734125000001214, -12.14583333196774007, 2.574251347313718519 ) ) ;
#48163=CARTESIAN_POINT ( 'NONE',  ( -2.499999999999996447, -78.83333333333332860, 4.330127018922195425 ) ) ;
#48166=CARTESIAN_POINT ( 'NONE',  ( -2.500000000000000444, -81.04166666393547303, -4.330127018922193649 ) ) ;
#48167=DIRECTION ( 'NONE',  ( -0.000000000000000000, 1.000000000000000000, -0.000000000000000000 ) ) ;
#48170=CARTESIAN_POINT ( 'NONE',  ( -2.229367062500000163, -21.72916666530107221, -3.861377020970580443 ) ) ;
#48172=CARTESIAN_POINT ( 'NONE',  ( -4.458734124999999437, -57.56249999863440081, 0.000000000000000000 ) ) ;
#48175=CARTESIAN_POINT ( 'NONE',  ( 2.730187237215162345E-16, -167.4375000013655779, -4.458734124999999437 ) ) ;
#48177=CARTESIAN_POINT ( 'NONE',  ( 3.061616997868383141E-16, -167.8750000027312126, -5.000000000000000000 ) ) ;
#48178=ORIENTED_EDGE ( 'NONE', *, *, #44512, .T. ) ;
#48185=CARTESIAN_POINT ( 'NONE',  ( -3.152801135295367985, -143.0625000013655779, 3.152801135295367096 ) ) ;
#48187=CARTESIAN_POINT ( 'NONE',  ( 5.000000000000000000, -70.41666666666667140, -2.886751345948130876 ) ) ;
#48189=CARTESIAN_POINT ( 'NONE',  ( -4.458734124999998549, -69.47916666530107932, 2.574251347313722516 ) ) ;
#48191=CARTESIAN_POINT ( 'NONE',  ( -2.499999999999996447, -42.70833333060214443, 4.330127018922195425 ) ) ;
#48192=CARTESIAN_POINT ( 'NONE',  ( 1.846868145590736310, -141.6250000013656347, 4.458734124999997661 ) ) ;
#48194=ORIENTED_EDGE ( 'NONE', *, *, #53528, .T. ) ;
#48196=DIRECTION ( 'NONE',  ( -0.000000000000000000, 1.000000000000000000, -0.000000000000000000 ) ) ;
#48199=CARTESIAN_POINT ( 'NONE',  ( -6.972266317189433020E-16, -14.12499999726881228, -5.000000000000000000 ) ) ;
#48202=CARTESIAN_POINT ( 'NONE',  ( 4.458734125000000326, 20.85416666803226349, 2.574251347313718519 ) ) ;
#48203=FACE_OUTER_BOUND ( 'NONE', #63282, .T. ) ;
#48208=CARTESIAN_POINT ( 'NONE',  ( 5.000000000000000000, -60.29166666393547303, -2.886751345948130876 ) ) ;
#48209=CARTESIAN_POINT ( 'NONE',  ( -4.458734124999999437, 3.604166668032260379, -2.574251347313719407 ) ) ;
#48210=CARTESIAN_POINT ( 'NONE',  ( 9.457646018065525792E-16, -25.31249999863440792, 5.148502694627439702 ) ) ;
#48211=CARTESIAN_POINT ( 'NONE',  ( -3.152801135295367096, -154.0625000013656063, -3.152801135295367541 ) ) ;
#48217=CARTESIAN_POINT ( 'NONE',  ( -2.229367062500000163, -70.72916666530107932, -3.861377020970580443 ) ) ;
#48219=DIRECTION ( 'NONE',  ( -0.000000000000000000, 1.000000000000000000, -0.000000000000000000 ) ) ;
#48220=CARTESIAN_POINT ( 'NONE',  ( 5.000000000000000888, 28.54166666939785202, 2.886751345948126879 ) ) ;
#48222=CARTESIAN_POINT ( 'NONE',  ( -2.500000000000000444, -14.16666666666666785, -4.330127018922193649 ) ) ;
#48223=CARTESIAN_POINT ( 'NONE',  ( -4.458734124999999437, -14.39583333196773474, -2.574251347313719407 ) ) ;
#48224=CARTESIAN_POINT ( 'NONE',  ( -3.152548672688508926E-16, -76.56249999863440792, -5.148502694627439702 ) ) ;
#48225=( BOUNDED_CURVE ( )  B_SPLINE_CURVE ( 2, ( #61407, #60458, #17015, #56263, #26343, #27296, #26984, #16384, #2866 ),
 .UNSPECIFIED., .F., .F. ) 
 B_SPLINE_CURVE_WITH_KNOTS ( ( 3, 2, 2, 2, 3 ),
 ( 0.9645833333333333481, 0.9652777777777777901, 0.9666666666666666741, 0.9680555555555555580, 0.9687500000000000000 ),
 .UNSPECIFIED. ) 
 CURVE ( )  GEOMETRIC_REPRESENTATION_ITEM ( )  RATIONAL_B_SPLINE_CURVE ( ( 0.9330127018922194093, 0.9330127018922194093, 1.000000000000000000, 0.8660254037844387076, 1.000000000000000000, 0.8660254037844387076, 1.000000000000000000, 0.9330127018922194093, 0.9330127018922194093 ) ) 
 REPRESENTATION_ITEM ( '' )  );
#48226=CARTESIAN_POINT ( 'NONE',  ( -8.190561711645485556E-16, -166.9375000013655779, 4.458734124999999437 ) ) ;
#48227=CARTESIAN_POINT ( 'NONE',  ( -2.499999999999996447, -20.70833333060214798, 4.330127018922195425 ) ) ;
#48228=CARTESIAN_POINT ( 'NONE',  ( -2.229367062499996610, -42.14583333196773651, 3.861377020970582219 ) ) ;
#48229=EDGE_LOOP ( 'NONE', ( #57768, #31013, #47239, #45163 ) ) ;
#48231=CARTESIAN_POINT ( 'NONE',  ( -2.229367062499996610, 8.604166668032261711, 3.861377020970582219 ) ) ;
#48234=CARTESIAN_POINT ( 'NONE',  ( -3.535250795749689387E-16, -61.25000000000000000, -5.773502691896257311 ) ) ;
#48235=CARTESIAN_POINT ( 'NONE',  ( 3.152801135295367541, -155.5625000013656063, -3.152801135295367541 ) ) ;
#48239=CARTESIAN_POINT ( 'NONE',  ( -3.535533905932738641, -161.3750000000000284, 3.535533905932737309 ) ) ;
#48240=CARTESIAN_POINT ( 'NONE',  ( 2.500000000000002220, 5.458333336064518981, 4.330127018922192761 ) ) ;
#48243=CARTESIAN_POINT ( 'NONE',  ( 4.458734125000001214, -8.145833331967736513, 2.574251347313718519 ) ) ;
#48244=CARTESIAN_POINT ( 'NONE',  ( 9.457646018065525792E-16, -41.31249999863440081, 5.148502694627439702 ) ) ;
#48246=CARTESIAN_POINT ( 'NONE',  ( 4.458734125000000326, -149.3750000013656347, -1.846868145590734978 ) ) ;
#48248=CARTESIAN_POINT ( 'NONE',  ( 5.000000000000000000, -167.1875000027312126, 2.071067811865478614 ) ) ;
#48250=CARTESIAN_POINT ( 'NONE',  ( -4.999999999999998224, 3.208333336064520758, 2.886751345948131764 ) ) ;
#48253=CARTESIAN_POINT ( 'NONE',  ( -4.458734124999999437, -77.64583333196773651, -2.574251347313719407 ) ) ;
#48254=ORIENTED_EDGE ( 'NONE', *, *, #61347, .T. ) ;
#48258=CARTESIAN_POINT ( 'NONE',  ( 4.458734125000001214, -1.895833331967737623, 2.574251347313718519 ) ) ;
#48259=CARTESIAN_POINT ( 'NONE',  ( -2.499999999999996447, -42.83333333333333570, 4.330127018922195425 ) ) ;
#48260=CARTESIAN_POINT ( 'NONE',  ( -8.190561711645485556E-16, -154.6875000013655779, 4.458734124999999437 ) ) ;
#48262=ORIENTED_EDGE ( 'NONE', *, *, #61683, .T. ) ;
#48267=EDGE_CURVE ( 'NONE', #22693, #44005, #49286, .T. ) ;
#48269=DIRECTION ( 'NONE',  ( -0.000000000000000000, 1.000000000000000000, -0.000000000000000000 ) ) ;
#48275=CARTESIAN_POINT ( 'NONE',  ( 9.457646018065525792E-16, 17.93750000136559208, 5.148502694627439702 ) ) ;
#48277=CARTESIAN_POINT ( 'NONE',  ( 4.458734124999998549, -10.97916666530107044, -2.574251347313721627 ) ) ;
#48278=CARTESIAN_POINT ( 'NONE',  ( 6.123233995736766282E-16, -170.0000000000000000, -5.000000000000000000 ) ) ;
#48280=CARTESIAN_POINT ( 'NONE',  ( 1.846868145590736310, -167.6250000013655779, 4.458734124999999437 ) ) ;
#48288=CARTESIAN_POINT ( 'NONE',  ( 0.000000000000000000, -170.0000000000000000, 0.000000000000000000 ) ) ;
#48289=VECTOR ( 'NONE', #28343, 1000.000000000000000 ) ;
#48290=ADVANCED_FACE ( 'NONE', ( #34564 ), #10447, .T. ) ;
#48292=CARTESIAN_POINT ( 'NONE',  ( -1.846868145590734756, -159.3750000013656063, -4.458734124999999437 ) ) ;
#48294=DIRECTION ( 'NONE',  ( -0.000000000000000000, 1.000000000000000000, -0.000000000000000000 ) ) ;
#48300=CARTESIAN_POINT ( 'NONE',  ( -9.184850993605147944E-16, -158.2500000000000000, 5.000000000000000000 ) ) ;
#48301=CARTESIAN_POINT ( 'NONE',  ( -5.000000000000000000, 1.000000000000000888, 0.000000000000000000 ) ) ;
#48303=CARTESIAN_POINT ( 'NONE',  ( 2.229367062500001939, -59.97916666530106511, 3.861377020970579999 ) ) ;
#48304=CARTESIAN_POINT ( 'NONE',  ( -9.184850993605147944E-16, -162.2500000000000000, 5.000000000000000000 ) ) ;
#48305=CARTESIAN_POINT ( 'NONE',  ( -2.500000000000000444, -0.04166666393548221214, -4.330127018922193649 ) ) ;
#48306=CARTESIAN_POINT ( 'NONE',  ( 4.458734125000001214, -28.89583333196774007, 2.574251347313718519 ) ) ;
#48310=CARTESIAN_POINT ( 'NONE',  ( 5.000000000000000000, -42.41666666666667140, -2.886751345948129988 ) ) ;
#48313=CARTESIAN_POINT ( 'NONE',  ( 2.500000000000002220, -64.66666666666665719, 4.330127018922192761 ) ) ;
#48314=CARTESIAN_POINT ( 'NONE',  ( 9.457646018065525792E-16, -70.06249999863439371, 5.148502694627439702 ) ) ;
#48315=CARTESIAN_POINT ( 'NONE',  ( -1.846868145590734756, -146.3750000013655779, -4.458734125000000326 ) ) ;
#48317=CARTESIAN_POINT ( 'NONE',  ( -4.458734124999999437, -78.31249999863440792, 0.000000000000000000 ) ) ;
#48319=CARTESIAN_POINT ( 'NONE',  ( -4.458734124999998549, -22.47916666530107577, 2.574251347313722516 ) ) ;
#48320=CARTESIAN_POINT ( 'NONE',  ( -2.499999999999996447, -66.70833333060214443, 4.330127018922195425 ) ) ;
#48323=CARTESIAN_POINT ( 'NONE',  ( -5.000000000000000888, -152.5625000027311842, 2.071067811865474617 ) ) ;
#48326=CARTESIAN_POINT ( 'NONE',  ( -1.510657702057710340E-15, 28.25000000000000000, 5.000000000000000000 ) ) ;
#48329=VECTOR ( 'NONE', #42513, 1000.000000000000000 ) ;
#48331=CARTESIAN_POINT ( 'NONE',  ( -1.339745962155660663, -2.794658198738523058, 4.999999999999972466 ) ) ;
#48333=CARTESIAN_POINT ( 'NONE',  ( -4.458734124999999437, -60.56249999863440081, 0.000000000000000000 ) ) ;
#48335=ORIENTED_EDGE ( 'NONE', *, *, #33933, .F. ) ;
#48337=CARTESIAN_POINT ( 'NONE',  ( -4.458734124999998549, 16.77083333469892779, 2.574251347313722516 ) ) ;
#48340=AXIS2_PLACEMENT_3D ( 'NONE', #49200, #24759, #39222 ) ;
#48341=CARTESIAN_POINT ( 'NONE',  ( 1.846868145590735200, -166.2500000013656063, -4.458734124999999437 ) ) ;
#48344=LINE ( 'NONE', #25168, #31548 ) ;
#48346=EDGE_CURVE ( 'NONE', #41941, #62409, #55879, .T. ) ;
#48347=EDGE_CURVE ( 'NONE', #44647, #42718, #33691, .T. ) ;
#48348=CARTESIAN_POINT ( 'NONE',  ( -5.000000000000000888, -162.6875000027311842, -2.071067811865475949 ) ) ;
#48352=CARTESIAN_POINT ( 'NONE',  ( 6.123233995736766282E-16, -170.0000000000000000, -5.000000000000000000 ) ) ;
#48355=CARTESIAN_POINT ( 'NONE',  ( 1.339745962155612702, -18.16965819600733312, -5.000000000000000000 ) ) ;
#48356=CYLINDRICAL_SURFACE ( 'NONE', #23236, 5.000000000000000000 ) ;
#48361=CARTESIAN_POINT ( 'NONE',  ( 5.000000000000000000, -151.1875000027312126, 2.071067811865478614 ) ) ;
#48367=CARTESIAN_POINT ( 'NONE',  ( 3.535533905932736864, -142.1250000000000000, 3.535533905932738641 ) ) ;
#48370=CARTESIAN_POINT ( 'NONE',  ( 3.152801135295366208, -167.8125000013656063, 3.152801135295367985 ) ) ;
#48371=CARTESIAN_POINT ( 'NONE',  ( 2.229367062500001939, -27.97916666530107221, 3.861377020970579999 ) ) ;
#48375=CARTESIAN_POINT ( 'NONE',  ( -3.152801135295367096, -148.0625000013655779, -3.152801135295367541 ) ) ;
#48377=CARTESIAN_POINT ( 'NONE',  ( -3.152548672688508926E-16, 29.18750000136559208, -5.148502694627439702 ) ) ;
#48379=CARTESIAN_POINT ( 'NONE',  ( -2.229367062500000163, -56.72916666530107221, -3.861377020970580443 ) ) ;
#48381=CARTESIAN_POINT ( 'NONE',  ( -5.000000000000000888, -162.4375000000000568, 2.071067811865474617 ) ) ;
#48382=CARTESIAN_POINT ( 'NONE',  ( 5.000000000000000888, 18.41666666666666430, 2.886751345948126879 ) ) ;
#48385=CARTESIAN_POINT ( 'NONE',  ( 4.458734125000001214, -4.895833331967740065, 2.574251347313718519 ) ) ;
#48387=CARTESIAN_POINT ( 'NONE',  ( 1.975475456537005874E-15, -8.750000000000000000, 5.000000000000000000 ) ) ;
#48388=CARTESIAN_POINT ( 'NONE',  ( 4.458734124999998549, 8.020833334698926009, -2.574251347313721627 ) ) ;
#48391=CARTESIAN_POINT ( 'NONE',  ( 2.229367062500001939, -51.97916666530107221, 3.861377020970579999 ) ) ;
#48392=CARTESIAN_POINT ( 'NONE',  ( 2.730187237215162345E-16, -160.4375000013655779, -4.458734124999999437 ) ) ;
#48393=CARTESIAN_POINT ( 'NONE',  ( 5.000000000000000000, -52.29166666393548013, -2.886751345948129988 ) ) ;
#48395=CARTESIAN_POINT ( 'NONE',  ( -2.229367062499996610, 3.604166668032260379, 3.861377020970582219 ) ) ;
#48398=CARTESIAN_POINT ( 'NONE',  ( -5.000000000000000888, -142.6875000027312126, -2.071067811865475949 ) ) ;
#48399=CARTESIAN_POINT ( 'NONE',  ( 1.846868145590736310, -158.6250000013655779, 4.458734124999999437 ) ) ;
#48400=ORIENTED_EDGE ( 'NONE', *, *, #39621, .F. ) ;
#48401=CARTESIAN_POINT ( 'NONE',  ( -6.972266317189433020E-16, -62.12499999726880162, -5.000000000000000000 ) ) ;
#48403=CARTESIAN_POINT ( 'NONE',  ( 2.500000000000002220, -47.54166666393547303, 4.330127018922192761 ) ) ;
#48404=CARTESIAN_POINT ( 'NONE',  ( -4.458734124999998549, -38.47916666530107221, 2.574251347313722516 ) ) ;
#48406=LINE ( 'NONE', #9792, #13133 ) ;
#48410=CARTESIAN_POINT ( 'NONE',  ( 4.458734124999998549, -85.97916666530107932, -2.574251347313721627 ) ) ;
#48412=CARTESIAN_POINT ( 'NONE',  ( -6.972266317189433020E-16, 24.87500000273118417, -5.000000000000000000 ) ) ;
#48414=CARTESIAN_POINT ( 'NONE',  ( 3.535533905932736864, -169.1250000000000284, 3.535533905932738641 ) ) ;
#48417=VECTOR ( 'NONE', #55574, 1000.000000000000000 ) ;
#48420=( BOUNDED_CURVE ( )  B_SPLINE_CURVE ( 2, ( #26552, #2133, #51641, #8207, #60661, #22689, #12706, #21736, #47435 ),
 .UNSPECIFIED., .F., .F. ) 
 B_SPLINE_CURVE_WITH_KNOTS ( ( 3, 2, 2, 2, 3 ),
 ( 0.7583333333333330817, 0.7624999999999997335, 0.7666666666666664964, 0.7708333333333331483, 0.7749999999999998002 ),
 .UNSPECIFIED. ) 
 CURVE ( )  GEOMETRIC_REPRESENTATION_ITEM ( )  RATIONAL_B_SPLINE_CURVE ( ( 1.000000000000003997, 0.9238795325112826307, 1.000000000000000000, 0.9238795325112867385, 1.000000000000000000, 0.9238795325112867385, 1.000000000000000000, 0.9238795325112908463, 0.9999999999999958922 ) ) 
 REPRESENTATION_ITEM ( '' )  );
#48422=EDGE_CURVE ( 'NONE', #42211, #48477, #46364, .T. ) ;
#48425=CARTESIAN_POINT ( 'NONE',  ( 0.000000000000000000, -170.0000000000000000, 0.000000000000000000 ) ) ;
#48426=CARTESIAN_POINT ( 'NONE',  ( -5.000000000000000000, -66.87499999726881583, 0.000000000000000000 ) ) ;
#48427=CARTESIAN_POINT ( 'NONE',  ( -4.458734124999999437, -85.56249999863439371, 0.000000000000000000 ) ) ;
#48434=CARTESIAN_POINT ( 'NONE',  ( -2.071067811865478170, -163.4375000027311842, 5.000000000000000000 ) ) ;
#48438=DIRECTION ( 'NONE',  ( -0.000000000000000000, 1.000000000000000000, -0.000000000000000000 ) ) ;
#48445=DIRECTION ( 'NONE',  ( 0.000000000000000000, 0.000000000000000000, 1.000000000000000000 ) ) ;
#48446=CARTESIAN_POINT ( 'NONE',  ( 4.458734124999998549, -13.72916666530107399, -2.574251347313721627 ) ) ;
#48448=CARTESIAN_POINT ( 'NONE',  ( -5.000000000000000888, -154.5625000000000000, -2.071067811865475949 ) ) ;
#48451=CARTESIAN_POINT ( 'NONE',  ( -3.152548672688508926E-16, -41.81249999863440081, -5.148502694627439702 ) ) ;
#48455=DIRECTION ( 'NONE',  ( 0.000000000000000000, 0.000000000000000000, 1.000000000000000000 ) ) ;
#48458=CARTESIAN_POINT ( 'NONE',  ( -4.458734124999999437, 10.68750000136559386, 0.000000000000000000 ) ) ;
#48460=CARTESIAN_POINT ( 'NONE',  ( -2.500000000000000444, -82.04166666393547303, -4.330127018922193649 ) ) ;
#48461=CARTESIAN_POINT ( 'NONE',  ( -3.535533905932737309, -165.7500000027312126, -3.535533905932738197 ) ) ;
#48464=CARTESIAN_POINT ( 'NONE',  ( 5.000000000000000000, 12.62500000273118417, -6.123233995736766282E-16 ) ) ;
#48466=CARTESIAN_POINT ( 'NONE',  ( -2.499999999999996447, -6.708333330602149758, 4.330127018922195425 ) ) ;
#48470=CARTESIAN_POINT ( 'NONE',  ( 5.000000000000000888, -30.58333333333332860, 2.886751345948126879 ) ) ;
#48471=CARTESIAN_POINT ( 'NONE',  ( -3.152548672688508926E-16, -33.56249999863440792, -5.148502694627439702 ) ) ;
#48472=CARTESIAN_POINT ( 'NONE',  ( -5.000000000000000000, -33.87499999726880873, 0.000000000000000000 ) ) ;
#48473=CARTESIAN_POINT ( 'NONE',  ( 9.457646018065525792E-16, -67.06249999863440792, 5.148502694627439702 ) ) ;
#48474=VERTEX_POINT ( 'NONE', #21711 ) ;
#48476=CARTESIAN_POINT ( 'NONE',  ( -2.229367062499996610, -15.39583333196773651, 3.861377020970582219 ) ) ;
#48477=VERTEX_POINT ( 'NONE', #1787 ) ;
#48478=CARTESIAN_POINT ( 'NONE',  ( 5.000000000000000000, -79.41666666666665719, -2.886751345948129988 ) ) ;
#48482=CARTESIAN_POINT ( 'NONE',  ( -2.499999999999996447, -82.70833333060214443, 4.330127018922195425 ) ) ;
#48484=ORIENTED_EDGE ( 'NONE', *, *, #32676, .T. ) ;
#48486=CARTESIAN_POINT ( 'NONE',  ( 2.229367062500001939, -22.22916666530107221, 3.861377020970579999 ) ) ;
#48487=CARTESIAN_POINT ( 'NONE',  ( 9.457646018065525792E-16, -60.31249999863440792, 5.148502694627439702 ) ) ;
#48490=CARTESIAN_POINT ( 'NONE',  ( -4.458734125000000326, -167.2500000013655779, -1.846868145590735644 ) ) ;
#48492=CARTESIAN_POINT ( 'NONE',  ( 1.339745962155615144, -8.580341798530293218, 4.999999999999999112 ) ) ;
#48493=ORIENTED_EDGE ( 'NONE', *, *, #26837, .T. ) ;
#48500=CARTESIAN_POINT ( 'NONE',  ( 1.846868145590735200, -145.5000000013655779, -4.458734125000000326 ) ) ;
#48502=CARTESIAN_POINT ( 'NONE',  ( -6.972266317189433020E-16, -61.25000000000000000, -5.000000000000000000 ) ) ;
#48504=CARTESIAN_POINT ( 'NONE',  ( 2.229367062500001939, -68.22916666530106511, 3.861377020970579999 ) ) ;
#48506=CARTESIAN_POINT ( 'NONE',  ( 1.975475456537005874E-15, -54.62499999726880873, 5.000000000000000000 ) ) ;
#48507=CARTESIAN_POINT ( 'NONE',  ( -3.152801135295367096, -141.0625000013655779, -3.152801135295367541 ) ) ;
#48510=CARTESIAN_POINT ( 'NONE',  ( -2.500000000000000444, -71.04166666393547303, -4.330127018922193649 ) ) ;
#48511=CARTESIAN_POINT ( 'NONE',  ( 5.000000000000000000, -160.0000000000000000, 0.000000000000000000 ) ) ;
#48516=CARTESIAN_POINT ( 'NONE',  ( 9.457646018065525792E-16, 20.68750000136559208, 5.148502694627439702 ) ) ;
#48517=CARTESIAN_POINT ( 'NONE',  ( -1.339745962155608039, 22.91965820146970856, -5.000000000000004441 ) ) ;
#48522=CARTESIAN_POINT ( 'NONE',  ( 0.000000000000000000, -170.0000000000000000, 5.000000000000000000 ) ) ;
#48523=CARTESIAN_POINT ( 'NONE',  ( -4.458734124999999437, 0.6041666680322611560, -2.574251347313719407 ) ) ;
#48525=CARTESIAN_POINT ( 'NONE',  ( 2.229367062500001939, -27.22916666530106866, 3.861377020970579999 ) ) ;
#48527=CARTESIAN_POINT ( 'NONE',  ( -3.152801135295367985, -156.8125000013656063, 3.152801135295367096 ) ) ;
#48530=CARTESIAN_POINT ( 'NONE',  ( 4.458734125000001214, 23.10416666803225993, 2.574251347313718519 ) ) ;
#48532=CYLINDRICAL_SURFACE ( 'NONE', #34891, 5.000000000000000000 ) ;
#48534=CARTESIAN_POINT ( 'NONE',  ( -4.458734124999999437, -73.56249999863439371, 0.000000000000000000 ) ) ;
#48537=CARTESIAN_POINT ( 'NONE',  ( -5.000000000000000000, 29.12500000273118417, 0.000000000000000000 ) ) ;
#48538=ORIENTED_EDGE ( 'NONE', *, *, #45606, .T. ) ;
#48539=CARTESIAN_POINT ( 'NONE',  ( -3.535533905932737309, -140.6250000000000000, -3.535533905932738197 ) ) ;
#48541=CARTESIAN_POINT ( 'NONE',  ( 5.000000000000000000, -13.49999999999999822, -6.123233995736766282E-16 ) ) ;
#48542=CARTESIAN_POINT ( 'NONE',  ( -2.229367062500000163, -16.47916666530107577, -3.861377020970580443 ) ) ;
#48543=CARTESIAN_POINT ( 'NONE',  ( 4.458734124999999437, -78.81249999863440792, -5.460374474430324690E-16 ) ) ;
#48544=CARTESIAN_POINT ( 'NONE',  ( 1.846868145590735200, -169.5000000013655495, -4.458734125000000326 ) ) ;
#48545=CARTESIAN_POINT ( 'NONE',  ( -5.000000000000000000, -20.87499999726881228, 0.000000000000000000 ) ) ;
#48546=CARTESIAN_POINT ( 'NONE',  ( -3.152548672688508926E-16, -49.56249999863440792, -5.148502694627439702 ) ) ;
#48547=ORIENTED_EDGE ( 'NONE', *, *, #38231, .F. ) ;
#48549=CARTESIAN_POINT ( 'NONE',  ( -4.458734124999999437, 3.354166668032260823, -2.574251347313719407 ) ) ;
#48552=CARTESIAN_POINT ( 'NONE',  ( 5.000000000000000000, -61.41666666666665719, -2.886751345948129988 ) ) ;
#48553=CARTESIAN_POINT ( 'NONE',  ( -1.846868145590737420, -155.0000000013656063, 4.458734124999999437 ) ) ;
#48556=CARTESIAN_POINT ( 'NONE',  ( -2.071067811865478170, -163.3125000000000000, 5.000000000000000000 ) ) ;
#48557=CARTESIAN_POINT ( 'NONE',  ( 3.535533905932738197, -167.8750000000000284, -3.535533905932738197 ) ) ;
#48559=CARTESIAN_POINT ( 'NONE',  ( -4.458734124999999437, -4.645833331967739177, -2.574251347313719407 ) ) ;
#48560=CARTESIAN_POINT ( 'NONE',  ( 4.458734125000001214, -48.14583333196773651, 2.574251347313718519 ) ) ;
#48561=VECTOR ( 'NONE', #11261, 1000.000000000000000 ) ;
#48562=LINE ( 'NONE', #4502, #4916 ) ;
#48563=CARTESIAN_POINT ( 'NONE',  ( -3.152801135295367985, -147.8125000013655779, 3.152801135295367096 ) ) ;
#48568=CYLINDRICAL_SURFACE ( 'NONE', #58040, 5.000000000000000000 ) ;
#48571=ORIENTED_EDGE ( 'NONE', *, *, #37065, .F. ) ;
#48574=CARTESIAN_POINT ( 'NONE',  ( -6.972266317189433020E-16, 22.74999999999999645, -5.000000000000000000 ) ) ;
#48575=CARTESIAN_POINT ( 'NONE',  ( 9.457646018065525792E-16, -1.062499998634405696, 5.148502694627439702 ) ) ;
#48576=CARTESIAN_POINT ( 'NONE',  ( 0.000000000000000000, -170.0000000000000000, 0.000000000000000000 ) ) ;
#48577=CARTESIAN_POINT ( 'NONE',  ( 4.458734124999997661, -152.5000000013656347, 1.846868145590737864 ) ) ;
#48581=CARTESIAN_POINT ( 'NONE',  ( -2.500000000000000444, -47.16666666666666430, -4.330127018922193649 ) ) ;
#48582=CARTESIAN_POINT ( 'NONE',  ( 5.000000000000000000, -40.49999999999999289, -6.123233995736766282E-16 ) ) ;
#48585=CARTESIAN_POINT ( 'NONE',  ( -6.972266317189433020E-16, -13.25000000000000000, -5.000000000000000000 ) ) ;
#48591=ORIENTED_EDGE ( 'NONE', *, *, #49593, .T. ) ;
#48592=CARTESIAN_POINT ( 'NONE',  ( 2.229367062500001939, 19.02083333469892779, 3.861377020970579999 ) ) ;
#48594=CARTESIAN_POINT ( 'NONE',  ( 2.229367062500001939, -9.229166665301075767, 3.861377020970579999 ) ) ;
#48595=CARTESIAN_POINT ( 'NONE',  ( -1.339745962155610925, -33.66965819600732601, 5.000000000000000000 ) ) ;
#48597=CARTESIAN_POINT ( 'NONE',  ( 3.152801135295367541, -167.3125000013656063, -3.152801135295367541 ) ) ;
#48598=CARTESIAN_POINT ( 'NONE',  ( 2.499999999999998668, -88.33333333333332860, -4.330127018922193649 ) ) ;
#48606=CARTESIAN_POINT ( 'NONE',  ( -4.458734125000000326, -153.1250000013656063, 1.846868145590734089 ) ) ;
#48610=ORIENTED_EDGE ( 'NONE', *, *, #9504, .F. ) ;
#48613=CARTESIAN_POINT ( 'NONE',  ( 5.000000000000000000, 12.58333333333333215, -2.886751345948130876 ) ) ;
#48614=CARTESIAN_POINT ( 'NONE',  ( 5.000000000000000000, 5.583333333333332149, -2.886751345948129988 ) ) ;
#48615=CARTESIAN_POINT ( 'NONE',  ( -2.229367062500000163, -62.47916666530106511, -3.861377020970580443 ) ) ;
#48616=CARTESIAN_POINT ( 'NONE',  ( -2.499999999999996447, 20.16666666666666430, 4.330127018922195425 ) ) ;
#48617=CARTESIAN_POINT ( 'NONE',  ( -2.499999999999996447, -2.708333330602146649, 4.330127018922195425 ) ) ;
#48618=CARTESIAN_POINT ( 'NONE',  ( -2.229367062499996610, -28.14583333196774007, 3.861377020970582219 ) ) ;
#48619=ORIENTED_EDGE ( 'NONE', *, *, #27461, .F. ) ;
#48620=CARTESIAN_POINT ( 'NONE',  ( 2.071067811865264563, -152.9375000027311842, -5.000000000000211386 ) ) ;
#48623=CARTESIAN_POINT ( 'NONE',  ( -2.500000000000000444, -47.16666666666666430, -4.330127018922193649 ) ) ;
#48624=LINE ( 'NONE', #24187, #20298 ) ;
#48627=CARTESIAN_POINT ( 'NONE',  ( -4.458734124999998549, -72.22916666530107932, 2.574251347313722516 ) ) ;
#48628=CARTESIAN_POINT ( 'NONE',  ( -4.458734124999999437, -145.1875000013656063, -5.460374474430324690E-16 ) ) ;
#48629=CARTESIAN_POINT ( 'NONE',  ( 4.458734125000001214, -78.89583333196772230, 2.574251347313718519 ) ) ;
#48630=EDGE_CURVE ( 'NONE', #57060, #46199, #9454, .T. ) ;
#48632=CARTESIAN_POINT ( 'NONE',  ( 2.229367062499998831, -24.89583333196773651, -3.861377020970580887 ) ) ;
#48633=CARTESIAN_POINT ( 'NONE',  ( 1.060575238724906964E-15, -67.62499999726881583, 5.773502691896257311 ) ) ;
#48635=CARTESIAN_POINT ( 'NONE',  ( -5.000000000000000888, -152.6875000027312126, -2.071067811865475949 ) ) ;
#48638=CARTESIAN_POINT ( 'NONE',  ( -6.972266317189433020E-16, 7.875000002731185056, -5.000000000000000000 ) ) ;
#48639=ORIENTED_EDGE ( 'NONE', *, *, #32028, .F. ) ;
#48640=CARTESIAN_POINT ( 'NONE',  ( 2.499999999999998668, 27.66666666666666430, -4.330127018922193649 ) ) ;
#48641=DIRECTION ( 'NONE',  ( 0.000000000000000000, 0.000000000000000000, 1.000000000000000000 ) ) ;
#48642=CARTESIAN_POINT ( 'NONE',  ( -4.458734124999999437, -57.56249999863440081, 0.000000000000000000 ) ) ;
#48644=ORIENTED_EDGE ( 'NONE', *, *, #31908, .F. ) ;
#48645=ADVANCED_FACE ( 'NONE', ( #6280 ), #45502, .T. ) ;
#48646=CARTESIAN_POINT ( 'NONE',  ( -2.500000000000000444, -23.04166666393548013, -4.330127018922193649 ) ) ;
#48647=CARTESIAN_POINT ( 'NONE',  ( -2.229367062499996610, 10.85416666803225993, 3.861377020970582219 ) ) ;
#48649=DIRECTION ( 'NONE',  ( -0.000000000000000000, 1.000000000000000000, -0.000000000000000000 ) ) ;
#48650=CARTESIAN_POINT ( 'NONE',  ( 1.846868145590736310, -165.6250000013656063, 4.458734124999997661 ) ) ;
#48651=ORIENTED_EDGE ( 'NONE', *, *, #36943, .T. ) ;
#48655=AXIS2_PLACEMENT_3D ( 'NONE', #17275, #36899, #12450 ) ;
#48656=CARTESIAN_POINT ( 'NONE',  ( 1.339745962155612702, 4.830341803992664218, -5.000000000000000000 ) ) ;
#48659=CARTESIAN_POINT ( 'NONE',  ( -6.972266317189433020E-16, -20.24999999999999289, -5.000000000000000000 ) ) ;
#48661=CARTESIAN_POINT ( 'NONE',  ( 5.000000000000000888, -18.45833333060214798, 2.886751345948126879 ) ) ;
#48662=DIRECTION ( 'NONE',  ( -0.000000000000000000, 1.000000000000000000, -0.000000000000000000 ) ) ;
#48665=CARTESIAN_POINT ( 'NONE',  ( -2.229367062500000163, 8.270833334698926009, -3.861377020970580443 ) ) ;
#48669=CARTESIAN_POINT ( 'NONE',  ( -5.000000000000000888, -150.5625000027311842, 2.071067811865474617 ) ) ;
#48674=CARTESIAN_POINT ( 'NONE',  ( -9.184850993605147944E-16, -144.2500000000000284, 5.000000000000000000 ) ) ;
#48676=CARTESIAN_POINT ( 'NONE',  ( -8.190561711645485556E-16, -164.9375000013655779, 4.458734124999999437 ) ) ;
#48677=CARTESIAN_POINT ( 'NONE',  ( -4.458734124999997661, -31.22916666530106866, 2.574251347313722516 ) ) ;
#48678=DIRECTION ( 'NONE',  ( 0.000000000000000000, 0.000000000000000000, 1.000000000000000000 ) ) ;
#48681=CARTESIAN_POINT ( 'NONE',  ( -3.152801135295367096, -145.0625000013655779, -3.152801135295367541 ) ) ;
#48682=ORIENTED_EDGE ( 'NONE', *, *, #27618, .F. ) ;
#48683=CARTESIAN_POINT ( 'NONE',  ( 5.000000000000000000, -90.37499999726880162, -6.123233995736766282E-16 ) ) ;
#48684=CARTESIAN_POINT ( 'NONE',  ( 1.975475456537005874E-15, 0.2500000000000001665, 5.000000000000000000 ) ) ;
#48685=CARTESIAN_POINT ( 'NONE',  ( -3.152548672688508926E-16, -56.81249999863440792, -5.148502694627439702 ) ) ;
#48687=CARTESIAN_POINT ( 'NONE',  ( 0.000000000000000000, -170.0000000000000000, 5.000000000000000000 ) ) ;
#48688=CARTESIAN_POINT ( 'NONE',  ( 5.000000000000000888, 21.41666666666666430, 2.886751345948126879 ) ) ;
#48691=CARTESIAN_POINT ( 'NONE',  ( -2.229367062500000163, -5.479166665301072214, -3.861377020970580443 ) ) ;
#48693=CARTESIAN_POINT ( 'NONE',  ( 0.000000000000000000, -170.0000000000000000, 0.000000000000000000 ) ) ;
#48699=CARTESIAN_POINT ( 'NONE',  ( -4.458734124999999437, -55.39583333196773651, -2.574251347313719407 ) ) ;
#48700=CARTESIAN_POINT ( 'NONE',  ( 4.458734124999999437, -154.6875000013656063, 0.000000000000000000 ) ) ;
#48701=ADVANCED_FACE ( 'NONE', ( #28413 ), #27784, .T. ) ;
#48703=CARTESIAN_POINT ( 'NONE',  ( -2.499999999999996447, -48.70833333060213732, 4.330127018922195425 ) ) ;
#48705=CARTESIAN_POINT ( 'NONE',  ( -3.152548672688508926E-16, 4.187500001365595637, -5.148502694627439702 ) ) ;
#48709=CARTESIAN_POINT ( 'NONE',  ( -3.152801135295367985, -161.8125000013656063, 3.152801135295367096 ) ) ;
#48713=CARTESIAN_POINT ( 'NONE',  ( 0.000000000000000000, -170.0000000000000000, 5.000000000000000000 ) ) ;
#48715=CARTESIAN_POINT ( 'NONE',  ( -4.458734124999998549, -45.47916666530105800, 2.574251347313722516 ) ) ;
#48716=ORIENTED_EDGE ( 'NONE', *, *, #46767, .T. ) ;
#48717=CARTESIAN_POINT ( 'NONE',  ( -9.184850993605147944E-16, -143.3750000027312126, 5.000000000000000000 ) ) ;
#48718=EDGE_CURVE ( 'NONE', #18754, #45557, #16040, .T. ) ;
#48720=ORIENTED_EDGE ( 'NONE', *, *, #27801, .F. ) ;
#48722=CARTESIAN_POINT ( 'NONE',  ( -2.229367062500000163, -88.72916666530106511, -3.861377020970580443 ) ) ;
#48725=CARTESIAN_POINT ( 'NONE',  ( -6.972266317189433020E-16, 8.750000000000000000, -5.000000000000000000 ) ) ;
#48728=CARTESIAN_POINT ( 'NONE',  ( 6.123233995736766282E-16, -170.0000000000000000, -5.000000000000000000 ) ) ;
#48731=CARTESIAN_POINT ( 'NONE',  ( 1.975475456537005874E-15, -80.62499999726881583, 5.000000000000000000 ) ) ;
#48732=CARTESIAN_POINT ( 'NONE',  ( -2.500000000000000444, -46.04166666393547303, -4.330127018922193649 ) ) ;
#48733=CARTESIAN_POINT ( 'NONE',  ( -4.458734124999998549, -86.47916666530107932, 2.574251347313722516 ) ) ;
#48736=ORIENTED_EDGE ( 'NONE', *, *, #14608, .T. ) ;
#48738=CARTESIAN_POINT ( 'NONE',  ( 5.000000000000000888, -162.0625000027312126, -2.071067811865475505 ) ) ;
#48740=EDGE_CURVE ( 'NONE', #8603, #15531, #51923, .T. ) ;
#48744=VECTOR ( 'NONE', #56501, 1000.000000000000000 ) ;
#48751=CARTESIAN_POINT ( 'NONE',  ( 4.458734124999998549, -14.72916666530107221, -2.574251347313721627 ) ) ;
#48752=DIRECTION ( 'NONE',  ( -0.000000000000000000, 1.000000000000000000, -0.000000000000000000 ) ) ;
#48753=CARTESIAN_POINT ( 'NONE',  ( -3.535533905932737309, -155.6250000000000000, -3.535533905932738197 ) ) ;
#48755=VERTEX_POINT ( 'NONE', #7864 ) ;
#48756=CARTESIAN_POINT ( 'NONE',  ( 4.458734125000000326, -40.14583333196773651, 2.574251347313718519 ) ) ;
#48757=CARTESIAN_POINT ( 'NONE',  ( 5.000000000000000000, -83.37499999726881583, -6.123233995736766282E-16 ) ) ;
#48762=CARTESIAN_POINT ( 'NONE',  ( 2.229367062500001939, 9.020833334698927786, 3.861377020970579999 ) ) ;
#48764=CARTESIAN_POINT ( 'NONE',  ( 1.975475456537005874E-15, -68.74999999999998579, 5.000000000000000000 ) ) ;
#48766=CARTESIAN_POINT ( 'NONE',  ( 2.229367062500001939, 20.77083333469892779, 3.861377020970579999 ) ) ;
#48768=CARTESIAN_POINT ( 'NONE',  ( 5.000000000000000888, 13.54166666939785202, 2.886751345948126879 ) ) ;
#48772=DIRECTION ( 'NONE',  ( 0.000000000000000000, 0.000000000000000000, 1.000000000000000000 ) ) ;
#48773=CARTESIAN_POINT ( 'NONE',  ( -2.499999999999996447, -34.83333333333332860, 4.330127018922195425 ) ) ;
#48774=CARTESIAN_POINT ( 'NONE',  ( -2.229367062499996610, -36.14583333196773651, 3.861377020970582219 ) ) ;
#48775=( BOUNDED_CURVE ( )  B_SPLINE_CURVE ( 2, ( #56617, #62070, #27952, #62387, #7407, #17983, #17685, #17367, #51468 ),
 .UNSPECIFIED., .F., .F. ) 
 B_SPLINE_CURVE_WITH_KNOTS ( ( 3, 2, 2, 2, 3 ),
 ( 0.8770833333333333259, 0.8777777777777777679, 0.8791666666666666519, 0.8805555555555555358, 0.8812499999999999778 ),
 .UNSPECIFIED. ) 
 CURVE ( )  GEOMETRIC_REPRESENTATION_ITEM ( )  RATIONAL_B_SPLINE_CURVE ( ( 0.9330127018922194093, 0.9330127018922194093, 1.000000000000000000, 0.8660254037844387076, 1.000000000000000000, 0.8660254037844387076, 1.000000000000000000, 0.9330127018922194093, 0.9330127018922194093 ) ) 
 REPRESENTATION_ITEM ( '' )  );
#48777=CARTESIAN_POINT ( 'NONE',  ( -5.000000000000000000, -32.95833333060215153, -2.886751345948128211 ) ) ;
#48778=EDGE_CURVE ( 'NONE', #24820, #25740, #18490, .T. ) ;
#48779=CARTESIAN_POINT ( 'NONE',  ( -2.229367062500000163, -67.47916666530106511, -3.861377020970580443 ) ) ;
#48780=ORIENTED_EDGE ( 'NONE', *, *, #56322, .T. ) ;
#48782=CARTESIAN_POINT ( 'NONE',  ( 4.458734125000001214, -14.89583333196773474, 2.574251347313718519 ) ) ;
#48783=CARTESIAN_POINT ( 'NONE',  ( 4.458734124999999437, -12.06249999863440081, -5.460374474430324690E-16 ) ) ;
#48784=VERTEX_POINT ( 'NONE', #12367 ) ;
#48785=EDGE_CURVE ( 'NONE', #18747, #10208, #59272, .T. ) ;
#48786=CARTESIAN_POINT ( 'NONE',  ( 1.060575238724906964E-15, -83.75000000000000000, 5.773502691896257311 ) ) ;
#48789=CARTESIAN_POINT ( 'NONE',  ( 5.000000000000000888, -84.45833333060214443, 2.886751345948126879 ) ) ;
#48790=FACE_OUTER_BOUND ( 'NONE', #2017, .T. ) ;
#48793=CARTESIAN_POINT ( 'NONE',  ( -4.458734124999999437, -25.56249999863440792, 0.000000000000000000 ) ) ;
#48795=ORIENTED_EDGE ( 'NONE', *, *, #39709, .T. ) ;
#48797=CARTESIAN_POINT ( 'NONE',  ( 3.152801135295366208, -165.8125000013656063, 3.152801135295367985 ) ) ;
#48798=EDGE_CURVE ( 'NONE', #39600, #7768, #28721, .T. ) ;
#48801=ORIENTED_EDGE ( 'NONE', *, *, #54198, .F. ) ;
#48802=EDGE_CURVE ( 'NONE', #38026, #42718, #48344, .T. ) ;
#48806=EDGE_CURVE ( 'NONE', #41613, #21757, #25051, .T. ) ;
#48807=CARTESIAN_POINT ( 'NONE',  ( -4.729367062499999719, -90.71874999795159056, 0.000000000000000000 ) ) ;
#48812=CARTESIAN_POINT ( 'NONE',  ( 1.846868145590736310, -144.8750000013655779, 4.458734124999999437 ) ) ;
#48816=CARTESIAN_POINT ( 'NONE',  ( -2.229367062499996610, -66.39583333196773651, 3.861377020970582219 ) ) ;
#48818=FACE_OUTER_BOUND ( 'NONE', #36945, .T. ) ;
#48819=CARTESIAN_POINT ( 'NONE',  ( 3.152801135295366208, -139.5625000013655779, 3.152801135295367985 ) ) ;
#48821=ORIENTED_EDGE ( 'NONE', *, *, #61491, .T. ) ;
#48822=CARTESIAN_POINT ( 'NONE',  ( 0.000000000000000000, -170.0000000000000000, 5.000000000000000000 ) ) ;
#48823=CARTESIAN_POINT ( 'NONE',  ( 2.071067811865582087, -160.1874999999999716, 4.999999999999894307 ) ) ;
#48828=CARTESIAN_POINT ( 'NONE',  ( 2.229367062500001939, 22.77083333469892423, 3.861377020970579999 ) ) ;
#48829=CARTESIAN_POINT ( 'NONE',  ( -1.339745962155614034, 27.20534180126147916, 4.999999999999999112 ) ) ;
#48834=CARTESIAN_POINT ( 'NONE',  ( 5.000000000000000000, -43.37499999726880873, -6.123233995736766282E-16 ) ) ;
#48835=CARTESIAN_POINT ( 'NONE',  ( 4.458734125000000326, 2.104166668032262599, 2.574251347313718519 ) ) ;
#48837=CARTESIAN_POINT ( 'NONE',  ( -4.458734124999997661, -25.47916666530106866, 2.574251347313722516 ) ) ;
#48841=CARTESIAN_POINT ( 'NONE',  ( -4.458734124999999437, 25.68750000136559208, 0.000000000000000000 ) ) ;
#48842=LINE ( 'NONE', #30500, #8183 ) ;
#48844=CARTESIAN_POINT ( 'NONE',  ( -3.152548672688508926E-16, -72.81249999863439371, -5.148502694627439702 ) ) ;
#48846=DIRECTION ( 'NONE',  ( 0.000000000000000000, 0.000000000000000000, 1.000000000000000000 ) ) ;
#48847=CARTESIAN_POINT ( 'NONE',  ( 3.535533905932736864, -156.2500000027312126, 3.535533905932738641 ) ) ;
#48849=CARTESIAN_POINT ( 'NONE',  ( 6.123233995736766282E-16, -170.0000000000000000, -5.000000000000000000 ) ) ;
#48852=CARTESIAN_POINT ( 'NONE',  ( -2.499999999999996447, -19.83333333333333570, 4.330127018922195425 ) ) ;
#48853=CARTESIAN_POINT ( 'NONE',  ( -4.458734124999998549, -23.22916666530107221, 2.574251347313722516 ) ) ;
#48854=CARTESIAN_POINT ( 'NONE',  ( 4.458734124999999437, -81.81249999863440792, -5.460374474430324690E-16 ) ) ;
#48855=CARTESIAN_POINT ( 'NONE',  ( 1.846868145590736310, -167.8750000013656063, 4.458734124999999437 ) ) ;
#48856=CARTESIAN_POINT ( 'NONE',  ( 5.000000000000000888, -16.45833333060214443, 2.886751345948126879 ) ) ;
#48857=CARTESIAN_POINT ( 'NONE',  ( 2.229367062499998831, -48.64583333196772941, -3.861377020970580887 ) ) ;
#48858=ORIENTED_EDGE ( 'NONE', *, *, #25496, .F. ) ;
#48860=CARTESIAN_POINT ( 'NONE',  ( 4.458734124999998549, 1.020833334698927120, -2.574251347313721627 ) ) ;
#48863=CARTESIAN_POINT ( 'NONE',  ( -5.000000000000000000, -59.08333333333334281, -2.886751345948128211 ) ) ;
#48864=CARTESIAN_POINT ( 'NONE',  ( -1.846868145590734756, -155.3750000013656347, -4.458734125000000326 ) ) ;
#48867=CARTESIAN_POINT ( 'NONE',  ( -3.535533905932738641, -162.3750000000000284, 3.535533905932737309 ) ) ;
#48870=CARTESIAN_POINT ( 'NONE',  ( 4.458734124999999437, -7.062499998634404363, -5.460374474430324690E-16 ) ) ;
#48871=CARTESIAN_POINT ( 'NONE',  ( -2.229367062500000163, -48.72916666530106511, -3.861377020970580443 ) ) ;
#48872=CARTESIAN_POINT ( 'NONE',  ( 5.000000000000000000, -151.1250000027312126, 0.000000000000000000 ) ) ;
#48873=CARTESIAN_POINT ( 'NONE',  ( -3.152801135295367096, -147.0625000013655779, -3.152801135295367541 ) ) ;
#48875=CARTESIAN_POINT ( 'NONE',  ( 2.499999999999998668, 8.666666666666666075, -4.330127018922193649 ) ) ;
#48881=EDGE_CURVE ( 'NONE', #24136, #25000, #46852, .T. ) ;
#48882=CARTESIAN_POINT ( 'NONE',  ( 0.000000000000000000, -170.0000000000000000, 0.000000000000000000 ) ) ;
#48883=EDGE_LOOP ( 'NONE', ( #28477, #2475, #16074, #27278 ) ) ;
#48885=EDGE_CURVE ( 'NONE', #47465, #24820, #22636, .T. ) ;
#48886=DIRECTION ( 'NONE',  ( -0.000000000000000000, 1.000000000000000000, -0.000000000000000000 ) ) ;
#48889=CARTESIAN_POINT ( 'NONE',  ( 2.229367062500001939, -3.979166665301070438, 3.861377020970579999 ) ) ;
#48891=CARTESIAN_POINT ( 'NONE',  ( -1.846868145590737420, -152.7500000013656063, 4.458734124999997661 ) ) ;
#48892=( BOUNDED_CURVE ( )  B_SPLINE_CURVE ( 2, ( #60087, #50101, #6057, #18465, #38086, #8500, #42587, #9122, #23614 ),
 .UNSPECIFIED., .F., .F. ) 
 B_SPLINE_CURVE_WITH_KNOTS ( ( 3, 2, 2, 2, 3 ),
 ( 0.3416666666666669516, 0.3458333333333336035, 0.3500000000000002554, 0.3541666666666669627, 0.3583333333333336146 ),
 .UNSPECIFIED. ) 
 CURVE ( )  GEOMETRIC_REPRESENTATION_ITEM ( )  RATIONAL_B_SPLINE_CURVE ( ( 0.9999999999999948930, 0.9238795325112918455, 1.000000000000000000, 0.9238795325112867385, 1.000000000000000000, 0.9238795325112867385, 1.000000000000000000, 0.9238795325112816315, 1.000000000000005107 ) ) 
 REPRESENTATION_ITEM ( '' )  );
#48894=ORIENTED_EDGE ( 'NONE', *, *, #19331, .T. ) ;
#48896=CARTESIAN_POINT ( 'NONE',  ( -5.000000000000000888, -148.5625000000000000, -2.071067811865475949 ) ) ;
#48897=CARTESIAN_POINT ( 'NONE',  ( 1.975475456537005874E-15, -40.74999999999999289, 5.000000000000000000 ) ) ;
#48899=CARTESIAN_POINT ( 'NONE',  ( -1.339745962155612258, 28.33034180399266333, 5.000000000000000000 ) ) ;
#48900=CARTESIAN_POINT ( 'NONE',  ( 5.000000000000000000, 8.625000002731184168, -6.123233995736766282E-16 ) ) ;
#48905=CARTESIAN_POINT ( 'NONE',  ( 0.000000000000000000, -170.0000000000000000, 5.000000000000000000 ) ) ;
#48906=ORIENTED_EDGE ( 'NONE', *, *, #46960, .F. ) ;
#48907=CARTESIAN_POINT ( 'NONE',  ( 9.457646018065525792E-16, 19.93750000136559208, 5.148502694627439702 ) ) ;
#48909=CARTESIAN_POINT ( 'NONE',  ( -4.458734124999999437, -8.645833331967736513, -2.574251347313719407 ) ) ;
#48910=CARTESIAN_POINT ( 'NONE',  ( -5.000000000000000000, -31.00000000000000000, 0.000000000000000000 ) ) ;
#48912=CARTESIAN_POINT ( 'NONE',  ( -8.190561711645485556E-16, -168.6875000013656063, 4.458734124999999437 ) ) ;
#48913=CARTESIAN_POINT ( 'NONE',  ( -5.000000000000000000, -20.87499999726881228, 0.000000000000000000 ) ) ;
#48916=CARTESIAN_POINT ( 'NONE',  ( -9.184850993605147944E-16, -141.3750000027312126, 5.000000000000000000 ) ) ;
#48919=CARTESIAN_POINT ( 'NONE',  ( 4.458734124999997661, -152.7500000013656063, 1.846868145590737864 ) ) ;
#48922=CYLINDRICAL_SURFACE ( 'NONE', #34542, 5.000000000000000000 ) ;
#48927=CARTESIAN_POINT ( 'NONE',  ( 5.000000000000000000, 2.583333333333333481, -2.886751345948129988 ) ) ;
#48928=CARTESIAN_POINT ( 'NONE',  ( -3.152548672688508926E-16, -65.56249999863440792, -5.148502694627439702 ) ) ;
#48929=EDGE_CURVE ( 'NONE', #43815, #20671, #59903, .T. ) ;
#48931=CARTESIAN_POINT ( 'NONE',  ( -4.999999999999999112, -2.791666663935477466, 2.886751345948131764 ) ) ;
#48932=CARTESIAN_POINT ( 'NONE',  ( -4.458734124999998549, -36.22916666530106511, 2.574251347313722516 ) ) ;
#48933=VERTEX_POINT ( 'NONE', #39007 ) ;
#48934=CARTESIAN_POINT ( 'NONE',  ( 1.975475456537005874E-15, -41.74999999999999289, 5.000000000000000000 ) ) ;
#48935=DIRECTION ( 'NONE',  ( 0.000000000000000000, 0.000000000000000000, 1.000000000000000000 ) ) ;
#48937=CARTESIAN_POINT ( 'NONE',  ( 5.000000000000000000, -46.50000000000000000, -6.123233995736766282E-16 ) ) ;
#48941=CARTESIAN_POINT ( 'NONE',  ( 2.229367062499998831, -67.64583333196773651, -3.861377020970580887 ) ) ;
#48942=CARTESIAN_POINT ( 'NONE',  ( -1.846868145590737420, -145.0000000013656063, 4.458734124999999437 ) ) ;
#48943=CARTESIAN_POINT ( 'NONE',  ( -4.458734124999999437, -84.39583333196773651, -2.574251347313719407 ) ) ;
#48945=CARTESIAN_POINT ( 'NONE',  ( 2.229367062500001939, -32.22916666530106511, 3.861377020970579999 ) ) ;
#48946=CARTESIAN_POINT ( 'NONE',  ( -5.000000000000000000, -72.95833333060214443, -2.886751345948128211 ) ) ;
#48947=ORIENTED_EDGE ( 'NONE', *, *, #46858, .T. ) ;
#48948=CARTESIAN_POINT ( 'NONE',  ( 5.000000000000000000, -51.41666666666666430, -2.886751345948130876 ) ) ;
#48949=VERTEX_POINT ( 'NONE', #58638 ) ;
#48951=CARTESIAN_POINT ( 'NONE',  ( 2.499999999999998668, 28.66666666666666785, -4.330127018922193649 ) ) ;
#48954=CARTESIAN_POINT ( 'NONE',  ( 6.123233995736766282E-16, -170.0000000000000000, -5.000000000000000000 ) ) ;
#48955=CARTESIAN_POINT ( 'NONE',  ( -3.152548672688508926E-16, -57.81249999863440081, -5.148502694627439702 ) ) ;
#48959=CARTESIAN_POINT ( 'NONE',  ( 1.975475456537005874E-15, -22.62499999726880873, 5.000000000000000000 ) ) ;
#48960=CARTESIAN_POINT ( 'NONE',  ( -4.458734124999998549, 14.77083333469892779, 2.574251347313722516 ) ) ;
#48962=CARTESIAN_POINT ( 'NONE',  ( 5.000000000000000000, -27.29166666393548013, -2.886751345948130876 ) ) ;
#48963=CARTESIAN_POINT ( 'NONE',  ( -3.152801135295367096, -166.0625000013656063, -3.152801135295367541 ) ) ;
#48964=AXIS2_PLACEMENT_3D ( 'NONE', #57335, #53120, #32231 ) ;
#48967=CARTESIAN_POINT ( 'NONE',  ( -5.000000000000000000, -153.5000000000000284, -6.123233995736766282E-16 ) ) ;
#48972=DIRECTION ( 'NONE',  ( 0.000000000000000000, 0.000000000000000000, 1.000000000000000000 ) ) ;
#48974=AXIS2_PLACEMENT_3D ( 'NONE', #10310, #5490, #35720 ) ;
#48978=CARTESIAN_POINT ( 'NONE',  ( -6.972266317189433020E-16, -61.25000000000000000, -5.000000000000000000 ) ) ;
#48982=CARTESIAN_POINT ( 'NONE',  ( 4.458734125000000326, 8.854166668032261711, 2.574251347313718519 ) ) ;
#48985=CARTESIAN_POINT ( 'NONE',  ( 2.071067811865476394, -150.3125000027312410, 5.000000000000000000 ) ) ;
#48986=DIRECTION ( 'NONE',  ( -0.000000000000000000, 1.000000000000000000, -0.000000000000000000 ) ) ;
#48987=EDGE_CURVE ( 'NONE', #48784, #47703, #54450, .T. ) ;
#48991=CARTESIAN_POINT ( 'NONE',  ( 2.071067811865475505, -142.8125000000000000, -5.000000000000000888 ) ) ;
#48993=CARTESIAN_POINT ( 'NONE',  ( -8.190561711645485556E-16, -165.9375000013655779, 4.458734124999999437 ) ) ;
#48994=CARTESIAN_POINT ( 'NONE',  ( 4.458734124999999437, -32.81249999863440792, -5.460374474430324690E-16 ) ) ;
#48996=FACE_OUTER_BOUND ( 'NONE', #45032, .T. ) ;
#48998=CARTESIAN_POINT ( 'NONE',  ( -3.152801135295367096, -144.0625000013655779, -3.152801135295367541 ) ) ;
#48999=VERTEX_POINT ( 'NONE', #49620 ) ;
#49000=CARTESIAN_POINT ( 'NONE',  ( 2.229367062500001939, 25.77083333469892779, 3.861377020970579999 ) ) ;
#49002=CARTESIAN_POINT ( 'NONE',  ( 4.458734125000000326, -63.14583333196774362, 2.574251347313718519 ) ) ;
#49005=CARTESIAN_POINT ( 'NONE',  ( -2.499999999999996447, 19.16666666666666430, 4.330127018922195425 ) ) ;
#49006=CARTESIAN_POINT ( 'NONE',  ( -5.000000000000000000, -89.08333333333332860, -2.886751345948128211 ) ) ;
#49007=CARTESIAN_POINT ( 'NONE',  ( 4.458734124999998549, -8.729166665301073991, -2.574251347313721627 ) ) ;
#49008=CARTESIAN_POINT ( 'NONE',  ( -1.339745962155610925, -22.79465819873851729, 5.000000000000000000 ) ) ;
#49012=CARTESIAN_POINT ( 'NONE',  ( 2.499999999999998668, 0.6666666666666660745, -4.330127018922193649 ) ) ;
#49016=CARTESIAN_POINT ( 'NONE',  ( -3.152548672688508926E-16, -53.56249999863439371, -5.148502694627439702 ) ) ;
#49017=CARTESIAN_POINT ( 'NONE',  ( 3.152801135295367541, -157.5625000013656063, -3.152801135295367541 ) ) ;
#49019=VECTOR ( 'NONE', #15533, 1000.000000000000000 ) ;
#49020=CARTESIAN_POINT ( 'NONE',  ( -4.999999999999999112, -48.79166666393547303, 2.886751345948131764 ) ) ;
#49021=VERTEX_POINT ( 'NONE', #6840 ) ;
#49022=AXIS2_PLACEMENT_3D ( 'NONE', #58328, #44472, #14564 ) ;
#49023=CARTESIAN_POINT ( 'NONE',  ( -4.458734124999998549, 3.520833334698929118, 2.574251347313722516 ) ) ;
#49024=ORIENTED_EDGE ( 'NONE', *, *, #59868, .T. ) ;
#49025=( BOUNDED_CURVE ( )  B_SPLINE_CURVE ( 2, ( #14703, #34322, #53947, #5062, #40420, #9877, #29484, #49120, #50400 ),
 .UNSPECIFIED., .F., .F. ) 
 B_SPLINE_CURVE_WITH_KNOTS ( ( 3, 2, 2, 2, 3 ),
 ( 0.7020833333333332815, 0.7027777777777777235, 0.7041666666666667185, 0.7055555555555556024, 0.7062500000000000444 ),
 .UNSPECIFIED. ) 
 CURVE ( )  GEOMETRIC_REPRESENTATION_ITEM ( )  RATIONAL_B_SPLINE_CURVE ( ( 0.9330127018922194093, 0.9330127018922194093, 1.000000000000000000, 0.8660254037844387076, 1.000000000000000000, 0.8660254037844387076, 1.000000000000000000, 0.9330127018922194093, 0.9330127018922194093 ) ) 
 REPRESENTATION_ITEM ( '' )  );
#49028=CARTESIAN_POINT ( 'NONE',  ( 3.152801135295366208, -155.5625000013656063, 3.152801135295367985 ) ) ;
#49032=CARTESIAN_POINT ( 'NONE',  ( -6.972266317189433020E-16, -30.12499999726880873, -5.000000000000000000 ) ) ;
#49033=CARTESIAN_POINT ( 'NONE',  ( -2.229367062500000163, -40.72916666530107221, -3.861377020970580443 ) ) ;
#49037=VERTEX_POINT ( 'NONE', #20994 ) ;
#49038=CARTESIAN_POINT ( 'NONE',  ( 4.458734124999998549, -88.97916666530107932, -2.574251347313721627 ) ) ;
#49042=CARTESIAN_POINT ( 'NONE',  ( 2.500000000000002220, -52.54166666393548013, 4.330127018922192761 ) ) ;
#49044=CARTESIAN_POINT ( 'NONE',  ( -2.499999999999996447, -61.70833333060214443, 4.330127018922195425 ) ) ;
#49049=FACE_OUTER_BOUND ( 'NONE', #37022, .T. ) ;
#49055=AXIS2_PLACEMENT_3D ( 'NONE', #29729, #29091, #5305 ) ;
#49058=CARTESIAN_POINT ( 'NONE',  ( -2.071067811865475061, -159.8125000027312126, -5.000000000000000888 ) ) ;
#49060=ADVANCED_FACE ( 'NONE', ( #31590 ), #21633, .T. ) ;
#49061=VECTOR ( 'NONE', #44409, 1000.000000000000000 ) ;
#49062=CARTESIAN_POINT ( 'NONE',  ( -1.339745962155601378, 21.79465819873851729, -5.000000000000007105 ) ) ;
#49064=FACE_OUTER_BOUND ( 'NONE', #22717, .T. ) ;
#49070=CARTESIAN_POINT ( 'NONE',  ( 0.000000000000000000, -170.0000000000000000, 0.000000000000000000 ) ) ;
#49071=CARTESIAN_POINT ( 'NONE',  ( -3.152548672688508926E-16, -12.56249999863440259, -5.148502694627439702 ) ) ;
#49072=CARTESIAN_POINT ( 'NONE',  ( 2.071067811865476394, -156.1875000000000000, 5.000000000000000000 ) ) ;
#49075=CARTESIAN_POINT ( 'NONE',  ( -2.229367062499996610, -42.39583333196773651, 3.861377020970582219 ) ) ;
#49079=CARTESIAN_POINT ( 'NONE',  ( 0.000000000000000000, -170.0000000000000000, 0.000000000000000000 ) ) ;
#49082=CARTESIAN_POINT ( 'NONE',  ( -4.458734124999999437, 8.687500001365595637, 0.000000000000000000 ) ) ;
#49083=EDGE_CURVE ( 'NONE', #61986, #35368, #61324, .T. ) ;
#49088=CARTESIAN_POINT ( 'NONE',  ( -2.229367062500000163, 23.27083333469892779, -3.861377020970580443 ) ) ;
#49090=CARTESIAN_POINT ( 'NONE',  ( -5.000000000000000000, 14.12500000273118594, 0.000000000000000000 ) ) ;
#49091=ORIENTED_EDGE ( 'NONE', *, *, #37086, .F. ) ;
#49093=ORIENTED_EDGE ( 'NONE', *, *, #18972, .T. ) ;
#49095=CARTESIAN_POINT ( 'NONE',  ( -2.499999999999996447, -35.83333333333332860, 4.330127018922195425 ) ) ;
#49096=CARTESIAN_POINT ( 'NONE',  ( 4.458734124999998549, -37.72916666530107221, -2.574251347313721627 ) ) ;
#49098=CARTESIAN_POINT ( 'NONE',  ( 5.000000000000000000, -34.37499999726881583, -6.123233995736766282E-16 ) ) ;
#49099=CARTESIAN_POINT ( 'NONE',  ( -2.229367062500000163, -63.47916666530106511, -3.861377020970580443 ) ) ;
#49102=CARTESIAN_POINT ( 'NONE',  ( 9.457646018065525792E-16, -13.06249999863440259, 5.148502694627439702 ) ) ;
#49103=CARTESIAN_POINT ( 'NONE',  ( -4.458734124999998549, -13.47916666530107221, 2.574251347313722516 ) ) ;
#49104=VERTEX_POINT ( 'NONE', #26132 ) ;
#49105=CARTESIAN_POINT ( 'NONE',  ( 2.499999999999998668, -81.33333333333332860, -4.330127018922193649 ) ) ;
#49106=CARTESIAN_POINT ( 'NONE',  ( 1.846868145590735200, -167.2500000013655779, -4.458734125000000326 ) ) ;
#49109=CARTESIAN_POINT ( 'NONE',  ( -5.000000000000000000, -82.95833333060213022, -2.886751345948128211 ) ) ;
#49110=CARTESIAN_POINT ( 'NONE',  ( -5.000000000000000000, -48.95833333060213732, -2.886751345948128211 ) ) ;
#49114=CARTESIAN_POINT ( 'NONE',  ( 9.457646018065525792E-16, -26.31249999863440792, 5.148502694627439702 ) ) ;
#49117=CARTESIAN_POINT ( 'NONE',  ( 1.846868145590736310, -165.8750000013656063, 4.458734124999999437 ) ) ;
#49120=CARTESIAN_POINT ( 'NONE',  ( 1.339745962155615144, -55.58034179853028434, 4.999999999999999112 ) ) ;
#49125=CARTESIAN_POINT ( 'NONE',  ( 3.152801135295367541, -144.5625000013655779, -3.152801135295367541 ) ) ;
#49130=ORIENTED_EDGE ( 'NONE', *, *, #61045, .F. ) ;
#49131=CARTESIAN_POINT ( 'NONE',  ( 4.458734125000000326, -140.6250000013656063, -1.846868145590734978 ) ) ;
#49136=CARTESIAN_POINT ( 'NONE',  ( 2.229367062499998831, -73.89583333196773651, -3.861377020970580887 ) ) ;
#49139=CARTESIAN_POINT ( 'NONE',  ( 1.339745962155624914, 14.83034180399266333, -4.999999999999991118 ) ) ;
#49148=CARTESIAN_POINT ( 'NONE',  ( -2.229367062500000163, 21.27083333469892779, -3.861377020970580443 ) ) ;
#49149=DIRECTION ( 'NONE',  ( 0.000000000000000000, 0.000000000000000000, 1.000000000000000000 ) ) ;
#49152=EDGE_CURVE ( 'NONE', #11358, #20646, #46390, .T. ) ;
#49156=CARTESIAN_POINT ( 'NONE',  ( -5.000000000000000000, -50.87499999726881583, 0.000000000000000000 ) ) ;
#49157=CARTESIAN_POINT ( 'NONE',  ( -4.458734124999999437, 3.687500001365594748, 0.000000000000000000 ) ) ;
#49159=CARTESIAN_POINT ( 'NONE',  ( 4.458734125000000326, -24.14583333196774362, 2.574251347313718519 ) ) ;
#49163=AXIS2_PLACEMENT_3D ( 'NONE', #14368, #28534, #43943 ) ;
#49166=CARTESIAN_POINT ( 'NONE',  ( 4.458734125000001214, 24.10416666803226349, 2.574251347313718519 ) ) ;
#49170=CARTESIAN_POINT ( 'NONE',  ( 4.458734125000000326, -72.14583333196773651, 2.574251347313718519 ) ) ;
#49173=CARTESIAN_POINT ( 'NONE',  ( -2.499999999999996447, -10.70833333060214621, 4.330127018922195425 ) ) ;
#49174=VERTEX_POINT ( 'NONE', #52487 ) ;
#49176=CARTESIAN_POINT ( 'NONE',  ( 6.123233995736766282E-16, -170.0000000000000000, -5.000000000000000000 ) ) ;
#49177=CARTESIAN_POINT ( 'NONE',  ( -2.500000000000000444, -17.16666666666666430, -4.330127018922193649 ) ) ;
#49178=CARTESIAN_POINT ( 'NONE',  ( 4.458734125000001214, -20.89583333196774007, 2.574251347313718519 ) ) ;
#49179=CARTESIAN_POINT ( 'NONE',  ( -4.458734124999999437, -85.39583333196773651, -2.574251347313719407 ) ) ;
#49180=VECTOR ( 'NONE', #56788, 1000.000000000000000 ) ;
#49181=( BOUNDED_CURVE ( )  B_SPLINE_CURVE ( 2, ( #51464, #27946, #46952, #21874, #32140, #42736, #12216, #37926, #12842 ),
 .UNSPECIFIED., .F., .F. ) 
 B_SPLINE_CURVE_WITH_KNOTS ( ( 3, 2, 2, 2, 3 ),
 ( 0.8416666666666664520, 0.8458333333333331039, 0.8499999999999997558, 0.8541666666666664076, 0.8583333333333330595 ),
 .UNSPECIFIED. ) 
 CURVE ( )  GEOMETRIC_REPRESENTATION_ITEM ( )  RATIONAL_B_SPLINE_CURVE ( ( 1.000000000000003997, 0.9238795325112826307, 1.000000000000000000, 0.9238795325112867385, 1.000000000000000000, 0.9238795325112867385, 1.000000000000000000, 0.9238795325112908463, 0.9999999999999958922 ) ) 
 REPRESENTATION_ITEM ( '' )  );
#49182=CARTESIAN_POINT ( 'NONE',  ( -4.458734125000000326, -167.2500000013655779, -1.846868145590735644 ) ) ;
#49183=CARTESIAN_POINT ( 'NONE',  ( 2.500000000000002220, -19.54166666393548013, 4.330127018922192761 ) ) ;
#49184=CARTESIAN_POINT ( 'NONE',  ( 9.457646018065525792E-16, -51.06249999863440792, 5.148502694627439702 ) ) ;
#49185=ORIENTED_EDGE ( 'NONE', *, *, #12508, .F. ) ;
#49187=CARTESIAN_POINT ( 'NONE',  ( 2.500000000000002220, -15.54166666393548191, 4.330127018922192761 ) ) ;
#49188=CARTESIAN_POINT ( 'NONE',  ( 4.458734124999998549, -0.9791666653010713262, -2.574251347313721627 ) ) ;
#49189=ORIENTED_EDGE ( 'NONE', *, *, #6344, .T. ) ;
#49191=CARTESIAN_POINT ( 'NONE',  ( 2.500000000000002220, -67.66666666666667140, 4.330127018922192761 ) ) ;
#49192=CARTESIAN_POINT ( 'NONE',  ( -3.152801135295367096, -155.3125000013656063, -3.152801135295367541 ) ) ;
#49194=CARTESIAN_POINT ( 'NONE',  ( -5.000000000000000000, -80.87499999726881583, 0.000000000000000000 ) ) ;
#49195=CARTESIAN_POINT ( 'NONE',  ( 2.071067811865476394, -164.1875000000000000, 5.000000000000000000 ) ) ;
#49198=CARTESIAN_POINT ( 'NONE',  ( -2.229367062500000163, -12.72916666530107044, -3.861377020970580443 ) ) ;
#49199=CARTESIAN_POINT ( 'NONE',  ( 4.458734125000001214, -45.14583333196774362, 2.574251347313718519 ) ) ;
#49200=CARTESIAN_POINT ( 'NONE',  ( 0.000000000000000000, -170.0000000000000000, 0.000000000000000000 ) ) ;
#49201=CARTESIAN_POINT ( 'NONE',  ( 4.458734124999999437, -150.5000000013656347, 1.846868145590737864 ) ) ;
#49204=EDGE_LOOP ( 'NONE', ( #11388, #31724, #18783, #38564 ) ) ;
#49206=CARTESIAN_POINT ( 'NONE',  ( -1.049326080737009628E-13, -5.624999997268816720, 5.000000000000000000 ) ) ;
#49215=CARTESIAN_POINT ( 'NONE',  ( -4.458734124999999437, -1.312499998634406140, 0.000000000000000000 ) ) ;
#49216=CARTESIAN_POINT ( 'NONE',  ( 0.000000000000000000, -170.0000000000000000, 0.000000000000000000 ) ) ;
#49217=CARTESIAN_POINT ( 'NONE',  ( -4.458734125000000326, -148.8750000013655779, 1.846868145590734089 ) ) ;
#49219=ORIENTED_EDGE ( 'NONE', *, *, #62555, .T. ) ;
#49222=CARTESIAN_POINT ( 'NONE',  ( 5.000000000000000888, -12.45833333060214976, 2.886751345948126879 ) ) ;
#49227=EDGE_CURVE ( 'NONE', #3670, #33371, #2531, .T. ) ;
#49229=CARTESIAN_POINT ( 'NONE',  ( 2.499999999999998668, -74.33333333333332860, -4.330127018922193649 ) ) ;
#49231=CARTESIAN_POINT ( 'NONE',  ( 2.499999999999998668, 9.666666666666667851, -4.330127018922193649 ) ) ;
#49232=CARTESIAN_POINT ( 'NONE',  ( 4.458734125000000326, 18.10416666803225993, 2.574251347313718519 ) ) ;
#49234=ORIENTED_EDGE ( 'NONE', *, *, #35006, .F. ) ;
#49235=CARTESIAN_POINT ( 'NONE',  ( -2.229367062500000163, -8.729166665301073991, -3.861377020970580443 ) ) ;
#49238=CARTESIAN_POINT ( 'NONE',  ( 4.458734124999999437, -167.5000000013655779, 1.846868145590737864 ) ) ;
#49239=CARTESIAN_POINT ( 'NONE',  ( 1.339745962155615144, -63.58034179853028434, 4.999999999999999112 ) ) ;
#49245=CARTESIAN_POINT ( 'NONE',  ( -1.339745962155610925, -54.66965819600732601, 5.000000000000000000 ) ) ;
#49246=CARTESIAN_POINT ( 'NONE',  ( 0.000000000000000000, -170.0000000000000000, 0.000000000000000000 ) ) ;
#49247=CARTESIAN_POINT ( 'NONE',  ( -4.458734124999999437, -155.2500000013656063, -1.846868145590735644 ) ) ;
#49251=LINE ( 'NONE', #4548, #49991 ) ;
#49256=DIRECTION ( 'NONE',  ( -0.000000000000000000, 1.000000000000000000, -0.000000000000000000 ) ) ;
#49257=ADVANCED_FACE ( 'NONE', ( #37998 ), #56999, .T. ) ;
#49258=CARTESIAN_POINT ( 'NONE',  ( -5.000000000000000000, -1.000000000000000888, 0.000000000000000000 ) ) ;
#49260=CARTESIAN_POINT ( 'NONE',  ( -2.229367062500000163, -68.47916666530107932, -3.861377020970580443 ) ) ;
#49261=CARTESIAN_POINT ( 'NONE',  ( -6.972266317189433020E-16, -55.12499999726880873, -5.000000000000000000 ) ) ;
#49263=CARTESIAN_POINT ( 'NONE',  ( 5.000000000000000888, -0.4583333306021480369, 2.886751345948126879 ) ) ;
#49264=CARTESIAN_POINT ( 'NONE',  ( 4.458734124999998549, -32.72916666530107221, -2.574251347313721627 ) ) ;
#49265=EDGE_LOOP ( 'NONE', ( #44591, #36624, #16780, #38165 ) ) ;
#49266=CARTESIAN_POINT ( 'NONE',  ( 0.000000000000000000, -170.0000000000000000, 0.000000000000000000 ) ) ;
#49268=ORIENTED_EDGE ( 'NONE', *, *, #5537, .F. ) ;
#49270=CARTESIAN_POINT ( 'NONE',  ( 5.000000000000000000, -51.50000000000000711, -6.123233995736766282E-16 ) ) ;
#49274=CARTESIAN_POINT ( 'NONE',  ( -3.152548672688508926E-16, -71.56249999863440792, -5.148502694627439702 ) ) ;
#49275=CARTESIAN_POINT ( 'NONE',  ( 3.152801135295367541, -145.5625000013655779, -3.152801135295367541 ) ) ;
#49276=CARTESIAN_POINT ( 'NONE',  ( -3.152548672688508926E-16, -81.56249999863440792, -5.148502694627439702 ) ) ;
#49278=CARTESIAN_POINT ( 'NONE',  ( 4.458734124999998549, -28.97916666530107577, -2.574251347313721627 ) ) ;
#49279=CARTESIAN_POINT ( 'NONE',  ( 1.060575238724906964E-15, -71.62499999726880162, 5.773502691896257311 ) ) ;
#49284=VERTEX_POINT ( 'NONE', #56687 ) ;
#49286=( BOUNDED_CURVE ( )  B_SPLINE_CURVE ( 2, ( #62292, #52627, #8874, #18214, #47787, #3745, #23367, #42965, #23677 ),
 .UNSPECIFIED., .F., .F. ) 
 B_SPLINE_CURVE_WITH_KNOTS ( ( 3, 2, 2, 2, 3 ),
 ( 0.5604166666666666741, 0.5611111111111111160, 0.5625000000000000000, 0.5638888888888888840, 0.5645833333333333259 ),
 .UNSPECIFIED. ) 
 CURVE ( )  GEOMETRIC_REPRESENTATION_ITEM ( )  RATIONAL_B_SPLINE_CURVE ( ( 0.9330127018922194093, 0.9330127018922194093, 1.000000000000000000, 0.8660254037844387076, 1.000000000000000000, 0.8660254037844387076, 1.000000000000000000, 0.9330127018922194093, 0.9330127018922194093 ) ) 
 REPRESENTATION_ITEM ( '' )  );
#49288=CARTESIAN_POINT ( 'NONE',  ( 9.457646018065525792E-16, -57.31249999863440081, 5.148502694627439702 ) ) ;
#49292=CARTESIAN_POINT ( 'NONE',  ( 3.061616997868383141E-16, -141.7500000000000284, -5.000000000000000000 ) ) ;
#49293=CARTESIAN_POINT ( 'NONE',  ( -4.458734124999999437, 13.60416666803226349, -2.574251347313719407 ) ) ;
#49295=CARTESIAN_POINT ( 'NONE',  ( 1.339745962155615144, -27.58034179853028789, 4.999999999999999112 ) ) ;
#49296=CARTESIAN_POINT ( 'NONE',  ( -4.458734125000000326, -166.8750000013656063, 1.846868145590734089 ) ) ;
#49297=ORIENTED_EDGE ( 'NONE', *, *, #10253, .F. ) ;
#49299=CARTESIAN_POINT ( 'NONE',  ( 1.975475456537005874E-15, -51.62499999726880873, 5.000000000000000000 ) ) ;
#49302=CARTESIAN_POINT ( 'NONE',  ( 1.975475456537005874E-15, 2.249999999999999556, 5.000000000000000000 ) ) ;
#49305=CARTESIAN_POINT ( 'NONE',  ( 1.975475456537005874E-15, -20.74999999999999645, 5.000000000000000000 ) ) ;
#49310=CARTESIAN_POINT ( 'NONE',  ( -2.229367062500000163, 7.270833334698929562, -3.861377020970580443 ) ) ;
#49313=CARTESIAN_POINT ( 'NONE',  ( 5.000000000000000000, -148.1250000027312126, 0.000000000000000000 ) ) ;
#49318=CARTESIAN_POINT ( 'NONE',  ( -5.000000000000000000, -142.5000000000000284, -6.123233995736766282E-16 ) ) ;
#49321=CARTESIAN_POINT ( 'NONE',  ( -3.152801135295367096, -166.3125000013656063, -3.152801135295367541 ) ) ;
#49322=CARTESIAN_POINT ( 'NONE',  ( -3.152548672688508926E-16, -36.56249999863441502, -5.148502694627439702 ) ) ;
#49324=CYLINDRICAL_SURFACE ( 'NONE', #37976, 5.000000000000000000 ) ;
#49326=CARTESIAN_POINT ( 'NONE',  ( -4.458734125000000326, -142.0000000013655495, -1.846868145590735644 ) ) ;
#49327=ORIENTED_EDGE ( 'NONE', *, *, #7055, .F. ) ;
#49328=CARTESIAN_POINT ( 'NONE',  ( -4.458734124999999437, 29.35416666803225993, -2.574251347313719407 ) ) ;
#49330=CARTESIAN_POINT ( 'NONE',  ( -2.229367062499996610, -64.39583333196773651, 3.861377020970582219 ) ) ;
#49332=CARTESIAN_POINT ( 'NONE',  ( 2.500000000000002220, -90.54166666393547303, 4.330127018922192761 ) ) ;
#49333=CARTESIAN_POINT ( 'NONE',  ( -5.000000000000000000, 12.00000000000000000, 0.000000000000000000 ) ) ;
#49334=CARTESIAN_POINT ( 'NONE',  ( -4.458734124999999437, -53.31249999863439371, 0.000000000000000000 ) ) ;
#49335=CARTESIAN_POINT ( 'NONE',  ( 4.458734124999998549, -5.729166665301072214, -2.574251347313721627 ) ) ;
#49336=CARTESIAN_POINT ( 'NONE',  ( -4.999999999999998224, 4.208333336064518093, 2.886751345948131764 ) ) ;
#49337=CARTESIAN_POINT ( 'NONE',  ( -5.000000000000000000, -9.000000000000001776, 0.000000000000000000 ) ) ;
#49339=CARTESIAN_POINT ( 'NONE',  ( 1.975475456537005874E-15, -66.62499999726881583, 5.000000000000000000 ) ) ;
#49343=CARTESIAN_POINT ( 'NONE',  ( 4.458734125000001214, -55.89583333196773651, 2.574251347313718519 ) ) ;
#49344=CARTESIAN_POINT ( 'NONE',  ( -1.846868145590734756, -155.3750000013656347, -4.458734125000000326 ) ) ;
#49346=CARTESIAN_POINT ( 'NONE',  ( 1.060575238724906964E-15, -54.62499999726880873, 5.773502691896257311 ) ) ;
#49348=CARTESIAN_POINT ( 'NONE',  ( -1.049326080737009628E-13, -4.750000000000003553, 5.000000000000000000 ) ) ;
#49349=CARTESIAN_POINT ( 'NONE',  ( -2.229367062499996610, 4.604166668032261711, 3.861377020970582219 ) ) ;
#49352=CARTESIAN_POINT ( 'NONE',  ( 0.000000000000000000, -170.0000000000000000, 0.000000000000000000 ) ) ;
#49353=CARTESIAN_POINT ( 'NONE',  ( 4.458734124999999437, -156.5000000013656347, 1.846868145590737864 ) ) ;
#49357=CARTESIAN_POINT ( 'NONE',  ( 1.975475456537005874E-15, -80.62499999726881583, 5.000000000000000000 ) ) ;
#49358=CARTESIAN_POINT ( 'NONE',  ( -4.458734124999999437, -42.64583333196773651, -2.574251347313719407 ) ) ;
#49361=CARTESIAN_POINT ( 'NONE',  ( 5.000000000000000888, 9.541666669397852019, 2.886751345948126879 ) ) ;
#49365=CARTESIAN_POINT ( 'NONE',  ( -3.152548672688508926E-16, 29.43750000136559564, -5.148502694627439702 ) ) ;
#49369=CARTESIAN_POINT ( 'NONE',  ( -5.000000000000000000, 23.91666666666666785, -2.886751345948128211 ) ) ;
#49371=CARTESIAN_POINT ( 'NONE',  ( -1.339745962155610925, -61.66965819600733312, 5.000000000000000000 ) ) ;
#49373=CARTESIAN_POINT ( 'NONE',  ( -6.972266317189433020E-16, -33.24999999999999289, -5.000000000000000000 ) ) ;
#49376=CARTESIAN_POINT ( 'NONE',  ( -2.499999999999996447, 5.166666666666666963, 4.330127018922195425 ) ) ;
#49378=DIRECTION ( 'NONE',  ( 0.000000000000000000, 0.000000000000000000, 1.000000000000000000 ) ) ;
#49380=AXIS2_PLACEMENT_3D ( 'NONE', #57953, #13572, #32550 ) ;
#49381=EDGE_CURVE ( 'NONE', #21692, #34622, #37457, .T. ) ;
#49383=EDGE_LOOP ( 'NONE', ( #40336, #49841, #29578, #50395 ) ) ;
#49384=CARTESIAN_POINT ( 'NONE',  ( -2.071067811865391128, -143.8125000027312126, -5.000000000000086153 ) ) ;
#49386=CARTESIAN_POINT ( 'NONE',  ( -2.071067811865478170, -161.4375000027312410, 5.000000000000000000 ) ) ;
#49388=VECTOR ( 'NONE', #39274, 1000.000000000000000 ) ;
#49389=CARTESIAN_POINT ( 'NONE',  ( 5.000000000000000000, -163.1875000027312126, 2.071067811865478614 ) ) ;
#49397=CARTESIAN_POINT ( 'NONE',  ( 0.000000000000000000, -170.0000000000000000, 5.000000000000000000 ) ) ;
#49398=CARTESIAN_POINT ( 'NONE',  ( 4.458734125000000326, -20.89583333196774007, 2.574251347313718519 ) ) ;
#49400=CARTESIAN_POINT ( 'NONE',  ( 3.535533905932738197, -155.8750000000000000, -3.535533905932738197 ) ) ;
#49402=ORIENTED_EDGE ( 'NONE', *, *, #15415, .F. ) ;
#49403=CARTESIAN_POINT ( 'NONE',  ( -4.458734124999999437, -46.64583333196774362, -2.574251347313719407 ) ) ;
#49404=CARTESIAN_POINT ( 'NONE',  ( -5.000000000000000000, 25.91666666666666430, -2.886751345948128211 ) ) ;
#49406=CARTESIAN_POINT ( 'NONE',  ( 5.000000000000000000, 29.50000000000000000, -6.123233995736766282E-16 ) ) ;
#49409=CARTESIAN_POINT ( 'NONE',  ( 9.457646018065525792E-16, 10.93750000136559208, 5.148502694627439702 ) ) ;
#49411=CARTESIAN_POINT ( 'NONE',  ( 2.500000000000002220, -82.66666666666667140, 4.330127018922192761 ) ) ;
#49412=CARTESIAN_POINT ( 'NONE',  ( 2.229367062499998831, 22.10416666803225993, -3.861377020970580887 ) ) ;
#49415=CARTESIAN_POINT ( 'NONE',  ( 2.499999999999998668, 6.791666669397851130, -4.330127018922193649 ) ) ;
#49416=ORIENTED_EDGE ( 'NONE', *, *, #12508, .T. ) ;
#49418=ORIENTED_EDGE ( 'NONE', *, *, #40828, .F. ) ;
#49420=CARTESIAN_POINT ( 'NONE',  ( -4.458734124999999437, -40.39583333196773651, -2.574251347313719407 ) ) ;
#49421=CARTESIAN_POINT ( 'NONE',  ( 1.060575238724906964E-15, -39.62499999726880873, 5.773502691896257311 ) ) ;
#49424=CARTESIAN_POINT ( 'NONE',  ( -4.458734124999999437, -14.31249999863440436, 0.000000000000000000 ) ) ;
#49425=CARTESIAN_POINT ( 'NONE',  ( -4.458734124999999437, -12.64583333196774007, -2.574251347313719407 ) ) ;
#49426=ORIENTED_EDGE ( 'NONE', *, *, #2713, .T. ) ;
#49427=CARTESIAN_POINT ( 'NONE',  ( 5.000000000000000888, -82.58333333333332860, 2.886751345948126879 ) ) ;
#49428=CARTESIAN_POINT ( 'NONE',  ( -6.972266317189433020E-16, 0.8750000027311866102, -5.000000000000000000 ) ) ;
#49430=CARTESIAN_POINT ( 'NONE',  ( 5.000000000000000888, -82.45833333060214443, 2.886751345948126879 ) ) ;
#49432=EDGE_LOOP ( 'NONE', ( #6518, #28466, #22792, #51607 ) ) ;
#49433=AXIS2_PLACEMENT_3D ( 'NONE', #4561, #38653, #23876 ) ;
#49436=CARTESIAN_POINT ( 'NONE',  ( -4.458734124999999437, -29.56249999863440436, 0.000000000000000000 ) ) ;
#49438=EDGE_LOOP ( 'NONE', ( #8472, #46838, #4532, #3625 ) ) ;
#49440=CARTESIAN_POINT ( 'NONE',  ( 4.458734124999999437, -163.6875000013655779, 0.000000000000000000 ) ) ;
#49442=CARTESIAN_POINT ( 'NONE',  ( 2.071067811865560326, -147.8125000000000000, -4.999999999999914735 ) ) ;
#49443=ORIENTED_EDGE ( 'NONE', *, *, #6409, .T. ) ;
#49445=CARTESIAN_POINT ( 'NONE',  ( -4.458734124999999437, -73.56249999863439371, 0.000000000000000000 ) ) ;
#49448=CARTESIAN_POINT ( 'NONE',  ( 4.458734124999999437, -145.6250000013655779, -1.846868145590734978 ) ) ;
#49450=CARTESIAN_POINT ( 'NONE',  ( -1.339745962155613146, 28.20534180126148271, 5.000000000000000000 ) ) ;
#49454=EDGE_CURVE ( 'NONE', #4902, #20671, #63394, .T. ) ;
#49457=EDGE_CURVE ( 'NONE', #13616, #43111, #58561, .T. ) ;
#49459=CARTESIAN_POINT ( 'NONE',  ( -6.972266317189433020E-16, 25.74999999999999645, -5.000000000000000000 ) ) ;
#49461=CARTESIAN_POINT ( 'NONE',  ( -4.458734124999998549, -75.47916666530107932, 2.574251347313722516 ) ) ;
#49463=CARTESIAN_POINT ( 'NONE',  ( 1.975475456537005874E-15, -68.74999999999998579, 5.000000000000000000 ) ) ;
#49466=ORIENTED_EDGE ( 'NONE', *, *, #24133, .F. ) ;
#49473=CARTESIAN_POINT ( 'NONE',  ( 2.229367062499998831, 17.10416666803225993, -3.861377020970580887 ) ) ;
#49474=CARTESIAN_POINT ( 'NONE',  ( -5.000000000000000000, 23.12500000273118417, 0.000000000000000000 ) ) ;
#49481=CARTESIAN_POINT ( 'NONE',  ( 2.229367062499998831, 3.354166668032259935, -3.861377020970580887 ) ) ;
#49483=CARTESIAN_POINT ( 'NONE',  ( 4.458734124999998549, -28.97916666530108287, -2.574251347313721627 ) ) ;
#49486=CARTESIAN_POINT ( 'NONE',  ( -2.229367062499996610, 23.85416666803225993, 3.861377020970582219 ) ) ;
#49488=DIRECTION ( 'NONE',  ( -0.000000000000000000, 1.000000000000000000, -0.000000000000000000 ) ) ;
#49489=CARTESIAN_POINT ( 'NONE',  ( 4.458734124999999437, -74.06249999863440792, -5.460374474430324690E-16 ) ) ;
#49492=CARTESIAN_POINT ( 'NONE',  ( 5.000000000000000888, 23.54166666939785202, 2.886751345948126879 ) ) ;
#49493=EDGE_LOOP ( 'NONE', ( #36011, #15338, #48538, #61883 ) ) ;
#49494=CARTESIAN_POINT ( 'NONE',  ( -5.000000000000000888, -140.4375000000000000, 2.071067811865474617 ) ) ;
#49496=CARTESIAN_POINT ( 'NONE',  ( 2.499999999999998668, -20.33333333333333570, -4.330127018922193649 ) ) ;
#49497=CARTESIAN_POINT ( 'NONE',  ( 2.229367062499998831, -21.64583333196774007, -3.861377020970580887 ) ) ;
#49498=CARTESIAN_POINT ( 'NONE',  ( 9.457646018065525792E-16, -81.06249999863440792, 5.148502694627439702 ) ) ;
#49499=CARTESIAN_POINT ( 'NONE',  ( 5.000000000000000888, -20.45833333060214798, 2.886751345948126879 ) ) ;
#49500=CARTESIAN_POINT ( 'NONE',  ( -3.152548672688508926E-16, -48.56249999863440792, -5.148502694627439702 ) ) ;
#49502=CARTESIAN_POINT ( 'NONE',  ( 1.339745962155615144, -70.58034179853028434, 4.999999999999999112 ) ) ;
#49504=CARTESIAN_POINT ( 'NONE',  ( 2.229367062499998831, 0.1041666680322607397, -3.861377020970580887 ) ) ;
#49507=CARTESIAN_POINT ( 'NONE',  ( -5.000000000000000000, -68.08333333333332860, -2.886751345948128211 ) ) ;
#49508=CARTESIAN_POINT ( 'NONE',  ( -1.846868145590737420, -153.0000000013656063, 4.458734124999999437 ) ) ;
#49511=CARTESIAN_POINT ( 'NONE',  ( 3.535533905932736864, -162.1250000000000284, 3.535533905932738641 ) ) ;
#49515=CARTESIAN_POINT ( 'NONE',  ( 4.458734125000001214, -10.14583333196773829, 2.574251347313718519 ) ) ;
#49516=CARTESIAN_POINT ( 'NONE',  ( -2.229367062500000163, -43.72916666530106511, -3.861377020970580443 ) ) ;
#49517=CARTESIAN_POINT ( 'NONE',  ( 0.000000000000000000, -170.0000000000000000, 0.000000000000000000 ) ) ;
#49518=CARTESIAN_POINT ( 'NONE',  ( 4.458734125000000326, -146.3750000013655779, -1.846868145590734978 ) ) ;
#49520=DIRECTION ( 'NONE',  ( -0.000000000000000000, 1.000000000000000000, -0.000000000000000000 ) ) ;
#49521=VERTEX_POINT ( 'NONE', #38312 ) ;
#49522=FACE_OUTER_BOUND ( 'NONE', #42388, .T. ) ;
#49523=CARTESIAN_POINT ( 'NONE',  ( -3.152548672688508926E-16, 29.18750000136559208, -5.148502694627439702 ) ) ;
#49530=EDGE_CURVE ( 'NONE', #1448, #26085, #4951, .T. ) ;
#49531=CARTESIAN_POINT ( 'NONE',  ( 2.499999999999998668, 11.79166666939785202, -4.330127018922193649 ) ) ;
#49532=CARTESIAN_POINT ( 'NONE',  ( 9.457646018065525792E-16, -5.062499998634401699, 5.148502694627439702 ) ) ;
#49534=CARTESIAN_POINT ( 'NONE',  ( 4.458734124999999437, -148.3750000013655779, -1.846868145590734978 ) ) ;
#49536=ORIENTED_EDGE ( 'NONE', *, *, #25677, .T. ) ;
#49538=CARTESIAN_POINT ( 'NONE',  ( -5.000000000000000000, -148.5000000000000284, -6.123233995736766282E-16 ) ) ;
#49549=CARTESIAN_POINT ( 'NONE',  ( -2.229367062499996610, 19.85416666803225993, 3.861377020970582219 ) ) ;
#49552=CARTESIAN_POINT ( 'NONE',  ( -4.458734124999999437, -10.56249999863440792, 0.000000000000000000 ) ) ;
#49554=CARTESIAN_POINT ( 'NONE',  ( -1.846868145590737420, -165.7500000013655495, 4.458734124999999437 ) ) ;
#49562=LINE ( 'NONE', #5821, #62510 ) ;
#49563=CARTESIAN_POINT ( 'NONE',  ( 1.975475456537005874E-15, -88.62499999726880162, 5.000000000000000000 ) ) ;
#49564=CARTESIAN_POINT ( 'NONE',  ( -4.458734124999999437, -153.2500000013656063, -1.846868145590735644 ) ) ;
#49571=CARTESIAN_POINT ( 'NONE',  ( 1.060575238724906964E-15, -1.750000000000001554, 5.773502691896257311 ) ) ;
#49572=CARTESIAN_POINT ( 'NONE',  ( -2.229367062499996610, -67.14583333196773651, 3.861377020970582219 ) ) ;
#49573=FACE_OUTER_BOUND ( 'NONE', #27051, .T. ) ;
#49574=CARTESIAN_POINT ( 'NONE',  ( -5.000000000000000000, -3.958333330602147537, -2.886751345948128211 ) ) ;
#49575=CARTESIAN_POINT ( 'NONE',  ( -2.229367062499996610, -33.14583333196772941, 3.861377020970582219 ) ) ;
#49576=ORIENTED_EDGE ( 'NONE', *, *, #8291, .T. ) ;
#49577=CARTESIAN_POINT ( 'NONE',  ( -2.499999999999996447, -77.83333333333334281, 4.330127018922195425 ) ) ;
#49579=ORIENTED_EDGE ( 'NONE', *, *, #27140, .F. ) ;
#49581=CARTESIAN_POINT ( 'NONE',  ( -5.000000000000000000, -48.08333333333332860, -2.886751345948128211 ) ) ;
#49584=CARTESIAN_POINT ( 'NONE',  ( 5.000000000000000000, -4.416666666666666075, -2.886751345948130876 ) ) ;
#49585=CARTESIAN_POINT ( 'NONE',  ( -4.458734124999999437, -70.31249999863439371, 0.000000000000000000 ) ) ;
#49586=CARTESIAN_POINT ( 'NONE',  ( -1.846868145590734756, -142.3750000013656063, -4.458734125000000326 ) ) ;
#49587=CARTESIAN_POINT ( 'NONE',  ( 4.458734125000001214, -79.89583333196773651, 2.574251347313718519 ) ) ;
#49589=CARTESIAN_POINT ( 'NONE',  ( 2.229367062499998831, -31.89583333196773651, -3.861377020970580887 ) ) ;
#49590=CARTESIAN_POINT ( 'NONE',  ( 5.000000000000000000, -72.37499999726880162, -6.123233995736766282E-16 ) ) ;
#49593=EDGE_CURVE ( 'NONE', #47703, #2151, #13604, .T. ) ;
#49595=ORIENTED_EDGE ( 'NONE', *, *, #6689, .T. ) ;
#49598=EDGE_CURVE ( 'NONE', #7443, #25868, #13220, .T. ) ;
#49601=CARTESIAN_POINT ( 'NONE',  ( -4.999999999999998224, -75.79166666393547303, 2.886751345948131764 ) ) ;
#49602=CARTESIAN_POINT ( 'NONE',  ( 4.458734124999999437, -59.06249999863440081, -5.460374474430324690E-16 ) ) ;
#49603=EDGE_CURVE ( 'NONE', #45427, #2557, #59522, .T. ) ;
#49606=EDGE_CURVE ( 'NONE', #27699, #39231, #15659, .T. ) ;
#49608=DIRECTION ( 'NONE',  ( 0.000000000000000000, 0.000000000000000000, 1.000000000000000000 ) ) ;
#49610=CARTESIAN_POINT ( 'NONE',  ( -3.152548672688508926E-16, 11.43750000136559386, -5.148502694627439702 ) ) ;
#49612=CARTESIAN_POINT ( 'NONE',  ( -2.499999999999996447, -0.8333333333333317050, 4.330127018922195425 ) ) ;
#49613=CARTESIAN_POINT ( 'NONE',  ( -1.846868145590737420, -160.7500000013655779, 4.458734124999997661 ) ) ;
#49619=ADVANCED_FACE ( 'NONE', ( #25415 ), #45033, .T. ) ;
#49620=CARTESIAN_POINT ( 'NONE',  ( 6.123233995736766282E-16, 30.00000000000000000, -5.000000000000000000 ) ) ;
#49623=CARTESIAN_POINT ( 'NONE',  ( 0.000000000000000000, -170.0000000000000000, 0.000000000000000000 ) ) ;
#49626=CARTESIAN_POINT ( 'NONE',  ( -2.499999999999996447, -20.83333333333333570, 4.330127018922195425 ) ) ;
#49629=LINE ( 'NONE', #30316, #47873 ) ;
#49632=CARTESIAN_POINT ( 'NONE',  ( -4.458734124999997661, 7.520833334698926009, 2.574251347313722516 ) ) ;
#49634=CARTESIAN_POINT ( 'NONE',  ( 5.000000000000000888, -150.0625000027312126, -2.071067811865475505 ) ) ;
#49639=CARTESIAN_POINT ( 'NONE',  ( 0.000000000000000000, -170.0000000000000000, 0.000000000000000000 ) ) ;
#49642=CARTESIAN_POINT ( 'NONE',  ( 2.730187237215162345E-16, -166.4375000013655779, -4.458734124999999437 ) ) ;
#49643=CARTESIAN_POINT ( 'NONE',  ( -3.535533905932738641, -160.3750000000000284, 3.535533905932737309 ) ) ;
#49644=CARTESIAN_POINT ( 'NONE',  ( 2.499999999999998668, -45.20833333060214443, -4.330127018922193649 ) ) ;
#49646=CARTESIAN_POINT ( 'NONE',  ( -4.458734125000001214, -142.8750000013656063, 1.846868145590734089 ) ) ;
#49647=ORIENTED_EDGE ( 'NONE', *, *, #51601, .F. ) ;
#49648=CARTESIAN_POINT ( 'NONE',  ( 2.229367062500001939, 27.77083333469892779, 3.861377020970579999 ) ) ;
#49650=CARTESIAN_POINT ( 'NONE',  ( -3.152548672688508926E-16, -60.81249999863440081, -5.148502694627439702 ) ) ;
#49653=CARTESIAN_POINT ( 'NONE',  ( 0.000000000000000000, -170.0000000000000000, 0.000000000000000000 ) ) ;
#49654=CARTESIAN_POINT ( 'NONE',  ( -2.499999999999996447, 12.16666666666666607, 4.330127018922195425 ) ) ;
#49655=CARTESIAN_POINT ( 'NONE',  ( -4.458734124999999437, -50.39583333196772941, -2.574251347313719407 ) ) ;
#49656=CARTESIAN_POINT ( 'NONE',  ( 4.458734124999999437, -13.81249999863440259, -5.460374474430324690E-16 ) ) ;
#49657=CARTESIAN_POINT ( 'NONE',  ( 5.000000000000000888, -166.0625000027312410, -2.071067811865475505 ) ) ;
#49658=DIRECTION ( 'NONE',  ( -0.000000000000000000, 1.000000000000000000, -0.000000000000000000 ) ) ;
#49660=CARTESIAN_POINT ( 'NONE',  ( 5.000000000000000000, -167.0624999999999716, 2.071067811865478614 ) ) ;
#49661=CARTESIAN_POINT ( 'NONE',  ( 2.626220312808019583E-14, 20.87500000273118062, -5.000000000000000000 ) ) ;
#49662=CARTESIAN_POINT ( 'NONE',  ( 0.000000000000000000, -170.0000000000000000, 5.000000000000000000 ) ) ;
#49665=CARTESIAN_POINT ( 'NONE',  ( -4.458734124999998549, -55.22916666530107932, 2.574251347313722516 ) ) ;
#49666=CARTESIAN_POINT ( 'NONE',  ( -3.152801135295367985, -156.0625000013656063, 3.152801135295367096 ) ) ;
#49667=CARTESIAN_POINT ( 'NONE',  ( -3.535250795749689387E-16, -55.12499999726880162, -5.773502691896257311 ) ) ;
#49670=CARTESIAN_POINT ( 'NONE',  ( 2.229367062500001939, 5.770833334698927786, 3.861377020970579999 ) ) ;
#49674=CARTESIAN_POINT ( 'NONE',  ( -3.152801135295367096, -155.0625000013656063, -3.152801135295367541 ) ) ;
#49676=CARTESIAN_POINT ( 'NONE',  ( 1.975475456537005874E-15, -87.62499999726880162, 5.000000000000000000 ) ) ;
#49679=CARTESIAN_POINT ( 'NONE',  ( 4.458734125000001214, -44.14583333196773651, 2.574251347313718519 ) ) ;
#49681=CARTESIAN_POINT ( 'NONE',  ( 3.535533905932736864, -143.2500000027311842, 3.535533905932738641 ) ) ;
#49684=CARTESIAN_POINT ( 'NONE',  ( -2.229367062499996610, 27.85416666803225993, 3.861377020970582219 ) ) ;
#49687=CARTESIAN_POINT ( 'NONE',  ( 1.255007937094098239E-14, 23.75000000000000000, -4.999999999999999112 ) ) ;
#49691=FACE_OUTER_BOUND ( 'NONE', #27570, .T. ) ;
#49692=EDGE_CURVE ( 'NONE', #40265, #61986, #44007, .T. ) ;
#49696=CYLINDRICAL_SURFACE ( 'NONE', #31701, 5.000000000000000000 ) ;
#49698=CARTESIAN_POINT ( 'NONE',  ( 5.275681513340003914E-14, 10.87500000273118239, -5.000000000000000000 ) ) ;
#49701=CARTESIAN_POINT ( 'NONE',  ( -2.071067811865477726, -169.6875000000000284, -4.999999999999996447 ) ) ;
#49703=CARTESIAN_POINT ( 'NONE',  ( -3.535533905932737309, -159.7500000027312126, -3.535533905932738197 ) ) ;
#49706=CARTESIAN_POINT ( 'NONE',  ( -9.184850993605147944E-16, -163.3750000027311842, 5.000000000000000000 ) ) ;
#49714=CARTESIAN_POINT ( 'NONE',  ( -3.535533905932738641, -141.5000000027311842, 3.535533905932737309 ) ) ;
#49715=CARTESIAN_POINT ( 'NONE',  ( 4.458734124999999437, -21.81249999863440436, -5.460374474430324690E-16 ) ) ;
#49717=CARTESIAN_POINT ( 'NONE',  ( -3.535533905932738641, -156.3750000000000000, 3.535533905932737309 ) ) ;
#49719=CARTESIAN_POINT ( 'NONE',  ( -4.458734125000000326, -156.0000000013656063, -1.846868145590735644 ) ) ;
#49720=ORIENTED_EDGE ( 'NONE', *, *, #32028, .T. ) ;
#49721=CARTESIAN_POINT ( 'NONE',  ( 9.457646018065525792E-16, -47.31249999863440792, 5.148502694627439702 ) ) ;
#49724=CARTESIAN_POINT ( 'NONE',  ( -2.499999999999996447, 28.16666666666666785, 4.330127018922195425 ) ) ;
#49726=VECTOR ( 'NONE', #6992, 1000.000000000000000 ) ;
#49727=CARTESIAN_POINT ( 'NONE',  ( -4.458734124999999437, 9.604166668032259935, -2.574251347313719407 ) ) ;
#49729=CARTESIAN_POINT ( 'NONE',  ( 1.339745962155612702, -37.16965819600733312, -5.000000000000000000 ) ) ;
#49731=CARTESIAN_POINT ( 'NONE',  ( 9.457646018065525792E-16, 22.68750000136559564, 5.148502694627439702 ) ) ;
#49733=CARTESIAN_POINT ( 'NONE',  ( 2.499999999999998668, 9.791666669397850242, -4.330127018922193649 ) ) ;
#49738=CARTESIAN_POINT ( 'NONE',  ( -2.229367062500000163, -39.47916666530107221, -3.861377020970580443 ) ) ;
#49739=( BOUNDED_CURVE ( )  B_SPLINE_CURVE ( 2, ( #36993, #46961, #60489, #36035, #60806, #2277, #41477, #55667, #61128 ),
 .UNSPECIFIED., .F., .F. ) 
 B_SPLINE_CURVE_WITH_KNOTS ( ( 3, 2, 2, 2, 3 ),
 ( 0.6249999999999996669, 0.6291666666666663188, 0.6333333333333328596, 0.6374999999999995115, 0.6416666666666662744 ),
 .UNSPECIFIED. ) 
 CURVE ( )  GEOMETRIC_REPRESENTATION_ITEM ( )  RATIONAL_B_SPLINE_CURVE ( ( 1.000000000000005995, 0.9238795325112806323, 1.000000000000000000, 0.9238795325112867385, 1.000000000000000000, 0.9238795325112867385, 1.000000000000000000, 0.9238795325112948431, 0.9999999999999918954 ) ) 
 REPRESENTATION_ITEM ( '' )  );
#49740=CARTESIAN_POINT ( 'NONE',  ( 2.499999999999998668, -40.20833333060214443, -4.330127018922193649 ) ) ;
#49742=CARTESIAN_POINT ( 'NONE',  ( 2.229367062500001939, -10.97916666530107044, 3.861377020970579999 ) ) ;
#49743=CARTESIAN_POINT ( 'NONE',  ( -4.458734124999998549, -18.47916666530106866, 2.574251347313722516 ) ) ;
#49745=CARTESIAN_POINT ( 'NONE',  ( -2.499999999999996447, -84.83333333333332860, 4.330127018922195425 ) ) ;
#49746=CARTESIAN_POINT ( 'NONE',  ( 3.152801135295367541, -167.3125000013656063, -3.152801135295367541 ) ) ;
#49748=CARTESIAN_POINT ( 'NONE',  ( 1.060575238724906964E-15, -85.62499999726880162, 5.773502691896257311 ) ) ;
#49749=CARTESIAN_POINT ( 'NONE',  ( -6.972266317189433020E-16, -28.25000000000000000, -5.000000000000000000 ) ) ;
#49752=CARTESIAN_POINT ( 'NONE',  ( -4.458734124999999437, -27.64583333196774007, -2.574251347313719407 ) ) ;
#49753=CARTESIAN_POINT ( 'NONE',  ( 2.500000000000002220, -5.541666663935480130, 4.330127018922192761 ) ) ;
#49754=VERTEX_POINT ( 'NONE', #46312 ) ;
#49755=CARTESIAN_POINT ( 'NONE',  ( 4.458734124999999437, -162.7500000013655779, 1.846868145590737864 ) ) ;
#49757=CARTESIAN_POINT ( 'NONE',  ( 2.071067811865645591, -156.1875000000000000, 4.999999999999830358 ) ) ;
#49760=CARTESIAN_POINT ( 'NONE',  ( -2.229367062499996610, -75.39583333196773651, 3.861377020970582219 ) ) ;
#49763=CARTESIAN_POINT ( 'NONE',  ( -3.152801135295367985, -146.0625000013655779, 3.152801135295367096 ) ) ;
#49766=CARTESIAN_POINT ( 'NONE',  ( -1.339745962155613812, -0.2053418012614791066, -5.000000000000000000 ) ) ;
#49769=CARTESIAN_POINT ( 'NONE',  ( -4.458734124999999437, -141.1875000013656063, -5.460374474430324690E-16 ) ) ;
#49772=CARTESIAN_POINT ( 'NONE',  ( -2.499999999999996447, -52.83333333333332860, 4.330127018922195425 ) ) ;
#49774=CARTESIAN_POINT ( 'NONE',  ( 4.458734124999998549, -73.97916666530106511, -2.574251347313721627 ) ) ;
#49775=CARTESIAN_POINT ( 'NONE',  ( 1.339745962155612702, -34.29465819873851729, -5.000000000000000000 ) ) ;
#49776=CARTESIAN_POINT ( 'NONE',  ( -5.000000000000000000, -70.08333333333332860, -2.886751345948128211 ) ) ;
#49780=CARTESIAN_POINT ( 'NONE',  ( 6.123233995736766282E-16, -170.0000000000000000, -5.000000000000000000 ) ) ;
#49786=CARTESIAN_POINT ( 'NONE',  ( 9.457646018065525792E-16, 17.68750000136559208, 5.148502694627439702 ) ) ;
#49794=CARTESIAN_POINT ( 'NONE',  ( -4.458734124999997661, -6.229166665301072214, 2.574251347313722516 ) ) ;
#49795=CARTESIAN_POINT ( 'NONE',  ( 2.229367062499998831, -28.89583333196774007, -3.861377020970580887 ) ) ;
#49796=( BOUNDED_CURVE ( )  B_SPLINE_CURVE ( 2, ( #54814, #1756, #1439, #21041, #20073, #39679, #21358, #11060, #30035 ),
 .UNSPECIFIED., .F., .F. ) 
 B_SPLINE_CURVE_WITH_KNOTS ( ( 3, 2, 2, 2, 3 ),
 ( 0.5062499999999999778, 0.5069444444444444198, 0.5083333333333333037, 0.5097222222222221877, 0.5104166666666666297 ),
 .UNSPECIFIED. ) 
 CURVE ( )  GEOMETRIC_REPRESENTATION_ITEM ( )  RATIONAL_B_SPLINE_CURVE ( ( 0.9330127018922194093, 0.9330127018922194093, 1.000000000000000000, 0.8660254037844387076, 1.000000000000000000, 0.8660254037844387076, 1.000000000000000000, 0.9330127018922194093, 0.9330127018922194093 ) ) 
 REPRESENTATION_ITEM ( '' )  );
#49801=CARTESIAN_POINT ( 'NONE',  ( 4.458734124999998549, 28.27083333469892779, -2.574251347313721627 ) ) ;
#49802=CARTESIAN_POINT ( 'NONE',  ( 2.500000000000002220, 26.45833333606451632, 4.330127018922192761 ) ) ;
#49803=CARTESIAN_POINT ( 'NONE',  ( -4.458734124999999437, -80.64583333196773651, -2.574251347313719407 ) ) ;
#49806=CARTESIAN_POINT ( 'NONE',  ( 5.000000000000000000, 23.62500000273118417, -6.123233995736766282E-16 ) ) ;
#49809=CARTESIAN_POINT ( 'NONE',  ( -5.000000000000000000, -56.87499999726880162, 0.000000000000000000 ) ) ;
#49810=CARTESIAN_POINT ( 'NONE',  ( -4.999999999999999112, -15.91666666666666963, 2.886751345948131764 ) ) ;
#49811=CARTESIAN_POINT ( 'NONE',  ( -2.229367062500000163, -22.47916666530107221, -3.861377020970580443 ) ) ;
#49812=CARTESIAN_POINT ( 'NONE',  ( 2.229367062499998831, -83.64583333196773651, -3.861377020970580887 ) ) ;
#49813=CARTESIAN_POINT ( 'NONE',  ( -3.535250795749689387E-16, -24.12499999726881583, -5.773502691896257311 ) ) ;
#49814=CARTESIAN_POINT ( 'NONE',  ( -4.458734124999998549, -48.22916666530106511, 2.574251347313722516 ) ) ;
#49815=EDGE_LOOP ( 'NONE', ( #12592, #26796, #59002, #4549 ) ) ;
#49817=FACE_OUTER_BOUND ( 'NONE', #43700, .T. ) ;
#49818=CARTESIAN_POINT ( 'NONE',  ( -2.229367062500000163, 3.270833334698929118, -3.861377020970580443 ) ) ;
#49819=VERTEX_POINT ( 'NONE', #42420 ) ;
#49820=( BOUNDED_CURVE ( )  B_SPLINE_CURVE ( 2, ( #45463, #60907, #46101, #25526, #50609, #20716, #25846, #11360, #59635 ),
 .UNSPECIFIED., .F., .F. ) 
 B_SPLINE_CURVE_WITH_KNOTS ( ( 3, 2, 2, 2, 3 ),
 ( 0.2270833333333333315, 0.2277777777777777735, 0.2291666666666666574, 0.2305555555555555691, 0.2312500000000000111 ),
 .UNSPECIFIED. ) 
 CURVE ( )  GEOMETRIC_REPRESENTATION_ITEM ( )  RATIONAL_B_SPLINE_CURVE ( ( 0.9330127018922194093, 0.9330127018922194093, 1.000000000000000000, 0.8660254037844387076, 1.000000000000000000, 0.8660254037844387076, 1.000000000000000000, 0.9330127018922194093, 0.9330127018922194093 ) ) 
 REPRESENTATION_ITEM ( '' )  );
#49822=CARTESIAN_POINT ( 'NONE',  ( -5.000000000000000000, -65.08333333333332860, -2.886751345948128211 ) ) ;
#49823=CARTESIAN_POINT ( 'NONE',  ( 1.846868145590736310, -152.8750000013655779, 4.458734124999999437 ) ) ;
#49825=CARTESIAN_POINT ( 'NONE',  ( -2.500000000000000444, -81.04166666393547303, -4.330127018922193649 ) ) ;
#49826=CARTESIAN_POINT ( 'NONE',  ( -2.071067811865478170, -160.3125000000000284, 5.000000000000000000 ) ) ;
#49827=CARTESIAN_POINT ( 'NONE',  ( 1.975475456537005874E-15, 11.24999999999999822, 5.000000000000000000 ) ) ;
#49829=CARTESIAN_POINT ( 'NONE',  ( -3.152548672688508926E-16, -11.81249999863440969, -5.148502694627439702 ) ) ;
#49830=CARTESIAN_POINT ( 'NONE',  ( -4.458734124999999437, -47.56249999863440792, 0.000000000000000000 ) ) ;
#49832=CARTESIAN_POINT ( 'NONE',  ( -4.458734125000001214, -142.8750000013656063, 1.846868145590734089 ) ) ;
#49836=CARTESIAN_POINT ( 'NONE',  ( 0.000000000000000000, -170.0000000000000000, 0.000000000000000000 ) ) ;
#49837=CARTESIAN_POINT ( 'NONE',  ( -5.000000000000000000, -68.87499999726880162, 0.000000000000000000 ) ) ;
#49840=CARTESIAN_POINT ( 'NONE',  ( 5.000000000000000888, -30.58333333333333215, 2.886751345948126879 ) ) ;
#49841=ORIENTED_EDGE ( 'NONE', *, *, #51089, .F. ) ;
#49846=CARTESIAN_POINT ( 'NONE',  ( -4.458734124999999437, -6.395833331967740953, -2.574251347313719407 ) ) ;
#49848=CARTESIAN_POINT ( 'NONE',  ( -3.152801135295367985, -147.8125000013655779, 3.152801135295367096 ) ) ;
#49851=CARTESIAN_POINT ( 'NONE',  ( -2.071067811865604735, -148.3124999999999716, 4.999999999999872990 ) ) ;
#49854=CARTESIAN_POINT ( 'NONE',  ( 2.499999999999998668, 1.791666669397853795, -4.330127018922193649 ) ) ;
#49857=LINE ( 'NONE', #35717, #48561 ) ;
#49861=CARTESIAN_POINT ( 'NONE',  ( -2.229367062500000163, 13.52083333469892779, -3.861377020970580443 ) ) ;
#49863=ORIENTED_EDGE ( 'NONE', *, *, #17739, .F. ) ;
#49864=CARTESIAN_POINT ( 'NONE',  ( -2.229367062500000163, -13.72916666530107221, -3.861377020970580443 ) ) ;
#49866=CARTESIAN_POINT ( 'NONE',  ( 1.846868145590736310, -164.6250000013655779, 4.458734124999999437 ) ) ;
#49873=CARTESIAN_POINT ( 'NONE',  ( -4.999999999999998224, -54.79166666393548013, 2.886751345948131764 ) ) ;
#49876=CARTESIAN_POINT ( 'NONE',  ( -3.152801135295367985, -150.0625000013655779, 3.152801135295367096 ) ) ;
#49883=DIRECTION ( 'NONE',  ( -0.000000000000000000, 1.000000000000000000, -0.000000000000000000 ) ) ;
#49884=CARTESIAN_POINT ( 'NONE',  ( -3.535250795749689387E-16, -1.250000000000001110, -5.773502691896257311 ) ) ;
#49886=CARTESIAN_POINT ( 'NONE',  ( 2.229367062500001939, -65.97916666530106511, 3.861377020970579999 ) ) ;
#49888=CARTESIAN_POINT ( 'NONE',  ( -5.000000000000000000, -8.874999997268814056, 0.000000000000000000 ) ) ;
#49889=CARTESIAN_POINT ( 'NONE',  ( -4.458734124999999437, -32.31249999863440792, 0.000000000000000000 ) ) ;
#49893=VERTEX_POINT ( 'NONE', #62063 ) ;
#49895=CARTESIAN_POINT ( 'NONE',  ( -2.499999999999996447, -51.83333333333332860, 4.330127018922195425 ) ) ;
#49896=DIRECTION ( 'NONE',  ( 0.000000000000000000, 0.000000000000000000, 1.000000000000000000 ) ) ;
#49898=CARTESIAN_POINT ( 'NONE',  ( -6.972266317189433020E-16, -42.12499999726880873, -5.000000000000000000 ) ) ;
#49899=CARTESIAN_POINT ( 'NONE',  ( -4.458734124999998549, -78.22916666530106511, 2.574251347313722516 ) ) ;
#49900=CARTESIAN_POINT ( 'NONE',  ( -4.458734125000000326, -143.2500000013655779, -1.846868145590735644 ) ) ;
#49901=CARTESIAN_POINT ( 'NONE',  ( -4.458734124999999437, -82.39583333196773651, -2.574251347313719407 ) ) ;
#49903=AXIS2_PLACEMENT_3D ( 'NONE', #11757, #21751, #41986 ) ;
#49904=CARTESIAN_POINT ( 'NONE',  ( 9.457646018065525792E-16, -30.31249999863440436, 5.148502694627439702 ) ) ;
#49906=DIRECTION ( 'NONE',  ( -0.000000000000000000, 1.000000000000000000, -0.000000000000000000 ) ) ;
#49907=ORIENTED_EDGE ( 'NONE', *, *, #36719, .F. ) ;
#49910=ORIENTED_EDGE ( 'NONE', *, *, #27271, .T. ) ;
#49912=CARTESIAN_POINT ( 'NONE',  ( 2.499999999999998668, -12.33333333333333570, -4.330127018922193649 ) ) ;
#49913=CARTESIAN_POINT ( 'NONE',  ( -2.229367062499996610, -63.39583333196774362, 3.861377020970582219 ) ) ;
#49920=CARTESIAN_POINT ( 'NONE',  ( 4.458734124999998549, 11.27083333469892779, -2.574251347313721627 ) ) ;
#49923=CARTESIAN_POINT ( 'NONE',  ( 2.730187237215162345E-16, -160.1875000013655779, -4.458734124999999437 ) ) ;
#49924=CARTESIAN_POINT ( 'NONE',  ( 0.000000000000000000, -170.0000000000000000, 0.000000000000000000 ) ) ;
#49929=DIRECTION ( 'NONE',  ( -0.000000000000000000, 1.000000000000000000, -0.000000000000000000 ) ) ;
#49930=( BOUNDED_CURVE ( )  B_SPLINE_CURVE ( 2, ( #31940, #3005, #41898, #12329, #17149, #18090, #12948, #36448, #37098 ),
 .UNSPECIFIED., .F., .F. ) 
 B_SPLINE_CURVE_WITH_KNOTS ( ( 3, 2, 2, 2, 3 ),
 ( 0.3854166666666666852, 0.3861111111111111271, 0.3875000000000000111, 0.3888888888888888951, 0.3895833333333333370 ),
 .UNSPECIFIED. ) 
 CURVE ( )  GEOMETRIC_REPRESENTATION_ITEM ( )  RATIONAL_B_SPLINE_CURVE ( ( 0.9330127018922194093, 0.9330127018922194093, 1.000000000000000000, 0.8660254037844387076, 1.000000000000000000, 0.8660254037844387076, 1.000000000000000000, 0.9330127018922194093, 0.9330127018922194093 ) ) 
 REPRESENTATION_ITEM ( '' )  );
#49931=CARTESIAN_POINT ( 'NONE',  ( 1.975475456537005874E-15, -40.62499999726879452, 5.000000000000000000 ) ) ;
#49934=DIRECTION ( 'NONE',  ( -0.000000000000000000, 1.000000000000000000, -0.000000000000000000 ) ) ;
#49940=CARTESIAN_POINT ( 'NONE',  ( 2.229367062499998831, 4.104166668032260823, -3.861377020970580887 ) ) ;
#49941=VECTOR ( 'NONE', #34212, 1000.000000000000000 ) ;
#49942=CARTESIAN_POINT ( 'NONE',  ( -3.535533905932738641, -161.5000000027312126, 3.535533905932737309 ) ) ;
#49944=CARTESIAN_POINT ( 'NONE',  ( 5.000000000000000888, -146.0625000027312126, -2.071067811865475505 ) ) ;
#49945=CARTESIAN_POINT ( 'NONE',  ( 1.975475456537005874E-15, -84.62499999726880162, 5.000000000000000000 ) ) ;
#49949=VECTOR ( 'NONE', #18219, 1000.000000000000000 ) ;
#49953=CARTESIAN_POINT ( 'NONE',  ( 5.000000000000000000, -141.1875000027312126, 2.071067811865478614 ) ) ;
#49954=EDGE_CURVE ( 'NONE', #11304, #38064, #78, .T. ) ;
#49956=CARTESIAN_POINT ( 'NONE',  ( 3.152801135295366208, -165.8125000013656063, 3.152801135295367985 ) ) ;
#49958=CARTESIAN_POINT ( 'NONE',  ( 3.061616997868383141E-16, -159.8750000027311842, -5.000000000000000000 ) ) ;
#49962=CARTESIAN_POINT ( 'NONE',  ( -4.458734124999998549, 22.52083333469892423, 2.574251347313722516 ) ) ;
#49963=ORIENTED_EDGE ( 'NONE', *, *, #9778, .F. ) ;
#49964=CARTESIAN_POINT ( 'NONE',  ( -4.458734124999999437, -62.64583333196774362, -2.574251347313719407 ) ) ;
#49966=CARTESIAN_POINT ( 'NONE',  ( 2.500000000000002220, 12.33333333333333215, 4.330127018922192761 ) ) ;
#49967=EDGE_CURVE ( 'NONE', #10973, #6056, #46100, .T. ) ;
#49968=CARTESIAN_POINT ( 'NONE',  ( 4.458734124999998549, -51.72916666530107221, -2.574251347313721627 ) ) ;
#49969=CARTESIAN_POINT ( 'NONE',  ( -2.229367062500000163, -10.47916666530106866, -3.861377020970580443 ) ) ;
#49971=CYLINDRICAL_SURFACE ( 'NONE', #14261, 5.000000000000000000 ) ;
#49972=CARTESIAN_POINT ( 'NONE',  ( -6.972266317189433020E-16, -27.12499999726881228, -5.000000000000000000 ) ) ;
#49973=ADVANCED_FACE ( 'NONE', ( #4148 ), #43366, .T. ) ;
#49976=CARTESIAN_POINT ( 'NONE',  ( 2.500000000000002220, 21.45833333606451987, 4.330127018922192761 ) ) ;
#49979=CARTESIAN_POINT ( 'NONE',  ( 9.457646018065525792E-16, -59.06249999863439371, 5.148502694627439702 ) ) ;
#49980=CARTESIAN_POINT ( 'NONE',  ( 1.846868145590736310, -156.8750000013655779, 4.458734124999999437 ) ) ;
#49981=CARTESIAN_POINT ( 'NONE',  ( -2.499999999999996447, -55.70833333060214443, 4.330127018922195425 ) ) ;
#49984=CARTESIAN_POINT ( 'NONE',  ( -4.458734124999999437, -1.562499998634406140, 0.000000000000000000 ) ) ;
#49988=CARTESIAN_POINT ( 'NONE',  ( 1.846868145590736310, -154.6250000013655779, 4.458734124999999437 ) ) ;
#49989=EDGE_LOOP ( 'NONE', ( #40172, #58454, #3091, #15616 ) ) ;
#49991=VECTOR ( 'NONE', #4871, 1000.000000000000000 ) ;
#49994=CARTESIAN_POINT ( 'NONE',  ( 4.458734124999998549, -44.97916666530107221, -2.574251347313721627 ) ) ;
#49996=ORIENTED_EDGE ( 'NONE', *, *, #27490, .T. ) ;
#50000=CARTESIAN_POINT ( 'NONE',  ( 4.458734124999999437, 27.18750000136559564, -5.460374474430324690E-16 ) ) ;
#50003=FACE_OUTER_BOUND ( 'NONE', #32822, .T. ) ;
#50004=FACE_OUTER_BOUND ( 'NONE', #52224, .T. ) ;
#50009=CARTESIAN_POINT ( 'NONE',  ( 5.000000000000000000, -157.1250000027311842, 0.000000000000000000 ) ) ;
#50012=CARTESIAN_POINT ( 'NONE',  ( 5.000000000000000000, -42.29166666393548724, -2.886751345948130876 ) ) ;
#50013=DIRECTION ( 'NONE',  ( -0.000000000000000000, 1.000000000000000000, -0.000000000000000000 ) ) ;
#50014=CARTESIAN_POINT ( 'NONE',  ( -2.229367062499996610, -90.39583333196773651, 3.861377020970582219 ) ) ;
#50015=FACE_OUTER_BOUND ( 'NONE', #30940, .T. ) ;
#50018=ORIENTED_EDGE ( 'NONE', *, *, #29545, .T. ) ;
#50019=CARTESIAN_POINT ( 'NONE',  ( -5.000000000000000888, -163.5625000027312126, 2.071067811865474617 ) ) ;
#50021=CARTESIAN_POINT ( 'NONE',  ( 5.000000000000000000, -156.1875000027312126, 2.071067811865478614 ) ) ;
#50029=EDGE_CURVE ( 'NONE', #42274, #12871, #63013, .T. ) ;
#50033=CARTESIAN_POINT ( 'NONE',  ( 1.339745962155615144, -48.58034179853029855, 4.999999999999999112 ) ) ;
#50034=CARTESIAN_POINT ( 'NONE',  ( -4.458734124999999437, -22.31249999863440436, 0.000000000000000000 ) ) ;
#50036=CARTESIAN_POINT ( 'NONE',  ( -5.000000000000000888, -149.5625000000000568, -2.071067811865475949 ) ) ;
#50038=CARTESIAN_POINT ( 'NONE',  ( -4.458734124999999437, -153.9375000013655779, -5.460374474430324690E-16 ) ) ;
#50040=CARTESIAN_POINT ( 'NONE',  ( -4.458734124999999437, -45.64583333196774362, -2.574251347313719407 ) ) ;
#50044=CARTESIAN_POINT ( 'NONE',  ( -3.152548672688508926E-16, -88.56249999863439371, -5.148502694627439702 ) ) ;
#50046=VECTOR ( 'NONE', #54375, 1000.000000000000000 ) ;
#50047=CARTESIAN_POINT ( 'NONE',  ( -2.229367062499996610, 5.854166668032262599, 3.861377020970582219 ) ) ;
#50050=CARTESIAN_POINT ( 'NONE',  ( -6.972266317189433020E-16, -5.124999997268812280, -5.000000000000000000 ) ) ;
#50051=CARTESIAN_POINT ( 'NONE',  ( 4.458734125000001214, 18.85416666803226349, 2.574251347313718519 ) ) ;
#50053=CARTESIAN_POINT ( 'NONE',  ( 2.499999999999998668, 5.791666669397853795, -4.330127018922193649 ) ) ;
#50059=CARTESIAN_POINT ( 'NONE',  ( -2.229367062500000163, -38.47916666530107221, -3.861377020970580443 ) ) ;
#50062=CARTESIAN_POINT ( 'NONE',  ( 2.500000000000002220, -37.54166666393548013, 4.330127018922192761 ) ) ;
#50063=ORIENTED_EDGE ( 'NONE', *, *, #34637, .T. ) ;
#50064=CARTESIAN_POINT ( 'NONE',  ( 4.458734124999999437, -15.81249999863440436, -5.460374474430324690E-16 ) ) ;
#50066=CARTESIAN_POINT ( 'NONE',  ( 5.000000000000000000, -83.49999999999998579, -6.123233995736766282E-16 ) ) ;
#50067=CARTESIAN_POINT ( 'NONE',  ( 4.458734125000000326, -168.3750000013655779, -1.846868145590734978 ) ) ;
#50068=CARTESIAN_POINT ( 'NONE',  ( 2.499999999999998668, -85.20833333060214443, -4.330127018922193649 ) ) ;
#50070=VERTEX_POINT ( 'NONE', #3834 ) ;
#50072=CARTESIAN_POINT ( 'NONE',  ( 4.458734124999998549, -27.97916666530107577, -2.574251347313721627 ) ) ;
#50075=CARTESIAN_POINT ( 'NONE',  ( 3.152801135295367541, -164.5625000013656063, -3.152801135295367541 ) ) ;
#50077=CARTESIAN_POINT ( 'NONE',  ( -6.972266317189433020E-16, -39.12499999726880162, -5.000000000000000000 ) ) ;
#50080=CARTESIAN_POINT ( 'NONE',  ( -4.458734124999998549, -75.47916666530107932, 2.574251347313722516 ) ) ;
#50083=CARTESIAN_POINT ( 'NONE',  ( 4.458734124999999437, -141.6875000013656063, 0.000000000000000000 ) ) ;
#50085=DIRECTION ( 'NONE',  ( -0.000000000000000000, 1.000000000000000000, -0.000000000000000000 ) ) ;
#50097=CARTESIAN_POINT ( 'NONE',  ( 4.458734124999999437, -74.06249999863440792, -5.460374474430324690E-16 ) ) ;
#50098=CARTESIAN_POINT ( 'NONE',  ( 2.499999999999998668, -34.33333333333332860, -4.330127018922193649 ) ) ;
#50101=CARTESIAN_POINT ( 'NONE',  ( -2.071067811865580754, -159.6874999999999716, -4.999999999999894307 ) ) ;
#50106=CARTESIAN_POINT ( 'NONE',  ( -2.229367062500000163, 17.27083333469892779, -3.861377020970580443 ) ) ;
#50107=FACE_OUTER_BOUND ( 'NONE', #36981, .T. ) ;
#50112=CARTESIAN_POINT ( 'NONE',  ( 0.000000000000000000, -170.0000000000000000, 0.000000000000000000 ) ) ;
#50113=CARTESIAN_POINT ( 'NONE',  ( 4.458734124999999437, -86.81249999863439371, -5.460374474430324690E-16 ) ) ;
#50114=CARTESIAN_POINT ( 'NONE',  ( -2.229367062499996610, -4.145833331967739177, 3.861377020970582219 ) ) ;
#50115=VERTEX_POINT ( 'NONE', #275 ) ;
#50116=CARTESIAN_POINT ( 'NONE',  ( 4.458734125000000326, -30.14583333196773651, 2.574251347313718519 ) ) ;
#50121=CARTESIAN_POINT ( 'NONE',  ( 2.229367062499998831, 20.35416666803225993, -3.861377020970580887 ) ) ;
#50124=CARTESIAN_POINT ( 'NONE',  ( 4.458734124999999437, -78.06249999863440792, -5.460374474430324690E-16 ) ) ;
#50127=CARTESIAN_POINT ( 'NONE',  ( -4.999999999999999112, 24.20833333606451987, 2.886751345948131764 ) ) ;
#50131=CARTESIAN_POINT ( 'NONE',  ( -3.535533905932737309, -149.6250000000000000, -3.535533905932738197 ) ) ;
#50132=CARTESIAN_POINT ( 'NONE',  ( 5.000000000000000000, -16.50000000000000000, -6.123233995736766282E-16 ) ) ;
#50133=CARTESIAN_POINT ( 'NONE',  ( -4.458734124999999437, -24.39583333196773651, -2.574251347313719407 ) ) ;
#50134=CARTESIAN_POINT ( 'NONE',  ( -3.152548672688508926E-16, -82.56249999863440792, -5.148502694627439702 ) ) ;
#50135=CARTESIAN_POINT ( 'NONE',  ( -4.999999999999999112, -25.79166666393547658, 2.886751345948131764 ) ) ;
#50136=CARTESIAN_POINT ( 'NONE',  ( 4.458734124999999437, -52.81249999863440792, -5.460374474430324690E-16 ) ) ;
#50137=ORIENTED_EDGE ( 'NONE', *, *, #36629, .T. ) ;
#50138=CARTESIAN_POINT ( 'NONE',  ( -6.972266317189433020E-16, -90.12499999726880162, -5.000000000000000000 ) ) ;
#50139=DIRECTION ( 'NONE',  ( -0.000000000000000000, 1.000000000000000000, -0.000000000000000000 ) ) ;
#50140=CARTESIAN_POINT ( 'NONE',  ( 4.458734124999999437, -6.062499998634403475, -5.460374474430324690E-16 ) ) ;
#50141=ORIENTED_EDGE ( 'NONE', *, *, #45902, .T. ) ;
#50143=CARTESIAN_POINT ( 'NONE',  ( 2.499999999999998668, -66.33333333333332860, -4.330127018922193649 ) ) ;
#50144=CARTESIAN_POINT ( 'NONE',  ( 2.730187237215162345E-16, -152.4375000013655779, -4.458734124999999437 ) ) ;
#50146=CARTESIAN_POINT ( 'NONE',  ( -1.339745962155613812, -81.08034179853028434, -5.000000000000000000 ) ) ;
#50147=CARTESIAN_POINT ( 'NONE',  ( 5.000000000000000000, -159.0000000000000000, 0.000000000000000000 ) ) ;
#50150=CARTESIAN_POINT ( 'NONE',  ( 4.458734124999998549, -12.97916666530107044, -2.574251347313721627 ) ) ;
#50152=CARTESIAN_POINT ( 'NONE',  ( 4.458734124999998549, -49.97916666530106511, -2.574251347313721627 ) ) ;
#50154=CARTESIAN_POINT ( 'NONE',  ( 3.152801135295367541, -146.3125000013655779, -3.152801135295367541 ) ) ;
#50156=CARTESIAN_POINT ( 'NONE',  ( 1.062108568985190270E-13, -11.12499999726881761, -4.999999999999999112 ) ) ;
#50158=CARTESIAN_POINT ( 'NONE',  ( 4.458734124999999437, 26.93750000136559564, -5.460374474430324690E-16 ) ) ;
#50160=CARTESIAN_POINT ( 'NONE',  ( 5.000000000000000000, -30.41666666666666785, -2.886751345948130876 ) ) ;
#50167=CARTESIAN_POINT ( 'NONE',  ( 2.500000000000002220, 11.45833333606451809, 4.330127018922192761 ) ) ;
#50168=CARTESIAN_POINT ( 'NONE',  ( 4.458734125000001214, -5.895833331967740953, 2.574251347313718519 ) ) ;
#50170=CARTESIAN_POINT ( 'NONE',  ( -3.152801135295367985, -149.8125000013655779, 3.152801135295367096 ) ) ;
#50171=( BOUNDED_CURVE ( )  B_SPLINE_CURVE ( 2, ( #17389, #12548, #45698, #55679, #7104, #41490, #2595, #30901, #26394 ),
 .UNSPECIFIED., .F., .F. ) 
 B_SPLINE_CURVE_WITH_KNOTS ( ( 3, 2, 2, 2, 3 ),
 ( 0.5479166666666667185, 0.5486111111111111605, 0.5500000000000000444, 0.5513888888888889284, 0.5520833333333333703 ),
 .UNSPECIFIED. ) 
 CURVE ( )  GEOMETRIC_REPRESENTATION_ITEM ( )  RATIONAL_B_SPLINE_CURVE ( ( 0.9330127018922194093, 0.9330127018922194093, 1.000000000000000000, 0.8660254037844387076, 1.000000000000000000, 0.8660254037844387076, 1.000000000000000000, 0.9330127018922194093, 0.9330127018922194093 ) ) 
 REPRESENTATION_ITEM ( '' )  );
#50178=VECTOR ( 'NONE', #36387, 1000.000000000000000 ) ;
#50182=CARTESIAN_POINT ( 'NONE',  ( 6.123233995736766282E-16, -170.0000000000000000, -5.000000000000000000 ) ) ;
#50184=CARTESIAN_POINT ( 'NONE',  ( 0.000000000000000000, -170.0000000000000000, 0.000000000000000000 ) ) ;
#50185=CARTESIAN_POINT ( 'NONE',  ( 5.000000000000000000, 9.499999999999998224, -6.123233995736766282E-16 ) ) ;
#50186=CARTESIAN_POINT ( 'NONE',  ( 4.458734125000000326, 10.10416666803226171, 2.574251347313718519 ) ) ;
#50189=CARTESIAN_POINT ( 'NONE',  ( -2.229367062499996610, -13.39583333196774007, 3.861377020970582219 ) ) ;
#50191=CARTESIAN_POINT ( 'NONE',  ( 4.458734124999999437, -163.5000000013655779, 1.846868145590737864 ) ) ;
#50192=CARTESIAN_POINT ( 'NONE',  ( -2.500000000000000444, -38.16666666666667140, -4.330127018922193649 ) ) ;
#50196=CIRCLE ( 'NONE', #18381, 5.000000000000000000 ) ;
#50198=CARTESIAN_POINT ( 'NONE',  ( -6.972266317189433020E-16, -29.12499999726881228, -5.000000000000000000 ) ) ;
#50199=CARTESIAN_POINT ( 'NONE',  ( 1.975475456537005874E-15, -63.62499999726880873, 5.000000000000000000 ) ) ;
#50201=CARTESIAN_POINT ( 'NONE',  ( -1.846868145590734756, -149.3750000013656063, -4.458734124999999437 ) ) ;
#50210=CARTESIAN_POINT ( 'NONE',  ( 1.060575238724906964E-15, -3.750000000000003553, 5.773502691896257311 ) ) ;
#50211=CARTESIAN_POINT ( 'NONE',  ( -4.458734124999999437, -67.31249999863440792, 0.000000000000000000 ) ) ;
#50213=CARTESIAN_POINT ( 'NONE',  ( -5.000000000000000000, -9.958333330602144429, -2.886751345948128211 ) ) ;
#50214=CARTESIAN_POINT ( 'NONE',  ( 4.458734125000001214, -35.89583333196773651, 2.574251347313718519 ) ) ;
#50215=ORIENTED_EDGE ( 'NONE', *, *, #13455, .F. ) ;
#50216=CARTESIAN_POINT ( 'NONE',  ( 3.061616997868383141E-16, -165.7500000000000000, -5.000000000000000000 ) ) ;
#50217=DIRECTION ( 'NONE',  ( -0.000000000000000000, 1.000000000000000000, -0.000000000000000000 ) ) ;
#50218=CARTESIAN_POINT ( 'NONE',  ( -4.458734124999998549, 14.52083333469892779, 2.574251347313722516 ) ) ;
#50221=CARTESIAN_POINT ( 'NONE',  ( 5.000000000000000000, -50.50000000000000000, -6.123233995736766282E-16 ) ) ;
#50223=VECTOR ( 'NONE', #47683, 1000.000000000000000 ) ;
#50225=CARTESIAN_POINT ( 'NONE',  ( -4.458734124999999437, -75.39583333196773651, -2.574251347313719407 ) ) ;
#50226=( BOUNDED_CURVE ( )  B_SPLINE_CURVE ( 2, ( #35611, #32044, #6984, #7306, #55237, #1852, #1222, #36246, #21134 ),
 .UNSPECIFIED., .F., .F. ) 
 B_SPLINE_CURVE_WITH_KNOTS ( ( 3, 2, 2, 2, 3 ),
 ( 0.07500000000000005274, 0.07916666666666671848, 0.08333333333333339810, 0.08750000000000007772, 0.09166666666666674346 ),
 .UNSPECIFIED. ) 
 CURVE ( )  GEOMETRIC_REPRESENTATION_ITEM ( )  RATIONAL_B_SPLINE_CURVE ( ( 0.9999999999999990008, 0.9238795325112877377, 1.000000000000000000, 0.9238795325112867385, 1.000000000000000000, 0.9238795325112867385, 1.000000000000000000, 0.9238795325112851842, 1.000000000000001554 ) ) 
 REPRESENTATION_ITEM ( '' )  );
#50227=CARTESIAN_POINT ( 'NONE',  ( -1.846868145590734756, -141.3750000013656063, -4.458734125000000326 ) ) ;
#50228=CARTESIAN_POINT ( 'NONE',  ( -4.458734124999999437, -80.31249999863440792, 0.000000000000000000 ) ) ;
#50231=CARTESIAN_POINT ( 'NONE',  ( -2.229367062499996610, -32.39583333196773651, 3.861377020970582219 ) ) ;
#50233=CARTESIAN_POINT ( 'NONE',  ( 0.000000000000000000, -170.0000000000000000, 5.000000000000000000 ) ) ;
#50236=CARTESIAN_POINT ( 'NONE',  ( -5.000000000000000000, 22.12500000273118417, 0.000000000000000000 ) ) ;
#50240=CARTESIAN_POINT ( 'NONE',  ( 2.229367062499998831, -63.89583333196772941, -3.861377020970580887 ) ) ;
#50243=ORIENTED_EDGE ( 'NONE', *, *, #4362, .F. ) ;
#50244=CYLINDRICAL_SURFACE ( 'NONE', #63501, 5.000000000000000000 ) ;
#50246=CARTESIAN_POINT ( 'NONE',  ( -4.458734124999999437, 5.604166668032262599, -2.574251347313719407 ) ) ;
#50249=CARTESIAN_POINT ( 'NONE',  ( -1.846868145590734756, -160.1250000013655779, -4.458734124999999437 ) ) ;
#50250=CARTESIAN_POINT ( 'NONE',  ( -5.000000000000000000, 19.04166666939784847, -2.886751345948128211 ) ) ;
#50251=ORIENTED_EDGE ( 'NONE', *, *, #26751, .T. ) ;
#50255=CARTESIAN_POINT ( 'NONE',  ( 1.339745962155615588, 25.83034180399265622, -4.999999999999997335 ) ) ;
#50257=CARTESIAN_POINT ( 'NONE',  ( 2.499999999999998668, -36.33333333333332860, -4.330127018922193649 ) ) ;
#50260=EDGE_CURVE ( 'NONE', #21155, #19310, #29834, .T. ) ;
#50261=CARTESIAN_POINT ( 'NONE',  ( 1.339745962155615144, 12.41965820146970501, 4.999999999999999112 ) ) ;
#50263=CARTESIAN_POINT ( 'NONE',  ( 2.229367062500001939, 27.02083333469892423, 3.861377020970579999 ) ) ;
#50266=CARTESIAN_POINT ( 'NONE',  ( 9.457646018065525792E-16, 3.687500001365594748, 5.148502694627439702 ) ) ;
#50267=AXIS2_PLACEMENT_3D ( 'NONE', #63499, #39902, #45379 ) ;
#50268=CARTESIAN_POINT ( 'NONE',  ( 2.071067811865392461, -146.3125000027312694, 5.000000000000084377 ) ) ;
#50270=CARTESIAN_POINT ( 'NONE',  ( 2.071067811865476394, -147.3125000027311842, 5.000000000000000000 ) ) ;
#50271=CARTESIAN_POINT ( 'NONE',  ( 1.975475456537005874E-15, -33.62499999726880873, 5.000000000000000000 ) ) ;
#50278=CARTESIAN_POINT ( 'NONE',  ( 1.339745962155612702, 3.705341801261478718, -5.000000000000000000 ) ) ;
#50280=CARTESIAN_POINT ( 'NONE',  ( 2.730187237215162345E-16, -160.4375000013655779, -4.458734124999999437 ) ) ;
#50283=CARTESIAN_POINT ( 'NONE',  ( 3.152801135295367541, -141.3125000013655779, -3.152801135295367541 ) ) ;
#50285=CARTESIAN_POINT ( 'NONE',  ( -2.229367062499996610, 25.60416666803225993, 3.861377020970582219 ) ) ;
#50286=ORIENTED_EDGE ( 'NONE', *, *, #28401, .F. ) ;
#50287=CARTESIAN_POINT ( 'NONE',  ( 2.229367062499998831, -63.89583333196772941, -3.861377020970580887 ) ) ;
#50289=CARTESIAN_POINT ( 'NONE',  ( -2.500000000000000444, -3.041666663935477910, -4.330127018922193649 ) ) ;
#50290=CARTESIAN_POINT ( 'NONE',  ( 5.000000000000000000, 14.58333333333333215, -2.886751345948129988 ) ) ;
#50291=CARTESIAN_POINT ( 'NONE',  ( -4.458734124999997661, -48.22916666530106511, 2.574251347313722516 ) ) ;
#50292=CARTESIAN_POINT ( 'NONE',  ( 4.458734124999999437, -11.81249999863440081, -5.460374474430324690E-16 ) ) ;
#50293=CARTESIAN_POINT ( 'NONE',  ( 0.000000000000000000, -170.0000000000000000, 5.000000000000000000 ) ) ;
#50294=EDGE_CURVE ( 'NONE', #59225, #35059, #40762, .T. ) ;
#50295=CARTESIAN_POINT ( 'NONE',  ( 1.975475456537005874E-15, 14.25000000000000000, 5.000000000000000000 ) ) ;
#50298=CARTESIAN_POINT ( 'NONE',  ( 1.060575238724906964E-15, -33.75000000000000000, 5.773502691896257311 ) ) ;
#50302=CARTESIAN_POINT ( 'NONE',  ( 2.229367062499998831, -60.64583333196774362, -3.861377020970580887 ) ) ;
#50303=CARTESIAN_POINT ( 'NONE',  ( 2.730187237215162345E-16, -152.4375000013655779, -4.458734124999999437 ) ) ;
#50304=CARTESIAN_POINT ( 'NONE',  ( -2.229367062500000163, -68.47916666530107932, -3.861377020970580443 ) ) ;
#50306=CARTESIAN_POINT ( 'NONE',  ( 2.499999999999998668, -56.20833333060214443, -4.330127018922193649 ) ) ;
#50308=CARTESIAN_POINT ( 'NONE',  ( -6.972266317189433020E-16, -26.25000000000000000, -5.000000000000000000 ) ) ;
#50309=CARTESIAN_POINT ( 'NONE',  ( 4.458734125000001214, -0.1458333319677394824, 2.574251347313718519 ) ) ;
#50313=CARTESIAN_POINT ( 'NONE',  ( 3.152801135295366208, -154.5625000013656063, 3.152801135295367985 ) ) ;
#50320=CARTESIAN_POINT ( 'NONE',  ( -4.458734124999998549, -48.47916666530106511, 2.574251347313722516 ) ) ;
#50322=EDGE_LOOP ( 'NONE', ( #28086, #41566, #26656, #47142 ) ) ;
#50324=EDGE_CURVE ( 'NONE', #29294, #60836, #22251, .T. ) ;
#50325=EDGE_CURVE ( 'NONE', #49104, #17322, #1876, .T. ) ;
#50326=CARTESIAN_POINT ( 'NONE',  ( 5.000000000000000000, 10.62500000273118594, -6.123233995736766282E-16 ) ) ;
#50328=CARTESIAN_POINT ( 'NONE',  ( 2.229367062499998831, 26.35416666803225993, -3.861377020970580887 ) ) ;
#50333=CARTESIAN_POINT ( 'NONE',  ( 1.975475456537005874E-15, 1.250000000000000000, 5.000000000000000000 ) ) ;
#50336=CARTESIAN_POINT ( 'NONE',  ( -5.000000000000000888, -157.5625000000000853, -2.071067811865475949 ) ) ;
#50340=EDGE_CURVE ( 'NONE', #34622, #50557, #30151, .T. ) ;
#50342=CARTESIAN_POINT ( 'NONE',  ( 4.458734125000001214, -88.14583333196773651, 2.574251347313718519 ) ) ;
#50346=CARTESIAN_POINT ( 'NONE',  ( -3.535533905932738641, -163.5000000027312126, 3.535533905932737309 ) ) ;
#50348=CARTESIAN_POINT ( 'NONE',  ( 3.535533905932736864, -157.2500000027312126, 3.535533905932738641 ) ) ;
#50358=CARTESIAN_POINT ( 'NONE',  ( 4.458734124999999437, -20.81249999863440081, -5.460374474430324690E-16 ) ) ;
#50360=CARTESIAN_POINT ( 'NONE',  ( -3.535533905932737309, -152.6250000000000000, -3.535533905932738197 ) ) ;
#50362=CARTESIAN_POINT ( 'NONE',  ( -1.846868145590734756, -150.1250000013655779, -4.458734125000000326 ) ) ;
#50363=ORIENTED_EDGE ( 'NONE', *, *, #548, .F. ) ;
#50364=VECTOR ( 'NONE', #26617, 1000.000000000000000 ) ;
#50365=CARTESIAN_POINT ( 'NONE',  ( -2.229367062499996610, -48.39583333196772941, 3.861377020970582219 ) ) ;
#50366=LINE ( 'NONE', #19812, #22277 ) ;
#50368=CARTESIAN_POINT ( 'NONE',  ( 4.458734125000001214, -89.89583333196775072, 2.574251347313718519 ) ) ;
#50369=CARTESIAN_POINT ( 'NONE',  ( -4.458734124999999437, 2.687500001365593860, 0.000000000000000000 ) ) ;
#50370=CARTESIAN_POINT ( 'NONE',  ( -5.000000000000000888, -160.5625000027312126, 2.071067811865474617 ) ) ;
#50371=CARTESIAN_POINT ( 'NONE',  ( 1.339745962155661996, -11.16965819600733667, -4.999999999999970690 ) ) ;
#50373=CARTESIAN_POINT ( 'NONE',  ( -4.458734124999999437, 16.43750000136559564, 0.000000000000000000 ) ) ;
#50375=CARTESIAN_POINT ( 'NONE',  ( 5.000000000000000000, 8.625000002731184168, -6.123233995736766282E-16 ) ) ;
#50376=ORIENTED_EDGE ( 'NONE', *, *, #11766, .T. ) ;
#50377=CARTESIAN_POINT ( 'NONE',  ( -6.972266317189433020E-16, -70.25000000000000000, -5.000000000000000000 ) ) ;
#50381=CARTESIAN_POINT ( 'NONE',  ( -4.458734124999998549, -43.22916666530105800, 2.574251347313722516 ) ) ;
#50382=CARTESIAN_POINT ( 'NONE',  ( -4.458734124999999437, -168.1875000013655779, -5.460374474430324690E-16 ) ) ;
#50383=CARTESIAN_POINT ( 'NONE',  ( 2.499999999999998668, -38.20833333060213732, -4.330127018922193649 ) ) ;
#50385=CARTESIAN_POINT ( 'NONE',  ( 2.229367062500001939, -15.97916666530107399, 3.861377020970579999 ) ) ;
#50387=CARTESIAN_POINT ( 'NONE',  ( 1.060575238724906964E-15, -88.74999999999998579, 5.773502691896257311 ) ) ;
#50388=CARTESIAN_POINT ( 'NONE',  ( -4.458734125000001214, -168.8750000013655779, 1.846868145590734089 ) ) ;
#50389=CARTESIAN_POINT ( 'NONE',  ( -4.999999999999999112, -86.79166666393548724, 2.886751345948131764 ) ) ;
#50390=CARTESIAN_POINT ( 'NONE',  ( 1.339745962155612702, -20.16965819600733312, -5.000000000000000000 ) ) ;
#50393=CARTESIAN_POINT ( 'NONE',  ( 9.457646018065525792E-16, -34.31249999863440792, 5.148502694627439702 ) ) ;
#50395=ORIENTED_EDGE ( 'NONE', *, *, #34543, .T. ) ;
#50396=EDGE_CURVE ( 'NONE', #29442, #27774, #48892, .T. ) ;
#50400=CARTESIAN_POINT ( 'NONE',  ( 1.975475456537005874E-15, -55.62499999726880873, 5.000000000000000000 ) ) ;
#50401=ADVANCED_FACE ( 'NONE', ( #41079 ), #22985, .T. ) ;
#50405=VECTOR ( 'NONE', #4085, 1000.000000000000000 ) ;
#50406=CARTESIAN_POINT ( 'NONE',  ( 9.457646018065525792E-16, -77.31249999863440792, 5.148502694627439702 ) ) ;
#50409=CARTESIAN_POINT ( 'NONE',  ( 1.846868145590736310, -140.8750000013656063, 4.458734124999997661 ) ) ;
#50412=CARTESIAN_POINT ( 'NONE',  ( 1.339745962155618697, 24.70534180126148627, -4.999999999999998224 ) ) ;
#50414=CARTESIAN_POINT ( 'NONE',  ( 2.229367062499998831, -45.64583333196774362, -3.861377020970580887 ) ) ;
#50415=VECTOR ( 'NONE', #58357, 1000.000000000000000 ) ;
#50421=CARTESIAN_POINT ( 'NONE',  ( 1.975475456537005874E-15, -37.62499999726880873, 5.000000000000000000 ) ) ;
#50424=FACE_OUTER_BOUND ( 'NONE', #49265, .T. ) ;
#50426=CARTESIAN_POINT ( 'NONE',  ( -3.152548672688508926E-16, -71.81249999863439371, -5.148502694627439702 ) ) ;
#50431=ORIENTED_EDGE ( 'NONE', *, *, #43261, .F. ) ;
#50434=CARTESIAN_POINT ( 'NONE',  ( 5.000000000000000000, -15.50000000000000000, -6.123233995736766282E-16 ) ) ;
#50439=CARTESIAN_POINT ( 'NONE',  ( 9.457646018065525792E-16, 16.68750000136559564, 5.148502694627439702 ) ) ;
#50440=CARTESIAN_POINT ( 'NONE',  ( 2.500000000000002220, -77.54166666393547303, 4.330127018922192761 ) ) ;
#50442=ADVANCED_FACE ( 'NONE', ( #57402 ), #48356, .T. ) ;
#50448=CARTESIAN_POINT ( 'NONE',  ( -3.152548672688508926E-16, -87.56249999863440792, -5.148502694627439702 ) ) ;
#50449=CARTESIAN_POINT ( 'NONE',  ( -2.229367062499996610, -2.145833331967737845, 3.861377020970582219 ) ) ;
#50450=CARTESIAN_POINT ( 'NONE',  ( 5.000000000000000000, -169.1250000027312126, 0.000000000000000000 ) ) ;
#50451=ORIENTED_EDGE ( 'NONE', *, *, #60368, .F. ) ;
#50452=CARTESIAN_POINT ( 'NONE',  ( -4.458734124999999437, -28.64583333196774007, -2.574251347313719407 ) ) ;
#50456=CARTESIAN_POINT ( 'NONE',  ( 9.457646018065525792E-16, 18.93750000136559208, 5.148502694627439702 ) ) ;
#50459=CARTESIAN_POINT ( 'NONE',  ( 4.458734125000000326, -78.14583333196775072, 2.574251347313718519 ) ) ;
#50462=CARTESIAN_POINT ( 'NONE',  ( -3.535250795749689387E-16, 26.87500000273118772, -5.773502691896257311 ) ) ;
#50464=CARTESIAN_POINT ( 'NONE',  ( 1.339745962155612702, -1.169658196007335338, -5.000000000000000000 ) ) ;
#50465=DIRECTION ( 'NONE',  ( 0.000000000000000000, 0.000000000000000000, 1.000000000000000000 ) ) ;
#50467=CARTESIAN_POINT ( 'NONE',  ( -2.499999999999996447, -25.83333333333333215, 4.330127018922195425 ) ) ;
#50468=CARTESIAN_POINT ( 'NONE',  ( -4.458734124999998549, -27.22916666530107221, 2.574251347313722516 ) ) ;
#50470=CARTESIAN_POINT ( 'NONE',  ( -3.152548672688508926E-16, -88.56249999863439371, -5.148502694627439702 ) ) ;
#50471=CARTESIAN_POINT ( 'NONE',  ( -2.499999999999996447, -21.70833333060214798, 4.330127018922195425 ) ) ;
#50472=CARTESIAN_POINT ( 'NONE',  ( 2.229367062499998831, -57.64583333196773651, -3.861377020970580887 ) ) ;
#50475=CARTESIAN_POINT ( 'NONE',  ( 1.162044386198238837E-16, 29.25000000000000000, 5.000000000000000000 ) ) ;
#50476=CARTESIAN_POINT ( 'NONE',  ( 2.229367062499998831, -3.895833331967739177, -3.861377020970580887 ) ) ;
#50478=CARTESIAN_POINT ( 'NONE',  ( -2.499999999999996447, -63.83333333333332860, 4.330127018922195425 ) ) ;
#50479=CARTESIAN_POINT ( 'NONE',  ( 3.152801135295366208, -151.8125000013655779, 3.152801135295367985 ) ) ;
#50481=CARTESIAN_POINT ( 'NONE',  ( 0.000000000000000000, -170.0000000000000000, 5.000000000000000000 ) ) ;
#50482=CARTESIAN_POINT ( 'NONE',  ( 3.535533905932736864, -157.1250000000000284, 3.535533905932738641 ) ) ;
#50483=CARTESIAN_POINT ( 'NONE',  ( 5.000000000000000000, -10.37499999726881583, -6.123233995736766282E-16 ) ) ;
#50485=CARTESIAN_POINT ( 'NONE',  ( 4.458734124999999437, -10.06249999863440614, -5.460374474430324690E-16 ) ) ;
#50486=CARTESIAN_POINT ( 'NONE',  ( 2.229367062500001939, -53.22916666530107221, 3.861377020970579999 ) ) ;
#50488=CARTESIAN_POINT ( 'NONE',  ( -4.458734125000000326, -143.0000000013655779, -1.846868145590735644 ) ) ;
#50492=CYLINDRICAL_SURFACE ( 'NONE', #34416, 5.000000000000000000 ) ;
#50493=CARTESIAN_POINT ( 'NONE',  ( -3.152548672688508926E-16, 25.18750000136558853, -5.148502694627439702 ) ) ;
#50500=CARTESIAN_POINT ( 'NONE',  ( 3.061616997868383141E-16, -154.8750000027311842, -5.000000000000000000 ) ) ;
#50501=CARTESIAN_POINT ( 'NONE',  ( -2.229367062499996610, -6.145833331967740953, 3.861377020970582219 ) ) ;
#50503=CARTESIAN_POINT ( 'NONE',  ( -8.190561711645485556E-16, -149.6875000013656063, 4.458734124999999437 ) ) ;
#50505=VERTEX_POINT ( 'NONE', #3990 ) ;
#50506=CARTESIAN_POINT ( 'NONE',  ( -2.499999999999996447, -62.70833333060214443, 4.330127018922195425 ) ) ;
#50509=VECTOR ( 'NONE', #23617, 1000.000000000000000 ) ;
#50510=CARTESIAN_POINT ( 'NONE',  ( 5.000000000000000000, -25.29166666393547658, -2.886751345948130876 ) ) ;
#50520=CARTESIAN_POINT ( 'NONE',  ( -3.152548672688508926E-16, 13.43750000136559386, -5.148502694627439702 ) ) ;
#50522=CARTESIAN_POINT ( 'NONE',  ( 4.458734124999999437, -14.06249999863440436, -5.460374474430324690E-16 ) ) ;
#50524=CARTESIAN_POINT ( 'NONE',  ( -8.190561711645485556E-16, -163.6875000013655779, 4.458734124999999437 ) ) ;
#50527=CARTESIAN_POINT ( 'NONE',  ( -4.999999999999998224, -76.91666666666667140, 2.886751345948131764 ) ) ;
#50529=CARTESIAN_POINT ( 'NONE',  ( 4.458734124999998549, -36.72916666530107221, -2.574251347313721627 ) ) ;
#50530=CARTESIAN_POINT ( 'NONE',  ( 5.000000000000000000, -60.41666666666665719, -2.886751345948130876 ) ) ;
#50532=LINE ( 'NONE', #5827, #40812 ) ;
#50538=CARTESIAN_POINT ( 'NONE',  ( -2.500000000000000444, -7.166666666666668739, -4.330127018922193649 ) ) ;
#50539=CARTESIAN_POINT ( 'NONE',  ( 4.458734125000000326, -70.89583333196773651, 2.574251347313718519 ) ) ;
#50540=CARTESIAN_POINT ( 'NONE',  ( -2.500000000000000444, -9.041666663935483683, -4.330127018922193649 ) ) ;
#50541=CARTESIAN_POINT ( 'NONE',  ( -2.229367062499996610, -38.14583333196773651, 3.861377020970582219 ) ) ;
#50542=ORIENTED_EDGE ( 'NONE', *, *, #50769, .T. ) ;
#50544=CARTESIAN_POINT ( 'NONE',  ( -4.458734124999999437, 12.35416666803225993, -2.574251347313719407 ) ) ;
#50547=CARTESIAN_POINT ( 'NONE',  ( -5.000000000000000000, -51.08333333333332860, -2.886751345948128211 ) ) ;
#50549=CARTESIAN_POINT ( 'NONE',  ( -2.499999999999996447, -34.83333333333332860, 4.330127018922195425 ) ) ;
#50550=CARTESIAN_POINT ( 'NONE',  ( 4.458734124999998549, -77.72916666530106511, -2.574251347313721627 ) ) ;
#50551=CARTESIAN_POINT ( 'NONE',  ( -8.190561711645485556E-16, -140.9375000013656063, 4.458734124999999437 ) ) ;
#50552=CARTESIAN_POINT ( 'NONE',  ( -2.229367062499996610, -85.14583333196773651, 3.861377020970582219 ) ) ;
#50554=CARTESIAN_POINT ( 'NONE',  ( -3.152548672688508926E-16, -35.81249999863440792, -5.148502694627439702 ) ) ;
#50556=CARTESIAN_POINT ( 'NONE',  ( -6.972266317189433020E-16, -38.12499999726880873, -5.000000000000000000 ) ) ;
#50557=VERTEX_POINT ( 'NONE', #56210 ) ;
#50562=( BOUNDED_SURFACE ( )  B_SPLINE_SURFACE ( 1, 2, ( 
 ( #53046, #52434, #8367, #8984, #23150, #42759, #37947, #57580, #33428, #33122, #38261, #52739, #28282, #57882, #28596, #43386, #44982, #49801, #9918, #53675, #29528, #59466, #5424, #25041, #9607, #44010, #44329, #14430, #24725, #24097, #38871, #29215, #15397, #63340, #25363, #34688, #24408, #39506, #4780, #40148, #63657, #10559, #10251, #34053, #19255, #58506, #19575, #949, #48841, #59142, #39823, #34360, #39189, #19891, #58814, #294, #35023, #15075, #14744, #15715, #53991, #54953, #10883, #35333, #4471, #54311, #20222, #49166, #5107, #29853, #49486, #44652, #613, #54636, #30170, #5745, #20550, #43692, #59793, #48530, #46579, #36292, #26960, #2520, #55284, #45621, #41101, #31448, #12157, #40469, #35977, #1577, #22136, #51090, #17300, #30499, #11827, #31138, #56235, #21178, #40784, #26002, #41731, #21505, #36928, #60431, #25689, #16357, #61379, #56555, #36603, #16031, #50121, #55605, #46257, #11522, #60109, #60746, #26315, #50762, #31776, #51407, #6706, #45298, #61067, #6077, #1263, #20866, #30826, #50456, #16670, #35659, #16988, #45934, #1897, #55915, #11204, #6396, #7027, #26638, #2216, #41417, #21819, #7350, #13423, #8290, #2838, #56870, #12787, #22456, #18248, #42369, #47821, #33047, #42683, #18567, #61697, #43314, #62949, #52662, #8597, #62326, #23402, #27894, #13734, #28207, #47516, #42054, #32409, #52039, #17627, #37874, #62009, #3780, #43002, #57507, #38189, #37244, #18865, #38483, #7979, #62647, #27270, #52971, #57811, #27577, #3467, #47210, #4095, #3154, #33356, #8911, #22774, #46897, #17927, #37549, #28525, #57190, #23080, #48142, #13110, #32727, #23717, #52354, #12476, #32088, #51724, #7664, #25283, #9222, #864, #20467, #44908, #14042, #219, #29776, #43619, #4705, #39114, #63261, #58742, #19180, #38793, #19817, #10171, #49409, #33667, #5030, #48458, #10484, #39426, #54561, #30096, #58431, #9535, #24649, #59067, #39743, #4396, #63580, #29140, #49727, #14992, #58111, #53286, #34604, #14669, #20147, #48762, #24330, #53602, #5672, #49082, #28835, #43933, #24016, #19500, #14360, #33981, #535, #34290, #53912, #9838, #5353, #29450, #44255, #54233, #24971, #44578, #59385, #15319, #34940, #54878, #6954, #46504, #7276, #36526, #40390, #60032, #26238, #26887, #26564, #11122, #35897, #1500, #31703, #50047, #12080, #35578, #50685, #41027, #51011, #6004, #21101, #55838, #20786, #16909, #40069, #2450, #36214, #1188, #11754, #59710, #6626, #15641, #15956, #51337, #31370, #55205, #46183, #30749, #40706, #45857, #35257, #2143, #60354, #16279, #11442, #21748, #25607, #41343, #55532, #10808, #30420, #50369, #1822, #60989, #31061, #6316, #56155, #45222, #25921, #21425, #45538, #60673, #16596, #32974, #51652, #23015, #41652, #8528, #7590, #28453, #28138, #13665, #56482, #32337, #48068, #52594, #27198, #18175, #46816, #61303, #57431, #3398, #62254, #18495, #23326, #47137, #2760, #3083, #47756, #42616, #37803, #22382, #17557, #17859, #41981, #61940, #17226, #12405, #8219, #13351, #61622, #3711, #37176, #56799, #36853, #33285, #12717, #57740, #52904, #38116, #32018, #42931, #62575, #51963, #8840, #27822, #57118, #7902, #22703, #37481, #13034, #27507, #22061, #42300, #32653, #52281, #47446, #4956, #58987, #34213, #23946, #34868, #14287, #58670, #43236, #20066, #19103, #4632, #62878, #14915, #54488, #38416, #48385, #34523, #28762, #29066, #14596, #39670, #29704, #48691, #24256, #39042, #49335, #53218, #54155, #63506, #59307, #18790, #38720, #53838, #10096, #43859, #4326, #19744, #39357, #9150, #19430, #464, #29375, #5279, #24899, #33597, #24577, #23642, #44500, #43548, #10416, #15242, #30027, #58041, #33906, #4023, #13971, #63193, #149, #58361, #53530, #9458, #49007, #44183, #9767, #50934, #11049, #54808, #30674, #60599, #6552, #26167, #10737, #45147, #45466, #15571, #25850, #25211, #39993, #35827, #45787, #30344, #1746, #49969, #5922, #44823, #41262, #25530, #21672, #60910, #2063, #20393, #11679, #55762, #1112, #21347, #55448, #21030, #20719, #50292, #1431, #40639, #59638, #36452, #40949, #40324, #5594, #59962, #50613, #16518, #16197, #15885, #16832, #35505, #60279, #785, #56954, #55124, #6240, #35190, #36140, #12875, #11363, #49656, #30987, #31297, #6874, #26489, #46105, #57592, #48223, #13194, #9304, #32493, #38883, #28607, #57276, #4180, #19266, #62726, #52123, #32817, #4481, #23795, #13520, #18012, #33137, #37636, #52445, #38272, #43397, #63042, #8066, #43087, #22862, #48542, #57896, #28919, #24109, #8380, #47601, #18650, #33439, #14126, #42453, #37958, #3554, #43705, #53057, #58517, #27668, #13820, #52751, #58197, #23162, #42771, #27981, #63352, #23484, #47296, #62415, #3248, #18335, #62095, #8681, #38568, #28295, #47907, #3863, #18950, #8995, #33752, #53370, #10263, #24737, #15727, #35346, #44340, #29226, #44995, #20878, #45310, #10895, #14755, #34372, #624, #1278, #961, #49178, #29865, #39516, #6088, #24420, #15412, #35035, #20234, #25374, #49497, #54965, #54647, #5435, #4794, #58825, #54001, #44021, #39835, #304, #49811, #10572, #44663, #20562, #63669, #40480, #14441, #9930, #40164, #48853, #30510, #59477, #29544, #25053, #5118, #25700, #19902, #59806, #30181, #19587, #39199, #59154, #15087, #50133, #34701, #5756, #34064, #54326, #53686, #9619, #26017, #55927, #46590, #11842, #1590, #27283, #11215, #2850, #22471, #46909, #16042, #2228, #31788, #45634, #6718, #12487, #30839, #22148, #2534, #11534, #51419, #21833, #31461, #35988, #21516, #51101, #7040, #50468, #60121, #7362, #55618, #35671, #31149, #61079, #26971, #26650, #16368, #55297, #26328, #46270, #6407, #32100, #50777, #60759, #21189, #41743, #40796, #60444, #51737, #45946, #41430, #17000, #61392, #1910, #41112, #12170, #16683, #36940, #36304, #36615, #56249, #17317, #56566, #7676, #8608, #42068, #22786, #14055, #57824, #42381, #8922, #3167, #3478, #52675, #33679, #4107, #23091, #42695, #13434, #23729, #27589, #33367, #37886, #53299, #17637, #13122, #28218, #48156, #62338, #62020, #13746, #52982, #47224, #18259, #38496, #3793, #43324, #28536, #7990, #43016, #61708, #62963, #17938, #48471, #18880, #9235, #12802, #52366, #4407, #58123, #37562, #38199, #57203, #37253, #28848, #23414, #18578, #56882, #32421, #57517, #32739, #33060, #52052, #62658, #8305, #27906, #47527, #47832, #53615, #231, #63273, #14370, #10185, #20157, #48774, #44589, #29153, #24344, #19192, #15651, #43945, #59723, #35268, #38805, #34953, #54890, #58444, #10819, #19512, #34618, #24982, #54572, #33994, #49096, #39753, #4719, #875, #24029, #30431, #59397, #63592, #15330, #50059, #54244, #43633, #39127, #9548, #10494, #58753, #30108, #14682, #5043, #29787, #34302, #49738, #24661, #44267, #59079, #5683, #53925, #25295, #19829, #9850, #29464, #39440, #49420, #44920, #15005, #5363, #20479, #40080, #547, #31072, #2459, #31383, #51347, #16919, #35590, #6965, #25620, #56168, #55216, #12414, #12091, #61314, #40402, #16290, #32026, #36536, #11134, #2153, #30760, #45232, #41354, #51021, #46193, #22070, #7286, #50696, #50381, #6639, #31713, #26575, #21759, #6327, #1510, #1833, #25932, #45869, #1199, #60042, #55848, #60997, #45551, #26897, #21113, #40718, #20799, #17239, #60366, #41662, #36863, #56493, #15966, #46515, #6016, #35910, #55542, #11764, #41038, #11453, #26247, #21434, #60684, #16606, #36224, #23336, #27516, #7601, #3094, #52602, #42938, #18184, #7911, #18798, #61949, #42625, #27208, #4030, #22711, #52290, #37184, #8227, #56809, #32348, #57439, #3718, #62581, #46826, #62264, #41993, #23649, #13359, #48076, #43245, #12726, #42309, #37811, #8536, #33291, #61633, #57128, #17868, #62885, #28146, #38422, #51662, #32982, #27832, #13672, #37489, #13044, #47146, #58048, #47763, #13978, #32662, #2771, #47454, #22392, #17566, #57748, #51972, #3406, #23022, #18503, #38124, #52910, #8847, #28461, #43866, #34877, #54498, #63514, #48391, #472, #40001, #795, #30036, #33914, #53539, #19753, #20402, #20074, #4639, #29382, #58679, #25221, #43554, #34530, #54163, #39364, #44510, #49016, #10423, #10104, #4964, #23950, #14295, #9465, #63200, #58995, #19438, #5289, #29712, #157, #39680, #19110, #59648, #33606, #29074, #59316, #4333, #49665, #14924, #48699, #24586, #24262, #44832, #39050, #15251, #49343, #38729, #58367, #14606, #34221, #5605, #53847, #44192, #24907, #9776, #53226, #9157, #28770, #11376, #2078, #30997, #20726, #46438, #30355, #21994, #41587, #2384, #35200, #21359, #50945, #1122, #25860, #60288, #35513, #15581, #45476, #6563, #54815, #31638, #30685, #16212, #10746, #26500, #49979, #5931, #51274, #11061, #26178, #16528, #46115, #25539, #40649, #31309, #59972, #56090, #45156, #40330, #11690, #15893, #6886, #55134, #45797, #50302, #6250, #7207, #21684, #1440, #41273, #21042, #35838, #1757, #26818, #60923, #55460, #50624, #40963, #16842, #60611, #36463, #36152, #55773, #12010, #32266, #47384, #3643, #42234, #61557, #13283, #32909, #2693, #22635, #57677, #22951, #42862, #8466, #27132, #62186, #17161, #47691, #46748, #3956, #23254, #52840, #31952, #7836, #23577, #28074, #22313, #57362, #41914, #36785, #52532, #42547, #37729, #13603, #62507, #61877, #17491, #17793, #18424, #18106, #38045, #37112, #56731, #57051, #12651, #37417, #56418, #51584, #3335, #33221, #51895, #8774, #27437, #47071, #12341, #28384, #3020, #48003, #61239, #7522, #12962, #32587, #52210, #8157, #27756, #48941, #14530, #19041, #4566, #58610, #38973, #33535, #29960, #14846, #38658, #62813, #58297, #44114, #34458, #9704, #57982, #13907, #14216, #59242, #9085, #53772, #54089, #29002, #33843, #34150, #28695, #29309, #29640, #4889, #48314, #10351, #53150, #49585, #5527, #43173, #18731, #24512, #10028, #4264, #53462, #24190, #23882, #43797, #43485, #63130, #77, #58917, #49274, #38356, #19678, #9391, #15174, #39290, #39606, #34799, #48627, #63444, #5210, #24829, #44435, #19361, #396, #19998, #54422, #45725, #11932, #25142, #6494, #25791, #50868, #40259, #35433, #20655, #16770, #16136, #31563, #59899, #20324, #15819, #36388, #60844, #31237, #10663, #56019, #55059, #40886, #10983, #54742, #35758, #20970, #30603, #26420, #46037, #50225, #39926, #55703, #51196, #44753, #21605, #25461, #45083, #11298, #714, #11617, #6174, #40571, #45402, #59573, #35127, #26105, #1677, #30923, #36074, #60212, #2001, #21279, #55382, #15506, #5853, #1049, #30279, #50550, #1368, #60531, #16455, #6811, #41199, #49899, #32831, #52459, #12265, #8081, #2313, #62109, #22560, #7449, #27363, #51512, #13209, #27057, #3263, #42160, #17090, #17416, #27683, #17722, #56970, #56344, #46675, #51818, #36711, #32187, #46360, #41514, #2945, #12888, #31878, #37337, #2620, #22238, #21917, #8395, #41838, #57293, #27996, #37650, #61167, #22875, #47310, #61483, #32507, #61796, #7760, #37031, #56657, #46997, #52139, #12574, #7128, #42468, #18028, #26744, #16022, #1889, #55908, #31130, #20859, #31767, #11194, #55595, #40140, #16979, #35649, #1568, #59784, #11819, #51399, #35326, #36590, #60101, #11514, #21493, #31438, #10874, #25993, #16659, #45291, #41407, #940, #7340, #60738, #25682, #36285, #26952, #50753, #20543, #1256, #56226, #51081, #40462, #7019, #55275, #45612, #6698, #12147, #26627, #21168, #40777, #35969, #46247, #50113, #2208, #60422, #15709, #54947, #30816, #26304, #21812, #16347, #50448, #61059, #30491, #6068, #45927, #6388, #41091, #26237, #45856, #59708, #30419, #34937, #50044, #54558, #30094, #55201, #1498, #21100, #5350, #60031, #39740, #1819, #11120, #21423, #41026, #10481, #863, #15954, #50368, #31060, #59381, #6003, #20785, #50682 ),
 ( #15315, #54876, #20466, #60670, #6315, #36212, #49406, #30748, #25606, #11441, #40066, #15640, #44905, #16594, #40389, #55836, #35256, #44574, #10807, #11750, #24968, #55530, #49724, #531, #45220, #40705, #1186, #5670, #35577, #25919, #45537, #6624, #20144, #60352, #25282, #16278, #35896, #62252, #27819, #31700, #51335, #17555, #18171, #61938, #2448, #27196, #56480, #23013, #41341, #32332, #51961, #37174, #42298, #46813, #32649, #7899, #2758, #21745, #12076, #7273, #60986, #56797, #61300, #3081, #27504, #61620, #37478, #16906, #37800, #57428, #26885, #17857, #46180, #8216, #12715, #46500, #22379, #22057, #42614, #41649, #57114, #47133, #36523, #2140, #56153, #17223, #36850, #12402, #22700, #51009, #13032, #32016, #31368, #52279, #6950, #51650, #7585, #26561, #47445, #41978, #3396, #42926, #52592, #48688, #58358, #53527, #9764, #14591, #38414, #18492, #58038, #24254, #33904, #9456, #38114, #8838, #9148, #62572, #53215, #8526, #3709, #63190, #29064, #57737, #4628, #13663, #33283, #28135, #4953, #52902, #49005, #24575, #29372, #47753, #39040, #19428, #28451, #43857, #19100, #48382, #48066, #13969, #28759, #4324, #23324, #147, #63504, #4020, #32970, #23640, #14285, #58668, #43545, #43234, #44180, #62876, #23944, #18787, #19742, #33595, #38718, #34211, #53836, #39354, #13349, #30985, #54486, #5920, #59960, #6238, #5276, #20390, #11046, #39668, #35823, #58985, #1744, #55122, #20063, #30671, #45784, #25527, #14912, #59305, #50610, #50290, #15238, #25847, #34865, #39990, #45145, #6550, #21028, #59636, #15568, #30341, #40636, #44498, #45464, #54806, #26165, #34521, #30025, #1108, #1429, #35188, #10413, #60276, #16195, #461, #10735, #15883, #49966, #20717, #49654, #5590, #49333, #40322, #25207, #55446, #35503, #11361, #21345, #44821, #54152, #10092, #783, #29702, #24897, #17781, #27120, #16830, #31941, #60908, #32574, #36449, #3006, #2679, #6872, #55759, #11676, #56078, #57035, #26487, #51569, #32252, #26802, #11998, #12330, #46102, #36774, #27425, #56405, #2061, #8141, #31295, #47372, #3321, #27743, #56717, #60596, #37400, #12949, #51261, #21981, #21669, #41575, #41260, #31625, #46733, #12635, #51882, #16516, #7508, #50931, #52195, #22299, #40946, #36138, #7195, #46423, #41899, #61545, #22623, #2372, #61226, #17150, #17477, #37099, #7822, #47056, #42219, #61865, #48614, #38033, #33209, #18413, #14515, #13895, #9690, #57665, #18091, #13591, #34136, #58596, #28990, #8455, #53756, #52827, #38643, #8762, #52520, #33521, #18719, #28368, #24177, #22940, #58284, #38344, #13269, #29298, #14203, #62494, #42534, #47989, #23868, #33829, #53138, #42851, #48927, #3943, #9071, #62170, #38959, #23564, #43160, #37714, #53447, #57352, #32892, #28061, #9379, #57971, #47678, #3630, #62800, #28681, #4553, #48301, #23237, #43783, #63430, #4253, #43471, #63117, #19029, #19346, #54075, #34445, #5834, #24497, #55041, #10014, #11285, #10967, #60200, #39275, #15161, #30911, #15804, #29625, #1035, #49258, #44101, #40245, #49884, #45068, #1353, #6160, #29946, #5197, #49571, #35421, #25448, #20639, #24815, #379, #699, #44418, #44738, #65, #58902, #54728, #59884, #19983, #30588, #39592, #59228, #19662, #16117, #34783, #40557, #35744, #20956, #14831, #50210, #25777, #54406, #45387, #10648, #30262, #55370, #4876, #10336, #20311, #5511, #25125, #39911, #59557, #15491, #35112, #51496, #41822, #17075, #6797, #17709, #60831, #41500, #26089, #2930, #1986, #51182, #45711, #61468, #37323, #21265, #22544, #46024, #61153, #7433, #17401, #60514, #11918, #2605, #31223, #27349, #50538, #56953, #46660, #11603, #22224, #12874, #36694, #6481, #50854, #42144, #37016, #26405, #56644, #21588, #31544, #56328, #61781, #12558, #7113, #26728, #21903, #32171, #36061, #46344, #41186, #51804, #1664, #40870, #46983, #16757, #36373, #12250, #16441, #7746, #56004, #2301, #31863, #55690, #27043, #33438, #53056, #18649, #43396, #28294, #33751, #8994, #47906, #22861, #13193, #32816, #42452, #38271, #62414, #4179, #28606, #62725, #38567, #18011, #63351, #19265, #52444, #63041, #47295, #9303, #57895, #8379, #23483, #27980, #24108, #47600, #58196, #13819, #62094, #3247, #37635, #3553, #48541, #57275, #43086, #23794, #18334, #23161, #3862, #42770, #48222, #18949, #14125, #37957, #38882, #57591, #58516, #32492, #52122, #53369, #8065, #28918, #4480, #13519, #33136, #52750, #8680, #43704, #27667, #20233, #30180, #49810, #34063, #25052, #4793, #30509, #39834, #10894, #50132, #39198, #29543, #44662, #15411, #59805, #24419, #19901, #49177, #6087, #35034, #1277, #14440, #59476, #15086, #40163, #5117, #24736, #9929, #25699, #5434, #20877, #44339, #9618, #303, #45309, #40479, #20561, #63668, #53685, #39515, #5755, #59153, #44020, #623, #10262, #34700, #15726, #29225, #34371, #48852, #54325, #54646, #19586, #58824, #29864, #49496, #14754, #25373, #54000, #10571, #44994, #960, #35345, #54964, #7361, #6406, #21515, #12169, #40795, #36939, #60120, #2849, #56248, #21188, #31787, #46908, #26649, #16041, #60443, #32099, #51418, #16367, #26970, #35987, #41111, #7039, #51736, #22147, #60758, #16682, #31460, #41742, #45633, #46589, #55926, #7675, #35670, #31148, #46269, #2533, #36303, #55617, #61391, #17316, #1589, #11841, #16999, #51100, #2227, #11533, #26016, #61078, #55296, #56565, #50776, #22470, #12486, #27282, #30838, #6717, #11214, #50467, #26327, #45945, #1909, #21832, #41429, #36614, #18577, #38495, #43323, #3477, #47223, #23090, #52981, #62657, #38198, #3166, #37561, #37885, #7989, #18258, #17636, #32420, #28217, #57823, #22785, #13745, #42380, #62019, #37252, #33678, #17937, #14054, #53298, #58122, #12801, #4106, #48155, #57202, #33366, #47831, #3792, #9234, #42067, #8921, #57516, #52051, #28847, #28535, #13121, #61707, #32738, #43015, #23728, #8607, #52365, #62962, #48470, #4406, #56881, #8304, #27905, #23413, #27588, #18879, #47526, #13433, #42694, #62337, #33059, #52674, #45471, #10184, #35833, #19828, #26172, #25855, #39439, #14369, #4718, #24343, #33993, #30679, #53924, #60283, #1436, #54243, #30993, #9547, #55768, #11685, #43944, #55454, #38804, #1752, #50298, #63591, #15004, #19511, #16524, #39126, #50619, #6245, #53614, #58443, #29152, #58752, #40958, #48773, #34617, #16205, #9849, #14681, #59078, #34301, #21037, #11370, #40644, #29463, #31303, #49095, #50939, #24028, #43632, #6558, #63272, #21353, #60606, #5042, #24660, #44266, #230, #45792, #36147, #19191, #22630, #42229, #26494, #17486, #60918, #22947, #12646, #3330, #42542, #31633, #21989, #37107, #7831, #52204, #16838, #12337, #41582, #62181, #27432, #57357, #6881, #51890, #7517, #32582, #61234, #17157, #2379, #18101, #61553, #13278, #36780, #2072, #56413, #37724, #32903, #12957, #56085, #46110, #31948, #61873, #51579, #36458, #56726, #2688, #27127, #8151, #21678, #46743, #7202, #32261, #41268, #37411, #22308, #41907, #47065, #12005, #51269, #3015, #17788, #57046, #27751, #47379, #26812, #46432, #48310, #42857, #33218, #52836, #62502, #58292, #18727, #24186, #9388, #19037, #58607, #38041, #19674, #39286, #8770, #19356, #3637, #29307, #38654, #28379, #43481, #48000, #44110, #3952, #14526, #14211, #18420, #23249, #57673, #23574, #4885, #13599, #63126, #43793, #38352, #43169, #23877, #62808, #4260, #38969, #33839, #57978, #58913, #13903, #14841, #52527, #8461, #4562, #28069, #48937, #24507, #33531, #53146, #9081, #28690, #53457, #28998, #48623, #63440, #34146, #47686, #53767, #9700, #73, #40255, #30920, #6491, #59238, #49581, #45078, #35431, #16133, #44431, #39921, #5523, #26101, #55056, #21276, #34454, #15816, #35123, #60209, #25138, #44749, #29956, #45722, #25458, #40883, #710, #29636, #20320, #1674, #60527, #40568, #19994, #54086, #59569, #50221, #15501, #392, #1045, #30275, #54738, #35755, #50547, #10659, #54417, #1365, #10024, #49270, #5206, #34795, #10980, #49895, #24825, #15171, #10346, #39602, #59896, #5848, #6171, #30600, #20651, #55379, #25788, #45399, #20968, #11295, #46993, #31234, #56966, #2616, #56015, #7445, #36384, #8077, #11927, #42156, #41834, #46034, #50864, #6808, #31559, #32503, #1997, #27053, #7756, #2310, #51192, #51508, #21602, #12260, #2941, #31874, #41196, #47305, #26417, #22871, #42464, #3259, #32183, #36071, #12885, #52135, #26740, #61163, #60841, #17086, #16767, #7124, #22234, #51814, #27359, #55700, #46671, #46356, #27678, #61478, #16452, #11614, #21913, #41510, #17412, #37027, #61792, #36706, #56340, #56653, #12570, #22554, #17719, #37333, #43407, #62738, #24119, #13529, #8692, #57602, #53698, #53067, #48863, #33148, #57289, #52763, #9630, #34075, #4491, #47611, #29238, #28304, #14136, #47918, #27992, #9007, #57907, #3876, #43718, #14453, #43097, #18346, #28929, #4807, #24431, #58529, #62428, #37969, #48234, #62105, #48552, #23495, #13831, #18660, #18024, #8390, #63052, #18962, #4192, #9315, #33450, #63364, #37646, #13205, #19279, #3565, #32827, #38282, #33763, #28619, #23172, #23805, #38578, #58209, #38894, #52456, #53382, #42783, #10905, #50478, #11224, #40491, #44352, #315, #30193, #30847, #30520, #15097, #39846, #5446, #35681, #54012, #45005, #971, #49822, #54976, #59489, #45323, #20573, #15424, #34384, #24747, #19913, #9942, #5766, #10273, #15738, #40179, #10581, #50143, #29557, #6418, #44033, #39527, #6098, #58837, #20888, #25384, #59165, #35046, #34714, #55309, #54340, #25711, #59816, #49191, #14766, #5129, #29877, #60132, #49507, #54658, #35355, #25064, #44674, #1290, #634, #16053, #10226, #19600, #20244, #39212, #40805, #32431, #52060, #12810, #41752, #45643, #2859, #22481, #36313, #7048, #11543, #26661, #31160, #6728, #31796, #61402, #17326, #1601, #36625, #16378, #42076, #51428, #61717, #17646, #50789, #41121, #56257, #26979, #7686, #35997, #31470, #60769, #37262, #46598, #26027, #21199, #7371, #46279, #51744, #16694, #55937, #21525, #56890, #17009, #60453, #11852, #55628, #51111, #2238, #26338, #21842, #45955, #1920, #2542, #36948, #56574, #41438, #12182, #61087, #22158, #12496, #32108, #27292, #46917, #23100, #18585, #8930, #53308, #17946, #13445, #42703, #43642, #28543, #58455, #7998, #52989, #8618, #33687, #62347, #18268, #3486, #63283, #62665, #14378, #37895, #3176, #57524, #19200, #38813, #14062, #57211, #34002, #33070, #23736, #52683, #37571, #38209, #3801, #28226, #9242, #24040, #47842, #27914, #38503, #27601, #47234, #4415, #8314, #47536, #57834, #22796, #58131, #23422, #43025, #13753, #42389, #13130, #48163, #4116, #33375, #18889, #43331, #28856, #62973, #48478, #62029, #52377, #32749, #43953, #59407, #19837, #25305, #10500, #20165, #59730, #39135, #20805, #40408, #34310, #20489, #4728, #30438, #39761, #29473, #44596, #9863, #45240, #49105, #15656, #15339, #19521, #24353, #63601, #5051, #6021, #58762, #556, #44926, #39451, #24669, #24989, #14692, #49427, #40087, #5371, #53933, #60047, #44277, #15971, #53625, #9556, #5689, #29161, #50066, #25626, #239, #48786, #881, #34962, #59087, #15013, #35274, #34628, #54253, #10194, #54578, #54896, #30115, #29794, #49745, #10825, #1206, #11142, #51668, #50704, #36231, #30766, #46523, #2780, #6335, #7610, #31081, #46200, #36544, #2465, #45558, #60692, #51354, #16296, #12421, #35598, #41999, #31720, #60373, #7293, #22400, #2160, #55222, #35919, #27215, #26903, #55548, #22076, #11459, #16612, #21767, #46832, #61322, #55858, #11772, #6971, #17245, #21119, #41672, #31390, #61640, #50387, #6646, #41360, #36869, #51029, #26253, #56499, #32033, #40726, #26581, #56176, #61004, #16929, #45876, #1516, #12097 ) ),
 .UNSPECIFIED., .F., .F., .F. ) 
 B_SPLINE_SURFACE_WITH_KNOTS ( ( 2, 2 ),
 ( 3, 2, 2, 2, 2, 2, 2, 2, 2, 2, 2, 2, 2, 2, 2, 2, 2, 2, 2, 2, 2, 2, 2, 2, 2, 2, 2, 2, 2, 2, 2, 2, 2, 2, 2, 2, 2, 2, 2, 2, 2, 2, 2, 2, 2, 2, 2, 2, 2, 2, 2, 2, 2, 2, 2, 2, 2, 2, 2, 2, 2, 2, 2, 2, 2, 2, 2, 2, 2, 2, 2, 2, 2, 2, 2, 2, 2, 2, 2, 2, 2, 2, 2, 2, 2, 2, 2, 2, 2, 2, 2, 2, 2, 2, 2, 2, 2, 2, 2, 2, 2, 2, 2, 2, 2, 2, 2, 2, 2, 2, 2, 2, 2, 2, 2, 2, 2, 2, 2, 2, 2, 2, 2, 2, 2, 2, 2, 2, 2, 2, 2, 2, 2, 2, 2, 2, 2, 2, 2, 2, 2, 2, 2, 2, 2, 2, 2, 2, 2, 2, 2, 2, 2, 2, 2, 2, 2, 2, 2, 2, 2, 2, 2, 2, 2, 2, 2, 2, 2, 2, 2, 2, 2, 2, 2, 2, 2, 2, 2, 2, 2, 2, 2, 2, 2, 2, 2, 2, 2, 2, 2, 2, 2, 2, 2, 2, 2, 2, 2, 2, 2, 2, 2, 2, 2, 2, 2, 2, 2, 2, 2, 2, 2, 2, 2, 2, 2, 2, 2, 2, 2, 2, 2, 2, 2, 2, 2, 2, 2, 2, 2, 2, 2, 2, 2, 2, 2, 2, 2, 2, 2, 2, 2, 2, 2, 2, 2, 2, 2, 2, 2, 2, 2, 2, 2, 2, 2, 2, 2, 2, 2, 2, 2, 2, 2, 2, 2, 2, 2, 2, 2, 2, 2, 2, 2, 2, 2, 2, 2, 2, 2, 2, 2, 2, 2, 2, 2, 2, 2, 2, 2, 2, 2, 2, 2, 2, 2, 2, 2, 2, 2, 2, 2, 2, 2, 2, 2, 2, 2, 2, 2, 2, 2, 2, 2, 2, 2, 2, 2, 2, 2, 2, 2, 2, 2, 2, 2, 2, 2, 2, 2, 2, 2, 2, 2, 2, 2, 2, 2, 2, 2, 2, 2, 2, 2, 2, 2, 2, 2, 2, 2, 2, 2, 2, 2, 2, 2, 2, 2, 2, 2, 2, 2, 2, 2, 2, 2, 2, 2, 2, 2, 2, 2, 2, 2, 2, 2, 2, 2, 2, 2, 2, 2, 2, 2, 2, 2, 2, 2, 2, 2, 2, 2, 2, 2, 2, 2, 2, 2, 2, 2, 2, 2, 2, 2, 2, 2, 2, 2, 2, 2, 2, 2, 2, 2, 2, 2, 2, 2, 2, 2, 2, 2, 2, 2, 2, 2, 2, 2, 2, 2, 2, 2, 2, 2, 2, 2, 2, 2, 2, 2, 2, 2, 2, 2, 2, 2, 2, 2, 2, 2, 2, 2, 2, 2, 2, 2, 2, 2, 2, 2, 2, 2, 2, 2, 2, 2, 2, 2, 2, 2, 2, 2, 2, 2, 2, 2, 2, 2, 2, 2, 2, 2, 2, 2, 2, 2, 2, 2, 2, 2, 2, 2, 2, 2, 2, 2, 2, 2, 2, 2, 2, 2, 2, 2, 2, 2, 2, 2, 2, 2, 2, 2, 2, 2, 2, 2, 2, 2, 2, 2, 2, 2, 2, 2, 2, 2, 2, 2, 2, 2, 2, 2, 2, 2, 2, 2, 2, 2, 2, 2, 2, 2, 2, 2, 2, 2, 2, 2, 2, 2, 2, 2, 2, 2, 2, 2, 2, 2, 2, 2, 2, 2, 2, 2, 2, 2, 2, 2, 2, 2, 2, 2, 2, 2, 2, 2, 2, 2, 2, 2, 2, 2, 2, 2, 2, 2, 2, 2, 2, 2, 2, 2, 2, 2, 2, 2, 2, 2, 2, 2, 2, 2, 2, 2, 2, 2, 2, 2, 2, 2, 2, 2, 2, 2, 2, 2, 2, 2, 2, 2, 2, 2, 2, 2, 2, 2, 2, 2, 2, 2, 2, 2, 2, 2, 2, 2, 2, 2, 2, 2, 2, 2, 2, 2, 2, 2, 2, 2, 2, 2, 2, 2, 2, 2, 2, 2, 2, 2, 2, 2, 2, 2, 2, 2, 2, 2, 2, 2, 2, 2, 2, 2, 2, 2, 2, 2, 2, 2, 2, 2, 2, 2, 2, 2, 2, 2, 2, 2, 2, 2, 2, 2, 2, 2, 2, 2, 2, 2, 2, 2, 2, 2, 2, 2, 2, 2, 2, 2, 2, 2, 2, 2, 2, 2, 2, 2, 2, 2, 2, 3 ),
 ( 0.000000000000000000, 1.000000000000000000 ),
 ( 0.000000000000000000, 0.001388888888888888942, 0.002777777777777777884, 0.004166666666666666609, 0.005555555555555555768, 0.006944444444444444059, 0.008333333333333333218, 0.009722222222222222376, 0.01111111111111111154, 0.01250000000000000069, 0.01388888888888888812, 0.01527777777777777728, 0.01666666666666666644, 0.01805555555555555386, 0.01944444444444444475, 0.02083333333333333218, 0.02222222222222222307, 0.02361111111111111049, 0.02500000000000000139, 0.02638888888888888881, 0.02777777777777777624, 0.02916666666666666713, 0.03055555555555555455, 0.03194444444444444198, 0.03333333333333333287, 0.03472222222222222376, 0.03611111111111110772, 0.03749999999999999861, 0.03888888888888888951, 0.04027777777777778040, 0.04166666666666666435, 0.04305555555555555525, 0.04444444444444444614, 0.04583333333333333010, 0.04722222222222222099, 0.04861111111111111188, 0.05000000000000000278, 0.05138888888888888673, 0.05277777777777777762, 0.05416666666666666852, 0.05555555555555555247, 0.05694444444444444337, 0.05833333333333333426, 0.05972222222222222515, 0.06111111111111110911, 0.06250000000000000000, 0.06388888888888888395, 0.06527777777777778179, 0.06666666666666666574, 0.06805555555555554970, 0.06944444444444444753, 0.07083333333333333148, 0.07222222222222221544, 0.07361111111111111327, 0.07499999999999999722, 0.07638888888888889506, 0.07777777777777777901, 0.07916666666666666297, 0.08055555555555556080, 0.08194444444444444475, 0.08333333333333332871, 0.08472222222222222654, 0.08611111111111111049, 0.08749999999999999445, 0.08888888888888889228, 0.09027777777777777624, 0.09166666666666666019, 0.09305555555555555802, 0.09444444444444444198, 0.09583333333333333981, 0.09722222222222222376, 0.09861111111111110772, 0.1000000000000000056, 0.1013888888888888895, 0.1027777777777777735, 0.1041666666666666713, 0.1055555555555555552, 0.1069444444444444392, 0.1083333333333333370, 0.1097222222222222210, 0.1111111111111111049, 0.1125000000000000028, 0.1138888888888888867, 0.1152777777777777846, 0.1166666666666666685, 0.1180555555555555525, 0.1194444444444444503, 0.1208333333333333343, 0.1222222222222222182, 0.1236111111111111160, 0.1250000000000000000, 0.1263888888888888840, 0.1277777777777777679, 0.1291666666666666796, 0.1305555555555555636, 0.1319444444444444475, 0.1333333333333333315, 0.1347222222222222154, 0.1361111111111110994, 0.1375000000000000111, 0.1388888888888888951, 0.1402777777777777790, 0.1416666666666666630, 0.1430555555555555469, 0.1444444444444444309, 0.1458333333333333426, 0.1472222222222222265, 0.1486111111111111105, 0.1499999999999999944, 0.1513888888888888784, 0.1527777777777777901, 0.1541666666666666741, 0.1555555555555555580, 0.1569444444444444420, 0.1583333333333333259, 0.1597222222222222099, 0.1611111111111111216, 0.1625000000000000056, 0.1638888888888888895, 0.1652777777777777735, 0.1666666666666666574, 0.1680555555555555691, 0.1694444444444444531, 0.1708333333333333370, 0.1722222222222222210, 0.1736111111111111049, 0.1749999999999999889, 0.1763888888888889006, 0.1777777777777777846, 0.1791666666666666685, 0.1805555555555555525, 0.1819444444444444364, 0.1833333333333333204, 0.1847222222222222321, 0.1861111111111111160, 0.1875000000000000000, 0.1888888888888888840, 0.1902777777777777679, 0.1916666666666666796, 0.1930555555555555636, 0.1944444444444444475, 0.1958333333333333315, 0.1972222222222222154, 0.1986111111111110994, 0.2000000000000000111, 0.2013888888888888951, 0.2027777777777777790, 0.2041666666666666630, 0.2055555555555555469, 0.2069444444444444309, 0.2083333333333333426, 0.2097222222222222265, 0.2111111111111111105, 0.2124999999999999944, 0.2138888888888888784, 0.2152777777777777901, 0.2166666666666666741, 0.2180555555555555580, 0.2194444444444444420, 0.2208333333333333259, 0.2222222222222222099, 0.2236111111111111216, 0.2250000000000000056, 0.2263888888888888895, 0.2277777777777777735, 0.2291666666666666574, 0.2305555555555555691, 0.2319444444444444531, 0.2333333333333333370, 0.2347222222222222210, 0.2361111111111111049, 0.2374999999999999889, 0.2388888888888889006, 0.2402777777777777846, 0.2416666666666666685, 0.2430555555555555525, 0.2444444444444444364, 0.2458333333333333204, 0.2472222222222222321, 0.2486111111111111160, 0.2500000000000000000, 0.2513888888888888840, 0.2527777777777777679, 0.2541666666666666519, 0.2555555555555555358, 0.2569444444444444198, 0.2583333333333333592, 0.2597222222222222432, 0.2611111111111111271, 0.2625000000000000111, 0.2638888888888888951, 0.2652777777777777790, 0.2666666666666666630, 0.2680555555555555469, 0.2694444444444444309, 0.2708333333333333148, 0.2722222222222221988, 0.2736111111111111382, 0.2750000000000000222, 0.2763888888888889062, 0.2777777777777777901, 0.2791666666666666741, 0.2805555555555555580, 0.2819444444444444420, 0.2833333333333333259, 0.2847222222222222099, 0.2861111111111110938, 0.2874999999999999778, 0.2888888888888888618, 0.2902777777777778012, 0.2916666666666666852, 0.2930555555555555691, 0.2944444444444444531, 0.2958333333333333370, 0.2972222222222222210, 0.2986111111111111049, 0.2999999999999999889, 0.3013888888888888729, 0.3027777777777777568, 0.3041666666666666408, 0.3055555555555555802, 0.3069444444444444642, 0.3083333333333333481, 0.3097222222222222321, 0.3111111111111111160, 0.3125000000000000000, 0.3138888888888888840, 0.3152777777777777679, 0.3166666666666666519, 0.3180555555555555358, 0.3194444444444444198, 0.3208333333333333592, 0.3222222222222222432, 0.3236111111111111271, 0.3250000000000000111, 0.3263888888888888951, 0.3277777777777777790, 0.3291666666666666630, 0.3305555555555555469, 0.3319444444444444309, 0.3333333333333333148, 0.3347222222222221988, 0.3361111111111111382, 0.3375000000000000222, 0.3388888888888889062, 0.3402777777777777901, 0.3416666666666666741, 0.3430555555555555580, 0.3444444444444444420, 0.3458333333333333259, 0.3472222222222222099, 0.3486111111111110938, 0.3499999999999999778, 0.3513888888888888618, 0.3527777777777778012, 0.3541666666666666852, 0.3555555555555555691, 0.3569444444444444531, 0.3583333333333333370, 0.3597222222222222210, 0.3611111111111111049, 0.3624999999999999889, 0.3638888888888888729, 0.3652777777777777568, 0.3666666666666666408, 0.3680555555555555802, 0.3694444444444444642, 0.3708333333333333481, 0.3722222222222222321, 0.3736111111111111160, 0.3750000000000000000, 0.3763888888888888840, 0.3777777777777777679, 0.3791666666666666519, 0.3805555555555555358, 0.3819444444444444198, 0.3833333333333333592, 0.3847222222222222432, 0.3861111111111111271, 0.3875000000000000111, 0.3888888888888888951, 0.3902777777777777790, 0.3916666666666666630, 0.3930555555555555469, 0.3944444444444444309, 0.3958333333333333148, 0.3972222222222221988, 0.3986111111111111382, 0.4000000000000000222, 0.4013888888888889062, 0.4027777777777777901, 0.4041666666666666741, 0.4055555555555555580, 0.4069444444444444420, 0.4083333333333333259, 0.4097222222222222099, 0.4111111111111110938, 0.4124999999999999778, 0.4138888888888888618, 0.4152777777777778012, 0.4166666666666666852, 0.4180555555555555691, 0.4194444444444444531, 0.4208333333333333370, 0.4222222222222222210, 0.4236111111111111049, 0.4249999999999999889, 0.4263888888888888729, 0.4277777777777777568, 0.4291666666666666408, 0.4305555555555555802, 0.4319444444444444642, 0.4333333333333333481, 0.4347222222222222321, 0.4361111111111111160, 0.4375000000000000000, 0.4388888888888888840, 0.4402777777777777679, 0.4416666666666666519, 0.4430555555555555358, 0.4444444444444444198, 0.4458333333333333592, 0.4472222222222222432, 0.4486111111111111271, 0.4500000000000000111, 0.4513888888888888951, 0.4527777777777777790, 0.4541666666666666630, 0.4555555555555555469, 0.4569444444444444309, 0.4583333333333333148, 0.4597222222222221988, 0.4611111111111111382, 0.4625000000000000222, 0.4638888888888889062, 0.4652777777777777901, 0.4666666666666666741, 0.4680555555555555580, 0.4694444444444444420, 0.4708333333333333259, 0.4722222222222222099, 0.4736111111111110938, 0.4749999999999999778, 0.4763888888888888618, 0.4777777777777778012, 0.4791666666666666852, 0.4805555555555555691, 0.4819444444444444531, 0.4833333333333333370, 0.4847222222222222210, 0.4861111111111111049, 0.4874999999999999889, 0.4888888888888888729, 0.4902777777777777568, 0.4916666666666666408, 0.4930555555555555802, 0.4944444444444444642, 0.4958333333333333481, 0.4972222222222222321, 0.4986111111111111160, 0.5000000000000000000, 0.5013888888888888840, 0.5027777777777777679, 0.5041666666666666519, 0.5055555555555555358, 0.5069444444444444198, 0.5083333333333333037, 0.5097222222222221877, 0.5111111111111110716, 0.5124999999999999556, 0.5138888888888888395, 0.5152777777777777235, 0.5166666666666667185, 0.5180555555555556024, 0.5194444444444444864, 0.5208333333333333703, 0.5222222222222222543, 0.5236111111111111382, 0.5250000000000000222, 0.5263888888888889062, 0.5277777777777777901, 0.5291666666666666741, 0.5305555555555555580, 0.5319444444444444420, 0.5333333333333333259, 0.5347222222222222099, 0.5361111111111110938, 0.5374999999999999778, 0.5388888888888888618, 0.5402777777777777457, 0.5416666666666666297, 0.5430555555555555136, 0.5444444444444443976, 0.5458333333333332815, 0.5472222222222222765, 0.5486111111111111605, 0.5500000000000000444, 0.5513888888888889284, 0.5527777777777778123, 0.5541666666666666963, 0.5555555555555555802, 0.5569444444444444642, 0.5583333333333333481, 0.5597222222222222321, 0.5611111111111111160, 0.5625000000000000000, 0.5638888888888888840, 0.5652777777777777679, 0.5666666666666666519, 0.5680555555555555358, 0.5694444444444444198, 0.5708333333333333037, 0.5722222222222221877, 0.5736111111111110716, 0.5749999999999999556, 0.5763888888888888395, 0.5777777777777777235, 0.5791666666666667185, 0.5805555555555556024, 0.5819444444444444864, 0.5833333333333333703, 0.5847222222222222543, 0.5861111111111111382, 0.5875000000000000222, 0.5888888888888889062, 0.5902777777777777901, 0.5916666666666666741, 0.5930555555555555580, 0.5944444444444444420, 0.5958333333333333259, 0.5972222222222222099, 0.5986111111111110938, 0.5999999999999999778, 0.6013888888888888618, 0.6027777777777777457, 0.6041666666666666297, 0.6055555555555555136, 0.6069444444444443976, 0.6083333333333332815, 0.6097222222222222765, 0.6111111111111111605, 0.6125000000000000444, 0.6138888888888889284, 0.6152777777777778123, 0.6166666666666666963, 0.6180555555555555802, 0.6194444444444444642, 0.6208333333333333481, 0.6222222222222222321, 0.6236111111111111160, 0.6250000000000000000, 0.6263888888888888840, 0.6277777777777777679, 0.6291666666666666519, 0.6305555555555555358, 0.6319444444444444198, 0.6333333333333333037, 0.6347222222222221877, 0.6361111111111110716, 0.6374999999999999556, 0.6388888888888888395, 0.6402777777777777235, 0.6416666666666667185, 0.6430555555555556024, 0.6444444444444444864, 0.6458333333333333703, 0.6472222222222222543, 0.6486111111111111382, 0.6500000000000000222, 0.6513888888888889062, 0.6527777777777777901, 0.6541666666666666741, 0.6555555555555555580, 0.6569444444444444420, 0.6583333333333333259, 0.6597222222222222099, 0.6611111111111110938, 0.6624999999999999778, 0.6638888888888888618, 0.6652777777777777457, 0.6666666666666666297, 0.6680555555555555136, 0.6694444444444443976, 0.6708333333333332815, 0.6722222222222222765, 0.6736111111111111605, 0.6750000000000000444, 0.6763888888888889284, 0.6777777777777778123, 0.6791666666666666963, 0.6805555555555555802, 0.6819444444444444642, 0.6833333333333333481, 0.6847222222222222321, 0.6861111111111111160, 0.6875000000000000000, 0.6888888888888888840, 0.6902777777777777679, 0.6916666666666666519, 0.6930555555555555358, 0.6944444444444444198, 0.6958333333333333037, 0.6972222222222221877, 0.6986111111111110716, 0.6999999999999999556, 0.7013888888888888395, 0.7027777777777777235, 0.7041666666666667185, 0.7055555555555556024, 0.7069444444444444864, 0.7083333333333333703, 0.7097222222222222543, 0.7111111111111111382, 0.7125000000000000222, 0.7138888888888889062, 0.7152777777777777901, 0.7166666666666666741, 0.7180555555555555580, 0.7194444444444444420, 0.7208333333333333259, 0.7222222222222222099, 0.7236111111111110938, 0.7249999999999999778, 0.7263888888888888618, 0.7277777777777777457, 0.7291666666666666297, 0.7305555555555555136, 0.7319444444444443976, 0.7333333333333332815, 0.7347222222222222765, 0.7361111111111111605, 0.7375000000000000444, 0.7388888888888889284, 0.7402777777777778123, 0.7416666666666666963, 0.7430555555555555802, 0.7444444444444444642, 0.7458333333333333481, 0.7472222222222222321, 0.7486111111111111160, 0.7500000000000000000, 0.7513888888888888840, 0.7527777777777777679, 0.7541666666666666519, 0.7555555555555555358, 0.7569444444444444198, 0.7583333333333333037, 0.7597222222222221877, 0.7611111111111110716, 0.7624999999999999556, 0.7638888888888888395, 0.7652777777777777235, 0.7666666666666667185, 0.7680555555555556024, 0.7694444444444444864, 0.7708333333333333703, 0.7722222222222222543, 0.7736111111111111382, 0.7750000000000000222, 0.7763888888888889062, 0.7777777777777777901, 0.7791666666666666741, 0.7805555555555555580, 0.7819444444444444420, 0.7833333333333333259, 0.7847222222222222099, 0.7861111111111110938, 0.7874999999999999778, 0.7888888888888888618, 0.7902777777777777457, 0.7916666666666666297, 0.7930555555555555136, 0.7944444444444443976, 0.7958333333333332815, 0.7972222222222222765, 0.7986111111111111605, 0.8000000000000000444, 0.8013888888888889284, 0.8027777777777778123, 0.8041666666666666963, 0.8055555555555555802, 0.8069444444444444642, 0.8083333333333333481, 0.8097222222222222321, 0.8111111111111111160, 0.8125000000000000000, 0.8138888888888888840, 0.8152777777777777679, 0.8166666666666666519, 0.8180555555555555358, 0.8194444444444444198, 0.8208333333333333037, 0.8222222222222221877, 0.8236111111111110716, 0.8249999999999999556, 0.8263888888888888395, 0.8277777777777777235, 0.8291666666666667185, 0.8305555555555556024, 0.8319444444444444864, 0.8333333333333333703, 0.8347222222222222543, 0.8361111111111111382, 0.8375000000000000222, 0.8388888888888889062, 0.8402777777777777901, 0.8416666666666666741, 0.8430555555555555580, 0.8444444444444444420, 0.8458333333333333259, 0.8472222222222222099, 0.8486111111111110938, 0.8499999999999999778, 0.8513888888888888618, 0.8527777777777777457, 0.8541666666666666297, 0.8555555555555555136, 0.8569444444444443976, 0.8583333333333332815, 0.8597222222222222765, 0.8611111111111111605, 0.8625000000000000444, 0.8638888888888889284, 0.8652777777777778123, 0.8666666666666666963, 0.8680555555555555802, 0.8694444444444444642, 0.8708333333333333481, 0.8722222222222222321, 0.8736111111111111160, 0.8750000000000000000, 0.8763888888888888840, 0.8777777777777777679, 0.8791666666666666519, 0.8805555555555555358, 0.8819444444444444198, 0.8833333333333333037, 0.8847222222222221877, 0.8861111111111110716, 0.8874999999999999556, 0.8888888888888888395, 0.8902777777777777235, 0.8916666666666667185, 0.8930555555555556024, 0.8944444444444444864, 0.8958333333333333703, 0.8972222222222222543, 0.8986111111111111382, 0.9000000000000000222, 0.9013888888888889062, 0.9027777777777777901, 0.9041666666666666741, 0.9055555555555555580, 0.9069444444444444420, 0.9083333333333333259, 0.9097222222222222099, 0.9111111111111110938, 0.9124999999999999778, 0.9138888888888888618, 0.9152777777777777457, 0.9166666666666666297, 0.9180555555555555136, 0.9194444444444443976, 0.9208333333333332815, 0.9222222222222222765, 0.9236111111111111605, 0.9250000000000000444, 0.9263888888888889284, 0.9277777777777778123, 0.9291666666666666963, 0.9305555555555555802, 0.9319444444444444642, 0.9333333333333333481, 0.9347222222222222321, 0.9361111111111111160, 0.9375000000000000000, 0.9388888888888888840, 0.9402777777777777679, 0.9416666666666666519, 0.9430555555555555358, 0.9444444444444444198, 0.9458333333333333037, 0.9472222222222221877, 0.9486111111111110716, 0.9499999999999999556, 0.9513888888888888395, 0.9527777777777777235, 0.9541666666666667185, 0.9555555555555556024, 0.9569444444444444864, 0.9583333333333333703, 0.9597222222222222543, 0.9611111111111111382, 0.9625000000000000222, 0.9638888888888889062, 0.9652777777777777901, 0.9666666666666666741, 0.9680555555555555580, 0.9694444444444444420, 0.9708333333333333259, 0.9722222222222222099, 0.9736111111111110938, 0.9749999999999999778, 0.9763888888888888618, 0.9777777777777777457, 0.9791666666666666297, 0.9805555555555555136, 0.9819444444444443976, 0.9833333333333332815, 0.9847222222222222765, 0.9861111111111111605, 0.9875000000000000444, 0.9888888888888889284, 0.9902777777777778123, 0.9916666666666666963, 0.9930555555555555802, 0.9944444444444444642, 0.9958333333333333481, 0.9972222222222222321, 0.9986111111111111160, 1.000000000000000000 ),
 .UNSPECIFIED. ) 
 GEOMETRIC_REPRESENTATION_ITEM ( )  RATIONAL_B_SPLINE_SURFACE ( (
 ( 1.000000000000000000, 0.8660254037844387076, 1.000000000000000000, 0.8660254037844387076, 1.000000000000000000, 0.8660254037844387076, 1.000000000000000000, 0.8660254037844387076, 1.000000000000000000, 0.8660254037844387076, 1.000000000000000000, 0.8660254037844387076, 1.000000000000000000, 0.8660254037844387076, 1.000000000000000000, 0.8660254037844387076, 1.000000000000000000, 0.8660254037844387076, 1.000000000000000000, 0.8660254037844387076, 1.000000000000000000, 0.8660254037844387076, 1.000000000000000000, 0.8660254037844387076, 1.000000000000000000, 0.8660254037844387076, 1.000000000000000000, 0.8660254037844387076, 1.000000000000000000, 0.8660254037844387076, 1.000000000000000000, 0.8660254037844387076, 1.000000000000000000, 0.8660254037844387076, 1.000000000000000000, 0.8660254037844387076, 1.000000000000000000, 0.8660254037844387076, 1.000000000000000000, 0.8660254037844387076, 1.000000000000000000, 0.8660254037844387076, 1.000000000000000000, 0.8660254037844387076, 1.000000000000000000, 0.8660254037844387076, 1.000000000000000000, 0.8660254037844387076, 1.000000000000000000, 0.8660254037844387076, 1.000000000000000000, 0.8660254037844387076, 1.000000000000000000, 0.8660254037844387076, 1.000000000000000000, 0.8660254037844387076, 1.000000000000000000, 0.8660254037844387076, 1.000000000000000000, 0.8660254037844387076, 1.000000000000000000, 0.8660254037844387076, 1.000000000000000000, 0.8660254037844387076, 1.000000000000000000, 0.8660254037844387076, 1.000000000000000000, 0.8660254037844387076, 1.000000000000000000, 0.8660254037844387076, 1.000000000000000000, 0.8660254037844387076, 1.000000000000000000, 0.8660254037844387076, 1.000000000000000000, 0.8660254037844387076, 1.000000000000000000, 0.8660254037844387076, 1.000000000000000000, 0.8660254037844387076, 1.000000000000000000, 0.8660254037844387076, 1.000000000000000000, 0.8660254037844387076, 1.000000000000000000, 0.8660254037844387076, 1.000000000000000000, 0.8660254037844387076, 1.000000000000000000, 0.8660254037844387076, 1.000000000000000000, 0.8660254037844387076, 1.000000000000000000, 0.8660254037844387076, 1.000000000000000000, 0.8660254037844387076, 1.000000000000000000, 0.8660254037844387076, 1.000000000000000000, 0.8660254037844387076, 1.000000000000000000, 0.8660254037844387076, 1.000000000000000000, 0.8660254037844387076, 1.000000000000000000, 0.8660254037844387076, 1.000000000000000000, 0.8660254037844387076, 1.000000000000000000, 0.8660254037844387076, 1.000000000000000000, 0.8660254037844387076, 1.000000000000000000, 0.8660254037844387076, 1.000000000000000000, 0.8660254037844387076, 1.000000000000000000, 0.8660254037844387076, 1.000000000000000000, 0.8660254037844387076, 1.000000000000000000, 0.8660254037844387076, 1.000000000000000000, 0.8660254037844387076, 1.000000000000000000, 0.8660254037844387076, 1.000000000000000000, 0.8660254037844387076, 1.000000000000000000, 0.8660254037844387076, 1.000000000000000000, 0.8660254037844387076, 1.000000000000000000, 0.8660254037844387076, 1.000000000000000000, 0.8660254037844387076, 1.000000000000000000, 0.8660254037844387076, 1.000000000000000000, 0.8660254037844387076, 1.000000000000000000, 0.8660254037844387076, 1.000000000000000000, 0.8660254037844387076, 1.000000000000000000, 0.8660254037844387076, 1.000000000000000000, 0.8660254037844387076, 1.000000000000000000, 0.8660254037844387076, 1.000000000000000000, 0.8660254037844387076, 1.000000000000000000, 0.8660254037844387076, 1.000000000000000000, 0.8660254037844387076, 1.000000000000000000, 0.8660254037844387076, 1.000000000000000000, 0.8660254037844387076, 1.000000000000000000, 0.8660254037844387076, 1.000000000000000000, 0.8660254037844387076, 1.000000000000000000, 0.8660254037844387076, 1.000000000000000000, 0.8660254037844387076, 1.000000000000000000, 0.8660254037844387076, 1.000000000000000000, 0.8660254037844387076, 1.000000000000000000, 0.8660254037844387076, 1.000000000000000000, 0.8660254037844387076, 1.000000000000000000, 0.8660254037844387076, 1.000000000000000000, 0.8660254037844387076, 1.000000000000000000, 0.8660254037844387076, 1.000000000000000000, 0.8660254037844387076, 1.000000000000000000, 0.8660254037844387076, 1.000000000000000000, 0.8660254037844387076, 1.000000000000000000, 0.8660254037844387076, 1.000000000000000000, 0.8660254037844387076, 1.000000000000000000, 0.8660254037844387076, 1.000000000000000000, 0.8660254037844387076, 1.000000000000000000, 0.8660254037844387076, 1.000000000000000000, 0.8660254037844387076, 1.000000000000000000, 0.8660254037844387076, 1.000000000000000000, 0.8660254037844387076, 1.000000000000000000, 0.8660254037844387076, 1.000000000000000000, 0.8660254037844387076, 1.000000000000000000, 0.8660254037844387076, 1.000000000000000000, 0.8660254037844387076, 1.000000000000000000, 0.8660254037844387076, 1.000000000000000000, 0.8660254037844387076, 1.000000000000000000, 0.8660254037844387076, 1.000000000000000000, 0.8660254037844387076, 1.000000000000000000, 0.8660254037844387076, 1.000000000000000000, 0.8660254037844387076, 1.000000000000000000, 0.8660254037844387076, 1.000000000000000000, 0.8660254037844387076, 1.000000000000000000, 0.8660254037844387076, 1.000000000000000000, 0.8660254037844387076, 1.000000000000000000, 0.8660254037844387076, 1.000000000000000000, 0.8660254037844387076, 1.000000000000000000, 0.8660254037844387076, 1.000000000000000000, 0.8660254037844387076, 1.000000000000000000, 0.8660254037844387076, 1.000000000000000000, 0.8660254037844387076, 1.000000000000000000, 0.8660254037844387076, 1.000000000000000000, 0.8660254037844387076, 1.000000000000000000, 0.8660254037844387076, 1.000000000000000000, 0.8660254037844387076, 1.000000000000000000, 0.8660254037844387076, 1.000000000000000000, 0.8660254037844387076, 1.000000000000000000, 0.8660254037844387076, 1.000000000000000000, 0.8660254037844387076, 1.000000000000000000, 0.8660254037844387076, 1.000000000000000000, 0.8660254037844387076, 1.000000000000000000, 0.8660254037844387076, 1.000000000000000000, 0.8660254037844387076, 1.000000000000000000, 0.8660254037844387076, 1.000000000000000000, 0.8660254037844387076, 1.000000000000000000, 0.8660254037844387076, 1.000000000000000000, 0.8660254037844387076, 1.000000000000000000, 0.8660254037844387076, 1.000000000000000000, 0.8660254037844387076, 1.000000000000000000, 0.8660254037844387076, 1.000000000000000000, 0.8660254037844387076, 1.000000000000000000, 0.8660254037844387076, 1.000000000000000000, 0.8660254037844387076, 1.000000000000000000, 0.8660254037844387076, 1.000000000000000000, 0.8660254037844387076, 1.000000000000000000, 0.8660254037844387076, 1.000000000000000000, 0.8660254037844387076, 1.000000000000000000, 0.8660254037844387076, 1.000000000000000000, 0.8660254037844387076, 1.000000000000000000, 0.8660254037844387076, 1.000000000000000000, 0.8660254037844387076, 1.000000000000000000, 0.8660254037844387076, 1.000000000000000000, 0.8660254037844387076, 1.000000000000000000, 0.8660254037844387076, 1.000000000000000000, 0.8660254037844387076, 1.000000000000000000, 0.8660254037844387076, 1.000000000000000000, 0.8660254037844387076, 1.000000000000000000, 0.8660254037844387076, 1.000000000000000000, 0.8660254037844387076, 1.000000000000000000, 0.8660254037844387076, 1.000000000000000000, 0.8660254037844387076, 1.000000000000000000, 0.8660254037844387076, 1.000000000000000000, 0.8660254037844387076, 1.000000000000000000, 0.8660254037844387076, 1.000000000000000000, 0.8660254037844387076, 1.000000000000000000, 0.8660254037844387076, 1.000000000000000000, 0.8660254037844387076, 1.000000000000000000, 0.8660254037844387076, 1.000000000000000000, 0.8660254037844387076, 1.000000000000000000, 0.8660254037844387076, 1.000000000000000000, 0.8660254037844387076, 1.000000000000000000, 0.8660254037844387076, 1.000000000000000000, 0.8660254037844387076, 1.000000000000000000, 0.8660254037844387076, 1.000000000000000000, 0.8660254037844387076, 1.000000000000000000, 0.8660254037844387076, 1.000000000000000000, 0.8660254037844387076, 1.000000000000000000, 0.8660254037844387076, 1.000000000000000000, 0.8660254037844387076, 1.000000000000000000, 0.8660254037844387076, 1.000000000000000000, 0.8660254037844387076, 1.000000000000000000, 0.8660254037844387076, 1.000000000000000000, 0.8660254037844387076, 1.000000000000000000, 0.8660254037844387076, 1.000000000000000000, 0.8660254037844387076, 1.000000000000000000, 0.8660254037844387076, 1.000000000000000000, 0.8660254037844387076, 1.000000000000000000, 0.8660254037844387076, 1.000000000000000000, 0.8660254037844387076, 1.000000000000000000, 0.8660254037844387076, 1.000000000000000000, 0.8660254037844387076, 1.000000000000000000, 0.8660254037844387076, 1.000000000000000000, 0.8660254037844387076, 1.000000000000000000, 0.8660254037844387076, 1.000000000000000000, 0.8660254037844387076, 1.000000000000000000, 0.8660254037844387076, 1.000000000000000000, 0.8660254037844387076, 1.000000000000000000, 0.8660254037844387076, 1.000000000000000000, 0.8660254037844387076, 1.000000000000000000, 0.8660254037844387076, 1.000000000000000000, 0.8660254037844387076, 1.000000000000000000, 0.8660254037844387076, 1.000000000000000000, 0.8660254037844387076, 1.000000000000000000, 0.8660254037844387076, 1.000000000000000000, 0.8660254037844387076, 1.000000000000000000, 0.8660254037844387076, 1.000000000000000000, 0.8660254037844387076, 1.000000000000000000, 0.8660254037844387076, 1.000000000000000000, 0.8660254037844387076, 1.000000000000000000, 0.8660254037844387076, 1.000000000000000000, 0.8660254037844387076, 1.000000000000000000, 0.8660254037844387076, 1.000000000000000000, 0.8660254037844387076, 1.000000000000000000, 0.8660254037844387076, 1.000000000000000000, 0.8660254037844387076, 1.000000000000000000, 0.8660254037844387076, 1.000000000000000000, 0.8660254037844387076, 1.000000000000000000, 0.8660254037844387076, 1.000000000000000000, 0.8660254037844387076, 1.000000000000000000, 0.8660254037844387076, 1.000000000000000000, 0.8660254037844387076, 1.000000000000000000, 0.8660254037844387076, 1.000000000000000000, 0.8660254037844387076, 1.000000000000000000, 0.8660254037844387076, 1.000000000000000000, 0.8660254037844387076, 1.000000000000000000, 0.8660254037844387076, 1.000000000000000000, 0.8660254037844387076, 1.000000000000000000, 0.8660254037844387076, 1.000000000000000000, 0.8660254037844387076, 1.000000000000000000, 0.8660254037844387076, 1.000000000000000000, 0.8660254037844387076, 1.000000000000000000, 0.8660254037844387076, 1.000000000000000000, 0.8660254037844387076, 1.000000000000000000, 0.8660254037844387076, 1.000000000000000000, 0.8660254037844387076, 1.000000000000000000, 0.8660254037844387076, 1.000000000000000000, 0.8660254037844387076, 1.000000000000000000, 0.8660254037844387076, 1.000000000000000000, 0.8660254037844387076, 1.000000000000000000, 0.8660254037844387076, 1.000000000000000000, 0.8660254037844387076, 1.000000000000000000, 0.8660254037844387076, 1.000000000000000000, 0.8660254037844387076, 1.000000000000000000, 0.8660254037844387076, 1.000000000000000000, 0.8660254037844387076, 1.000000000000000000, 0.8660254037844387076, 1.000000000000000000, 0.8660254037844387076, 1.000000000000000000, 0.8660254037844387076, 1.000000000000000000, 0.8660254037844387076, 1.000000000000000000, 0.8660254037844387076, 1.000000000000000000, 0.8660254037844387076, 1.000000000000000000, 0.8660254037844387076, 1.000000000000000000, 0.8660254037844387076, 1.000000000000000000, 0.8660254037844387076, 1.000000000000000000, 0.8660254037844387076, 1.000000000000000000, 0.8660254037844387076, 1.000000000000000000, 0.8660254037844387076, 1.000000000000000000, 0.8660254037844387076, 1.000000000000000000, 0.8660254037844387076, 1.000000000000000000, 0.8660254037844387076, 1.000000000000000000, 0.8660254037844387076, 1.000000000000000000, 0.8660254037844387076, 1.000000000000000000, 0.8660254037844387076, 1.000000000000000000, 0.8660254037844387076, 1.000000000000000000, 0.8660254037844387076, 1.000000000000000000, 0.8660254037844387076, 1.000000000000000000, 0.8660254037844387076, 1.000000000000000000, 0.8660254037844387076, 1.000000000000000000, 0.8660254037844387076, 1.000000000000000000, 0.8660254037844387076, 1.000000000000000000, 0.8660254037844387076, 1.000000000000000000, 0.8660254037844387076, 1.000000000000000000, 0.8660254037844387076, 1.000000000000000000, 0.8660254037844387076, 1.000000000000000000, 0.8660254037844387076, 1.000000000000000000, 0.8660254037844387076, 1.000000000000000000, 0.8660254037844387076, 1.000000000000000000, 0.8660254037844387076, 1.000000000000000000, 0.8660254037844387076, 1.000000000000000000, 0.8660254037844387076, 1.000000000000000000, 0.8660254037844387076, 1.000000000000000000, 0.8660254037844387076, 1.000000000000000000, 0.8660254037844387076, 1.000000000000000000, 0.8660254037844387076, 1.000000000000000000, 0.8660254037844387076, 1.000000000000000000, 0.8660254037844387076, 1.000000000000000000, 0.8660254037844387076, 1.000000000000000000, 0.8660254037844387076, 1.000000000000000000, 0.8660254037844387076, 1.000000000000000000, 0.8660254037844387076, 1.000000000000000000, 0.8660254037844387076, 1.000000000000000000, 0.8660254037844387076, 1.000000000000000000, 0.8660254037844387076, 1.000000000000000000, 0.8660254037844387076, 1.000000000000000000, 0.8660254037844387076, 1.000000000000000000, 0.8660254037844387076, 1.000000000000000000, 0.8660254037844387076, 1.000000000000000000, 0.8660254037844387076, 1.000000000000000000, 0.8660254037844387076, 1.000000000000000000, 0.8660254037844387076, 1.000000000000000000, 0.8660254037844387076, 1.000000000000000000, 0.8660254037844387076, 1.000000000000000000, 0.8660254037844387076, 1.000000000000000000, 0.8660254037844387076, 1.000000000000000000, 0.8660254037844387076, 1.000000000000000000, 0.8660254037844387076, 1.000000000000000000, 0.8660254037844387076, 1.000000000000000000, 0.8660254037844387076, 1.000000000000000000, 0.8660254037844387076, 1.000000000000000000, 0.8660254037844387076, 1.000000000000000000, 0.8660254037844387076, 1.000000000000000000, 0.8660254037844387076, 1.000000000000000000, 0.8660254037844387076, 1.000000000000000000, 0.8660254037844387076, 1.000000000000000000, 0.8660254037844387076, 1.000000000000000000, 0.8660254037844387076, 1.000000000000000000, 0.8660254037844387076, 1.000000000000000000, 0.8660254037844387076, 1.000000000000000000, 0.8660254037844387076, 1.000000000000000000, 0.8660254037844387076, 1.000000000000000000, 0.8660254037844387076, 1.000000000000000000, 0.8660254037844387076, 1.000000000000000000, 0.8660254037844387076, 1.000000000000000000, 0.8660254037844387076, 1.000000000000000000, 0.8660254037844387076, 1.000000000000000000, 0.8660254037844387076, 1.000000000000000000, 0.8660254037844387076, 1.000000000000000000, 0.8660254037844387076, 1.000000000000000000, 0.8660254037844387076, 1.000000000000000000, 0.8660254037844387076, 1.000000000000000000, 0.8660254037844387076, 1.000000000000000000, 0.8660254037844387076, 1.000000000000000000, 0.8660254037844387076, 1.000000000000000000, 0.8660254037844387076, 1.000000000000000000, 0.8660254037844387076, 1.000000000000000000, 0.8660254037844387076, 1.000000000000000000, 0.8660254037844387076, 1.000000000000000000, 0.8660254037844387076, 1.000000000000000000, 0.8660254037844387076, 1.000000000000000000, 0.8660254037844387076, 1.000000000000000000, 0.8660254037844387076, 1.000000000000000000, 0.8660254037844387076, 1.000000000000000000, 0.8660254037844387076, 1.000000000000000000, 0.8660254037844387076, 1.000000000000000000, 0.8660254037844387076, 1.000000000000000000, 0.8660254037844387076, 1.000000000000000000, 0.8660254037844387076, 1.000000000000000000, 0.8660254037844387076, 1.000000000000000000, 0.8660254037844387076, 1.000000000000000000, 0.8660254037844387076, 1.000000000000000000, 0.8660254037844387076, 1.000000000000000000, 0.8660254037844387076, 1.000000000000000000, 0.8660254037844387076, 1.000000000000000000, 0.8660254037844387076, 1.000000000000000000, 0.8660254037844387076, 1.000000000000000000, 0.8660254037844387076, 1.000000000000000000, 0.8660254037844387076, 1.000000000000000000, 0.8660254037844387076, 1.000000000000000000, 0.8660254037844387076, 1.000000000000000000, 0.8660254037844387076, 1.000000000000000000, 0.8660254037844387076, 1.000000000000000000, 0.8660254037844387076, 1.000000000000000000, 0.8660254037844387076, 1.000000000000000000, 0.8660254037844387076, 1.000000000000000000, 0.8660254037844387076, 1.000000000000000000, 0.8660254037844387076, 1.000000000000000000, 0.8660254037844387076, 1.000000000000000000, 0.8660254037844387076, 1.000000000000000000, 0.8660254037844387076, 1.000000000000000000, 0.8660254037844387076, 1.000000000000000000, 0.8660254037844387076, 1.000000000000000000, 0.8660254037844387076, 1.000000000000000000, 0.8660254037844387076, 1.000000000000000000, 0.8660254037844387076, 1.000000000000000000, 0.8660254037844387076, 1.000000000000000000, 0.8660254037844387076, 1.000000000000000000, 0.8660254037844387076, 1.000000000000000000, 0.8660254037844387076, 1.000000000000000000, 0.8660254037844387076, 1.000000000000000000, 0.8660254037844387076, 1.000000000000000000, 0.8660254037844387076, 1.000000000000000000, 0.8660254037844387076, 1.000000000000000000, 0.8660254037844387076, 1.000000000000000000, 0.8660254037844387076, 1.000000000000000000, 0.8660254037844387076, 1.000000000000000000, 0.8660254037844387076, 1.000000000000000000, 0.8660254037844387076, 1.000000000000000000, 0.8660254037844387076, 1.000000000000000000, 0.8660254037844387076, 1.000000000000000000, 0.8660254037844387076, 1.000000000000000000, 0.8660254037844387076, 1.000000000000000000, 0.8660254037844387076, 1.000000000000000000, 0.8660254037844387076, 1.000000000000000000, 0.8660254037844387076, 1.000000000000000000, 0.8660254037844387076, 1.000000000000000000, 0.8660254037844387076, 1.000000000000000000, 0.8660254037844387076, 1.000000000000000000, 0.8660254037844387076, 1.000000000000000000, 0.8660254037844387076, 1.000000000000000000, 0.8660254037844387076, 1.000000000000000000, 0.8660254037844387076, 1.000000000000000000, 0.8660254037844387076, 1.000000000000000000, 0.8660254037844387076, 1.000000000000000000, 0.8660254037844387076, 1.000000000000000000, 0.8660254037844387076, 1.000000000000000000, 0.8660254037844387076, 1.000000000000000000, 0.8660254037844387076, 1.000000000000000000, 0.8660254037844387076, 1.000000000000000000, 0.8660254037844387076, 1.000000000000000000, 0.8660254037844387076, 1.000000000000000000, 0.8660254037844387076, 1.000000000000000000, 0.8660254037844387076, 1.000000000000000000, 0.8660254037844387076, 1.000000000000000000, 0.8660254037844387076, 1.000000000000000000, 0.8660254037844387076, 1.000000000000000000, 0.8660254037844387076, 1.000000000000000000, 0.8660254037844387076, 1.000000000000000000, 0.8660254037844387076, 1.000000000000000000, 0.8660254037844387076, 1.000000000000000000, 0.8660254037844387076, 1.000000000000000000, 0.8660254037844387076, 1.000000000000000000, 0.8660254037844387076, 1.000000000000000000, 0.8660254037844387076, 1.000000000000000000, 0.8660254037844387076, 1.000000000000000000, 0.8660254037844387076, 1.000000000000000000, 0.8660254037844387076, 1.000000000000000000, 0.8660254037844387076, 1.000000000000000000, 0.8660254037844387076, 1.000000000000000000, 0.8660254037844387076, 1.000000000000000000, 0.8660254037844387076, 1.000000000000000000, 0.8660254037844387076, 1.000000000000000000, 0.8660254037844387076, 1.000000000000000000, 0.8660254037844387076, 1.000000000000000000, 0.8660254037844387076, 1.000000000000000000, 0.8660254037844387076, 1.000000000000000000, 0.8660254037844387076, 1.000000000000000000, 0.8660254037844387076, 1.000000000000000000, 0.8660254037844387076, 1.000000000000000000, 0.8660254037844387076, 1.000000000000000000, 0.8660254037844387076, 1.000000000000000000, 0.8660254037844387076, 1.000000000000000000, 0.8660254037844387076, 1.000000000000000000, 0.8660254037844387076, 1.000000000000000000, 0.8660254037844387076, 1.000000000000000000, 0.8660254037844387076, 1.000000000000000000, 0.8660254037844387076, 1.000000000000000000, 0.8660254037844387076, 1.000000000000000000, 0.8660254037844387076, 1.000000000000000000, 0.8660254037844387076, 1.000000000000000000, 0.8660254037844387076, 1.000000000000000000, 0.8660254037844387076, 1.000000000000000000, 0.8660254037844387076, 1.000000000000000000, 0.8660254037844387076, 1.000000000000000000, 0.8660254037844387076, 1.000000000000000000, 0.8660254037844387076, 1.000000000000000000, 0.8660254037844387076, 1.000000000000000000, 0.8660254037844387076, 1.000000000000000000, 0.8660254037844387076, 1.000000000000000000, 0.8660254037844387076, 1.000000000000000000, 0.8660254037844387076, 1.000000000000000000, 0.8660254037844387076, 1.000000000000000000, 0.8660254037844387076, 1.000000000000000000, 0.8660254037844387076, 1.000000000000000000, 0.8660254037844387076, 1.000000000000000000, 0.8660254037844387076, 1.000000000000000000, 0.8660254037844387076, 1.000000000000000000, 0.8660254037844387076, 1.000000000000000000, 0.8660254037844387076, 1.000000000000000000, 0.8660254037844387076, 1.000000000000000000, 0.8660254037844387076, 1.000000000000000000, 0.8660254037844387076, 1.000000000000000000, 0.8660254037844387076, 1.000000000000000000, 0.8660254037844387076, 1.000000000000000000, 0.8660254037844387076, 1.000000000000000000, 0.8660254037844387076, 1.000000000000000000, 0.8660254037844387076, 1.000000000000000000, 0.8660254037844387076, 1.000000000000000000, 0.8660254037844387076, 1.000000000000000000, 0.8660254037844387076, 1.000000000000000000, 0.8660254037844387076, 1.000000000000000000, 0.8660254037844387076, 1.000000000000000000, 0.8660254037844387076, 1.000000000000000000, 0.8660254037844387076, 1.000000000000000000, 0.8660254037844387076, 1.000000000000000000, 0.8660254037844387076, 1.000000000000000000, 0.8660254037844387076, 1.000000000000000000, 0.8660254037844387076, 1.000000000000000000, 0.8660254037844387076, 1.000000000000000000, 0.8660254037844387076, 1.000000000000000000, 0.8660254037844387076, 1.000000000000000000, 0.8660254037844387076, 1.000000000000000000, 0.8660254037844387076, 1.000000000000000000, 0.8660254037844387076, 1.000000000000000000, 0.8660254037844387076, 1.000000000000000000, 0.8660254037844387076, 1.000000000000000000, 0.8660254037844387076, 1.000000000000000000, 0.8660254037844387076, 1.000000000000000000, 0.8660254037844387076, 1.000000000000000000, 0.8660254037844387076, 1.000000000000000000, 0.8660254037844387076, 1.000000000000000000, 0.8660254037844387076, 1.000000000000000000, 0.8660254037844387076, 1.000000000000000000, 0.8660254037844387076, 1.000000000000000000, 0.8660254037844387076, 1.000000000000000000, 0.8660254037844387076, 1.000000000000000000, 0.8660254037844387076, 1.000000000000000000, 0.8660254037844387076, 1.000000000000000000, 0.8660254037844387076, 1.000000000000000000, 0.8660254037844387076, 1.000000000000000000, 0.8660254037844387076, 1.000000000000000000, 0.8660254037844387076, 1.000000000000000000, 0.8660254037844387076, 1.000000000000000000, 0.8660254037844387076, 1.000000000000000000, 0.8660254037844387076, 1.000000000000000000, 0.8660254037844387076, 1.000000000000000000, 0.8660254037844387076, 1.000000000000000000, 0.8660254037844387076, 1.000000000000000000, 0.8660254037844387076, 1.000000000000000000, 0.8660254037844387076, 1.000000000000000000, 0.8660254037844387076, 1.000000000000000000, 0.8660254037844387076, 1.000000000000000000, 0.8660254037844387076, 1.000000000000000000, 0.8660254037844387076, 1.000000000000000000, 0.8660254037844387076, 1.000000000000000000, 0.8660254037844387076, 1.000000000000000000, 0.8660254037844387076, 1.000000000000000000, 0.8660254037844387076, 1.000000000000000000, 0.8660254037844387076, 1.000000000000000000, 0.8660254037844387076, 1.000000000000000000, 0.8660254037844387076, 1.000000000000000000, 0.8660254037844387076, 1.000000000000000000, 0.8660254037844387076, 1.000000000000000000, 0.8660254037844387076, 1.000000000000000000, 0.8660254037844387076, 1.000000000000000000, 0.8660254037844387076, 1.000000000000000000, 0.8660254037844387076, 1.000000000000000000, 0.8660254037844387076, 1.000000000000000000, 0.8660254037844387076, 1.000000000000000000, 0.8660254037844387076, 1.000000000000000000, 0.8660254037844387076, 1.000000000000000000, 0.8660254037844387076, 1.000000000000000000, 0.8660254037844387076, 1.000000000000000000, 0.8660254037844387076, 1.000000000000000000, 0.8660254037844387076, 1.000000000000000000, 0.8660254037844387076, 1.000000000000000000, 0.8660254037844387076, 1.000000000000000000, 0.8660254037844387076, 1.000000000000000000, 0.8660254037844387076, 1.000000000000000000, 0.8660254037844387076, 1.000000000000000000, 0.8660254037844387076, 1.000000000000000000, 0.8660254037844387076, 1.000000000000000000, 0.8660254037844387076, 1.000000000000000000, 0.8660254037844387076, 1.000000000000000000, 0.8660254037844387076, 1.000000000000000000, 0.8660254037844387076, 1.000000000000000000, 0.8660254037844387076, 1.000000000000000000, 0.8660254037844387076, 1.000000000000000000, 0.8660254037844387076, 1.000000000000000000, 0.8660254037844387076, 1.000000000000000000, 0.8660254037844387076, 1.000000000000000000, 0.8660254037844387076, 1.000000000000000000, 0.8660254037844387076, 1.000000000000000000, 0.8660254037844387076, 1.000000000000000000, 0.8660254037844387076, 1.000000000000000000, 0.8660254037844387076, 1.000000000000000000, 0.8660254037844387076, 1.000000000000000000, 0.8660254037844387076, 1.000000000000000000, 0.8660254037844387076, 1.000000000000000000, 0.8660254037844387076, 1.000000000000000000, 0.8660254037844387076, 1.000000000000000000, 0.8660254037844387076, 1.000000000000000000, 0.8660254037844387076, 1.000000000000000000, 0.8660254037844387076, 1.000000000000000000, 0.8660254037844387076, 1.000000000000000000, 0.8660254037844387076, 1.000000000000000000, 0.8660254037844387076, 1.000000000000000000, 0.8660254037844387076, 1.000000000000000000, 0.8660254037844387076, 1.000000000000000000, 0.8660254037844387076, 1.000000000000000000, 0.8660254037844387076, 1.000000000000000000, 0.8660254037844387076, 1.000000000000000000, 0.8660254037844387076, 1.000000000000000000, 0.8660254037844387076, 1.000000000000000000, 0.8660254037844387076, 1.000000000000000000, 0.8660254037844387076, 1.000000000000000000, 0.8660254037844387076, 1.000000000000000000, 0.8660254037844387076, 1.000000000000000000, 0.8660254037844387076, 1.000000000000000000, 0.8660254037844387076, 1.000000000000000000, 0.8660254037844387076, 1.000000000000000000, 0.8660254037844387076, 1.000000000000000000, 0.8660254037844387076, 1.000000000000000000, 0.8660254037844387076, 1.000000000000000000, 0.8660254037844387076, 1.000000000000000000, 0.8660254037844387076, 1.000000000000000000, 0.8660254037844387076, 1.000000000000000000, 0.8660254037844387076, 1.000000000000000000, 0.8660254037844387076, 1.000000000000000000, 0.8660254037844387076, 1.000000000000000000, 0.8660254037844387076, 1.000000000000000000, 0.8660254037844387076, 1.000000000000000000, 0.8660254037844387076, 1.000000000000000000, 0.8660254037844387076, 1.000000000000000000, 0.8660254037844387076, 1.000000000000000000, 0.8660254037844387076, 1.000000000000000000, 0.8660254037844387076, 1.000000000000000000, 0.8660254037844387076, 1.000000000000000000, 0.8660254037844387076, 1.000000000000000000, 0.8660254037844387076, 1.000000000000000000, 0.8660254037844387076, 1.000000000000000000, 0.8660254037844387076, 1.000000000000000000, 0.8660254037844387076, 1.000000000000000000, 0.8660254037844387076, 1.000000000000000000, 0.8660254037844387076, 1.000000000000000000, 0.8660254037844387076, 1.000000000000000000, 0.8660254037844387076, 1.000000000000000000, 0.8660254037844387076, 1.000000000000000000, 0.8660254037844387076, 1.000000000000000000, 0.8660254037844387076, 1.000000000000000000, 0.8660254037844387076, 1.000000000000000000, 0.8660254037844387076, 1.000000000000000000, 0.8660254037844387076, 1.000000000000000000, 0.8660254037844387076, 1.000000000000000000, 0.8660254037844387076, 1.000000000000000000, 0.8660254037844387076, 1.000000000000000000, 0.8660254037844387076, 1.000000000000000000, 0.8660254037844387076, 1.000000000000000000, 0.8660254037844387076, 1.000000000000000000, 0.8660254037844387076, 1.000000000000000000, 0.8660254037844387076, 1.000000000000000000, 0.8660254037844387076, 1.000000000000000000, 0.8660254037844387076, 1.000000000000000000, 0.8660254037844387076, 1.000000000000000000, 0.8660254037844387076, 1.000000000000000000, 0.8660254037844387076, 1.000000000000000000, 0.8660254037844387076, 1.000000000000000000, 0.8660254037844387076, 1.000000000000000000, 0.8660254037844387076, 1.000000000000000000, 0.8660254037844387076, 1.000000000000000000, 0.8660254037844387076, 1.000000000000000000, 0.8660254037844387076, 1.000000000000000000, 0.8660254037844387076, 1.000000000000000000, 0.8660254037844387076, 1.000000000000000000, 0.8660254037844387076, 1.000000000000000000, 0.8660254037844387076, 1.000000000000000000, 0.8660254037844387076, 1.000000000000000000, 0.8660254037844387076, 1.000000000000000000, 0.8660254037844387076, 1.000000000000000000, 0.8660254037844387076, 1.000000000000000000, 0.8660254037844387076, 1.000000000000000000, 0.8660254037844387076, 1.000000000000000000, 0.8660254037844387076, 1.000000000000000000, 0.8660254037844387076, 1.000000000000000000, 0.8660254037844387076, 1.000000000000000000, 0.8660254037844387076, 1.000000000000000000, 0.8660254037844387076, 1.000000000000000000, 0.8660254037844387076, 1.000000000000000000, 0.8660254037844387076, 1.000000000000000000, 0.8660254037844387076, 1.000000000000000000, 0.8660254037844387076, 1.000000000000000000, 0.8660254037844387076, 1.000000000000000000, 0.8660254037844387076, 1.000000000000000000, 0.8660254037844387076, 1.000000000000000000, 0.8660254037844387076, 1.000000000000000000, 0.8660254037844387076, 1.000000000000000000, 0.8660254037844387076, 1.000000000000000000, 0.8660254037844387076, 1.000000000000000000, 0.8660254037844387076, 1.000000000000000000, 0.8660254037844387076, 1.000000000000000000, 0.8660254037844387076, 1.000000000000000000, 0.8660254037844387076, 1.000000000000000000, 0.8660254037844387076, 1.000000000000000000, 0.8660254037844387076, 1.000000000000000000, 0.8660254037844387076, 1.000000000000000000, 0.8660254037844387076, 1.000000000000000000, 0.8660254037844387076, 1.000000000000000000, 0.8660254037844387076, 1.000000000000000000, 0.8660254037844387076, 1.000000000000000000, 0.8660254037844387076, 1.000000000000000000, 0.8660254037844387076, 1.000000000000000000, 0.8660254037844387076, 1.000000000000000000, 0.8660254037844387076, 1.000000000000000000, 0.8660254037844387076, 1.000000000000000000, 0.8660254037844387076, 1.000000000000000000, 0.8660254037844387076, 1.000000000000000000, 0.8660254037844387076, 1.000000000000000000, 0.8660254037844387076, 1.000000000000000000, 0.8660254037844387076, 1.000000000000000000, 0.8660254037844387076, 1.000000000000000000, 0.8660254037844387076, 1.000000000000000000, 0.8660254037844387076, 1.000000000000000000, 0.8660254037844387076, 1.000000000000000000, 0.8660254037844387076, 1.000000000000000000, 0.8660254037844387076, 1.000000000000000000, 0.8660254037844387076, 1.000000000000000000, 0.8660254037844387076, 1.000000000000000000, 0.8660254037844387076, 1.000000000000000000, 0.8660254037844387076, 1.000000000000000000, 0.8660254037844387076, 1.000000000000000000, 0.8660254037844387076, 1.000000000000000000, 0.8660254037844387076, 1.000000000000000000, 0.8660254037844387076, 1.000000000000000000, 0.8660254037844387076, 1.000000000000000000, 0.8660254037844387076, 1.000000000000000000, 0.8660254037844387076, 1.000000000000000000, 0.8660254037844387076, 1.000000000000000000, 0.8660254037844387076, 1.000000000000000000, 0.8660254037844387076, 1.000000000000000000, 0.8660254037844387076, 1.000000000000000000, 0.8660254037844387076, 1.000000000000000000, 0.8660254037844387076, 1.000000000000000000, 0.8660254037844387076, 1.000000000000000000, 0.8660254037844387076, 1.000000000000000000, 0.8660254037844387076, 1.000000000000000000, 0.8660254037844387076, 1.000000000000000000, 0.8660254037844387076, 1.000000000000000000, 0.8660254037844387076, 1.000000000000000000, 0.8660254037844387076, 1.000000000000000000, 0.8660254037844387076, 1.000000000000000000),
 ( 1.000000000000000000, 0.8660254037844387076, 1.000000000000000000, 0.8660254037844387076, 1.000000000000000000, 0.8660254037844387076, 1.000000000000000000, 0.8660254037844387076, 1.000000000000000000, 0.8660254037844387076, 1.000000000000000000, 0.8660254037844387076, 1.000000000000000000, 0.8660254037844387076, 1.000000000000000000, 0.8660254037844387076, 1.000000000000000000, 0.8660254037844387076, 1.000000000000000000, 0.8660254037844387076, 1.000000000000000000, 0.8660254037844387076, 1.000000000000000000, 0.8660254037844387076, 1.000000000000000000, 0.8660254037844387076, 1.000000000000000000, 0.8660254037844387076, 1.000000000000000000, 0.8660254037844387076, 1.000000000000000000, 0.8660254037844387076, 1.000000000000000000, 0.8660254037844387076, 1.000000000000000000, 0.8660254037844387076, 1.000000000000000000, 0.8660254037844387076, 1.000000000000000000, 0.8660254037844387076, 1.000000000000000000, 0.8660254037844387076, 1.000000000000000000, 0.8660254037844387076, 1.000000000000000000, 0.8660254037844387076, 1.000000000000000000, 0.8660254037844387076, 1.000000000000000000, 0.8660254037844387076, 1.000000000000000000, 0.8660254037844387076, 1.000000000000000000, 0.8660254037844387076, 1.000000000000000000, 0.8660254037844387076, 1.000000000000000000, 0.8660254037844387076, 1.000000000000000000, 0.8660254037844387076, 1.000000000000000000, 0.8660254037844387076, 1.000000000000000000, 0.8660254037844387076, 1.000000000000000000, 0.8660254037844387076, 1.000000000000000000, 0.8660254037844387076, 1.000000000000000000, 0.8660254037844387076, 1.000000000000000000, 0.8660254037844387076, 1.000000000000000000, 0.8660254037844387076, 1.000000000000000000, 0.8660254037844387076, 1.000000000000000000, 0.8660254037844387076, 1.000000000000000000, 0.8660254037844387076, 1.000000000000000000, 0.8660254037844387076, 1.000000000000000000, 0.8660254037844387076, 1.000000000000000000, 0.8660254037844387076, 1.000000000000000000, 0.8660254037844387076, 1.000000000000000000, 0.8660254037844387076, 1.000000000000000000, 0.8660254037844387076, 1.000000000000000000, 0.8660254037844387076, 1.000000000000000000, 0.8660254037844387076, 1.000000000000000000, 0.8660254037844387076, 1.000000000000000000, 0.8660254037844387076, 1.000000000000000000, 0.8660254037844387076, 1.000000000000000000, 0.8660254037844387076, 1.000000000000000000, 0.8660254037844387076, 1.000000000000000000, 0.8660254037844387076, 1.000000000000000000, 0.8660254037844387076, 1.000000000000000000, 0.8660254037844387076, 1.000000000000000000, 0.8660254037844387076, 1.000000000000000000, 0.8660254037844387076, 1.000000000000000000, 0.8660254037844387076, 1.000000000000000000, 0.8660254037844387076, 1.000000000000000000, 0.8660254037844387076, 1.000000000000000000, 0.8660254037844387076, 1.000000000000000000, 0.8660254037844387076, 1.000000000000000000, 0.8660254037844387076, 1.000000000000000000, 0.8660254037844387076, 1.000000000000000000, 0.8660254037844387076, 1.000000000000000000, 0.8660254037844387076, 1.000000000000000000, 0.8660254037844387076, 1.000000000000000000, 0.8660254037844387076, 1.000000000000000000, 0.8660254037844387076, 1.000000000000000000, 0.8660254037844387076, 1.000000000000000000, 0.8660254037844387076, 1.000000000000000000, 0.8660254037844387076, 1.000000000000000000, 0.8660254037844387076, 1.000000000000000000, 0.8660254037844387076, 1.000000000000000000, 0.8660254037844387076, 1.000000000000000000, 0.8660254037844387076, 1.000000000000000000, 0.8660254037844387076, 1.000000000000000000, 0.8660254037844387076, 1.000000000000000000, 0.8660254037844387076, 1.000000000000000000, 0.8660254037844387076, 1.000000000000000000, 0.8660254037844387076, 1.000000000000000000, 0.8660254037844387076, 1.000000000000000000, 0.8660254037844387076, 1.000000000000000000, 0.8660254037844387076, 1.000000000000000000, 0.8660254037844387076, 1.000000000000000000, 0.8660254037844387076, 1.000000000000000000, 0.8660254037844387076, 1.000000000000000000, 0.8660254037844387076, 1.000000000000000000, 0.8660254037844387076, 1.000000000000000000, 0.8660254037844387076, 1.000000000000000000, 0.8660254037844387076, 1.000000000000000000, 0.8660254037844387076, 1.000000000000000000, 0.8660254037844387076, 1.000000000000000000, 0.8660254037844387076, 1.000000000000000000, 0.8660254037844387076, 1.000000000000000000, 0.8660254037844387076, 1.000000000000000000, 0.8660254037844387076, 1.000000000000000000, 0.8660254037844387076, 1.000000000000000000, 0.8660254037844387076, 1.000000000000000000, 0.8660254037844387076, 1.000000000000000000, 0.8660254037844387076, 1.000000000000000000, 0.8660254037844387076, 1.000000000000000000, 0.8660254037844387076, 1.000000000000000000, 0.8660254037844387076, 1.000000000000000000, 0.8660254037844387076, 1.000000000000000000, 0.8660254037844387076, 1.000000000000000000, 0.8660254037844387076, 1.000000000000000000, 0.8660254037844387076, 1.000000000000000000, 0.8660254037844387076, 1.000000000000000000, 0.8660254037844387076, 1.000000000000000000, 0.8660254037844387076, 1.000000000000000000, 0.8660254037844387076, 1.000000000000000000, 0.8660254037844387076, 1.000000000000000000, 0.8660254037844387076, 1.000000000000000000, 0.8660254037844387076, 1.000000000000000000, 0.8660254037844387076, 1.000000000000000000, 0.8660254037844387076, 1.000000000000000000, 0.8660254037844387076, 1.000000000000000000, 0.8660254037844387076, 1.000000000000000000, 0.8660254037844387076, 1.000000000000000000, 0.8660254037844387076, 1.000000000000000000, 0.8660254037844387076, 1.000000000000000000, 0.8660254037844387076, 1.000000000000000000, 0.8660254037844387076, 1.000000000000000000, 0.8660254037844387076, 1.000000000000000000, 0.8660254037844387076, 1.000000000000000000, 0.8660254037844387076, 1.000000000000000000, 0.8660254037844387076, 1.000000000000000000, 0.8660254037844387076, 1.000000000000000000, 0.8660254037844387076, 1.000000000000000000, 0.8660254037844387076, 1.000000000000000000, 0.8660254037844387076, 1.000000000000000000, 0.8660254037844387076, 1.000000000000000000, 0.8660254037844387076, 1.000000000000000000, 0.8660254037844387076, 1.000000000000000000, 0.8660254037844387076, 1.000000000000000000, 0.8660254037844387076, 1.000000000000000000, 0.8660254037844387076, 1.000000000000000000, 0.8660254037844387076, 1.000000000000000000, 0.8660254037844387076, 1.000000000000000000, 0.8660254037844387076, 1.000000000000000000, 0.8660254037844387076, 1.000000000000000000, 0.8660254037844387076, 1.000000000000000000, 0.8660254037844387076, 1.000000000000000000, 0.8660254037844387076, 1.000000000000000000, 0.8660254037844387076, 1.000000000000000000, 0.8660254037844387076, 1.000000000000000000, 0.8660254037844387076, 1.000000000000000000, 0.8660254037844387076, 1.000000000000000000, 0.8660254037844387076, 1.000000000000000000, 0.8660254037844387076, 1.000000000000000000, 0.8660254037844387076, 1.000000000000000000, 0.8660254037844387076, 1.000000000000000000, 0.8660254037844387076, 1.000000000000000000, 0.8660254037844387076, 1.000000000000000000, 0.8660254037844387076, 1.000000000000000000, 0.8660254037844387076, 1.000000000000000000, 0.8660254037844387076, 1.000000000000000000, 0.8660254037844387076, 1.000000000000000000, 0.8660254037844387076, 1.000000000000000000, 0.8660254037844387076, 1.000000000000000000, 0.8660254037844387076, 1.000000000000000000, 0.8660254037844387076, 1.000000000000000000, 0.8660254037844387076, 1.000000000000000000, 0.8660254037844387076, 1.000000000000000000, 0.8660254037844387076, 1.000000000000000000, 0.8660254037844387076, 1.000000000000000000, 0.8660254037844387076, 1.000000000000000000, 0.8660254037844387076, 1.000000000000000000, 0.8660254037844387076, 1.000000000000000000, 0.8660254037844387076, 1.000000000000000000, 0.8660254037844387076, 1.000000000000000000, 0.8660254037844387076, 1.000000000000000000, 0.8660254037844387076, 1.000000000000000000, 0.8660254037844387076, 1.000000000000000000, 0.8660254037844387076, 1.000000000000000000, 0.8660254037844387076, 1.000000000000000000, 0.8660254037844387076, 1.000000000000000000, 0.8660254037844387076, 1.000000000000000000, 0.8660254037844387076, 1.000000000000000000, 0.8660254037844387076, 1.000000000000000000, 0.8660254037844387076, 1.000000000000000000, 0.8660254037844387076, 1.000000000000000000, 0.8660254037844387076, 1.000000000000000000, 0.8660254037844387076, 1.000000000000000000, 0.8660254037844387076, 1.000000000000000000, 0.8660254037844387076, 1.000000000000000000, 0.8660254037844387076, 1.000000000000000000, 0.8660254037844387076, 1.000000000000000000, 0.8660254037844387076, 1.000000000000000000, 0.8660254037844387076, 1.000000000000000000, 0.8660254037844387076, 1.000000000000000000, 0.8660254037844387076, 1.000000000000000000, 0.8660254037844387076, 1.000000000000000000, 0.8660254037844387076, 1.000000000000000000, 0.8660254037844387076, 1.000000000000000000, 0.8660254037844387076, 1.000000000000000000, 0.8660254037844387076, 1.000000000000000000, 0.8660254037844387076, 1.000000000000000000, 0.8660254037844387076, 1.000000000000000000, 0.8660254037844387076, 1.000000000000000000, 0.8660254037844387076, 1.000000000000000000, 0.8660254037844387076, 1.000000000000000000, 0.8660254037844387076, 1.000000000000000000, 0.8660254037844387076, 1.000000000000000000, 0.8660254037844387076, 1.000000000000000000, 0.8660254037844387076, 1.000000000000000000, 0.8660254037844387076, 1.000000000000000000, 0.8660254037844387076, 1.000000000000000000, 0.8660254037844387076, 1.000000000000000000, 0.8660254037844387076, 1.000000000000000000, 0.8660254037844387076, 1.000000000000000000, 0.8660254037844387076, 1.000000000000000000, 0.8660254037844387076, 1.000000000000000000, 0.8660254037844387076, 1.000000000000000000, 0.8660254037844387076, 1.000000000000000000, 0.8660254037844387076, 1.000000000000000000, 0.8660254037844387076, 1.000000000000000000, 0.8660254037844387076, 1.000000000000000000, 0.8660254037844387076, 1.000000000000000000, 0.8660254037844387076, 1.000000000000000000, 0.8660254037844387076, 1.000000000000000000, 0.8660254037844387076, 1.000000000000000000, 0.8660254037844387076, 1.000000000000000000, 0.8660254037844387076, 1.000000000000000000, 0.8660254037844387076, 1.000000000000000000, 0.8660254037844387076, 1.000000000000000000, 0.8660254037844387076, 1.000000000000000000, 0.8660254037844387076, 1.000000000000000000, 0.8660254037844387076, 1.000000000000000000, 0.8660254037844387076, 1.000000000000000000, 0.8660254037844387076, 1.000000000000000000, 0.8660254037844387076, 1.000000000000000000, 0.8660254037844387076, 1.000000000000000000, 0.8660254037844387076, 1.000000000000000000, 0.8660254037844387076, 1.000000000000000000, 0.8660254037844387076, 1.000000000000000000, 0.8660254037844387076, 1.000000000000000000, 0.8660254037844387076, 1.000000000000000000, 0.8660254037844387076, 1.000000000000000000, 0.8660254037844387076, 1.000000000000000000, 0.8660254037844387076, 1.000000000000000000, 0.8660254037844387076, 1.000000000000000000, 0.8660254037844387076, 1.000000000000000000, 0.8660254037844387076, 1.000000000000000000, 0.8660254037844387076, 1.000000000000000000, 0.8660254037844387076, 1.000000000000000000, 0.8660254037844387076, 1.000000000000000000, 0.8660254037844387076, 1.000000000000000000, 0.8660254037844387076, 1.000000000000000000, 0.8660254037844387076, 1.000000000000000000, 0.8660254037844387076, 1.000000000000000000, 0.8660254037844387076, 1.000000000000000000, 0.8660254037844387076, 1.000000000000000000, 0.8660254037844387076, 1.000000000000000000, 0.8660254037844387076, 1.000000000000000000, 0.8660254037844387076, 1.000000000000000000, 0.8660254037844387076, 1.000000000000000000, 0.8660254037844387076, 1.000000000000000000, 0.8660254037844387076, 1.000000000000000000, 0.8660254037844387076, 1.000000000000000000, 0.8660254037844387076, 1.000000000000000000, 0.8660254037844387076, 1.000000000000000000, 0.8660254037844387076, 1.000000000000000000, 0.8660254037844387076, 1.000000000000000000, 0.8660254037844387076, 1.000000000000000000, 0.8660254037844387076, 1.000000000000000000, 0.8660254037844387076, 1.000000000000000000, 0.8660254037844387076, 1.000000000000000000, 0.8660254037844387076, 1.000000000000000000, 0.8660254037844387076, 1.000000000000000000, 0.8660254037844387076, 1.000000000000000000, 0.8660254037844387076, 1.000000000000000000, 0.8660254037844387076, 1.000000000000000000, 0.8660254037844387076, 1.000000000000000000, 0.8660254037844387076, 1.000000000000000000, 0.8660254037844387076, 1.000000000000000000, 0.8660254037844387076, 1.000000000000000000, 0.8660254037844387076, 1.000000000000000000, 0.8660254037844387076, 1.000000000000000000, 0.8660254037844387076, 1.000000000000000000, 0.8660254037844387076, 1.000000000000000000, 0.8660254037844387076, 1.000000000000000000, 0.8660254037844387076, 1.000000000000000000, 0.8660254037844387076, 1.000000000000000000, 0.8660254037844387076, 1.000000000000000000, 0.8660254037844387076, 1.000000000000000000, 0.8660254037844387076, 1.000000000000000000, 0.8660254037844387076, 1.000000000000000000, 0.8660254037844387076, 1.000000000000000000, 0.8660254037844387076, 1.000000000000000000, 0.8660254037844387076, 1.000000000000000000, 0.8660254037844387076, 1.000000000000000000, 0.8660254037844387076, 1.000000000000000000, 0.8660254037844387076, 1.000000000000000000, 0.8660254037844387076, 1.000000000000000000, 0.8660254037844387076, 1.000000000000000000, 0.8660254037844387076, 1.000000000000000000, 0.8660254037844387076, 1.000000000000000000, 0.8660254037844387076, 1.000000000000000000, 0.8660254037844387076, 1.000000000000000000, 0.8660254037844387076, 1.000000000000000000, 0.8660254037844387076, 1.000000000000000000, 0.8660254037844387076, 1.000000000000000000, 0.8660254037844387076, 1.000000000000000000, 0.8660254037844387076, 1.000000000000000000, 0.8660254037844387076, 1.000000000000000000, 0.8660254037844387076, 1.000000000000000000, 0.8660254037844387076, 1.000000000000000000, 0.8660254037844387076, 1.000000000000000000, 0.8660254037844387076, 1.000000000000000000, 0.8660254037844387076, 1.000000000000000000, 0.8660254037844387076, 1.000000000000000000, 0.8660254037844387076, 1.000000000000000000, 0.8660254037844387076, 1.000000000000000000, 0.8660254037844387076, 1.000000000000000000, 0.8660254037844387076, 1.000000000000000000, 0.8660254037844387076, 1.000000000000000000, 0.8660254037844387076, 1.000000000000000000, 0.8660254037844387076, 1.000000000000000000, 0.8660254037844387076, 1.000000000000000000, 0.8660254037844387076, 1.000000000000000000, 0.8660254037844387076, 1.000000000000000000, 0.8660254037844387076, 1.000000000000000000, 0.8660254037844387076, 1.000000000000000000, 0.8660254037844387076, 1.000000000000000000, 0.8660254037844387076, 1.000000000000000000, 0.8660254037844387076, 1.000000000000000000, 0.8660254037844387076, 1.000000000000000000, 0.8660254037844387076, 1.000000000000000000, 0.8660254037844387076, 1.000000000000000000, 0.8660254037844387076, 1.000000000000000000, 0.8660254037844387076, 1.000000000000000000, 0.8660254037844387076, 1.000000000000000000, 0.8660254037844387076, 1.000000000000000000, 0.8660254037844387076, 1.000000000000000000, 0.8660254037844387076, 1.000000000000000000, 0.8660254037844387076, 1.000000000000000000, 0.8660254037844387076, 1.000000000000000000, 0.8660254037844387076, 1.000000000000000000, 0.8660254037844387076, 1.000000000000000000, 0.8660254037844387076, 1.000000000000000000, 0.8660254037844387076, 1.000000000000000000, 0.8660254037844387076, 1.000000000000000000, 0.8660254037844387076, 1.000000000000000000, 0.8660254037844387076, 1.000000000000000000, 0.8660254037844387076, 1.000000000000000000, 0.8660254037844387076, 1.000000000000000000, 0.8660254037844387076, 1.000000000000000000, 0.8660254037844387076, 1.000000000000000000, 0.8660254037844387076, 1.000000000000000000, 0.8660254037844387076, 1.000000000000000000, 0.8660254037844387076, 1.000000000000000000, 0.8660254037844387076, 1.000000000000000000, 0.8660254037844387076, 1.000000000000000000, 0.8660254037844387076, 1.000000000000000000, 0.8660254037844387076, 1.000000000000000000, 0.8660254037844387076, 1.000000000000000000, 0.8660254037844387076, 1.000000000000000000, 0.8660254037844387076, 1.000000000000000000, 0.8660254037844387076, 1.000000000000000000, 0.8660254037844387076, 1.000000000000000000, 0.8660254037844387076, 1.000000000000000000, 0.8660254037844387076, 1.000000000000000000, 0.8660254037844387076, 1.000000000000000000, 0.8660254037844387076, 1.000000000000000000, 0.8660254037844387076, 1.000000000000000000, 0.8660254037844387076, 1.000000000000000000, 0.8660254037844387076, 1.000000000000000000, 0.8660254037844387076, 1.000000000000000000, 0.8660254037844387076, 1.000000000000000000, 0.8660254037844387076, 1.000000000000000000, 0.8660254037844387076, 1.000000000000000000, 0.8660254037844387076, 1.000000000000000000, 0.8660254037844387076, 1.000000000000000000, 0.8660254037844387076, 1.000000000000000000, 0.8660254037844387076, 1.000000000000000000, 0.8660254037844387076, 1.000000000000000000, 0.8660254037844387076, 1.000000000000000000, 0.8660254037844387076, 1.000000000000000000, 0.8660254037844387076, 1.000000000000000000, 0.8660254037844387076, 1.000000000000000000, 0.8660254037844387076, 1.000000000000000000, 0.8660254037844387076, 1.000000000000000000, 0.8660254037844387076, 1.000000000000000000, 0.8660254037844387076, 1.000000000000000000, 0.8660254037844387076, 1.000000000000000000, 0.8660254037844387076, 1.000000000000000000, 0.8660254037844387076, 1.000000000000000000, 0.8660254037844387076, 1.000000000000000000, 0.8660254037844387076, 1.000000000000000000, 0.8660254037844387076, 1.000000000000000000, 0.8660254037844387076, 1.000000000000000000, 0.8660254037844387076, 1.000000000000000000, 0.8660254037844387076, 1.000000000000000000, 0.8660254037844387076, 1.000000000000000000, 0.8660254037844387076, 1.000000000000000000, 0.8660254037844387076, 1.000000000000000000, 0.8660254037844387076, 1.000000000000000000, 0.8660254037844387076, 1.000000000000000000, 0.8660254037844387076, 1.000000000000000000, 0.8660254037844387076, 1.000000000000000000, 0.8660254037844387076, 1.000000000000000000, 0.8660254037844387076, 1.000000000000000000, 0.8660254037844387076, 1.000000000000000000, 0.8660254037844387076, 1.000000000000000000, 0.8660254037844387076, 1.000000000000000000, 0.8660254037844387076, 1.000000000000000000, 0.8660254037844387076, 1.000000000000000000, 0.8660254037844387076, 1.000000000000000000, 0.8660254037844387076, 1.000000000000000000, 0.8660254037844387076, 1.000000000000000000, 0.8660254037844387076, 1.000000000000000000, 0.8660254037844387076, 1.000000000000000000, 0.8660254037844387076, 1.000000000000000000, 0.8660254037844387076, 1.000000000000000000, 0.8660254037844387076, 1.000000000000000000, 0.8660254037844387076, 1.000000000000000000, 0.8660254037844387076, 1.000000000000000000, 0.8660254037844387076, 1.000000000000000000, 0.8660254037844387076, 1.000000000000000000, 0.8660254037844387076, 1.000000000000000000, 0.8660254037844387076, 1.000000000000000000, 0.8660254037844387076, 1.000000000000000000, 0.8660254037844387076, 1.000000000000000000, 0.8660254037844387076, 1.000000000000000000, 0.8660254037844387076, 1.000000000000000000, 0.8660254037844387076, 1.000000000000000000, 0.8660254037844387076, 1.000000000000000000, 0.8660254037844387076, 1.000000000000000000, 0.8660254037844387076, 1.000000000000000000, 0.8660254037844387076, 1.000000000000000000, 0.8660254037844387076, 1.000000000000000000, 0.8660254037844387076, 1.000000000000000000, 0.8660254037844387076, 1.000000000000000000, 0.8660254037844387076, 1.000000000000000000, 0.8660254037844387076, 1.000000000000000000, 0.8660254037844387076, 1.000000000000000000, 0.8660254037844387076, 1.000000000000000000, 0.8660254037844387076, 1.000000000000000000, 0.8660254037844387076, 1.000000000000000000, 0.8660254037844387076, 1.000000000000000000, 0.8660254037844387076, 1.000000000000000000, 0.8660254037844387076, 1.000000000000000000, 0.8660254037844387076, 1.000000000000000000, 0.8660254037844387076, 1.000000000000000000, 0.8660254037844387076, 1.000000000000000000, 0.8660254037844387076, 1.000000000000000000, 0.8660254037844387076, 1.000000000000000000, 0.8660254037844387076, 1.000000000000000000, 0.8660254037844387076, 1.000000000000000000, 0.8660254037844387076, 1.000000000000000000, 0.8660254037844387076, 1.000000000000000000, 0.8660254037844387076, 1.000000000000000000, 0.8660254037844387076, 1.000000000000000000, 0.8660254037844387076, 1.000000000000000000, 0.8660254037844387076, 1.000000000000000000, 0.8660254037844387076, 1.000000000000000000, 0.8660254037844387076, 1.000000000000000000, 0.8660254037844387076, 1.000000000000000000, 0.8660254037844387076, 1.000000000000000000, 0.8660254037844387076, 1.000000000000000000, 0.8660254037844387076, 1.000000000000000000, 0.8660254037844387076, 1.000000000000000000, 0.8660254037844387076, 1.000000000000000000, 0.8660254037844387076, 1.000000000000000000, 0.8660254037844387076, 1.000000000000000000, 0.8660254037844387076, 1.000000000000000000, 0.8660254037844387076, 1.000000000000000000, 0.8660254037844387076, 1.000000000000000000, 0.8660254037844387076, 1.000000000000000000, 0.8660254037844387076, 1.000000000000000000, 0.8660254037844387076, 1.000000000000000000, 0.8660254037844387076, 1.000000000000000000, 0.8660254037844387076, 1.000000000000000000, 0.8660254037844387076, 1.000000000000000000, 0.8660254037844387076, 1.000000000000000000, 0.8660254037844387076, 1.000000000000000000, 0.8660254037844387076, 1.000000000000000000, 0.8660254037844387076, 1.000000000000000000, 0.8660254037844387076, 1.000000000000000000, 0.8660254037844387076, 1.000000000000000000, 0.8660254037844387076, 1.000000000000000000, 0.8660254037844387076, 1.000000000000000000, 0.8660254037844387076, 1.000000000000000000, 0.8660254037844387076, 1.000000000000000000, 0.8660254037844387076, 1.000000000000000000, 0.8660254037844387076, 1.000000000000000000, 0.8660254037844387076, 1.000000000000000000, 0.8660254037844387076, 1.000000000000000000, 0.8660254037844387076, 1.000000000000000000, 0.8660254037844387076, 1.000000000000000000, 0.8660254037844387076, 1.000000000000000000, 0.8660254037844387076, 1.000000000000000000, 0.8660254037844387076, 1.000000000000000000, 0.8660254037844387076, 1.000000000000000000, 0.8660254037844387076, 1.000000000000000000, 0.8660254037844387076, 1.000000000000000000, 0.8660254037844387076, 1.000000000000000000, 0.8660254037844387076, 1.000000000000000000, 0.8660254037844387076, 1.000000000000000000, 0.8660254037844387076, 1.000000000000000000, 0.8660254037844387076, 1.000000000000000000, 0.8660254037844387076, 1.000000000000000000, 0.8660254037844387076, 1.000000000000000000, 0.8660254037844387076, 1.000000000000000000, 0.8660254037844387076, 1.000000000000000000, 0.8660254037844387076, 1.000000000000000000, 0.8660254037844387076, 1.000000000000000000, 0.8660254037844387076, 1.000000000000000000, 0.8660254037844387076, 1.000000000000000000, 0.8660254037844387076, 1.000000000000000000, 0.8660254037844387076, 1.000000000000000000, 0.8660254037844387076, 1.000000000000000000, 0.8660254037844387076, 1.000000000000000000, 0.8660254037844387076, 1.000000000000000000, 0.8660254037844387076, 1.000000000000000000, 0.8660254037844387076, 1.000000000000000000, 0.8660254037844387076, 1.000000000000000000, 0.8660254037844387076, 1.000000000000000000, 0.8660254037844387076, 1.000000000000000000, 0.8660254037844387076, 1.000000000000000000, 0.8660254037844387076, 1.000000000000000000, 0.8660254037844387076, 1.000000000000000000, 0.8660254037844387076, 1.000000000000000000, 0.8660254037844387076, 1.000000000000000000, 0.8660254037844387076, 1.000000000000000000, 0.8660254037844387076, 1.000000000000000000, 0.8660254037844387076, 1.000000000000000000, 0.8660254037844387076, 1.000000000000000000, 0.8660254037844387076, 1.000000000000000000, 0.8660254037844387076, 1.000000000000000000, 0.8660254037844387076, 1.000000000000000000, 0.8660254037844387076, 1.000000000000000000, 0.8660254037844387076, 1.000000000000000000, 0.8660254037844387076, 1.000000000000000000, 0.8660254037844387076, 1.000000000000000000, 0.8660254037844387076, 1.000000000000000000, 0.8660254037844387076, 1.000000000000000000, 0.8660254037844387076, 1.000000000000000000, 0.8660254037844387076, 1.000000000000000000, 0.8660254037844387076, 1.000000000000000000, 0.8660254037844387076, 1.000000000000000000, 0.8660254037844387076, 1.000000000000000000, 0.8660254037844387076, 1.000000000000000000, 0.8660254037844387076, 1.000000000000000000, 0.8660254037844387076, 1.000000000000000000, 0.8660254037844387076, 1.000000000000000000, 0.8660254037844387076, 1.000000000000000000, 0.8660254037844387076, 1.000000000000000000, 0.8660254037844387076, 1.000000000000000000, 0.8660254037844387076, 1.000000000000000000, 0.8660254037844387076, 1.000000000000000000, 0.8660254037844387076, 1.000000000000000000, 0.8660254037844387076, 1.000000000000000000, 0.8660254037844387076, 1.000000000000000000, 0.8660254037844387076, 1.000000000000000000, 0.8660254037844387076, 1.000000000000000000, 0.8660254037844387076, 1.000000000000000000, 0.8660254037844387076, 1.000000000000000000, 0.8660254037844387076, 1.000000000000000000, 0.8660254037844387076, 1.000000000000000000, 0.8660254037844387076, 1.000000000000000000, 0.8660254037844387076, 1.000000000000000000, 0.8660254037844387076, 1.000000000000000000, 0.8660254037844387076, 1.000000000000000000, 0.8660254037844387076, 1.000000000000000000, 0.8660254037844387076, 1.000000000000000000, 0.8660254037844387076, 1.000000000000000000, 0.8660254037844387076, 1.000000000000000000, 0.8660254037844387076, 1.000000000000000000, 0.8660254037844387076, 1.000000000000000000, 0.8660254037844387076, 1.000000000000000000, 0.8660254037844387076, 1.000000000000000000, 0.8660254037844387076, 1.000000000000000000, 0.8660254037844387076, 1.000000000000000000, 0.8660254037844387076, 1.000000000000000000, 0.8660254037844387076, 1.000000000000000000, 0.8660254037844387076, 1.000000000000000000, 0.8660254037844387076, 1.000000000000000000, 0.8660254037844387076, 1.000000000000000000, 0.8660254037844387076, 1.000000000000000000, 0.8660254037844387076, 1.000000000000000000, 0.8660254037844387076, 1.000000000000000000, 0.8660254037844387076, 1.000000000000000000, 0.8660254037844387076, 1.000000000000000000, 0.8660254037844387076, 1.000000000000000000, 0.8660254037844387076, 1.000000000000000000, 0.8660254037844387076, 1.000000000000000000, 0.8660254037844387076, 1.000000000000000000, 0.8660254037844387076, 1.000000000000000000, 0.8660254037844387076, 1.000000000000000000, 0.8660254037844387076, 1.000000000000000000, 0.8660254037844387076, 1.000000000000000000, 0.8660254037844387076, 1.000000000000000000, 0.8660254037844387076, 1.000000000000000000, 0.8660254037844387076, 1.000000000000000000, 0.8660254037844387076, 1.000000000000000000, 0.8660254037844387076, 1.000000000000000000, 0.8660254037844387076, 1.000000000000000000, 0.8660254037844387076, 1.000000000000000000, 0.8660254037844387076, 1.000000000000000000, 0.8660254037844387076, 1.000000000000000000, 0.8660254037844387076, 1.000000000000000000, 0.8660254037844387076, 1.000000000000000000, 0.8660254037844387076, 1.000000000000000000, 0.8660254037844387076, 1.000000000000000000, 0.8660254037844387076, 1.000000000000000000, 0.8660254037844387076, 1.000000000000000000, 0.8660254037844387076, 1.000000000000000000, 0.8660254037844387076, 1.000000000000000000, 0.8660254037844387076, 1.000000000000000000, 0.8660254037844387076, 1.000000000000000000, 0.8660254037844387076, 1.000000000000000000, 0.8660254037844387076, 1.000000000000000000, 0.8660254037844387076, 1.000000000000000000, 0.8660254037844387076, 1.000000000000000000, 0.8660254037844387076, 1.000000000000000000, 0.8660254037844387076, 1.000000000000000000, 0.8660254037844387076, 1.000000000000000000, 0.8660254037844387076, 1.000000000000000000, 0.8660254037844387076, 1.000000000000000000, 0.8660254037844387076, 1.000000000000000000, 0.8660254037844387076, 1.000000000000000000, 0.8660254037844387076, 1.000000000000000000, 0.8660254037844387076, 1.000000000000000000, 0.8660254037844387076, 1.000000000000000000, 0.8660254037844387076, 1.000000000000000000, 0.8660254037844387076, 1.000000000000000000, 0.8660254037844387076, 1.000000000000000000, 0.8660254037844387076, 1.000000000000000000, 0.8660254037844387076, 1.000000000000000000, 0.8660254037844387076, 1.000000000000000000, 0.8660254037844387076, 1.000000000000000000, 0.8660254037844387076, 1.000000000000000000, 0.8660254037844387076, 1.000000000000000000, 0.8660254037844387076, 1.000000000000000000, 0.8660254037844387076, 1.000000000000000000, 0.8660254037844387076, 1.000000000000000000, 0.8660254037844387076, 1.000000000000000000, 0.8660254037844387076, 1.000000000000000000, 0.8660254037844387076, 1.000000000000000000, 0.8660254037844387076, 1.000000000000000000, 0.8660254037844387076, 1.000000000000000000, 0.8660254037844387076, 1.000000000000000000, 0.8660254037844387076, 1.000000000000000000, 0.8660254037844387076, 1.000000000000000000, 0.8660254037844387076, 1.000000000000000000, 0.8660254037844387076, 1.000000000000000000, 0.8660254037844387076, 1.000000000000000000, 0.8660254037844387076, 1.000000000000000000, 0.8660254037844387076, 1.000000000000000000, 0.8660254037844387076, 1.000000000000000000, 0.8660254037844387076, 1.000000000000000000, 0.8660254037844387076, 1.000000000000000000, 0.8660254037844387076, 1.000000000000000000, 0.8660254037844387076, 1.000000000000000000, 0.8660254037844387076, 1.000000000000000000, 0.8660254037844387076, 1.000000000000000000, 0.8660254037844387076, 1.000000000000000000, 0.8660254037844387076, 1.000000000000000000, 0.8660254037844387076, 1.000000000000000000, 0.8660254037844387076, 1.000000000000000000, 0.8660254037844387076, 1.000000000000000000, 0.8660254037844387076, 1.000000000000000000, 0.8660254037844387076, 1.000000000000000000, 0.8660254037844387076, 1.000000000000000000, 0.8660254037844387076, 1.000000000000000000, 0.8660254037844387076, 1.000000000000000000, 0.8660254037844387076, 1.000000000000000000, 0.8660254037844387076, 1.000000000000000000, 0.8660254037844387076, 1.000000000000000000, 0.8660254037844387076, 1.000000000000000000, 0.8660254037844387076, 1.000000000000000000, 0.8660254037844387076, 1.000000000000000000, 0.8660254037844387076, 1.000000000000000000, 0.8660254037844387076, 1.000000000000000000, 0.8660254037844387076, 1.000000000000000000, 0.8660254037844387076, 1.000000000000000000, 0.8660254037844387076, 1.000000000000000000, 0.8660254037844387076, 1.000000000000000000, 0.8660254037844387076, 1.000000000000000000, 0.8660254037844387076, 1.000000000000000000, 0.8660254037844387076, 1.000000000000000000, 0.8660254037844387076, 1.000000000000000000, 0.8660254037844387076, 1.000000000000000000, 0.8660254037844387076, 1.000000000000000000, 0.8660254037844387076, 1.000000000000000000, 0.8660254037844387076, 1.000000000000000000, 0.8660254037844387076, 1.000000000000000000, 0.8660254037844387076, 1.000000000000000000, 0.8660254037844387076, 1.000000000000000000, 0.8660254037844387076, 1.000000000000000000, 0.8660254037844387076, 1.000000000000000000, 0.8660254037844387076, 1.000000000000000000, 0.8660254037844387076, 1.000000000000000000, 0.8660254037844387076, 1.000000000000000000, 0.8660254037844387076, 1.000000000000000000, 0.8660254037844387076, 1.000000000000000000, 0.8660254037844387076, 1.000000000000000000, 0.8660254037844387076, 1.000000000000000000, 0.8660254037844387076, 1.000000000000000000, 0.8660254037844387076, 1.000000000000000000, 0.8660254037844387076, 1.000000000000000000, 0.8660254037844387076, 1.000000000000000000, 0.8660254037844387076, 1.000000000000000000, 0.8660254037844387076, 1.000000000000000000, 0.8660254037844387076, 1.000000000000000000, 0.8660254037844387076, 1.000000000000000000, 0.8660254037844387076, 1.000000000000000000, 0.8660254037844387076, 1.000000000000000000, 0.8660254037844387076, 1.000000000000000000, 0.8660254037844387076, 1.000000000000000000, 0.8660254037844387076, 1.000000000000000000, 0.8660254037844387076, 1.000000000000000000, 0.8660254037844387076, 1.000000000000000000, 0.8660254037844387076, 1.000000000000000000, 0.8660254037844387076, 1.000000000000000000, 0.8660254037844387076, 1.000000000000000000) ) ) 
 REPRESENTATION_ITEM ( '' )  SURFACE ( )  );
#50564=CARTESIAN_POINT ( 'NONE',  ( 2.229367062499998831, -61.89583333196774362, -3.861377020970580887 ) ) ;
#50566=VERTEX_POINT ( 'NONE', #12132 ) ;
#50567=CARTESIAN_POINT ( 'NONE',  ( -6.972266317189433020E-16, -59.12499999726880873, -5.000000000000000000 ) ) ;
#50571=CARTESIAN_POINT ( 'NONE',  ( -4.458734124999998549, 5.770833334698927786, 2.574251347313722516 ) ) ;
#50572=CARTESIAN_POINT ( 'NONE',  ( -2.499999999999996447, -75.83333333333334281, 4.330127018922195425 ) ) ;
#50573=CARTESIAN_POINT ( 'NONE',  ( 1.846868145590735200, -159.2500000013656063, -4.458734124999999437 ) ) ;
#50575=VERTEX_POINT ( 'NONE', #23297 ) ;
#50579=CARTESIAN_POINT ( 'NONE',  ( 2.500000000000002220, 25.45833333606451987, 4.330127018922192761 ) ) ;
#50583=CARTESIAN_POINT ( 'NONE',  ( -2.500000000000000444, 5.833333333333333037, -4.330127018922193649 ) ) ;
#50586=CARTESIAN_POINT ( 'NONE',  ( -6.972266317189433020E-16, -82.12499999726881583, -5.000000000000000000 ) ) ;
#50589=CARTESIAN_POINT ( 'NONE',  ( -4.458734124999997661, 0.5208333346989266754, 2.574251347313722516 ) ) ;
#50592=CARTESIAN_POINT ( 'NONE',  ( 5.000000000000000000, -147.1250000027312126, 0.000000000000000000 ) ) ;
#50597=CARTESIAN_POINT ( 'NONE',  ( -3.535533905932738641, -140.3750000000000000, 3.535533905932737309 ) ) ;
#50599=CARTESIAN_POINT ( 'NONE',  ( -1.846868145590737420, -161.0000000013656063, 4.458734124999997661 ) ) ;
#50600=CARTESIAN_POINT ( 'NONE',  ( -2.071067811865372921, -159.4375000027312410, 5.000000000000104805 ) ) ;
#50602=CARTESIAN_POINT ( 'NONE',  ( -1.339745962155610925, -90.66965819600733312, 5.000000000000000000 ) ) ;
#50603=EDGE_LOOP ( 'NONE', ( #58628, #31036, #9976, #43340 ) ) ;
#50604=CARTESIAN_POINT ( 'NONE',  ( 2.229367062500001939, 23.77083333469892779, 3.861377020970579999 ) ) ;
#50609=CARTESIAN_POINT ( 'NONE',  ( 5.000000000000000000, 2.499999999999998668, -6.123233995736766282E-16 ) ) ;
#50610=CARTESIAN_POINT ( 'NONE',  ( 2.499999999999998668, 14.66666666666666607, -4.330127018922193649 ) ) ;
#50612=CARTESIAN_POINT ( 'NONE',  ( 4.458734124999999437, -52.81249999863440792, -5.460374474430324690E-16 ) ) ;
#50613=CARTESIAN_POINT ( 'NONE',  ( -3.152548672688508926E-16, -12.56249999863440081, -5.148502694627439702 ) ) ;
#50618=CARTESIAN_POINT ( 'NONE',  ( 0.000000000000000000, -170.0000000000000000, 0.000000000000000000 ) ) ;
#50619=CARTESIAN_POINT ( 'NONE',  ( -3.535250795749689387E-16, -34.25000000000000711, -5.773502691896257311 ) ) ;
#50623=CARTESIAN_POINT ( 'NONE',  ( -5.000000000000000000, -140.6250000027312126, -6.123233995736766282E-16 ) ) ;
#50624=CARTESIAN_POINT ( 'NONE',  ( 2.229367062499998831, -61.64583333196774362, -3.861377020970580887 ) ) ;
#50625=CARTESIAN_POINT ( 'NONE',  ( 1.846868145590736310, -150.8750000013655779, 4.458734124999999437 ) ) ;
#50627=CARTESIAN_POINT ( 'NONE',  ( -2.229367062499996610, -67.14583333196773651, 3.861377020970582219 ) ) ;
#50630=CARTESIAN_POINT ( 'NONE',  ( -4.999999999999999112, -57.79166666393548013, 2.886751345948131764 ) ) ;
#50636=CARTESIAN_POINT ( 'NONE',  ( 1.846868145590735200, -153.2500000013655779, -4.458734125000000326 ) ) ;
#50641=CARTESIAN_POINT ( 'NONE',  ( 9.457646018065525792E-16, -48.31249999863440081, 5.148502694627439702 ) ) ;
#50642=ORIENTED_EDGE ( 'NONE', *, *, #60597, .F. ) ;
#50645=CARTESIAN_POINT ( 'NONE',  ( 4.458734124999999437, 24.18750000136559564, -5.460374474430324690E-16 ) ) ;
#50649=ORIENTED_EDGE ( 'NONE', *, *, #57478, .F. ) ;
#50651=CARTESIAN_POINT ( 'NONE',  ( 1.339745962155661996, -28.16965819600733312, -4.999999999999970690 ) ) ;
#50654=CARTESIAN_POINT ( 'NONE',  ( -5.000000000000000000, -1.874999997268814944, 0.000000000000000000 ) ) ;
#50664=CARTESIAN_POINT ( 'NONE',  ( -5.000000000000000888, -155.5625000027311842, 2.071067811865474617 ) ) ;
#50665=ORIENTED_EDGE ( 'NONE', *, *, #6773, .F. ) ;
#50673=CARTESIAN_POINT ( 'NONE',  ( 4.458734125000000326, -17.89583333196773651, 2.574251347313718519 ) ) ;
#50674=DIRECTION ( 'NONE',  ( -0.000000000000000000, 1.000000000000000000, -0.000000000000000000 ) ) ;
#50675=CARTESIAN_POINT ( 'NONE',  ( 3.535533905932736864, -151.1250000000000000, 3.535533905932738641 ) ) ;
#50677=CARTESIAN_POINT ( 'NONE',  ( -8.190561711645485556E-16, -152.6875000013656063, 4.458734124999999437 ) ) ;
#50679=CARTESIAN_POINT ( 'NONE',  ( 2.229367062500001939, -46.22916666530106511, 3.861377020970579999 ) ) ;
#50682=CARTESIAN_POINT ( 'NONE',  ( -4.458734124999999437, -90.31249999863440792, 0.000000000000000000 ) ) ;
#50685=CARTESIAN_POINT ( 'NONE',  ( -4.458734124999999437, 5.604166668032262599, -2.574251347313719407 ) ) ;
#50687=CARTESIAN_POINT ( 'NONE',  ( 1.339745962155615144, 13.29465819873852084, 4.999999999999999112 ) ) ;
#50689=CARTESIAN_POINT ( 'NONE',  ( -4.458734124999999437, 14.35416666803226171, -2.574251347313719407 ) ) ;
#50691=CARTESIAN_POINT ( 'NONE',  ( 1.060575238724906964E-15, 5.375000002731184168, 5.773502691896257311 ) ) ;
#50692=ORIENTED_EDGE ( 'NONE', *, *, #31092, .F. ) ;
#50693=CARTESIAN_POINT ( 'NONE',  ( 3.535533905932736864, -162.2500000027312126, 3.535533905932738641 ) ) ;
#50695=CARTESIAN_POINT ( 'NONE',  ( 1.339745962155614256, 27.83034180399267044, -4.999999999999999112 ) ) ;
#50696=CARTESIAN_POINT ( 'NONE',  ( -2.229367062499996610, -43.14583333196773651, 3.861377020970582219 ) ) ;
#50697=CARTESIAN_POINT ( 'NONE',  ( 2.730187237215162345E-16, -162.4375000013655779, -4.458734124999999437 ) ) ;
#50699=CARTESIAN_POINT ( 'NONE',  ( 1.060575238724906964E-15, -37.62499999726881583, 5.773502691896257311 ) ) ;
#50701=CARTESIAN_POINT ( 'NONE',  ( -2.229367062500000163, -18.47916666530106866, -3.861377020970580443 ) ) ;
#50704=CARTESIAN_POINT ( 'NONE',  ( -3.535250795749689387E-16, -85.24999999999998579, -5.773502691896257311 ) ) ;
#50705=CARTESIAN_POINT ( 'NONE',  ( 3.152801135295366208, -164.5625000013656063, 3.152801135295367985 ) ) ;
#50706=CARTESIAN_POINT ( 'NONE',  ( -2.499999999999996447, -87.70833333060214443, 4.330127018922195425 ) ) ;
#50710=CARTESIAN_POINT ( 'NONE',  ( 9.457646018065525792E-16, -30.31249999863440436, 5.148502694627439702 ) ) ;
#50711=CARTESIAN_POINT ( 'NONE',  ( -6.972266317189433020E-16, -29.25000000000000000, -5.000000000000000000 ) ) ;
#50715=CARTESIAN_POINT ( 'NONE',  ( -6.972266317189433020E-16, -15.25000000000000000, -5.000000000000000000 ) ) ;
#50717=CARTESIAN_POINT ( 'NONE',  ( -6.972266317189433020E-16, -26.25000000000000000, -5.000000000000000000 ) ) ;
#50719=CARTESIAN_POINT ( 'NONE',  ( 2.229367062499998831, -82.89583333196773651, -3.861377020970580887 ) ) ;
#50722=CARTESIAN_POINT ( 'NONE',  ( 4.458734124999997661, -140.7500000013655779, 1.846868145590737864 ) ) ;
#50723=CARTESIAN_POINT ( 'NONE',  ( 0.000000000000000000, -170.0000000000000000, 5.000000000000000000 ) ) ;
#50725=CARTESIAN_POINT ( 'NONE',  ( -2.229367062499996610, -44.14583333196774362, 3.861377020970582219 ) ) ;
#50726=CARTESIAN_POINT ( 'NONE',  ( -2.498395430326213474E-14, 21.24999999999999289, 5.000000000000000000 ) ) ;
#50727=EDGE_CURVE ( 'NONE', #54333, #43422, #49629, .T. ) ;
#50729=DIRECTION ( 'NONE',  ( -0.000000000000000000, 1.000000000000000000, -0.000000000000000000 ) ) ;
#50734=CARTESIAN_POINT ( 'NONE',  ( 2.229367062499998831, -80.89583333196773651, -3.861377020970580887 ) ) ;
#50737=CARTESIAN_POINT ( 'NONE',  ( 0.000000000000000000, -170.0000000000000000, 0.000000000000000000 ) ) ;
#50740=CARTESIAN_POINT ( 'NONE',  ( 3.535533905932738197, -145.8750000000000000, -3.535533905932738197 ) ) ;
#50741=CARTESIAN_POINT ( 'NONE',  ( -6.972266317189433020E-16, -68.24999999999998579, -5.000000000000000000 ) ) ;
#50743=CARTESIAN_POINT ( 'NONE',  ( -3.535533905932738641, -168.5000000027312126, 3.535533905932737309 ) ) ;
#50745=CARTESIAN_POINT ( 'NONE',  ( 2.229367062500001939, 16.77083333469892779, 3.861377020970579999 ) ) ;
#50752=CARTESIAN_POINT ( 'NONE',  ( -2.499999999999996447, -13.70833333060214976, 4.330127018922195425 ) ) ;
#50753=CARTESIAN_POINT ( 'NONE',  ( -2.229367062500000163, -85.47916666530107932, -3.861377020970580443 ) ) ;
#50754=CARTESIAN_POINT ( 'NONE',  ( -2.229367062499996610, -5.145833331967740065, 3.861377020970582219 ) ) ;
#50757=CARTESIAN_POINT ( 'NONE',  ( -4.458734124999999437, -32.64583333196773651, -2.574251347313719407 ) ) ;
#50758=( BOUNDED_CURVE ( )  B_SPLINE_CURVE ( 2, ( #35648, #39499, #30815, #30490, #49156, #1255, #59135, #39181, #14738 ),
 .UNSPECIFIED., .F., .F. ) 
 B_SPLINE_CURVE_WITH_KNOTS ( ( 3, 2, 2, 2, 3 ),
 ( 0.6645833333333333037, 0.6652777777777777457, 0.6666666666666666297, 0.6680555555555555136, 0.6687499999999999556 ),
 .UNSPECIFIED. ) 
 CURVE ( )  GEOMETRIC_REPRESENTATION_ITEM ( )  RATIONAL_B_SPLINE_CURVE ( ( 0.9330127018922194093, 0.9330127018922194093, 1.000000000000000000, 0.8660254037844387076, 1.000000000000000000, 0.8660254037844387076, 1.000000000000000000, 0.9330127018922194093, 0.9330127018922194093 ) ) 
 REPRESENTATION_ITEM ( '' )  );
#50762=CARTESIAN_POINT ( 'NONE',  ( -4.458734124999998549, 19.77083333469892779, 2.574251347313722516 ) ) ;
#50764=EDGE_CURVE ( 'NONE', #54593, #46416, #11531, .T. ) ;
#50766=CARTESIAN_POINT ( 'NONE',  ( 2.500000000000002220, -28.66666666666666785, 4.330127018922192761 ) ) ;
#50767=CARTESIAN_POINT ( 'NONE',  ( 4.458734124999998549, -79.97916666530106511, -2.574251347313721627 ) ) ;
#50769=EDGE_CURVE ( 'NONE', #18978, #30981, #20167, .T. ) ;
#50771=CARTESIAN_POINT ( 'NONE',  ( -5.000000000000000000, 25.12500000273118417, 0.000000000000000000 ) ) ;
#50772=ORIENTED_EDGE ( 'NONE', *, *, #21251, .T. ) ;
#50774=CYLINDRICAL_SURFACE ( 'NONE', #9346, 5.000000000000000000 ) ;
#50776=CARTESIAN_POINT ( 'NONE',  ( -3.535250795749689387E-16, -25.25000000000000355, -5.773502691896257311 ) ) ;
#50777=CARTESIAN_POINT ( 'NONE',  ( -2.229367062500000163, -28.47916666530107221, -3.861377020970580443 ) ) ;
#50778=CARTESIAN_POINT ( 'NONE',  ( 4.458734125000000326, -88.89583333196773651, 2.574251347313718519 ) ) ;
#50779=EDGE_CURVE ( 'NONE', #50505, #34696, #41573, .T. ) ;
#50780=AXIS2_PLACEMENT_3D ( 'NONE', #40530, #39565, #59530 ) ;
#50781=CARTESIAN_POINT ( 'NONE',  ( 2.500000000000002220, -21.54166666393548013, 4.330127018922192761 ) ) ;
#50782=CARTESIAN_POINT ( 'NONE',  ( -4.458734124999998549, -56.22916666530107221, 2.574251347313722516 ) ) ;
#50785=CARTESIAN_POINT ( 'NONE',  ( 1.339745962155615144, -74.58034179853031276, 4.999999999999999112 ) ) ;
#50787=CARTESIAN_POINT ( 'NONE',  ( -4.458734124999998549, -2.479166665301069550, 2.574251347313722516 ) ) ;
#50789=CARTESIAN_POINT ( 'NONE',  ( -5.000000000000000000, -71.08333333333332860, -2.886751345948128211 ) ) ;
#50790=EDGE_CURVE ( 'NONE', #26750, #328, #3479, .T. ) ;
#50791=CARTESIAN_POINT ( 'NONE',  ( -3.152801135295367985, -152.0625000013655779, 3.152801135295367096 ) ) ;
#50793=CYLINDRICAL_SURFACE ( 'NONE', #33740, 5.000000000000000000 ) ;
#50794=( BOUNDED_CURVE ( )  B_SPLINE_CURVE ( 2, ( #37049, #36729, #9574, #47632, #22894, #56677, #46691, #37667, #12904 ),
 .UNSPECIFIED., .F., .F. ) 
 B_SPLINE_CURVE_WITH_KNOTS ( ( 3, 2, 2, 2, 3 ),
 ( 0.2687499999999999889, 0.2694444444444444309, 0.2708333333333333148, 0.2722222222222221988, 0.2729166666666666963 ),
 .UNSPECIFIED. ) 
 CURVE ( )  GEOMETRIC_REPRESENTATION_ITEM ( )  RATIONAL_B_SPLINE_CURVE ( ( 0.9330127018922194093, 0.9330127018922194093, 1.000000000000000000, 0.8660254037844387076, 1.000000000000000000, 0.8660254037844387076, 1.000000000000000000, 0.9330127018922167448, 0.9330127018922194093 ) ) 
 REPRESENTATION_ITEM ( '' )  );
#50795=CARTESIAN_POINT ( 'NONE',  ( -5.000000000000000000, -159.5000000000000000, -6.123233995736766282E-16 ) ) ;
#50797=CARTESIAN_POINT ( 'NONE',  ( 5.000000000000000000, -71.37499999726880162, -6.123233995736766282E-16 ) ) ;
#50798=CARTESIAN_POINT ( 'NONE',  ( 5.000000000000000888, -10.45833333060214443, 2.886751345948126879 ) ) ;
#50800=CARTESIAN_POINT ( 'NONE',  ( 4.458734124999998549, -17.97916666530106866, -2.574251347313721627 ) ) ;
#50801=CARTESIAN_POINT ( 'NONE',  ( 4.458734124999998549, -51.97916666530107221, -2.574251347313721627 ) ) ;
#50804=CARTESIAN_POINT ( 'NONE',  ( -3.152801135295367096, -145.0625000013655779, -3.152801135295367541 ) ) ;
#50806=VERTEX_POINT ( 'NONE', #17939 ) ;
#50808=CARTESIAN_POINT ( 'NONE',  ( 2.229367062500001939, 24.77083333469892779, 3.861377020970579999 ) ) ;
#50810=CARTESIAN_POINT ( 'NONE',  ( 2.500000000000002220, -50.66666666666666430, 4.330127018922192761 ) ) ;
#50814=CARTESIAN_POINT ( 'NONE',  ( -2.229367062500000163, -60.72916666530106511, -3.861377020970580443 ) ) ;
#50816=CARTESIAN_POINT ( 'NONE',  ( 2.229367062500001939, -8.979166665301075767, 3.861377020970579999 ) ) ;
#50818=CARTESIAN_POINT ( 'NONE',  ( 1.846868145590736310, -146.6250000013655779, 4.458734124999997661 ) ) ;
#50821=CARTESIAN_POINT ( 'NONE',  ( -6.972266317189433020E-16, -27.12499999726881228, -5.000000000000000000 ) ) ;
#50825=CARTESIAN_POINT ( 'NONE',  ( -6.972266317189433020E-16, -35.12499999726880873, -5.000000000000000000 ) ) ;
#50831=CARTESIAN_POINT ( 'NONE',  ( -1.339745962155613812, -90.08034179853029855, -5.000000000000000000 ) ) ;
#50834=CARTESIAN_POINT ( 'NONE',  ( -4.458734124999997661, 10.77083333469892956, 2.574251347313722516 ) ) ;
#50836=CARTESIAN_POINT ( 'NONE',  ( 2.229367062500001939, -13.22916666530107221, 3.861377020970579999 ) ) ;
#50838=CARTESIAN_POINT ( 'NONE',  ( -3.152801135295367985, -163.8125000013656063, 3.152801135295367096 ) ) ;
#50842=CARTESIAN_POINT ( 'NONE',  ( -2.499999999999996447, 10.16666666666666785, 4.330127018922195425 ) ) ;
#50844=CARTESIAN_POINT ( 'NONE',  ( 4.458734124999999437, -37.81249999863440792, -5.460374474430324690E-16 ) ) ;
#50845=ADVANCED_FACE ( 'NONE', ( #57518 ), #7991, .T. ) ;
#50853=DIRECTION ( 'NONE',  ( 0.000000000000000000, 0.000000000000000000, 1.000000000000000000 ) ) ;
#50854=CARTESIAN_POINT ( 'NONE',  ( -2.499999999999996447, -7.833333333333331261, 4.330127018922195425 ) ) ;
#50855=CARTESIAN_POINT ( 'NONE',  ( 4.458734124999999437, -73.81249999863440792, -5.460374474430324690E-16 ) ) ;
#50857=CARTESIAN_POINT ( 'NONE',  ( 1.060575238724906964E-15, -8.624999997268814056, 5.773502691896257311 ) ) ;
#50858=CARTESIAN_POINT ( 'NONE',  ( -3.152548672688508926E-16, -39.56249999863440081, -5.148502694627439702 ) ) ;
#50859=ORIENTED_EDGE ( 'NONE', *, *, #41306, .T. ) ;
#50861=CARTESIAN_POINT ( 'NONE',  ( 4.458734124999998549, 11.02083333469892779, -2.574251347313721627 ) ) ;
#50864=CARTESIAN_POINT ( 'NONE',  ( -5.000000000000000000, -54.08333333333332860, -2.886751345948128211 ) ) ;
#50868=CARTESIAN_POINT ( 'NONE',  ( -4.458734124999999437, -73.39583333196773651, -2.574251347313719407 ) ) ;
#50869=CARTESIAN_POINT ( 'NONE',  ( 3.535533905932738197, -168.8750000000000284, -3.535533905932738197 ) ) ;
#50871=CARTESIAN_POINT ( 'NONE',  ( -4.458734124999999437, -86.31249999863439371, 0.000000000000000000 ) ) ;
#50874=CARTESIAN_POINT ( 'NONE',  ( -4.458734124999998549, -33.47916666530107221, 2.574251347313722516 ) ) ;
#50875=EDGE_CURVE ( 'NONE', #53932, #61278, #32422, .T. ) ;
#50877=ORIENTED_EDGE ( 'NONE', *, *, #8217, .F. ) ;
#50882=CARTESIAN_POINT ( 'NONE',  ( -2.499999999999996447, -18.70833333060214798, 4.330127018922195425 ) ) ;
#50883=CARTESIAN_POINT ( 'NONE',  ( 2.229367062499998831, -65.89583333196773651, -3.861377020970580887 ) ) ;
#50885=ORIENTED_EDGE ( 'NONE', *, *, #39714, .F. ) ;
#50887=( BOUNDED_CURVE ( )  B_SPLINE_CURVE ( 2, ( #52873, #29035, #23913, #28422, #4600, #39014, #50583, #54458, #428 ),
 .UNSPECIFIED., .F., .F. ) 
 B_SPLINE_CURVE_WITH_KNOTS ( ( 3, 2, 2, 2, 3 ),
 ( 0.1979166666666666574, 0.1986111111111110994, 0.2000000000000000111, 0.2013888888888888951, 0.2020833333333333370 ),
 .UNSPECIFIED. ) 
 CURVE ( )  GEOMETRIC_REPRESENTATION_ITEM ( )  RATIONAL_B_SPLINE_CURVE ( ( 0.9330127018922194093, 0.9330127018922194093, 1.000000000000000000, 0.8660254037844387076, 1.000000000000000000, 0.8660254037844387076, 1.000000000000000000, 0.9330127018922194093, 0.9330127018922194093 ) ) 
 REPRESENTATION_ITEM ( '' )  );
#50889=VERTEX_POINT ( 'NONE', #53844 ) ;
#50891=CARTESIAN_POINT ( 'NONE',  ( 4.458734125000001214, 6.104166668032262599, 2.574251347313718519 ) ) ;
#50893=CARTESIAN_POINT ( 'NONE',  ( 3.152801135295366208, -162.5625000013656063, 3.152801135295367985 ) ) ;
#50895=ORIENTED_EDGE ( 'NONE', *, *, #42915, .F. ) ;
#50901=DIRECTION ( 'NONE',  ( -0.000000000000000000, 1.000000000000000000, -0.000000000000000000 ) ) ;
#50904=CARTESIAN_POINT ( 'NONE',  ( -4.458734124999999437, 25.68750000136559208, 0.000000000000000000 ) ) ;
#50907=CARTESIAN_POINT ( 'NONE',  ( 4.458734124999999437, 0.9375000013655959696, -5.460374474430324690E-16 ) ) ;
#50910=CARTESIAN_POINT ( 'NONE',  ( -3.535533905932737309, -146.7500000027311842, -3.535533905932738197 ) ) ;
#50916=EDGE_CURVE ( 'NONE', #46199, #63065, #48153, .T. ) ;
#50919=CARTESIAN_POINT ( 'NONE',  ( -8.190561711645485556E-16, -162.9375000013655779, 4.458734124999999437 ) ) ;
#50920=CARTESIAN_POINT ( 'NONE',  ( -5.000000000000000000, -159.6250000027311842, -6.123233995736766282E-16 ) ) ;
#50922=CARTESIAN_POINT ( 'NONE',  ( -1.846868145590737420, -139.7500000013655779, 4.458734124999999437 ) ) ;
#50925=CARTESIAN_POINT ( 'NONE',  ( -4.458734124999999437, 24.35416666803225993, -2.574251347313719407 ) ) ;
#50931=CARTESIAN_POINT ( 'NONE',  ( -2.499999999999996447, 7.166666666666665186, 4.330127018922195425 ) ) ;
#50932=CARTESIAN_POINT ( 'NONE',  ( 4.458734124999999437, -54.81249999863440081, -5.460374474430324690E-16 ) ) ;
#50934=CARTESIAN_POINT ( 'NONE',  ( 2.229367062500001939, -8.979166665301075767, 3.861377020970579999 ) ) ;
#50935=CARTESIAN_POINT ( 'NONE',  ( 2.500000000000002220, -6.666666666666667851, 4.330127018922192761 ) ) ;
#50937=CARTESIAN_POINT ( 'NONE',  ( 0.000000000000000000, -170.0000000000000000, 0.000000000000000000 ) ) ;
#50939=CARTESIAN_POINT ( 'NONE',  ( -4.999999999999999112, -35.91666666666666430, 2.886751345948131764 ) ) ;
#50940=CARTESIAN_POINT ( 'NONE',  ( 1.255007937094098239E-14, 23.87500000273118062, -4.999999999999999112 ) ) ;
#50941=CARTESIAN_POINT ( 'NONE',  ( -5.000000000000000000, 14.91666666666666607, -2.886751345948128211 ) ) ;
#50945=CARTESIAN_POINT ( 'NONE',  ( 4.458734125000001214, -57.89583333196773651, 2.574251347313718519 ) ) ;
#50946=CARTESIAN_POINT ( 'NONE',  ( -1.846868145590734756, -152.3750000013655779, -4.458734125000000326 ) ) ;
#50947=CARTESIAN_POINT ( 'NONE',  ( 4.458734124999998549, -70.72916666530107932, -2.574251347313721627 ) ) ;
#50949=CARTESIAN_POINT ( 'NONE',  ( 4.458734124999999437, -22.06249999863440436, -5.460374474430324690E-16 ) ) ;
#50950=CARTESIAN_POINT ( 'NONE',  ( -5.000000000000000000, -58.95833333060213732, -2.886751345948128211 ) ) ;
#50951=ORIENTED_EDGE ( 'NONE', *, *, #13645, .T. ) ;
#50953=ORIENTED_EDGE ( 'NONE', *, *, #17739, .T. ) ;
#50957=CARTESIAN_POINT ( 'NONE',  ( -4.458734125000000326, -151.0000000013656063, -1.846868145590735644 ) ) ;
#50961=CARTESIAN_POINT ( 'NONE',  ( 1.975475456537005874E-15, -8.750000000000000000, 5.000000000000000000 ) ) ;
#50962=CARTESIAN_POINT ( 'NONE',  ( -4.458734124999999437, -48.56249999863440792, 0.000000000000000000 ) ) ;
#50966=CARTESIAN_POINT ( 'NONE',  ( -2.229367062499996610, 22.85416666803225993, 3.861377020970582219 ) ) ;
#50968=CARTESIAN_POINT ( 'NONE',  ( 5.000000000000000000, -13.37499999726881050, -6.123233995736766282E-16 ) ) ;
#50969=DIRECTION ( 'NONE',  ( -0.000000000000000000, 1.000000000000000000, -0.000000000000000000 ) ) ;
#50971=EDGE_LOOP ( 'NONE', ( #5861, #24200, #26233, #4967 ) ) ;
#50975=EDGE_CURVE ( 'NONE', #5037, #43626, #54743, .T. ) ;
#50976=VECTOR ( 'NONE', #43701, 1000.000000000000000 ) ;
#50979=CARTESIAN_POINT ( 'NONE',  ( -2.071067811865351604, -157.3125000000000284, 5.000000000000126121 ) ) ;
#50984=CARTESIAN_POINT ( 'NONE',  ( 0.000000000000000000, -170.0000000000000000, 0.000000000000000000 ) ) ;
#50986=ORIENTED_EDGE ( 'NONE', *, *, #35911, .T. ) ;
#50988=CARTESIAN_POINT ( 'NONE',  ( 6.123233995736766282E-16, -170.0000000000000000, -5.000000000000000000 ) ) ;
#50990=CARTESIAN_POINT ( 'NONE',  ( 2.071067811865475505, -156.9375000027312126, -5.000000000000000888 ) ) ;
#50991=VERTEX_POINT ( 'NONE', #60285 ) ;
#51000=CARTESIAN_POINT ( 'NONE',  ( 4.458734124999998549, -24.72916666530106866, -2.574251347313721627 ) ) ;
#51002=CARTESIAN_POINT ( 'NONE',  ( -5.000000000000000000, -150.5000000000000284, -6.123233995736766282E-16 ) ) ;
#51004=CARTESIAN_POINT ( 'NONE',  ( 3.152801135295366208, -153.5625000013656063, 3.152801135295367985 ) ) ;
#51005=VERTEX_POINT ( 'NONE', #25536 ) ;
#51006=CARTESIAN_POINT ( 'NONE',  ( 9.457646018065525792E-16, -52.31249999863440792, 5.148502694627439702 ) ) ;
#51009=CARTESIAN_POINT ( 'NONE',  ( 5.000000000000000000, 22.58333333333333570, -2.886751345948129988 ) ) ;
#51011=CARTESIAN_POINT ( 'NONE',  ( -3.152548672688508926E-16, 5.437500001365592084, -5.148502694627439702 ) ) ;
#51012=CARTESIAN_POINT ( 'NONE',  ( 1.975475456537005874E-15, 13.24999999999999822, 5.000000000000000000 ) ) ;
#51013=CARTESIAN_POINT ( 'NONE',  ( -6.972266317189433020E-16, -7.249999999999998224, -5.000000000000000000 ) ) ;
#51014=CARTESIAN_POINT ( 'NONE',  ( 4.458734124999998549, 17.02083333469892423, -2.574251347313721627 ) ) ;
#51015=CARTESIAN_POINT ( 'NONE',  ( 5.000000000000000000, 5.625000002731185056, -6.123233995736766282E-16 ) ) ;
#51018=ORIENTED_EDGE ( 'NONE', *, *, #8728, .F. ) ;
#51019=AXIS2_PLACEMENT_3D ( 'NONE', #24942, #14640, #49378 ) ;
#51020=DIRECTION ( 'NONE',  ( 0.000000000000000000, 0.000000000000000000, 1.000000000000000000 ) ) ;
#51021=CARTESIAN_POINT ( 'NONE',  ( 4.458734124999999437, -42.81249999863440081, -5.460374474430324690E-16 ) ) ;
#51022=CARTESIAN_POINT ( 'NONE',  ( -4.458734125000001214, -165.1250000013656063, 1.846868145590734089 ) ) ;
#51025=CARTESIAN_POINT ( 'NONE',  ( 5.000000000000000000, -45.29166666393546592, -2.886751345948129988 ) ) ;
#51027=CARTESIAN_POINT ( 'NONE',  ( -4.458734124999999437, -17.39583333196773651, -2.574251347313719407 ) ) ;
#51028=VERTEX_POINT ( 'NONE', #59969 ) ;
#51029=CARTESIAN_POINT ( 'NONE',  ( -5.000000000000000000, -89.08333333333334281, -2.886751345948128211 ) ) ;
#51030=CARTESIAN_POINT ( 'NONE',  ( 3.152801135295366208, -165.5625000013656063, 3.152801135295367985 ) ) ;
#51031=CARTESIAN_POINT ( 'NONE',  ( -5.000000000000000000, -34.95833333060213732, -2.886751345948128211 ) ) ;
#51034=CARTESIAN_POINT ( 'NONE',  ( 2.229367062499998831, -31.89583333196773651, -3.861377020970580887 ) ) ;
#51035=CARTESIAN_POINT ( 'NONE',  ( -1.339745962155623360, 20.33034180399266333, 4.999999999999991118 ) ) ;
#51036=EDGE_LOOP ( 'NONE', ( #777, #41052, #22933 ) ) ;
#51043=CARTESIAN_POINT ( 'NONE',  ( -4.458734124999999437, -79.64583333196772230, -2.574251347313719407 ) ) ;
#51045=DIRECTION ( 'NONE',  ( 0.000000000000000000, 0.000000000000000000, 1.000000000000000000 ) ) ;
#51046=CARTESIAN_POINT ( 'NONE',  ( -1.846868145590737420, -143.0000000013655779, 4.458734124999997661 ) ) ;
#51047=CARTESIAN_POINT ( 'NONE',  ( -4.999999999999998224, 6.208333336064520758, 2.886751345948131764 ) ) ;
#51049=CARTESIAN_POINT ( 'NONE',  ( 4.458734124999998549, -46.72916666530106511, -2.574251347313721627 ) ) ;
#51050=CARTESIAN_POINT ( 'NONE',  ( -1.339745962155613812, 20.79465819873852084, -5.000000000000000000 ) ) ;
#51053=CARTESIAN_POINT ( 'NONE',  ( 0.000000000000000000, -170.0000000000000000, 5.000000000000000000 ) ) ;
#51056=CARTESIAN_POINT ( 'NONE',  ( -1.339745962155613812, -73.20534180126146850, -5.000000000000000000 ) ) ;
#51058=CARTESIAN_POINT ( 'NONE',  ( 4.458734124999998549, -81.97916666530106511, -2.574251347313721627 ) ) ;
#51069=CARTESIAN_POINT ( 'NONE',  ( 4.458734124999999437, 11.93750000136559564, -5.460374474430324690E-16 ) ) ;
#51070=CARTESIAN_POINT ( 'NONE',  ( 1.339745962155615144, -77.58034179853028434, 4.999999999999999112 ) ) ;
#51072=( BOUNDED_CURVE ( )  B_SPLINE_CURVE ( 2, ( #6825, #36725, #50882, #55715, #12588, #52150, #27069, #32201, #26431 ),
 .UNSPECIFIED., .F., .F. ) 
 B_SPLINE_CURVE_WITH_KNOTS ( ( 3, 2, 2, 2, 3 ),
 ( 0.3979166666666666963, 0.3986111111111111382, 0.4000000000000000222, 0.4013888888888889062, 0.4020833333333333481 ),
 .UNSPECIFIED. ) 
 CURVE ( )  GEOMETRIC_REPRESENTATION_ITEM ( )  RATIONAL_B_SPLINE_CURVE ( ( 0.9330127018922194093, 0.9330127018922220739, 1.000000000000000000, 0.8660254037844387076, 1.000000000000000000, 0.8660254037844387076, 1.000000000000000000, 0.9330127018922194093, 0.9330127018922194093 ) ) 
 REPRESENTATION_ITEM ( '' )  );
#51074=EDGE_CURVE ( 'NONE', #21872, #25868, #21355, .T. ) ;
#51078=EDGE_CURVE ( 'NONE', #10933, #35595, #24672, .T. ) ;
#51080=CARTESIAN_POINT ( 'NONE',  ( -2.071067811865538566, -163.6875000000000000, -4.999999999999937828 ) ) ;
#51081=CARTESIAN_POINT ( 'NONE',  ( 4.458734124999999437, -85.81249999863439371, -5.460374474430324690E-16 ) ) ;
#51082=CARTESIAN_POINT ( 'NONE',  ( 4.458734124999998549, -5.729166665301072214, -2.574251347313721627 ) ) ;
#51085=CARTESIAN_POINT ( 'NONE',  ( -2.229367062499996610, -37.39583333196773651, 3.861377020970582219 ) ) ;
#51089=EDGE_CURVE ( 'NONE', #46416, #34465, #19781, .T. ) ;
#51090=CARTESIAN_POINT ( 'NONE',  ( 9.457646018065525792E-16, 21.93750000136559208, 5.148502694627439702 ) ) ;
#51091=CARTESIAN_POINT ( 'NONE',  ( 5.000000000000000888, -53.58333333333333570, 2.886751345948126879 ) ) ;
#51092=CARTESIAN_POINT ( 'NONE',  ( -5.000000000000000000, -25.87499999726881583, 0.000000000000000000 ) ) ;
#51093=CARTESIAN_POINT ( 'NONE',  ( -4.458734124999997661, -80.47916666530105090, 2.574251347313722516 ) ) ;
#51096=CARTESIAN_POINT ( 'NONE',  ( -4.999999999999999112, 18.20833333606451987, 2.886751345948131764 ) ) ;
#51099=CARTESIAN_POINT ( 'NONE',  ( -3.535533905932738641, -149.3750000000000000, 3.535533905932737309 ) ) ;
#51100=CARTESIAN_POINT ( 'NONE',  ( 2.500000000000002220, -24.66666666666666430, 4.330127018922192761 ) ) ;
#51101=CARTESIAN_POINT ( 'NONE',  ( 9.457646018065525792E-16, -27.06249999863440081, 5.148502694627439702 ) ) ;
#51102=CARTESIAN_POINT ( 'NONE',  ( 2.229367062500001939, -87.97916666530107932, 3.861377020970579999 ) ) ;
#51103=CARTESIAN_POINT ( 'NONE',  ( -3.535250795749689387E-16, -26.12499999726881583, -5.773502691896257311 ) ) ;
#51105=CARTESIAN_POINT ( 'NONE',  ( -2.229367062500000163, -53.47916666530107221, -3.861377020970580443 ) ) ;
#51107=CARTESIAN_POINT ( 'NONE',  ( 2.500000000000002220, -49.66666666666666430, 4.330127018922192761 ) ) ;
#51108=CARTESIAN_POINT ( 'NONE',  ( -6.972266317189433020E-16, -18.25000000000000000, -5.000000000000000000 ) ) ;
#51109=CARTESIAN_POINT ( 'NONE',  ( -2.229367062499996610, -4.395833331967740065, 3.861377020970582219 ) ) ;
#51110=ORIENTED_EDGE ( 'NONE', *, *, #18173, .T. ) ;
#51111=CARTESIAN_POINT ( 'NONE',  ( -5.000000000000000000, -73.00000000000000000, 0.000000000000000000 ) ) ;
#51115=CARTESIAN_POINT ( 'NONE',  ( -2.499999999999996447, -71.70833333060214443, 4.330127018922195425 ) ) ;
#51119=CARTESIAN_POINT ( 'NONE',  ( 4.458734125000001214, -18.14583333196773651, 2.574251347313718519 ) ) ;
#51121=CARTESIAN_POINT ( 'NONE',  ( 9.457646018065525792E-16, -51.31249999863440792, 5.148502694627439702 ) ) ;
#51124=CARTESIAN_POINT ( 'NONE',  ( -4.458734125000000326, -169.2500000013655779, -1.846868145590735644 ) ) ;
#51126=CYLINDRICAL_SURFACE ( 'NONE', #53300, 5.000000000000000000 ) ;
#51128=ORIENTED_EDGE ( 'NONE', *, *, #4296, .T. ) ;
#51129=LINE ( 'NONE', #60785, #2636 ) ;
#51130=CARTESIAN_POINT ( 'NONE',  ( 4.458734124999999437, 23.93750000136559564, -5.460374474430324690E-16 ) ) ;
#51132=CYLINDRICAL_SURFACE ( 'NONE', #62008, 5.000000000000000000 ) ;
#51133=EDGE_CURVE ( 'NONE', #31959, #53780, #1754, .T. ) ;
#51137=EDGE_CURVE ( 'NONE', #44836, #40158, #31247, .T. ) ;
#51138=CARTESIAN_POINT ( 'NONE',  ( -4.458734124999999437, -150.1875000013656063, -5.460374474430324690E-16 ) ) ;
#51141=CARTESIAN_POINT ( 'NONE',  ( 4.458734125000001214, -62.14583333196774362, 2.574251347313718519 ) ) ;
#51142=DIRECTION ( 'NONE',  ( -1.000000000000000000, 0.000000000000000000, -0.000000000000000000 ) ) ;
#51144=CARTESIAN_POINT ( 'NONE',  ( -3.152801135295367985, -145.8125000013655779, 3.152801135295367096 ) ) ;
#51146=VERTEX_POINT ( 'NONE', #41584 ) ;
#51148=CYLINDRICAL_SURFACE ( 'NONE', #19536, 5.000000000000000000 ) ;
#51151=CARTESIAN_POINT ( 'NONE',  ( -2.229367062500000163, 29.27083333469892779, -3.861377020970580443 ) ) ;
#51153=CARTESIAN_POINT ( 'NONE',  ( -5.000000000000000000, -6.083333333333336590, -2.886751345948128211 ) ) ;
#51158=CARTESIAN_POINT ( 'NONE',  ( 1.975475456537005874E-15, -56.62499999726880162, 5.000000000000000000 ) ) ;
#51161=CARTESIAN_POINT ( 'NONE',  ( 2.229367062499998831, 11.35416666803225993, -3.861377020970580887 ) ) ;
#51163=CARTESIAN_POINT ( 'NONE',  ( -4.458734124999999437, -13.64583333196774184, -2.574251347313719407 ) ) ;
#51165=CARTESIAN_POINT ( 'NONE',  ( 1.846868145590736310, -161.6250000013656063, 4.458734124999999437 ) ) ;
#51166=CARTESIAN_POINT ( 'NONE',  ( -6.972266317189433020E-16, -38.25000000000000000, -5.000000000000000000 ) ) ;
#51170=LINE ( 'NONE', #18245, #21406 ) ;
#51172=CARTESIAN_POINT ( 'NONE',  ( -3.152548672688508926E-16, -33.56249999863440792, -5.148502694627439702 ) ) ;
#51173=CARTESIAN_POINT ( 'NONE',  ( 0.000000000000000000, -170.0000000000000000, 5.000000000000000000 ) ) ;
#51176=CARTESIAN_POINT ( 'NONE',  ( 5.000000000000000000, -89.41666666666665719, -2.886751345948130876 ) ) ;
#51180=( BOUNDED_CURVE ( )  B_SPLINE_CURVE ( 2, ( #22826, #4144, #48191, #18298, #47261, #63008, #22506, #42101, #3206 ),
 .UNSPECIFIED., .F., .T. ) 
 B_SPLINE_CURVE_WITH_KNOTS ( ( 3, 2, 2, 2, 3 ),
 ( 0.5979166666666666519, 0.5986111111111110938, 0.5999999999999999778, 0.6013888888888888618, 0.6020833333333333037 ),
 .UNSPECIFIED. ) 
 CURVE ( )  GEOMETRIC_REPRESENTATION_ITEM ( )  RATIONAL_B_SPLINE_CURVE ( ( 0.9330127018922194093, 0.9330127018922194093, 1.000000000000000000, 0.8660254037844387076, 1.000000000000000000, 0.8660254037844387076, 1.000000000000000000, 0.9330127018922194093, 0.9330127018922194093 ) ) 
 REPRESENTATION_ITEM ( '' )  );
#51181=FACE_OUTER_BOUND ( 'NONE', #52485, .T. ) ;
#51182=CARTESIAN_POINT ( 'NONE',  ( -4.999999999999999112, -5.916666666666666963, 2.886751345948131764 ) ) ;
#51183=CARTESIAN_POINT ( 'NONE',  ( -2.229367062500000163, -70.47916666530107932, -3.861377020970580443 ) ) ;
#51185=CARTESIAN_POINT ( 'NONE',  ( -5.000000000000000000, -4.958333330602147981, -2.886751345948128211 ) ) ;
#51186=CARTESIAN_POINT ( 'NONE',  ( -4.458734124999999437, -38.31249999863439371, 0.000000000000000000 ) ) ;
#51189=CARTESIAN_POINT ( 'NONE',  ( 9.457646018065525792E-16, 14.68750000136559208, 5.148502694627439702 ) ) ;
#51191=CARTESIAN_POINT ( 'NONE',  ( 5.000000000000000888, -81.45833333060213022, 2.886751345948126879 ) ) ;
#51192=CARTESIAN_POINT ( 'NONE',  ( 1.060575238724906964E-15, -54.75000000000000000, 5.773502691896257311 ) ) ;
#51193=CARTESIAN_POINT ( 'NONE',  ( 1.846868145590736310, -161.8750000013656063, 4.458734124999999437 ) ) ;
#51195=DIRECTION ( 'NONE',  ( -0.000000000000000000, 1.000000000000000000, -0.000000000000000000 ) ) ;
#51196=CARTESIAN_POINT ( 'NONE',  ( 2.229367062499998831, -75.64583333196773651, -3.861377020970580887 ) ) ;
#51197=CARTESIAN_POINT ( 'NONE',  ( -5.000000000000000888, -168.4375000000000568, 2.071067811865474617 ) ) ;
#51198=CARTESIAN_POINT ( 'NONE',  ( 2.229367062499998831, -88.64583333196773651, -3.861377020970580887 ) ) ;
#51200=CARTESIAN_POINT ( 'NONE',  ( -4.458734124999999437, -34.64583333196773651, -2.574251347313719407 ) ) ;
#51202=ORIENTED_EDGE ( 'NONE', *, *, #28756, .T. ) ;
#51208=LINE ( 'NONE', #16466, #42475 ) ;
#51209=CARTESIAN_POINT ( 'NONE',  ( -4.458734124999998549, -66.47916666530106511, 2.574251347313722516 ) ) ;
#51217=CARTESIAN_POINT ( 'NONE',  ( -2.229367062499996610, 9.854166668032261711, 3.861377020970582219 ) ) ;
#51218=FACE_OUTER_BOUND ( 'NONE', #53670, .T. ) ;
#51219=CARTESIAN_POINT ( 'NONE',  ( 4.458734124999999437, -158.4375000013655779, 0.000000000000000000 ) ) ;
#51227=CARTESIAN_POINT ( 'NONE',  ( -9.184850993605147944E-16, -140.2500000000000000, 5.000000000000000000 ) ) ;
#51229=CARTESIAN_POINT ( 'NONE',  ( 6.123233995736766282E-16, -170.0000000000000000, -5.000000000000000000 ) ) ;
#51232=CARTESIAN_POINT ( 'NONE',  ( -4.458734124999999437, 29.68750000136559208, 0.000000000000000000 ) ) ;
#51233=EDGE_CURVE ( 'NONE', #35553, #27844, #61706, .T. ) ;
#51236=CARTESIAN_POINT ( 'NONE',  ( -2.229367062499996610, -0.3958333319677397322, 3.861377020970582219 ) ) ;
#51237=CARTESIAN_POINT ( 'NONE',  ( 0.000000000000000000, -170.0000000000000000, 5.000000000000000000 ) ) ;
#51239=EDGE_CURVE ( 'NONE', #16219, #59810, #44381, .T. ) ;
#51240=CARTESIAN_POINT ( 'NONE',  ( 2.071067811865475505, -146.9375000027311842, -5.000000000000000888 ) ) ;
#51241=CARTESIAN_POINT ( 'NONE',  ( 1.339745962155612702, -33.16965819600733312, -5.000000000000000000 ) ) ;
#51245=DIRECTION ( 'NONE',  ( 0.000000000000000000, 0.000000000000000000, 1.000000000000000000 ) ) ;
#51249=CARTESIAN_POINT ( 'NONE',  ( -4.458734124999999437, -163.2500000013656063, -1.846868145590735644 ) ) ;
#51252=CARTESIAN_POINT ( 'NONE',  ( 2.730187237215162345E-16, -141.1875000013656063, -4.458734124999999437 ) ) ;
#51254=CARTESIAN_POINT ( 'NONE',  ( 2.229367062499998831, 22.10416666803225993, -3.861377020970580887 ) ) ;
#51255=EDGE_LOOP ( 'NONE', ( #54289, #19771, #7743, #56256 ) ) ;
#51258=AXIS2_PLACEMENT_3D ( 'NONE', #36455, #12002, #31630 ) ;
#51261=CARTESIAN_POINT ( 'NONE',  ( -4.999999999999999112, 8.083333333333330373, 2.886751345948131764 ) ) ;
#51263=CARTESIAN_POINT ( 'NONE',  ( -2.229367062499996610, -55.14583333196773651, 3.861377020970582219 ) ) ;
#51265=CYLINDRICAL_SURFACE ( 'NONE', #61182, 5.000000000000000000 ) ;
#51267=CARTESIAN_POINT ( 'NONE',  ( -4.999999999999998224, 0.2083333360645180099, 2.886751345948131764 ) ) ;
#51269=CARTESIAN_POINT ( 'NONE',  ( 1.060575238724906964E-15, -41.74999999999999289, 5.773502691896257311 ) ) ;
#51270=CARTESIAN_POINT ( 'NONE',  ( -2.499999999999996447, 13.29166666939785379, 4.330127018922195425 ) ) ;
#51271=CARTESIAN_POINT ( 'NONE',  ( -4.999999999999998224, -44.91666666666666430, 2.886751345948131764 ) ) ;
#51274=CARTESIAN_POINT ( 'NONE',  ( -4.458734124999998549, -59.22916666530106511, 2.574251347313722516 ) ) ;
#51275=CARTESIAN_POINT ( 'NONE',  ( 1.846868145590736310, -152.8750000013655779, 4.458734124999999437 ) ) ;
#51276=CARTESIAN_POINT ( 'NONE',  ( -2.229367062500000163, -69.47916666530107932, -3.861377020970580443 ) ) ;
#51278=CARTESIAN_POINT ( 'NONE',  ( 2.229367062499998831, -20.89583333196774007, -3.861377020970580887 ) ) ;
#51280=CARTESIAN_POINT ( 'NONE',  ( 2.500000000000002220, -63.54166666393547303, 4.330127018922192761 ) ) ;
#51283=ORIENTED_EDGE ( 'NONE', *, *, #57306, .T. ) ;
#51287=CARTESIAN_POINT ( 'NONE',  ( -3.152801135295367096, -151.0625000013655779, -3.152801135295367541 ) ) ;
#51292=CARTESIAN_POINT ( 'NONE',  ( -2.229367062500000163, -49.72916666530107221, -3.861377020970580443 ) ) ;
#51293=ORIENTED_EDGE ( 'NONE', *, *, #443, .T. ) ;
#51296=CARTESIAN_POINT ( 'NONE',  ( 4.458734124999999437, 22.18750000136559564, -5.460374474430324690E-16 ) ) ;
#51299=CARTESIAN_POINT ( 'NONE',  ( -4.458734124999999437, -168.0000000013656347, -1.846868145590735644 ) ) ;
#51305=CARTESIAN_POINT ( 'NONE',  ( 5.000000000000000888, -157.0625000027311842, -2.071067811865475505 ) ) ;
#51309=DIRECTION ( 'NONE',  ( 0.8660254037844313801, -0.5000000000000125455, 0.000000000000000000 ) ) ;
#51312=VERTEX_POINT ( 'NONE', #23878 ) ;
#51315=CARTESIAN_POINT ( 'NONE',  ( 2.071067811865475505, -158.9375000027311842, -5.000000000000000888 ) ) ;
#51316=ORIENTED_EDGE ( 'NONE', *, *, #23681, .F. ) ;
#51321=CARTESIAN_POINT ( 'NONE',  ( 3.061616997868383141E-16, -148.7500000000000284, -5.000000000000000000 ) ) ;
#51324=CARTESIAN_POINT ( 'NONE',  ( -4.999999999999998224, -89.91666666666667140, 2.886751345948131764 ) ) ;
#51325=CARTESIAN_POINT ( 'NONE',  ( -2.229367062499996610, -24.14583333196773651, 3.861377020970582219 ) ) ;
#51327=CARTESIAN_POINT ( 'NONE',  ( 5.000000000000000000, -151.0000000000000284, 0.000000000000000000 ) ) ;
#51329=CARTESIAN_POINT ( 'NONE',  ( -1.846868145590734756, -151.1250000013655779, -4.458734125000000326 ) ) ;
#51331=CARTESIAN_POINT ( 'NONE',  ( 2.229367062500001939, -52.22916666530107221, 3.861377020970579999 ) ) ;
#51333=CARTESIAN_POINT ( 'NONE',  ( 1.975475456537005874E-15, -58.62499999726879452, 5.000000000000000000 ) ) ;
#51335=CARTESIAN_POINT ( 'NONE',  ( 2.499999999999998668, 26.66666666666666430, -4.330127018922193649 ) ) ;
#51337=CARTESIAN_POINT ( 'NONE',  ( 4.458734124999999437, 4.187500001365595637, -5.460374474430324690E-16 ) ) ;
#51338=CARTESIAN_POINT ( 'NONE',  ( 3.061616997868383141E-16, -142.7500000000000284, -5.000000000000000000 ) ) ;
#51339=CARTESIAN_POINT ( 'NONE',  ( 2.500000000000002220, -41.54166666393548013, 4.330127018922192761 ) ) ;
#51341=CARTESIAN_POINT ( 'NONE',  ( 9.457646018065525792E-16, 14.68750000136559208, 5.148502694627439702 ) ) ;
#51342=CARTESIAN_POINT ( 'NONE',  ( 5.000000000000000888, 2.541666669397851130, 2.886751345948126879 ) ) ;
#51343=VERTEX_POINT ( 'NONE', #18728 ) ;
#51346=CARTESIAN_POINT ( 'NONE',  ( -4.999999999999998224, -70.91666666666667140, 2.886751345948131764 ) ) ;
#51347=CARTESIAN_POINT ( 'NONE',  ( -4.458734124999998549, -41.22916666530107221, 2.574251347313722516 ) ) ;
#51348=CARTESIAN_POINT ( 'NONE',  ( 1.846868145590736310, -165.8750000013656063, 4.458734124999999437 ) ) ;
#51350=CARTESIAN_POINT ( 'NONE',  ( 5.000000000000000000, -47.29166666393547303, -2.886751345948129988 ) ) ;
#51351=VERTEX_POINT ( 'NONE', #38353 ) ;
#51352=CARTESIAN_POINT ( 'NONE',  ( 9.457646018065525792E-16, -17.06249999863440792, 5.148502694627439702 ) ) ;
#51353=EDGE_LOOP ( 'NONE', ( #22255, #60753, #33856, #52372 ) ) ;
#51354=CARTESIAN_POINT ( 'NONE',  ( 2.499999999999998668, -86.33333333333332860, -4.330127018922193649 ) ) ;
#51355=CARTESIAN_POINT ( 'NONE',  ( -1.846868145590734756, -163.1250000013656063, -4.458734125000000326 ) ) ;
#51356=VERTEX_POINT ( 'NONE', #57359 ) ;
#51358=CARTESIAN_POINT ( 'NONE',  ( -4.458734124999999437, -32.56249999863440792, 0.000000000000000000 ) ) ;
#51360=ORIENTED_EDGE ( 'NONE', *, *, #13457, .T. ) ;
#51363=CARTESIAN_POINT ( 'NONE',  ( -5.000000000000000000, -28.95833333060214443, -2.886751345948128211 ) ) ;
#51364=VERTEX_POINT ( 'NONE', #24508 ) ;
#51365=CARTESIAN_POINT ( 'NONE',  ( -5.000000000000000888, -161.4375000000000000, 2.071067811865474617 ) ) ;
#51367=CARTESIAN_POINT ( 'NONE',  ( -4.458734124999998549, -80.47916666530106511, 2.574251347313722516 ) ) ;
#51370=CARTESIAN_POINT ( 'NONE',  ( -1.846868145590737420, -144.0000000013655779, 4.458734124999997661 ) ) ;
#51372=CARTESIAN_POINT ( 'NONE',  ( -5.000000000000000000, 6.041666669397852019, -2.886751345948128211 ) ) ;
#51374=CARTESIAN_POINT ( 'NONE',  ( -4.458734124999997661, -44.22916666530106511, 2.574251347313722516 ) ) ;
#51377=CARTESIAN_POINT ( 'NONE',  ( 2.071067811865306751, -153.9375000027312410, -5.000000000000171418 ) ) ;
#51382=CARTESIAN_POINT ( 'NONE',  ( -4.458734124999998549, -77.47916666530106511, 2.574251347313722516 ) ) ;
#51386=VERTEX_POINT ( 'NONE', #42859 ) ;
#51388=CARTESIAN_POINT ( 'NONE',  ( 2.499999999999998668, -47.33333333333333570, -4.330127018922193649 ) ) ;
#51390=CARTESIAN_POINT ( 'NONE',  ( 5.000000000000000888, -168.0625000027312126, -2.071067811865475505 ) ) ;
#51392=CARTESIAN_POINT ( 'NONE',  ( 2.229367062500001939, 9.770833334698927786, 3.861377020970579999 ) ) ;
#51398=CARTESIAN_POINT ( 'NONE',  ( -4.999999999999998224, -15.79166666393548191, 2.886751345948131764 ) ) ;
#51399=CARTESIAN_POINT ( 'NONE',  ( 2.229367062500001939, -83.97916666530106511, 3.861377020970579999 ) ) ;
#51400=CARTESIAN_POINT ( 'NONE',  ( 4.458734125000000326, -10.89583333196773651, 2.574251347313718519 ) ) ;
#51402=CARTESIAN_POINT ( 'NONE',  ( 4.458734124999998549, -32.97916666530106511, -2.574251347313721627 ) ) ;
#51406=CARTESIAN_POINT ( 'NONE',  ( 1.846868145590735200, -148.5000000013656347, -4.458734124999999437 ) ) ;
#51407=CARTESIAN_POINT ( 'NONE',  ( -4.458734124999999437, 19.60416666803225993, -2.574251347313719407 ) ) ;
#51409=DIRECTION ( 'NONE',  ( -0.000000000000000000, 1.000000000000000000, -0.000000000000000000 ) ) ;
#51410=CARTESIAN_POINT ( 'NONE',  ( 4.458734125000000326, -82.14583333196772230, 2.574251347313718519 ) ) ;
#51413=CARTESIAN_POINT ( 'NONE',  ( -2.500000000000000444, 16.95833333606451987, -4.330127018922193649 ) ) ;
#51414=ORIENTED_EDGE ( 'NONE', *, *, #41313, .F. ) ;
#51415=CARTESIAN_POINT ( 'NONE',  ( 2.499999999999998668, -25.33333333333333215, -4.330127018922193649 ) ) ;
#51418=CARTESIAN_POINT ( 'NONE',  ( 5.000000000000000000, -22.41666666666666785, -2.886751345948129988 ) ) ;
#51419=CARTESIAN_POINT ( 'NONE',  ( 2.229367062499998831, -26.64583333196774007, -3.861377020970580887 ) ) ;
#51420=EDGE_CURVE ( 'NONE', #18873, #43870, #63441, .T. ) ;
#51421=CARTESIAN_POINT ( 'NONE',  ( 2.229367062499998831, -86.64583333196773651, -3.861377020970580887 ) ) ;
#51422=CARTESIAN_POINT ( 'NONE',  ( -2.500000000000000444, -31.04166666393548368, -4.330127018922193649 ) ) ;
#51423=CARTESIAN_POINT ( 'NONE',  ( 2.229367062499998831, -55.64583333196773651, -3.861377020970580887 ) ) ;
#51424=ORIENTED_EDGE ( 'NONE', *, *, #1109, .T. ) ;
#51426=CARTESIAN_POINT ( 'NONE',  ( 4.458734124999999437, -9.062499998634406140, -5.460374474430324690E-16 ) ) ;
#51427=ORIENTED_EDGE ( 'NONE', *, *, #42910, .F. ) ;
#51428=CARTESIAN_POINT ( 'NONE',  ( -2.499999999999996447, -70.83333333333332860, 4.330127018922195425 ) ) ;
#51433=CARTESIAN_POINT ( 'NONE',  ( -4.999999999999999112, -77.79166666393547303, 2.886751345948131764 ) ) ;
#51434=CARTESIAN_POINT ( 'NONE',  ( -1.339745962155613812, -54.08034179853029144, -5.000000000000000000 ) ) ;
#51435=AXIS2_PLACEMENT_3D ( 'NONE', #49639, #16183, #1415 ) ;
#51437=CARTESIAN_POINT ( 'NONE',  ( -2.229367062500000163, -14.72916666530107221, -3.861377020970580443 ) ) ;
#51438=CARTESIAN_POINT ( 'NONE',  ( -4.458734124999998549, -50.47916666530107221, 2.574251347313722516 ) ) ;
#51440=CARTESIAN_POINT ( 'NONE',  ( 5.000000000000000888, 10.41666666666666785, 2.886751345948126879 ) ) ;
#51441=SURFACE_STYLE_FILL_AREA ( #8010 ) ;
#51442=CARTESIAN_POINT ( 'NONE',  ( 4.458734125000000326, -141.3750000013656063, -1.846868145590734978 ) ) ;
#51445=CARTESIAN_POINT ( 'NONE',  ( 3.061616997868383141E-16, -147.8750000027312126, -5.000000000000000000 ) ) ;
#51446=ORIENTED_EDGE ( 'NONE', *, *, #59690, .T. ) ;
#51449=CARTESIAN_POINT ( 'NONE',  ( -2.499999999999996447, -12.70833333060214798, 4.330127018922195425 ) ) ;
#51452=( BOUNDED_CURVE ( )  B_SPLINE_CURVE ( 2, ( #2785, #51035, #61960, #42004, #8241, #61645, #17578, #21452, #27843 ),
 .UNSPECIFIED., .F., .F. ) 
 B_SPLINE_CURVE_WITH_KNOTS ( ( 3, 2, 2, 2, 3 ),
 ( 0.07291666666666667129, 0.07361111111111111327, 0.07499999999999999722, 0.07638888888888889506, 0.07708333333333333703 ),
 .UNSPECIFIED. ) 
 CURVE ( )  GEOMETRIC_REPRESENTATION_ITEM ( )  RATIONAL_B_SPLINE_CURVE ( ( 0.9330127018922194093, 0.9330127018922200755, 1.000000000000000000, 0.8660254037844387076, 1.000000000000000000, 0.8660254037844387076, 1.000000000000000000, 0.9330127018922194093, 0.9330127018922194093 ) ) 
 REPRESENTATION_ITEM ( '' )  );
#51454=CARTESIAN_POINT ( 'NONE',  ( 3.152801135295366208, -146.8125000013655779, 3.152801135295367985 ) ) ;
#51456=CARTESIAN_POINT ( 'NONE',  ( 0.000000000000000000, -170.0000000000000000, 0.000000000000000000 ) ) ;
#51458=CARTESIAN_POINT ( 'NONE',  ( -4.458734124999999437, -62.56249999863440792, 0.000000000000000000 ) ) ;
#51460=CARTESIAN_POINT ( 'NONE',  ( -3.152801135295367096, -145.0625000013655779, -3.152801135295367541 ) ) ;
#51462=ORIENTED_EDGE ( 'NONE', *, *, #47318, .T. ) ;
#51464=CARTESIAN_POINT ( 'NONE',  ( 3.061616997868383141E-16, -144.7500000000000284, -5.000000000000000000 ) ) ;
#51467=CARTESIAN_POINT ( 'NONE',  ( 4.458734124999998549, 29.02083333469893134, -2.574251347313721627 ) ) ;
#51468=CARTESIAN_POINT ( 'NONE',  ( 1.975475456537005874E-15, -76.62499999726880162, 5.000000000000000000 ) ) ;
#51474=CARTESIAN_POINT ( 'NONE',  ( -6.972266317189433020E-16, -56.12499999726880162, -5.000000000000000000 ) ) ;
#51476=CARTESIAN_POINT ( 'NONE',  ( -4.458734124999999437, 6.604166668032259935, -2.574251347313719407 ) ) ;
#51478=CARTESIAN_POINT ( 'NONE',  ( 2.229367062500001939, -22.22916666530107221, 3.861377020970579999 ) ) ;
#51480=CARTESIAN_POINT ( 'NONE',  ( -1.846868145590737420, -160.7500000013655779, 4.458734124999999437 ) ) ;
#51481=CARTESIAN_POINT ( 'NONE',  ( -6.972266317189433020E-16, 15.87500000273118417, -5.000000000000000000 ) ) ;
#51482=VECTOR ( 'NONE', #35033, 1000.000000000000000 ) ;
#51486=CARTESIAN_POINT ( 'NONE',  ( 4.458734124999998549, -37.72916666530107221, -2.574251347313721627 ) ) ;
#51487=CARTESIAN_POINT ( 'NONE',  ( 5.000000000000000000, 19.70833333606451632, -2.886751345948130876 ) ) ;
#51488=CARTESIAN_POINT ( 'NONE',  ( 4.458734124999999437, -68.06249999863440792, -5.460374474430324690E-16 ) ) ;
#51491=CARTESIAN_POINT ( 'NONE',  ( 1.339745962155612702, -89.29465819873851729, -5.000000000000000000 ) ) ;
#51495=CARTESIAN_POINT ( 'NONE',  ( 0.000000000000000000, -170.0000000000000000, 0.000000000000000000 ) ) ;
#51496=CARTESIAN_POINT ( 'NONE',  ( -5.000000000000000000, -5.083333333333334814, -2.886751345948128211 ) ) ;
#51497=EDGE_CURVE ( 'NONE', #44325, #14472, #48624, .T. ) ;
#51498=CARTESIAN_POINT ( 'NONE',  ( 9.457646018065525792E-16, -71.06249999863439371, 5.148502694627439702 ) ) ;
#51500=CARTESIAN_POINT ( 'NONE',  ( -5.000000000000000000, -10.95833333060214621, -2.886751345948128211 ) ) ;
#51501=CARTESIAN_POINT ( 'NONE',  ( -4.458734124999998549, -41.22916666530107221, 2.574251347313722516 ) ) ;
#51503=CARTESIAN_POINT ( 'NONE',  ( 3.535533905932736864, -144.1250000000000000, 3.535533905932738641 ) ) ;
#51504=CARTESIAN_POINT ( 'NONE',  ( -2.229367062500000163, 10.27083333469892779, -3.861377020970580443 ) ) ;
#51505=EDGE_LOOP ( 'NONE', ( #48639, #1463, #19023, #35927 ) ) ;
#51506=( BOUNDED_CURVE ( )  B_SPLINE_CURVE ( 2, ( #53244, #9180, #28792, #11632, #175, #16470, #4981, #26435, #1695 ),
 .UNSPECIFIED., .F., .F. ) 
 B_SPLINE_CURVE_WITH_KNOTS ( ( 3, 2, 2, 2, 3 ),
 ( 0.4083333333333336590, 0.4125000000000003109, 0.4166666666666670182, 0.4208333333333336701, 0.4250000000000003220 ),
 .UNSPECIFIED. ) 
 CURVE ( )  GEOMETRIC_REPRESENTATION_ITEM ( )  RATIONAL_B_SPLINE_CURVE ( ( 0.9999999999999938938, 0.9238795325112928447, 1.000000000000000000, 0.9238795325112867385, 1.000000000000000000, 0.9238795325112867385, 1.000000000000000000, 0.9238795325112806323, 1.000000000000005995 ) ) 
 REPRESENTATION_ITEM ( '' )  );
#51507=CARTESIAN_POINT ( 'NONE',  ( 5.000000000000000000, -81.29166666393547303, -2.886751345948130876 ) ) ;
#51508=CARTESIAN_POINT ( 'NONE',  ( -2.499999999999996447, -54.83333333333332860, 4.330127018922195425 ) ) ;
#51509=CARTESIAN_POINT ( 'NONE',  ( -8.190561711645485556E-16, -161.9375000013655779, 4.458734124999999437 ) ) ;
#51512=CARTESIAN_POINT ( 'NONE',  ( 9.457646018065525792E-16, -79.06249999863440792, 5.148502694627439702 ) ) ;
#51513=CARTESIAN_POINT ( 'NONE',  ( 3.152801135295366208, -140.8125000013655779, 3.152801135295367985 ) ) ;
#51514=CARTESIAN_POINT ( 'NONE',  ( -4.458734124999999437, -87.39583333196773651, -2.574251347313719407 ) ) ;
#51516=CARTESIAN_POINT ( 'NONE',  ( -2.229367062499996610, 1.604166668032262155, 3.861377020970582219 ) ) ;
#51517=CARTESIAN_POINT ( 'NONE',  ( -3.152548672688508926E-16, -36.81249999863440792, -5.148502694627439702 ) ) ;
#51518=CARTESIAN_POINT ( 'NONE',  ( 1.339745962155612702, -72.29465819873850307, -5.000000000000000000 ) ) ;
#51519=EDGE_CURVE ( 'NONE', #21623, #27699, #24288, .T. ) ;
#51522=ADVANCED_FACE ( 'NONE', ( #30276 ), #44750, .T. ) ;
#51523=CARTESIAN_POINT ( 'NONE',  ( 3.061616997868383141E-16, -141.7500000000000284, -5.000000000000000000 ) ) ;
#51524=DIRECTION ( 'NONE',  ( -0.000000000000000000, 1.000000000000000000, -0.000000000000000000 ) ) ;
#51525=CARTESIAN_POINT ( 'NONE',  ( 2.229367062499998831, -68.89583333196773651, -3.861377020970580887 ) ) ;
#51527=ORIENTED_EDGE ( 'NONE', *, *, #53864, .T. ) ;
#51528=CARTESIAN_POINT ( 'NONE',  ( 5.000000000000000888, -5.583333333333336590, 2.886751345948126879 ) ) ;
#51531=CARTESIAN_POINT ( 'NONE',  ( 2.229367062500001939, 7.020833334698928674, 3.861377020970579999 ) ) ;
#51533=CARTESIAN_POINT ( 'NONE',  ( 4.458734124999997661, -155.5000000013656063, 1.846868145590737864 ) ) ;
#51537=CARTESIAN_POINT ( 'NONE',  ( -5.000000000000000000, -25.08333333333333215, -2.886751345948128211 ) ) ;
#51539=EDGE_CURVE ( 'NONE', #25291, #17887, #21870, .T. ) ;
#51541=DIRECTION ( 'NONE',  ( -0.000000000000000000, 1.000000000000000000, -0.000000000000000000 ) ) ;
#51544=CARTESIAN_POINT ( 'NONE',  ( 9.457646018065525792E-16, 23.93750000136559564, 5.148502694627439702 ) ) ;
#51547=CARTESIAN_POINT ( 'NONE',  ( 2.229367062499998831, -2.895833331967738289, -3.861377020970580887 ) ) ;
#51549=CARTESIAN_POINT ( 'NONE',  ( -2.071067811865306307, -149.8125000027311842, -5.000000000000171418 ) ) ;
#51551=CARTESIAN_POINT ( 'NONE',  ( -2.071067811865475061, -142.8125000027312126, -5.000000000000000888 ) ) ;
#51552=CARTESIAN_POINT ( 'NONE',  ( 5.000000000000000888, -158.9375000000000000, -2.071067811865475505 ) ) ;
#51557=CARTESIAN_POINT ( 'NONE',  ( 1.339745962155615144, -22.70534180126147916, 4.999999999999999112 ) ) ;
#51559=CARTESIAN_POINT ( 'NONE',  ( 4.458734124999999437, -159.6875000013655779, 0.000000000000000000 ) ) ;
#51561=CARTESIAN_POINT ( 'NONE',  ( -2.071067811865562991, -147.3125000000000000, 4.999999999999913847 ) ) ;
#51563=CARTESIAN_POINT ( 'NONE',  ( 4.458734124999999437, 17.93750000136559208, -5.460374474430324690E-16 ) ) ;
#51564=ORIENTED_EDGE ( 'NONE', *, *, #40815, .F. ) ;
#51568=CARTESIAN_POINT ( 'NONE',  ( -6.972266317189433020E-16, -37.25000000000000000, -5.000000000000000000 ) ) ;
#51569=CARTESIAN_POINT ( 'NONE',  ( 2.499999999999998668, 9.666666666666667851, -4.330127018922193649 ) ) ;
#51570=CARTESIAN_POINT ( 'NONE',  ( -4.458734124999999437, -57.31249999863440081, 0.000000000000000000 ) ) ;
#51573=ADVANCED_FACE ( 'NONE', ( #19675 ), #29637, .T. ) ;
#51574=DIRECTION ( 'NONE',  ( -0.000000000000000000, 1.000000000000000000, -0.000000000000000000 ) ) ;
#51575=CARTESIAN_POINT ( 'NONE',  ( -5.000000000000000000, -37.87499999726881583, 0.000000000000000000 ) ) ;
#51578=CARTESIAN_POINT ( 'NONE',  ( -5.000000000000000000, -24.87499999726881583, 0.000000000000000000 ) ) ;
#51579=CARTESIAN_POINT ( 'NONE',  ( 5.000000000000000000, -40.41666666666667140, -2.886751345948129988 ) ) ;
#51583=EDGE_CURVE ( 'NONE', #49037, #42676, #28429, .T. ) ;
#51584=CARTESIAN_POINT ( 'NONE',  ( -2.229367062499996610, -66.14583333196773651, 3.861377020970582219 ) ) ;
#51585=CARTESIAN_POINT ( 'NONE',  ( -4.458734124999999437, -153.1875000013656063, -5.460374474430324690E-16 ) ) ;
#51586=CARTESIAN_POINT ( 'NONE',  ( -4.458734124999999437, -69.39583333196773651, -2.574251347313719407 ) ) ;
#51588=ADVANCED_FACE ( 'NONE', ( #31702 ), #61939, .T. ) ;
#51590=CARTESIAN_POINT ( 'NONE',  ( 4.458734124999998549, -19.97916666530106866, -2.574251347313721627 ) ) ;
#51591=CARTESIAN_POINT ( 'NONE',  ( -5.000000000000000000, -61.87499999726880873, 0.000000000000000000 ) ) ;
#51592=VERTEX_POINT ( 'NONE', #2142 ) ;
#51593=CARTESIAN_POINT ( 'NONE',  ( -5.000000000000000000, -49.00000000000000000, 0.000000000000000000 ) ) ;
#51597=CYLINDRICAL_SURFACE ( 'NONE', #4000, 5.000000000000000000 ) ;
#51598=CARTESIAN_POINT ( 'NONE',  ( -3.152801135295367985, -150.8125000013655779, 3.152801135295367096 ) ) ;
#51601=EDGE_CURVE ( 'NONE', #5304, #34281, #36852, .T. ) ;
#51606=CARTESIAN_POINT ( 'NONE',  ( -2.229367062500000163, -46.72916666530106511, -3.861377020970580443 ) ) ;
#51607=ORIENTED_EDGE ( 'NONE', *, *, #18972, .F. ) ;
#51610=CARTESIAN_POINT ( 'NONE',  ( -2.229367062500000163, 21.52083333469892779, -3.861377020970580443 ) ) ;
#51613=CARTESIAN_POINT ( 'NONE',  ( 4.458734124999999437, -168.3750000013655779, -1.846868145590734978 ) ) ;
#51614=ORIENTED_EDGE ( 'NONE', *, *, #380, .F. ) ;
#51616=CARTESIAN_POINT ( 'NONE',  ( -2.500000000000000444, -86.04166666393547303, -4.330127018922193649 ) ) ;
#51618=CARTESIAN_POINT ( 'NONE',  ( 2.500000000000002220, -69.54166666393547303, 4.330127018922192761 ) ) ;
#51627=CARTESIAN_POINT ( 'NONE',  ( -9.184850993605147944E-16, -159.2500000000000000, 5.000000000000000000 ) ) ;
#51629=CARTESIAN_POINT ( 'NONE',  ( -3.535533905932738641, -154.5000000027312126, 3.535533905932737309 ) ) ;
#51630=ORIENTED_EDGE ( 'NONE', *, *, #59743, .T. ) ;
#51634=( BOUNDED_CURVE ( )  B_SPLINE_CURVE ( 2, ( #25097, #11257, #59525, #50510, #40213, #15459, #36030, #55009, #45676 ),
 .UNSPECIFIED., .F., .F. ) 
 B_SPLINE_CURVE_WITH_KNOTS ( ( 3, 2, 2, 2, 3 ),
 ( 0.4520833333333333370, 0.4527777777777777790, 0.4541666666666666630, 0.4555555555555555469, 0.4562499999999999889 ),
 .UNSPECIFIED. ) 
 CURVE ( )  GEOMETRIC_REPRESENTATION_ITEM ( )  RATIONAL_B_SPLINE_CURVE ( ( 0.9330127018922194093, 0.9330127018922194093, 1.000000000000000000, 0.8660254037844387076, 1.000000000000000000, 0.8660254037844387076, 1.000000000000000000, 0.9330127018922194093, 0.9330127018922194093 ) ) 
 REPRESENTATION_ITEM ( '' )  );
#51636=CARTESIAN_POINT ( 'NONE',  ( -5.000000000000000000, -147.5000000000000284, -6.123233995736766282E-16 ) ) ;
#51640=CARTESIAN_POINT ( 'NONE',  ( -2.229367062499996610, -23.14583333196773651, 3.861377020970582219 ) ) ;
#51641=CARTESIAN_POINT ( 'NONE',  ( 3.535533905932736864, -147.1250000000000000, 3.535533905932738641 ) ) ;
#51644=CARTESIAN_POINT ( 'NONE',  ( 4.458734125000000326, -151.3750000013656063, -1.846868145590734978 ) ) ;
#51645=VERTEX_POINT ( 'NONE', #2759 ) ;
#51646=DIRECTION ( 'NONE',  ( -0.000000000000000000, 1.000000000000000000, -0.000000000000000000 ) ) ;
#51647=CARTESIAN_POINT ( 'NONE',  ( -2.229367062500000163, -50.72916666530107221, -3.861377020970580443 ) ) ;
#51648=CARTESIAN_POINT ( 'NONE',  ( 5.000000000000000000, -58.29166666393548013, -2.886751345948130876 ) ) ;
#51650=CARTESIAN_POINT ( 'NONE',  ( -4.999999999999999112, 22.08333333333333215, 2.886751345948131764 ) ) ;
#51651=FACE_OUTER_BOUND ( 'NONE', #5085, .T. ) ;
#51652=CARTESIAN_POINT ( 'NONE',  ( -4.458734124999999437, 1.604166668032262155, -2.574251347313719407 ) ) ;
#51653=( BOUNDED_CURVE ( )  B_SPLINE_CURVE ( 2, ( #13161, #46313, #32784, #46629, #52093, #2270, #41469, #8032, #52415 ),
 .UNSPECIFIED., .F., .F. ) 
 B_SPLINE_CURVE_WITH_KNOTS ( ( 3, 2, 2, 2, 3 ),
 ( 0.1104166666666666630, 0.1111111111111111049, 0.1125000000000000028, 0.1138888888888888867, 0.1145833333333333426 ),
 .UNSPECIFIED. ) 
 CURVE ( )  GEOMETRIC_REPRESENTATION_ITEM ( )  RATIONAL_B_SPLINE_CURVE ( ( 0.9330127018922194093, 0.9330127018922194093, 1.000000000000000000, 0.8660254037844387076, 1.000000000000000000, 0.8660254037844387076, 1.000000000000000000, 0.9330127018922187432, 0.9330127018922194093 ) ) 
 REPRESENTATION_ITEM ( '' )  );
#51654=CARTESIAN_POINT ( 'NONE',  ( -3.535533905932737309, -160.7500000027312126, -3.535533905932738197 ) ) ;
#51656=CARTESIAN_POINT ( 'NONE',  ( 2.500000000000002220, -7.666666666666668739, 4.330127018922192761 ) ) ;
#51657=CARTESIAN_POINT ( 'NONE',  ( -4.458734124999999437, 17.35416666803225993, -2.574251347313719407 ) ) ;
#51658=CARTESIAN_POINT ( 'NONE',  ( 5.000000000000000000, 3.625000002731186388, -6.123233995736766282E-16 ) ) ;
#51659=ORIENTED_EDGE ( 'NONE', *, *, #59964, .F. ) ;
#51662=CARTESIAN_POINT ( 'NONE',  ( 2.229367062499998831, -49.64583333196772941, -3.861377020970580887 ) ) ;
#51663=CARTESIAN_POINT ( 'NONE',  ( -4.458734125000000326, -163.2500000013655495, -1.846868145590735644 ) ) ;
#51664=CARTESIAN_POINT ( 'NONE',  ( 5.000000000000000000, -47.37499999726880873, -6.123233995736766282E-16 ) ) ;
#51666=CARTESIAN_POINT ( 'NONE',  ( -4.458734124999998549, -24.22916666530107577, 2.574251347313722516 ) ) ;
#51667=ORIENTED_EDGE ( 'NONE', *, *, #44891, .T. ) ;
#51668=CARTESIAN_POINT ( 'NONE',  ( -2.500000000000000444, -85.16666666666667140, -4.330127018922193649 ) ) ;
#51669=CARTESIAN_POINT ( 'NONE',  ( 3.152801135295367541, -164.3125000013656063, -3.152801135295367541 ) ) ;
#51670=ADVANCED_FACE ( 'NONE', ( #51651 ), #32335, .T. ) ;
#51673=CARTESIAN_POINT ( 'NONE',  ( -2.229367062499996610, -34.39583333196772941, 3.861377020970582219 ) ) ;
#51676=EDGE_CURVE ( 'NONE', #23803, #50991, #61302, .T. ) ;
#51682=CARTESIAN_POINT ( 'NONE',  ( -2.229367062500000163, -78.72916666530106511, -3.861377020970580443 ) ) ;
#51684=CARTESIAN_POINT ( 'NONE',  ( 3.061616997868383141E-16, -142.7500000000000284, -5.000000000000000000 ) ) ;
#51685=CARTESIAN_POINT ( 'NONE',  ( 5.000000000000000888, -9.583333333333332149, 2.886751345948126879 ) ) ;
#51686=CARTESIAN_POINT ( 'NONE',  ( 2.499999999999998668, 20.66666666666666785, -4.330127018922193649 ) ) ;
#51688=CARTESIAN_POINT ( 'NONE',  ( 2.229367062500001939, -47.97916666530106511, 3.861377020970579999 ) ) ;
#51691=CARTESIAN_POINT ( 'NONE',  ( -9.184850993605147944E-16, -159.3750000027311842, 5.000000000000000000 ) ) ;
#51696=CARTESIAN_POINT ( 'NONE',  ( -4.458734124999999437, -79.64583333196772230, -2.574251347313719407 ) ) ;
#51702=DIRECTION ( 'NONE',  ( -0.000000000000000000, 1.000000000000000000, -0.000000000000000000 ) ) ;
#51704=CARTESIAN_POINT ( 'NONE',  ( -5.000000000000000000, -4.999999999999997335, 0.000000000000000000 ) ) ;
#51706=CARTESIAN_POINT ( 'NONE',  ( 9.457646018065525792E-16, 11.68750000136559564, 5.148502694627439702 ) ) ;
#51707=DIRECTION ( 'NONE',  ( -0.000000000000000000, 1.000000000000000000, -0.000000000000000000 ) ) ;
#51712=CARTESIAN_POINT ( 'NONE',  ( -3.535533905932737309, -163.6250000000000284, -3.535533905932738197 ) ) ;
#51713=CARTESIAN_POINT ( 'NONE',  ( -3.535533905932737309, -152.6250000000000000, -3.535533905932738197 ) ) ;
#51714=CARTESIAN_POINT ( 'NONE',  ( -3.152548672688508926E-16, -6.562499998634404363, -5.148502694627439702 ) ) ;
#51717=CARTESIAN_POINT ( 'NONE',  ( 4.458734124999999437, -33.06249999863440792, -5.460374474430324690E-16 ) ) ;
#51722=CARTESIAN_POINT ( 'NONE',  ( -1.846868145590737420, -151.0000000013656063, 4.458734124999997661 ) ) ;
#51724=CARTESIAN_POINT ( 'NONE',  ( -2.229367062500000163, 12.52083333469892601, -3.861377020970580443 ) ) ;
#51726=DIRECTION ( 'NONE',  ( 0.000000000000000000, 0.000000000000000000, 1.000000000000000000 ) ) ;
#51727=CARTESIAN_POINT ( 'NONE',  ( -3.152548672688508926E-16, -81.81249999863440792, -5.148502694627439702 ) ) ;
#51730=CARTESIAN_POINT ( 'NONE',  ( 5.000000000000000000, 17.70833333606451632, -2.886751345948129988 ) ) ;
#51731=ORIENTED_EDGE ( 'NONE', *, *, #32159, .T. ) ;
#51733=( BOUNDED_CURVE ( )  B_SPLINE_CURVE ( 2, ( #48934, #58289, #18725, #54083, #33215, #52833, #58604, #23571, #19034 ),
 .UNSPECIFIED., .F., .F. ) 
 B_SPLINE_CURVE_WITH_KNOTS ( ( 3, 2, 2, 2, 3 ),
 ( 0.5979166666666666519, 0.5986111111111110938, 0.5999999999999999778, 0.6013888888888888618, 0.6020833333333333037 ),
 .UNSPECIFIED. ) 
 CURVE ( )  GEOMETRIC_REPRESENTATION_ITEM ( )  RATIONAL_B_SPLINE_CURVE ( ( 0.9330127018922194093, 0.9330127018922194093, 1.000000000000000000, 0.8660254037844387076, 1.000000000000000000, 0.8660254037844387076, 1.000000000000000000, 0.9330127018922194093, 0.9330127018922194093 ) ) 
 REPRESENTATION_ITEM ( '' )  );
#51736=CARTESIAN_POINT ( 'NONE',  ( -4.999999999999999112, -22.91666666666666785, 2.886751345948131764 ) ) ;
#51737=CARTESIAN_POINT ( 'NONE',  ( 2.229367062500001939, -28.97916666530107221, 3.861377020970579999 ) ) ;
#51738=CARTESIAN_POINT ( 'NONE',  ( 5.000000000000000888, -27.45833333060214798, 2.886751345948126879 ) ) ;
#51739=CARTESIAN_POINT ( 'NONE',  ( 4.458734124999999437, -58.81249999863440081, -5.460374474430324690E-16 ) ) ;
#51741=LINE ( 'NONE', #37259, #14864 ) ;
#51742=CARTESIAN_POINT ( 'NONE',  ( -4.458734124999999437, -8.645833331967736513, -2.574251347313719407 ) ) ;
#51744=CARTESIAN_POINT ( 'NONE',  ( -3.535250795749689387E-16, -72.24999999999998579, -5.773502691896257311 ) ) ;
#51747=CARTESIAN_POINT ( 'NONE',  ( 5.000000000000000000, -77.29166666393545881, -2.886751345948129988 ) ) ;
#51751=CARTESIAN_POINT ( 'NONE',  ( 2.229367062500001939, -18.22916666530106866, 3.861377020970579999 ) ) ;
#51752=CARTESIAN_POINT ( 'NONE',  ( 4.458734124999999437, -56.06249999863440081, -5.460374474430324690E-16 ) ) ;
#51755=CARTESIAN_POINT ( 'NONE',  ( 1.846868145590735200, -169.5000000013655495, -4.458734125000000326 ) ) ;
#51761=CARTESIAN_POINT ( 'NONE',  ( 0.000000000000000000, -170.0000000000000000, 0.000000000000000000 ) ) ;
#51764=CARTESIAN_POINT ( 'NONE',  ( 4.458734124999999437, -147.7500000013655779, 1.846868145590737864 ) ) ;
#51766=FACE_OUTER_BOUND ( 'NONE', #45821, .T. ) ;
#51768=CARTESIAN_POINT ( 'NONE',  ( 2.229367062500001939, -62.22916666530106511, 3.861377020970579999 ) ) ;
#51770=FACE_OUTER_BOUND ( 'NONE', #11501, .T. ) ;
#51771=CARTESIAN_POINT ( 'NONE',  ( 3.152801135295366208, -145.5625000013655779, 3.152801135295367985 ) ) ;
#51777=DIRECTION ( 'NONE',  ( -0.000000000000000000, 1.000000000000000000, -0.000000000000000000 ) ) ;
#51780=CARTESIAN_POINT ( 'NONE',  ( -3.152548672688508926E-16, 29.18750000136559208, -5.148502694627439702 ) ) ;
#51781=DIRECTION ( 'NONE',  ( 0.000000000000000000, 0.000000000000000000, 1.000000000000000000 ) ) ;
#51785=LINE ( 'NONE', #36995, #42741 ) ;
#51786=CARTESIAN_POINT ( 'NONE',  ( -5.000000000000000000, -15.08333333333333215, -2.886751345948128211 ) ) ;
#51787=CARTESIAN_POINT ( 'NONE',  ( 4.458734125000000326, 6.104166668032262599, 2.574251347313718519 ) ) ;
#51789=CARTESIAN_POINT ( 'NONE',  ( -3.152548672688508926E-16, -18.81249999863440792, -5.148502694627439702 ) ) ;
#51791=CARTESIAN_POINT ( 'NONE',  ( -4.458734125000000326, -159.0000000013656063, -1.846868145590735644 ) ) ;
#51792=CARTESIAN_POINT ( 'NONE',  ( 2.500000000000002220, 23.33333333333333215, 4.330127018922192761 ) ) ;
#51796=CARTESIAN_POINT ( 'NONE',  ( -3.152548672688508926E-16, -38.56249999863440081, -5.148502694627439702 ) ) ;
#51798=CARTESIAN_POINT ( 'NONE',  ( 9.457646018065525792E-16, -69.31249999863439371, 5.148502694627439702 ) ) ;
#51800=CARTESIAN_POINT ( 'NONE',  ( 5.000000000000000000, -152.1875000027312126, 2.071067811865478614 ) ) ;
#51804=CARTESIAN_POINT ( 'NONE',  ( -3.535250795749689387E-16, -9.250000000000001776, -5.773502691896257311 ) ) ;
#51805=CARTESIAN_POINT ( 'NONE',  ( 4.458734124999998549, -69.72916666530107932, -2.574251347313721627 ) ) ;
#51807=CARTESIAN_POINT ( 'NONE',  ( -3.535250795749689387E-16, -13.12499999726881050, -5.773502691896257311 ) ) ;
#51808=CARTESIAN_POINT ( 'NONE',  ( 4.458734124999999437, -41.81249999863440081, -5.460374474430324690E-16 ) ) ;
#51809=EDGE_LOOP ( 'NONE', ( #7691, #23590, #6035, #37988 ) ) ;
#51811=CARTESIAN_POINT ( 'NONE',  ( -4.458734124999999437, 5.354166668032262599, -2.574251347313719407 ) ) ;
#51813=CARTESIAN_POINT ( 'NONE',  ( 2.499999999999998668, -34.20833333060213732, -4.330127018922193649 ) ) ;
#51814=CARTESIAN_POINT ( 'NONE',  ( 2.500000000000002220, -56.66666666666667140, 4.330127018922192761 ) ) ;
#51815=CARTESIAN_POINT ( 'NONE',  ( 4.458734124999999437, -159.6875000013655779, 0.000000000000000000 ) ) ;
#51818=CARTESIAN_POINT ( 'NONE',  ( 9.457646018065525792E-16, -80.06249999863439371, 5.148502694627439702 ) ) ;
#51819=CARTESIAN_POINT ( 'NONE',  ( 5.000000000000000888, -167.9375000000000000, -2.071067811865475505 ) ) ;
#51820=CARTESIAN_POINT ( 'NONE',  ( -4.458734124999999437, -88.31249999863439371, 0.000000000000000000 ) ) ;
#51822=CARTESIAN_POINT ( 'NONE',  ( -4.458734124999999437, 0.4375000013655955255, 0.000000000000000000 ) ) ;
#51823=CARTESIAN_POINT ( 'NONE',  ( 9.457646018065525792E-16, -37.31249999863440792, 5.148502694627439702 ) ) ;
#51824=( BOUNDED_CURVE ( )  B_SPLINE_CURVE ( 2, ( #45565, #54263, #60380, #10509, #891, #11152, #49753, #30123, #35926 ),
 .UNSPECIFIED., .F., .F. ) 
 B_SPLINE_CURVE_WITH_KNOTS ( ( 3, 2, 2, 2, 3 ),
 ( 0.2854166666666666519, 0.2861111111111110938, 0.2874999999999999778, 0.2888888888888888618, 0.2895833333333333592 ),
 .UNSPECIFIED. ) 
 CURVE ( )  GEOMETRIC_REPRESENTATION_ITEM ( )  RATIONAL_B_SPLINE_CURVE ( ( 0.9330127018922194093, 0.9330127018922194093, 1.000000000000000000, 0.8660254037844387076, 1.000000000000000000, 0.8660254037844387076, 1.000000000000000000, 0.9330127018922167448, 0.9330127018922194093 ) ) 
 REPRESENTATION_ITEM ( '' )  );
#51825=CARTESIAN_POINT ( 'NONE',  ( 5.000000000000000888, -16.45833333060214443, 2.886751345948126879 ) ) ;
#51827=CARTESIAN_POINT ( 'NONE',  ( -6.972266317189433020E-16, 15.87500000273118417, -5.000000000000000000 ) ) ;
#51829=CARTESIAN_POINT ( 'NONE',  ( -5.000000000000000000, -141.5000000000000284, -6.123233995736766282E-16 ) ) ;
#51831=CARTESIAN_POINT ( 'NONE',  ( 4.458734124999998549, -70.97916666530107932, -2.574251347313721627 ) ) ;
#51834=VERTEX_POINT ( 'NONE', #18174 ) ;
#51835=CARTESIAN_POINT ( 'NONE',  ( -9.184850993605147944E-16, -150.3750000027312126, 5.000000000000000000 ) ) ;
#51838=CARTESIAN_POINT ( 'NONE',  ( -5.000000000000000000, 2.999999999999999112, 0.000000000000000000 ) ) ;
#51839=CARTESIAN_POINT ( 'NONE',  ( 2.229367062500001939, 2.020833334698927786, 3.861377020970579999 ) ) ;
#51840=CARTESIAN_POINT ( 'NONE',  ( -2.500000000000000444, -33.04166666393547303, -4.330127018922193649 ) ) ;
#51841=CARTESIAN_POINT ( 'NONE',  ( 4.458734124999999437, -155.3750000013656063, -1.846868145590734978 ) ) ;
#51843=ORIENTED_EDGE ( 'NONE', *, *, #1594, .T. ) ;
#51848=DIRECTION ( 'NONE',  ( 0.000000000000000000, 0.000000000000000000, 1.000000000000000000 ) ) ;
#51850=VECTOR ( 'NONE', #6725, 1000.000000000000000 ) ;
#51856=CARTESIAN_POINT ( 'NONE',  ( 9.457646018065525792E-16, 24.93750000136559208, 5.148502694627439702 ) ) ;
#51858=CARTESIAN_POINT ( 'NONE',  ( -2.229367062500000163, -3.729166665301070438, -3.861377020970580443 ) ) ;
#51861=CARTESIAN_POINT ( 'NONE',  ( 5.000000000000000000, -143.1250000027312126, 0.000000000000000000 ) ) ;
#51862=CARTESIAN_POINT ( 'NONE',  ( -2.499999999999996447, -20.70833333060214798, 4.330127018922195425 ) ) ;
#51863=EDGE_CURVE ( 'NONE', #54901, #46689, #33315, .T. ) ;
#51867=DIRECTION ( 'NONE',  ( -0.000000000000000000, 1.000000000000000000, -0.000000000000000000 ) ) ;
#51871=CARTESIAN_POINT ( 'NONE',  ( 3.152801135295367541, -156.5625000013656063, -3.152801135295367541 ) ) ;
#51874=DIRECTION ( 'NONE',  ( 0.000000000000000000, 0.000000000000000000, 1.000000000000000000 ) ) ;
#51876=CARTESIAN_POINT ( 'NONE',  ( -3.152548672688508926E-16, 18.18750000136559564, -5.148502694627439702 ) ) ;
#51882=CARTESIAN_POINT ( 'NONE',  ( 5.000000000000000888, 7.416666666666665186, 2.886751345948126879 ) ) ;
#51883=CARTESIAN_POINT ( 'NONE',  ( 4.458734125000000326, -54.89583333196774362, 2.574251347313718519 ) ) ;
#51884=CARTESIAN_POINT ( 'NONE',  ( -6.972266317189433020E-16, -53.12499999726880162, -5.000000000000000000 ) ) ;
#51889=CARTESIAN_POINT ( 'NONE',  ( -5.000000000000000888, -151.6875000027312126, -2.071067811865475949 ) ) ;
#51890=CARTESIAN_POINT ( 'NONE',  ( -2.499999999999996447, -38.83333333333332860, 4.330127018922195425 ) ) ;
#51894=CARTESIAN_POINT ( 'NONE',  ( -5.000000000000000000, 12.91666666666666607, -2.886751345948128211 ) ) ;
#51895=CARTESIAN_POINT ( 'NONE',  ( -4.458734124999999437, -66.39583333196773651, -2.574251347313719407 ) ) ;
#51896=CARTESIAN_POINT ( 'NONE',  ( -4.458734125000001214, -148.1250000013655779, 1.846868145590734089 ) ) ;
#51897=CARTESIAN_POINT ( 'NONE',  ( -4.458734124999999437, -72.39583333196775072, -2.574251347313719407 ) ) ;
#51899=CARTESIAN_POINT ( 'NONE',  ( 4.458734125000001214, -20.14583333196774007, 2.574251347313718519 ) ) ;
#51900=CARTESIAN_POINT ( 'NONE',  ( -5.000000000000000000, -61.95833333060215153, -2.886751345948128211 ) ) ;
#51901=ORIENTED_EDGE ( 'NONE', *, *, #33394, .T. ) ;
#51905=( BOUNDED_CURVE ( )  B_SPLINE_CURVE ( 2, ( #40559, #26093, #21905, #45390, #60202, #36063, #31549, #56006, #55692 ),
 .UNSPECIFIED., .F., .F. ) 
 B_SPLINE_CURVE_WITH_KNOTS ( ( 3, 2, 2, 2, 3 ),
 ( 0.3895833333333333370, 0.3902777777777777790, 0.3916666666666666630, 0.3930555555555555469, 0.3937499999999999889 ),
 .UNSPECIFIED. ) 
 CURVE ( )  GEOMETRIC_REPRESENTATION_ITEM ( )  RATIONAL_B_SPLINE_CURVE ( ( 0.9330127018922194093, 0.9330127018922194093, 1.000000000000000000, 0.8660254037844387076, 1.000000000000000000, 0.8660254037844387076, 1.000000000000000000, 0.9330127018922194093, 0.9330127018922194093 ) ) 
 REPRESENTATION_ITEM ( '' )  );
#51909=CARTESIAN_POINT ( 'NONE',  ( 1.975475456537005874E-15, -53.62499999726880162, 5.000000000000000000 ) ) ;
#51911=CARTESIAN_POINT ( 'NONE',  ( 5.000000000000000000, -8.416666666666669627, -2.886751345948130876 ) ) ;
#51912=CARTESIAN_POINT ( 'NONE',  ( 2.229367062500001939, -56.22916666530107221, 3.861377020970579999 ) ) ;
#51913=ORIENTED_EDGE ( 'NONE', *, *, #27971, .F. ) ;
#51916=CARTESIAN_POINT ( 'NONE',  ( 4.458734124999999437, 17.18750000136559564, -5.460374474430324690E-16 ) ) ;
#51919=CARTESIAN_POINT ( 'NONE',  ( 5.000000000000000000, -165.0000000000000000, 0.000000000000000000 ) ) ;
#51920=( BOUNDED_CURVE ( )  B_SPLINE_CURVE ( 2, ( #47291, #3242, #22541, #51800, #41495, #37011, #27976, #37954, #61148 ),
 .UNSPECIFIED., .F., .F. ) 
 B_SPLINE_CURVE_WITH_KNOTS ( ( 3, 2, 2, 2, 3 ),
 ( 0.5583333333333337922, 0.5625000000000004441, 0.5666666666666670960, 0.5708333333333338588, 0.5750000000000005107 ),
 .UNSPECIFIED. ) 
 CURVE ( )  GEOMETRIC_REPRESENTATION_ITEM ( )  RATIONAL_B_SPLINE_CURVE ( ( 0.9999999999999918954, 0.9238795325112948431, 1.000000000000000000, 0.9238795325112867385, 1.000000000000000000, 0.9238795325112867385, 1.000000000000000000, 0.9238795325112766355, 1.000000000000010214 ) ) 
 REPRESENTATION_ITEM ( '' )  );
#51921=VERTEX_POINT ( 'NONE', #39041 ) ;
#51923=LINE ( 'NONE', #17822, #15065 ) ;
#51926=EDGE_CURVE ( 'NONE', #9545, #19516, #46475, .T. ) ;
#51936=CYLINDRICAL_SURFACE ( 'NONE', #1212, 5.000000000000000000 ) ;
#51938=CARTESIAN_POINT ( 'NONE',  ( 3.535533905932738197, -155.0000000027312126, -3.535533905932738197 ) ) ;
#51943=EDGE_CURVE ( 'NONE', #4579, #14700, #8527, .T. ) ;
#51946=CARTESIAN_POINT ( 'NONE',  ( 2.071067811865476394, -147.1875000000000284, 5.000000000000000000 ) ) ;
#51948=ADVANCED_FACE ( 'NONE', ( #3710 ), #4955, .T. ) ;
#51950=CARTESIAN_POINT ( 'NONE',  ( 1.339745962155618697, 22.83034180399266688, -4.999999999999998224 ) ) ;
#51951=CARTESIAN_POINT ( 'NONE',  ( 9.457646018065525792E-16, -25.06249999863440792, 5.148502694627439702 ) ) ;
#51952=CARTESIAN_POINT ( 'NONE',  ( 3.061616997868383141E-16, -157.8750000027311842, -5.000000000000000000 ) ) ;
#51953=CARTESIAN_POINT ( 'NONE',  ( -1.339745962155610925, 9.330341803992663330, 5.000000000000000000 ) ) ;
#51955=CARTESIAN_POINT ( 'NONE',  ( 1.846868145590735200, -149.2500000013655779, -4.458734125000000326 ) ) ;
#51956=ORIENTED_EDGE ( 'NONE', *, *, #53943, .T. ) ;
#51958=CARTESIAN_POINT ( 'NONE',  ( 4.458734125000000326, -53.14583333196773651, 2.574251347313718519 ) ) ;
#51961=CARTESIAN_POINT ( 'NONE',  ( -2.500000000000000444, 25.83333333333333215, -4.330127018922193649 ) ) ;
#51962=DIRECTION ( 'NONE',  ( -0.000000000000000000, 1.000000000000000000, -0.000000000000000000 ) ) ;
#51963=CARTESIAN_POINT ( 'NONE',  ( -2.229367062500000163, -2.479166665301069106, -3.861377020970580443 ) ) ;
#51964=CARTESIAN_POINT ( 'NONE',  ( 5.000000000000000000, -48.41666666666666430, -2.886751345948130876 ) ) ;
#51965=CARTESIAN_POINT ( 'NONE',  ( 5.000000000000000888, -140.9375000000000284, -2.071067811865475505 ) ) ;
#51966=CARTESIAN_POINT ( 'NONE',  ( 1.339745962155615144, -7.705341801261480938, 4.999999999999999112 ) ) ;
#51967=CARTESIAN_POINT ( 'NONE',  ( 2.229367062499998831, 8.104166668032261711, -3.861377020970580887 ) ) ;
#51968=ORIENTED_EDGE ( 'NONE', *, *, #29322, .T. ) ;
#51970=ORIENTED_EDGE ( 'NONE', *, *, #41156, .T. ) ;
#51972=CARTESIAN_POINT ( 'NONE',  ( 2.229367062500001939, -50.97916666530107221, 3.861377020970579999 ) ) ;
#51973=CARTESIAN_POINT ( 'NONE',  ( -1.846868145590734756, -159.3750000013656347, -4.458734125000000326 ) ) ;
#51974=CARTESIAN_POINT ( 'NONE',  ( -2.500000000000000444, -44.04166666393546592, -4.330127018922193649 ) ) ;
#51975=ORIENTED_EDGE ( 'NONE', *, *, #4992, .T. ) ;
#51976=CARTESIAN_POINT ( 'NONE',  ( 2.229367062500001939, -24.97916666530106866, 3.861377020970579999 ) ) ;
#51977=ORIENTED_EDGE ( 'NONE', *, *, #5820, .F. ) ;
#51978=CARTESIAN_POINT ( 'NONE',  ( -5.000000000000000000, -142.6250000027312126, -6.123233995736766282E-16 ) ) ;
#51979=CARTESIAN_POINT ( 'NONE',  ( -8.190561711645485556E-16, -163.6875000013655779, 4.458734124999999437 ) ) ;
#51982=CARTESIAN_POINT ( 'NONE',  ( -2.229367062500000163, -39.72916666530107221, -3.861377020970580443 ) ) ;
#51983=DIRECTION ( 'NONE',  ( -0.000000000000000000, 1.000000000000000000, -0.000000000000000000 ) ) ;
#51984=ORIENTED_EDGE ( 'NONE', *, *, #54679, .F. ) ;
#51985=VECTOR ( 'NONE', #18913, 1000.000000000000000 ) ;
#51989=ORIENTED_EDGE ( 'NONE', *, *, #43588, .T. ) ;
#51990=CARTESIAN_POINT ( 'NONE',  ( -2.500000000000000444, -60.04166666393547303, -4.330127018922193649 ) ) ;
#51992=CARTESIAN_POINT ( 'NONE',  ( -4.458734124999999437, -79.56249999863440792, 0.000000000000000000 ) ) ;
#51994=CYLINDRICAL_SURFACE ( 'NONE', #44945, 5.000000000000000000 ) ;
#52001=( BOUNDED_CURVE ( )  B_SPLINE_CURVE ( 2, ( #57914, #13835, #33455, #53072, #12890, #22877, #48240, #24124, #4197 ),
 .UNSPECIFIED., .F., .F. ) 
 B_SPLINE_CURVE_WITH_KNOTS ( ( 3, 2, 2, 2, 3 ),
 ( 0.1937500000000000056, 0.1944444444444444475, 0.1958333333333333315, 0.1972222222222222154, 0.1979166666666666574 ),
 .UNSPECIFIED. ) 
 CURVE ( )  GEOMETRIC_REPRESENTATION_ITEM ( )  RATIONAL_B_SPLINE_CURVE ( ( 0.9330127018922194093, 0.9330127018922194093, 1.000000000000000000, 0.8660254037844387076, 1.000000000000000000, 0.8660254037844387076, 1.000000000000000000, 0.9330127018922194093, 0.9330127018922194093 ) ) 
 REPRESENTATION_ITEM ( '' )  );
#52003=CARTESIAN_POINT ( 'NONE',  ( -9.184850993605147944E-16, -154.3750000027311842, 5.000000000000000000 ) ) ;
#52004=EDGE_CURVE ( 'NONE', #21047, #23493, #48067, .T. ) ;
#52007=CYLINDRICAL_SURFACE ( 'NONE', #57143, 5.000000000000000000 ) ;
#52009=CARTESIAN_POINT ( 'NONE',  ( 9.457646018065525792E-16, -81.31249999863440792, 5.148502694627439702 ) ) ;
#52012=ORIENTED_EDGE ( 'NONE', *, *, #36761, .T. ) ;
#52013=LINE ( 'NONE', #61673, #37155 ) ;
#52015=CARTESIAN_POINT ( 'NONE',  ( 5.000000000000000888, -164.0625000027312126, -2.071067811865475505 ) ) ;
#52017=CARTESIAN_POINT ( 'NONE',  ( -4.458734124999999437, 10.35416666803225993, -2.574251347313719407 ) ) ;
#52020=( BOUNDED_CURVE ( )  B_SPLINE_CURVE ( 2, ( #24814, #58283, #13590, #9378, #57664, #14202, #38958, #33828, #28989 ),
 .UNSPECIFIED., .F., .F. ) 
 B_SPLINE_CURVE_WITH_KNOTS ( ( 3, 2, 2, 2, 3 ),
 ( 0.2583333333333335813, 0.2625000000000002331, 0.2666666666666668850, 0.2708333333333335369, 0.2750000000000002442 ),
 .UNSPECIFIED. ) 
 CURVE ( )  GEOMETRIC_REPRESENTATION_ITEM ( )  RATIONAL_B_SPLINE_CURVE ( ( 0.9999999999999958922, 0.9238795325112908463, 1.000000000000000000, 0.9238795325112867385, 1.000000000000000000, 0.9238795325112867385, 1.000000000000000000, 0.9238795325112826307, 1.000000000000003997 ) ) 
 REPRESENTATION_ITEM ( '' )  );
#52024=CARTESIAN_POINT ( 'NONE',  ( -2.071067811865404451, -163.3125000000000284, 5.000000000000073719 ) ) ;
#52026=CARTESIAN_POINT ( 'NONE',  ( -4.458734124999999437, -10.39583333196773474, -2.574251347313719407 ) ) ;
#52027=DIRECTION ( 'NONE',  ( 0.000000000000000000, 0.000000000000000000, 1.000000000000000000 ) ) ;
#52029=VERTEX_POINT ( 'NONE', #18789 ) ;
#52030=CARTESIAN_POINT ( 'NONE',  ( -3.152548672688508926E-16, -35.81249999863440792, -5.148502694627439702 ) ) ;
#52032=ADVANCED_FACE ( 'NONE', ( #38115 ), #13664, .T. ) ;
#52036=AXIS2_PLACEMENT_3D ( 'NONE', #55614, #45306, #44991 ) ;
#52038=CARTESIAN_POINT ( 'NONE',  ( -3.152801135295367096, -151.3125000013655779, -3.152801135295367541 ) ) ;
#52039=CARTESIAN_POINT ( 'NONE',  ( -4.458734124999999437, 15.60416666803225993, -2.574251347313719407 ) ) ;
#52041=CARTESIAN_POINT ( 'NONE',  ( 1.975475456537005874E-15, -81.62499999726881583, 5.000000000000000000 ) ) ;
#52042=CARTESIAN_POINT ( 'NONE',  ( -1.339745962155610925, -64.66965819600733312, 5.000000000000000000 ) ) ;
#52043=CARTESIAN_POINT ( 'NONE',  ( 4.458734124999999437, -86.06249999863439371, -5.460374474430324690E-16 ) ) ;
#52046=CARTESIAN_POINT ( 'NONE',  ( 1.060575238724906964E-15, 18.37500000273118772, 5.773502691896257311 ) ) ;
#52048=CARTESIAN_POINT ( 'NONE',  ( -6.972266317189433020E-16, -79.24999999999998579, -5.000000000000000000 ) ) ;
#52049=DIRECTION ( 'NONE',  ( -0.000000000000000000, 1.000000000000000000, -0.000000000000000000 ) ) ;
#52050=CARTESIAN_POINT ( 'NONE',  ( 2.499999999999998668, -52.33333333333332860, -4.330127018922193649 ) ) ;
#52051=CARTESIAN_POINT ( 'NONE',  ( 2.500000000000002220, -29.66666666666666785, 4.330127018922192761 ) ) ;
#52052=CARTESIAN_POINT ( 'NONE',  ( -2.229367062499996610, -35.14583333196772941, 3.861377020970582219 ) ) ;
#52053=CARTESIAN_POINT ( 'NONE',  ( 1.339745962155612702, 0.7053418012614794952, -5.000000000000000000 ) ) ;
#52054=CARTESIAN_POINT ( 'NONE',  ( 5.000000000000000000, -27.29166666393547658, -2.886751345948129988 ) ) ;
#52055=CARTESIAN_POINT ( 'NONE',  ( -2.229367062500000163, -59.47916666530106511, -3.861377020970580443 ) ) ;
#52058=CARTESIAN_POINT ( 'NONE',  ( 2.229367062500001939, -9.229166665301075767, 3.861377020970579999 ) ) ;
#52060=CARTESIAN_POINT ( 'NONE',  ( -3.535250795749689387E-16, -69.24999999999998579, -5.773502691896257311 ) ) ;
#52063=CARTESIAN_POINT ( 'NONE',  ( -2.500000000000000444, -76.04166666393547303, -4.330127018922193649 ) ) ;
#52064=CARTESIAN_POINT ( 'NONE',  ( 3.061616997868383141E-16, -150.8750000027312126, -5.000000000000000000 ) ) ;
#52065=ORIENTED_EDGE ( 'NONE', *, *, #14545, .F. ) ;
#52067=CARTESIAN_POINT ( 'NONE',  ( -4.458734124999998549, -24.47916666530107577, 2.574251347313722516 ) ) ;
#52068=CARTESIAN_POINT ( 'NONE',  ( 4.458734124999998549, -58.97916666530105800, -2.574251347313721627 ) ) ;
#52070=CARTESIAN_POINT ( 'NONE',  ( -1.846868145590737420, -141.7500000013655779, 4.458734124999999437 ) ) ;
#52072=CARTESIAN_POINT ( 'NONE',  ( 1.975475456537005874E-15, -52.62499999726880873, 5.000000000000000000 ) ) ;
#52082=CARTESIAN_POINT ( 'NONE',  ( -3.152801135295367096, -147.3125000013655779, -3.152801135295367541 ) ) ;
#52086=CARTESIAN_POINT ( 'NONE',  ( -2.229367062500000163, -64.72916666530106511, -3.861377020970580443 ) ) ;
#52087=CARTESIAN_POINT ( 'NONE',  ( -6.972266317189433020E-16, -62.24999999999999289, -5.000000000000000000 ) ) ;
#52089=CARTESIAN_POINT ( 'NONE',  ( 4.458734124999999437, -144.3750000013656063, -1.846868145590734978 ) ) ;
#52092=CARTESIAN_POINT ( 'NONE',  ( -5.000000000000000000, -164.6250000027311842, -6.123233995736766282E-16 ) ) ;
#52093=CARTESIAN_POINT ( 'NONE',  ( 5.000000000000000000, 16.50000000000000000, -6.123233995736766282E-16 ) ) ;
#52098=CYLINDRICAL_SURFACE ( 'NONE', #26314, 5.000000000000000000 ) ;
#52101=CARTESIAN_POINT ( 'NONE',  ( 1.339745962155615144, -56.58034179853028434, 4.999999999999999112 ) ) ;
#52102=CARTESIAN_POINT ( 'NONE',  ( 5.000000000000000888, 21.41666666666666430, 2.886751345948126879 ) ) ;
#52103=CARTESIAN_POINT ( 'NONE',  ( -3.152548672688508926E-16, 8.437500001365595637, -5.148502694627439702 ) ) ;
#52105=CARTESIAN_POINT ( 'NONE',  ( -2.229367062499996610, -21.39583333196774007, 3.861377020970582219 ) ) ;
#52107=CARTESIAN_POINT ( 'NONE',  ( 4.458734125000000326, -158.3750000013655779, -1.846868145590734978 ) ) ;
#52111=CARTESIAN_POINT ( 'NONE',  ( 6.042630808230842148E-15, 26.75000000000000000, -4.999999999999999112 ) ) ;
#52112=CARTESIAN_POINT ( 'NONE',  ( 9.457646018065525792E-16, -39.06249999863440081, 5.148502694627439702 ) ) ;
#52114=CARTESIAN_POINT ( 'NONE',  ( 4.458734124999999437, -70.06249999863439371, -5.460374474430324690E-16 ) ) ;
#52116=CARTESIAN_POINT ( 'NONE',  ( -2.499999999999996447, -40.83333333333333570, 4.330127018922195425 ) ) ;
#52118=ORIENTED_EDGE ( 'NONE', *, *, #42476, .T. ) ;
#52122=CARTESIAN_POINT ( 'NONE',  ( -2.499999999999996447, -14.83333333333333037, 4.330127018922195425 ) ) ;
#52123=CARTESIAN_POINT ( 'NONE',  ( -4.458734124999998549, -15.22916666530107754, 2.574251347313722516 ) ) ;
#52125=CARTESIAN_POINT ( 'NONE',  ( -2.229367062500000163, -78.47916666530106511, -3.861377020970580443 ) ) ;
#52127=CARTESIAN_POINT ( 'NONE',  ( 1.975475456537005874E-15, -72.62499999726878741, 5.000000000000000000 ) ) ;
#52128=CARTESIAN_POINT ( 'NONE',  ( 5.000000000000000888, -14.45833333060214976, 2.886751345948126879 ) ) ;
#52129=CARTESIAN_POINT ( 'NONE',  ( 4.458734124999999437, -43.81249999863440081, -5.460374474430324690E-16 ) ) ;
#52130=VERTEX_POINT ( 'NONE', #53752 ) ;
#52132=CARTESIAN_POINT ( 'NONE',  ( -4.458734124999998549, 8.520833334698926009, 2.574251347313722516 ) ) ;
#52133=ORIENTED_EDGE ( 'NONE', *, *, #8369, .F. ) ;
#52134=CARTESIAN_POINT ( 'NONE',  ( 1.339745962155615144, -81.58034179853029855, 4.999999999999999112 ) ) ;
#52135=CARTESIAN_POINT ( 'NONE',  ( -5.000000000000000000, -55.99999999999999289, 0.000000000000000000 ) ) ;
#52136=CARTESIAN_POINT ( 'NONE',  ( 1.846868145590736310, -159.8750000013655779, 4.458734124999999437 ) ) ;
#52139=CARTESIAN_POINT ( 'NONE',  ( -4.458734124999999437, -82.31249999863440792, 0.000000000000000000 ) ) ;
#52140=CARTESIAN_POINT ( 'NONE',  ( 5.000000000000000000, -166.0625000000000000, 2.071067811865478614 ) ) ;
#52143=CARTESIAN_POINT ( 'NONE',  ( 4.458734124999999437, -2.062499998634406584, -5.460374474430324690E-16 ) ) ;
#52144=CARTESIAN_POINT ( 'NONE',  ( 9.457646018065525792E-16, -43.31249999863440792, 5.148502694627439702 ) ) ;
#52147=CARTESIAN_POINT ( 'NONE',  ( -6.972266317189433020E-16, -86.25000000000001421, -5.000000000000000000 ) ) ;
#52150=CARTESIAN_POINT ( 'NONE',  ( -5.000000000000000000, -18.95833333060214798, -2.886751345948128211 ) ) ;
#52151=CARTESIAN_POINT ( 'NONE',  ( 9.457646018065525792E-16, -68.31249999863442213, 5.148502694627439702 ) ) ;
#52153=ORIENTED_EDGE ( 'NONE', *, *, #10676, .T. ) ;
#52154=CARTESIAN_POINT ( 'NONE',  ( -5.000000000000000000, -150.6250000027312126, -6.123233995736766282E-16 ) ) ;
#52158=CARTESIAN_POINT ( 'NONE',  ( -4.458734124999999437, 1.604166668032262155, -2.574251347313719407 ) ) ;
#52160=CARTESIAN_POINT ( 'NONE',  ( 3.152801135295366208, -158.5625000013656063, 3.152801135295367985 ) ) ;
#52162=ORIENTED_EDGE ( 'NONE', *, *, #44364, .T. ) ;
#52172=CARTESIAN_POINT ( 'NONE',  ( 2.229367062499998831, 22.35416666803225993, -3.861377020970580887 ) ) ;
#52174=CARTESIAN_POINT ( 'NONE',  ( -4.458734124999999437, -1.562499998634406140, 0.000000000000000000 ) ) ;
#52177=CARTESIAN_POINT ( 'NONE',  ( -9.184850993605147944E-16, -142.3750000027312126, 5.000000000000000000 ) ) ;
#52182=CARTESIAN_POINT ( 'NONE',  ( 1.975475456537005874E-15, -86.75000000000001421, 5.000000000000000000 ) ) ;
#52183=CYLINDRICAL_SURFACE ( 'NONE', #22381, 5.000000000000000000 ) ;
#52185=CARTESIAN_POINT ( 'NONE',  ( 3.152801135295366208, -155.8125000013656063, 3.152801135295367985 ) ) ;
#52188=ORIENTED_EDGE ( 'NONE', *, *, #1539, .F. ) ;
#52189=CARTESIAN_POINT ( 'NONE',  ( 4.458734124999998549, 16.02083333469892423, -2.574251347313721627 ) ) ;
#52190=EDGE_LOOP ( 'NONE', ( #22724, #55657, #61251, #38916 ) ) ;
#52195=CARTESIAN_POINT ( 'NONE',  ( -4.999999999999999112, 7.083333333333333037, 2.886751345948131764 ) ) ;
#52196=CARTESIAN_POINT ( 'NONE',  ( 2.229367062500001939, -62.97916666530106511, 3.861377020970579999 ) ) ;
#52198=DIRECTION ( 'NONE',  ( 0.000000000000000000, 0.000000000000000000, 1.000000000000000000 ) ) ;
#52200=CARTESIAN_POINT ( 'NONE',  ( -4.458734124999999437, -30.39583333196773651, -2.574251347313719407 ) ) ;
#52204=CARTESIAN_POINT ( 'NONE',  ( -2.500000000000000444, -38.16666666666667140, -4.330127018922193649 ) ) ;
#52205=CARTESIAN_POINT ( 'NONE',  ( 6.123233995736766282E-16, -170.0000000000000000, -5.000000000000000000 ) ) ;
#52209=CYLINDRICAL_SURFACE ( 'NONE', #21450, 5.000000000000000000 ) ;
#52210=CARTESIAN_POINT ( 'NONE',  ( -4.458734124999999437, -67.39583333196773651, -2.574251347313719407 ) ) ;
#52211=CARTESIAN_POINT ( 'NONE',  ( -8.190561711645485556E-16, -147.9375000013656063, 4.458734124999999437 ) ) ;
#52212=CARTESIAN_POINT ( 'NONE',  ( 4.458734124999998549, -73.72916666530106511, -2.574251347313721627 ) ) ;
#52213=EDGE_CURVE ( 'NONE', #26895, #14751, #4247, .T. ) ;
#52216=CARTESIAN_POINT ( 'NONE',  ( 2.229367062499998831, -25.89583333196773651, -3.861377020970580887 ) ) ;
#52217=CARTESIAN_POINT ( 'NONE',  ( 2.500000000000002220, -60.54166666393547303, 4.330127018922192761 ) ) ;
#52219=LINE ( 'NONE', #45804, #39475 ) ;
#52220=VERTEX_POINT ( 'NONE', #24491 ) ;
#52224=EDGE_LOOP ( 'NONE', ( #3473, #1851, #19693, #30493 ) ) ;
#52226=CARTESIAN_POINT ( 'NONE',  ( -1.339745962155610925, -55.66965819600732601, 5.000000000000000000 ) ) ;
#52227=CARTESIAN_POINT ( 'NONE',  ( -4.458734124999998549, -56.47916666530107221, 2.574251347313722516 ) ) ;
#52228=EDGE_LOOP ( 'NONE', ( #42560, #25232, #24038, #56071 ) ) ;
#52230=ADVANCED_FACE ( 'NONE', ( #58278 ), #48922, .T. ) ;
#52232=EDGE_CURVE ( 'NONE', #45099, #5936, #44096, .T. ) ;
#52234=CARTESIAN_POINT ( 'NONE',  ( 2.229367062499998831, 20.35416666803225993, -3.861377020970580887 ) ) ;
#52236=CARTESIAN_POINT ( 'NONE',  ( 1.339745962155602488, 20.41965820146970145, 5.000000000000007105 ) ) ;
#52237=CARTESIAN_POINT ( 'NONE',  ( 3.061616997868383141E-16, -164.7500000000000000, -5.000000000000000000 ) ) ;
#52238=EDGE_LOOP ( 'NONE', ( #55613, #49536, #21419, #40333 ) ) ;
#52242=EDGE_CURVE ( 'NONE', #39123, #41613, #49251, .T. ) ;
#52243=FACE_OUTER_BOUND ( 'NONE', #61247, .T. ) ;
#52246=CARTESIAN_POINT ( 'NONE',  ( 5.000000000000000000, 4.583333333333331261, -2.886751345948130876 ) ) ;
#52247=CARTESIAN_POINT ( 'NONE',  ( 5.000000000000000000, -161.0000000000000000, 0.000000000000000000 ) ) ;
#52248=FACE_OUTER_BOUND ( 'NONE', #49815, .T. ) ;
#52257=CARTESIAN_POINT ( 'NONE',  ( 5.000000000000000888, -155.0625000027312126, -2.071067811865475505 ) ) ;
#52260=VECTOR ( 'NONE', #33298, 1000.000000000000000 ) ;
#52264=CARTESIAN_POINT ( 'NONE',  ( 2.071067811865476394, -145.1875000000000284, 5.000000000000000000 ) ) ;
#52268=CARTESIAN_POINT ( 'NONE',  ( -1.846868145590737420, -169.0000000013655779, 4.458734124999997661 ) ) ;
#52269=CARTESIAN_POINT ( 'NONE',  ( -3.152548672688508926E-16, -24.56249999863440792, -5.148502694627439702 ) ) ;
#52270=CARTESIAN_POINT ( 'NONE',  ( 1.339745962155615144, 14.29465819873852084, 4.999999999999999112 ) ) ;
#52273=CARTESIAN_POINT ( 'NONE',  ( 1.846868145590735200, -148.2500000013656063, -4.458734125000000326 ) ) ;
#52274=EDGE_LOOP ( 'NONE', ( #60218, #52188, #51462, #5063 ) ) ;
#52276=CARTESIAN_POINT ( 'NONE',  ( -4.458734124999999437, -53.56249999863439371, 0.000000000000000000 ) ) ;
#52279=CARTESIAN_POINT ( 'NONE',  ( 1.060575238724906964E-15, 22.24999999999999645, 5.773502691896257311 ) ) ;
#52280=CARTESIAN_POINT ( 'NONE',  ( 0.000000000000000000, -170.0000000000000000, 0.000000000000000000 ) ) ;
#52281=CARTESIAN_POINT ( 'NONE',  ( -2.229367062500000163, -3.479166665301069994, -3.861377020970580443 ) ) ;
#52282=CARTESIAN_POINT ( 'NONE',  ( 5.000000000000000888, -48.58333333333333570, 2.886751345948126879 ) ) ;
#52283=CARTESIAN_POINT ( 'NONE',  ( -2.071067811865538566, -164.6875000000000284, -4.999999999999937828 ) ) ;
#52284=CARTESIAN_POINT ( 'NONE',  ( 4.458734125000001214, 10.85416666803225993, 2.574251347313718519 ) ) ;
#52287=CARTESIAN_POINT ( 'NONE',  ( 2.500000000000002220, -42.66666666666667140, 4.330127018922192761 ) ) ;
#52288=VERTEX_POINT ( 'NONE', #63424 ) ;
#52289=CARTESIAN_POINT ( 'NONE',  ( -2.500000000000000444, -71.16666666666667140, -4.330127018922193649 ) ) ;
#52290=CARTESIAN_POINT ( 'NONE',  ( -2.229367062500000163, -47.47916666530106511, -3.861377020970580443 ) ) ;
#52291=CARTESIAN_POINT ( 'NONE',  ( -1.846868145590737420, -159.0000000013656063, 4.458734124999999437 ) ) ;
#52292=EDGE_CURVE ( 'NONE', #5936, #57819, #45341, .T. ) ;
#52294=CARTESIAN_POINT ( 'NONE',  ( -4.999999999999999112, -46.79166666393546592, 2.886751345948131764 ) ) ;
#52296=VERTEX_POINT ( 'NONE', #25771 ) ;
#52297=CARTESIAN_POINT ( 'NONE',  ( 2.229367062500001939, -25.97916666530106866, 3.861377020970579999 ) ) ;
#52298=ORIENTED_EDGE ( 'NONE', *, *, #7927, .F. ) ;
#52300=CARTESIAN_POINT ( 'NONE',  ( 1.846868145590735200, -162.2500000013656347, -4.458734125000000326 ) ) ;
#52302=( BOUNDED_SURFACE ( )  B_SPLINE_SURFACE ( 1, 2, ( 
 ( #48537, #24103, #23790, #63037, #38878, #47902, #43699, #48220, #33130, #58192, #39195, #34059, #58820, #24732, #44334, #38563, #300, #19897, #3858, #23479, #43082, #62720, #18645, #8990, #4175, #1272, #31144, #50462, #10258, #45304, #59472, #20873, #35340, #40474, #20555, #40157, #15721, #34695, #25694, #5430, #44657, #15406, #15081, #20229, #6713, #25369, #16036, #59800, #50771, #54320, #16362, #54959, #26322, #45940, #6402, #6083, #60115, #35665, #11528, #50127, #619, #29859, #1903, #21510, #5751, #55290, #49806, #49492, #11209, #25047, #10889, #59149, #40790, #30832, #26011, #45628, #1583, #21183, #60437, #35983, #39829, #35030, #55612, #54642, #10566, #30176, #44989, #955, #30505, #7033, #22142, #42061, #37249, #17308, #57196, #7985, #41424, #46584, #56876, #27583, #27900, #46263, #32094, #36298, #32415, #12481, #11836, #61386, #61703, #47218, #41107, #36934, #37556, #55921, #17932, #61073, #17632, #31782, #13116, #32733, #7670, #3161, #31455, #52360, #7356, #36611, #2222, #3472, #12795, #52046, #8298, #51096, #47521, #16677, #60752, #26644, #56560, #51730, #21826, #26966, #16994, #22780, #56242, #12163, #27277, #42375, #51413, #46903, #2527, #41737, #22464, #2844, #62014, #33361, #28530, #33054, #19185, #53608, #14675, #33988, #18253, #14048, #37880, #23408, #24021, #9542, #29146, #52976, #43625, #38798, #52668, #58437, #63267, #14364, #33672, #23723, #13428, #48148, #24338, #34296, #49090, #39120, #43319, #62955, #18872, #4100, #57512, #48768, #53291, #38489, #8602, #58116, #43939, #53919, #23085, #58747, #9227, #28840, #48464, #4401, #28212, #4713, #47826, #3786, #9844, #29459, #8917, #63586, #13740, #43007, #19507, #62653, #42688, #62332, #18572, #38193, #57818, #20794, #15962, #60037, #6322, #6011, #24655, #40712, #1194, #25927, #40397, #45546, #35904, #15324, #31067, #34611, #49733, #25613, #35584, #44915, #21107, #55211, #5358, #10489, #11128, #30755, #55538, #10179, #59718, #225, #50375, #40075, #39432, #25289, #45227, #1506, #5036, #870, #60361, #19823, #16285, #24977, #11448, #59391, #44261, #59073, #35263, #14998, #54238, #29782, #34948, #541, #49415, #44584, #20152, #39749, #54567, #30102, #5678, #20473, #15647, #54884, #10814, #30426, #50053, #16914, #51015, #38036, #47994, #50691, #46509, #2765, #6960, #17233, #36531, #56163, #32021, #6634, #46188, #60994, #12085, #60678, #46821, #18415, #43164, #61627, #45862, #41657, #1828, #26570, #51658, #57668, #13594, #31708, #7595, #22387, #16601, #41988, #27203, #33213, #52831, #13899, #41348, #51342, #2148, #21429, #21753, #7281, #8765, #26892, #26242, #28373, #3946, #41032, #18723, #23569, #62803, #38347, #57973, #2454, #36219, #55843, #11759, #31378, #22065, #61309, #36858, #56487, #12409, #4256, #68, #59231, #10018, #58907, #48305, #39279, #4879, #39595, #23871, #49263, #9076, #5200, #19668, #34788, #9694, #33835, #53452, #24818, #44424, #384, #19987, #29301, #24181, #28993, #28685, #14834, #54080, #33526, #38649, #15164, #43787, #43476, #58287, #14519, #38963, #29629, #48617, #48931, #24501, #63434, #19349, #34448, #63121, #34141, #4556, #53141, #53760, #54410, #10340, #44104, #29949, #49574, #58601, #5517, #25130, #44742, #703, #20313, #39914, #59562, #19032, #14206, #9383, #51185, #6801, #30268, #1667, #15808, #21269, #55373, #40876, #40560, #60203, #35747, #54731, #45715, #25451, #1038, #35424, #35117, #40248, #26733, #45391, #36064, #16125, #7117, #10652, #36377, #11288, #46348, #2304, #26409, #26094, #60518, #16444, #31550, #6484, #59888, #56007, #30914, #21906, #41503, #46027, #55693, #11607, #31227, #15494, #50857, #55048, #60834, #49888, #6163, #50540, #10971, #5839, #30592, #1990, #11921, #25780, #45071, #21594, #41189, #20644, #50213, #16760, #1356, #20960, #52449, #56647, #18339, #3558, #62420, #57282, #8384, #61785, #51500, #47604, #17079, #31867, #27671, #23166, #37639, #22865, #12253, #3252, #32496, #42775, #7437, #13198, #36698, #32820, #47298, #37961, #37327, #61471, #17405, #27985, #57595, #13523, #33141, #56958, #51807, #12563, #56333, #42456, #18016, #61156, #2609, #52756, #7749, #27046, #22227, #42149, #2934, #8685, #32175, #12878, #52128, #27352, #46985, #62099, #46664, #17712, #22547, #41827, #8070, #28298, #47911, #3868, #23488, #37020, #4484, #29230, #54004, #58828, #38887, #58521, #28922, #34067, #14446, #53690, #48856, #15090, #34376, #57900, #4799, #43400, #24423, #19271, #44025, #24113, #43711, #63355, #18653, #9622, #53060, #28611, #63045, #62731, #4184, #54331, #9308, #63672, #19592, #34706, #38275, #39204, #14758, #59157, #9934, #23798, #24741, #5438, #33756, #29549, #18955, #13824, #38571, #49183, #307, #53374, #43090, #5121, #44344, #33443, #10265, #19905, #39520, #29869, #49499, #58202, #9000, #48227, #14129, #48545, #16371, #25703, #15416, #11536, #44666, #59481, #55301, #50781, #1593, #50471, #39838, #30841, #60124, #31153, #35038, #40799, #626, #60446, #11217, #26330, #1281, #25376, #44998, #35990, #55621, #6721, #45948, #20880, #15729, #20565, #20236, #6410, #45636, #25056, #30185, #1913, #35348, #54649, #49813, #6090, #30512, #21192, #40169, #40482, #16045, #54969, #10897, #26020, #10574, #45314, #59808, #5758, #35674, #21518, #41114, #60762, #16687, #36306, #50135, #55930, #11845, #31463, #51103, #963, #56568, #61710, #42070, #17640, #12804, #42697, #62023, #21835, #56884, #7365, #32425, #46911, #52054, #32102, #51738, #27286, #46272, #37256, #17003, #56251, #26973, #26654, #31790, #18262, #36942, #27593, #7680, #62341, #2231, #27908, #2853, #37889, #57519, #17940, #7992, #37565, #57205, #12490, #47227, #22789, #36618, #42383, #3170, #13124, #32742, #22474, #61081, #52369, #8307, #13437, #33063, #23094, #47529, #3480, #7042, #41432, #12174, #51422, #46592, #2536, #22152, #41746, #17320, #61395, #43325, #3795, #38806, #18579, #28850, #59080, #34303, #9549, #53618, #4720, #63594, #43946, #53926, #29154, #8611, #24662, #48777, #9854, #24346, #29465, #19830, #62965, #15007, #38201, #33681, #19514, #39128, #48472, #5044, #58755, #52983, #58124, #14685, #49098, #39443, #57827, #43634, #47836, #44270, #24031, #23416, #9236, #232, #52677, #28220, #4408, #43019, #62659, #13747, #8924, #33368, #18882, #28537, #48157, #19193, #4110, #23730, #38497, #14056, #53302, #63276, #58447, #14371, #33995, #6642, #44590, #41041, #10188, #31076, #26249, #30433, #50062, #50699, #876, #34955, #21115, #45872, #34620, #6017, #50383, #54573, #1201, #20482, #40081, #15967, #54246, #30110, #44921, #59725, #550, #30762, #1512, #1835, #45554, #29788, #25622, #49421, #10495, #35594, #60369, #5365, #21437, #15652, #49740, #59399, #60688, #11138, #6330, #24983, #20159, #39755, #15332, #5684, #25300, #45235, #20801, #35270, #54892, #10821, #40722, #40404, #60043, #55218, #25935, #16292, #35915, #55544, #11455, #61636, #36227, #12093, #26899, #22072, #26577, #12728, #47149, #8231, #27520, #11767, #7606, #31386, #16923, #17568, #3097, #22714, #46519, #37187, #32352, #46196, #51974, #56811, #7915, #27211, #17241, #6967, #41667, #17872, #27834, #42627, #32665, #36865, #56495, #12416, #61317, #51025, #42311, #21763, #2156, #47456, #23024, #2461, #46828, #7289, #41356, #2775, #61000, #32029, #16608, #61951, #37491, #57132, #13048, #52294, #3408, #55853, #36539, #56172, #31716, #51350, #51664, #22395, #41995, #29385, #8849, #24588, #28150, #43247, #63202, #58370, #38424, #14610, #29076, #62583, #4034, #14297, #48703, #49020, #3720, #53228, #57441, #53542, #33609, #32985, #18801, #19113, #4643, #62266, #58050, #58681, #13363, #39053, #18506, #38731, #52912, #34223, #53850, #28776, #28465, #18191, #9467, #33917, #52604, #4966, #24264, #43869, #9779, #63516, #57751, #19440, #37813, #8538, #47765, #23340, #62888, #42942, #38127, #13675, #33294, #48393, #48079, #23653, #23953, #13980, #4335, #9160, #43557, #58998, #59974, #19756, #15897, #30359, #45479, #20405, #44513, #476, #35516, #55139, #11065, #30689, #40004, #34879, #39682, #39367, #5935, #1127, #44194, #49346, #25864, #54501, #14926, #5291, #25224, #49667, #40332, #59321, #59651, #35202, #10425, #30038, #49981, #34533, #44835, #15254, #160, #799, #50306, #25541, #15583, #45159, #54818, #5610, #20728, #6255, #1443, #10749, #21046, #40652, #60292, #16218, #35841, #55465, #11381, #31002, #54168, #50630, #20077, #6567, #10108, #29714, #24909, #7212, #46443, #1761, #56423, #36158, #11695, #46120, #45802, #50950, #37423, #56095, #46754, #26826, #61882, #21364, #47077, #2389, #57057, #17798, #37118, #36792, #12346, #31957, #42241, #17166, #6891, #7841, #52217, #16848, #21999, #26506, #60615, #2085, #41594, #3025, #27443, #22318, #17496, #61244, #16535, #12657, #40969, #55780, #51591, #51900, #2699, #7527, #31315, #27138, #41920, #32273, #21689, #61562, #41280, #56736, #22641, #12967, #32592, #60928, #36469, #26183, #12015, #31645, #51280, #48009, #62513, #3649, #47389, #33540, #28701, #8162, #13289, #53467, #18430, #3340, #32914, #52845, #13609, #4270, #23262, #23582, #62820, #38051, #57683, #57987, #22956, #8779, #42867, #27762, #28389, #23888, #13913, #3962, #53155, #43178, #33227, #9093, #19047, #43490, #18737, #38361, #48320, #63135, #38663, #58302, #14222, #43802, #33849, #42552, #9397, #8471, #29007, #48633, #4572, #24197, #63449, #19367, #62193, #38978, #18112, #57368, #28079, #37735, #52537, #58616, #14536, #34155, #47696, #26665, #9711, #11858, #54427, #2242, #46284, #1925, #720, #39932, #59578, #7052, #44758, #34464, #36318, #17014, #44441, #34805, #54094, #24518, #10033, #10356, #31474, #401, #53777, #21530, #11548, #44119, #21846, #31165, #50797, #41442, #45961, #49279, #51115, #60774, #20003, #29315, #19685, #29965, #55633, #6733, #49590, #61091, #41126, #29646, #59249, #26342, #16699, #48946, #58922, #20330, #4894, #55943, #25147, #83, #5533, #39295, #14851, #5216, #15511, #24834, #39612, #15180, #35132, #57214, #27295, #8621, #13450, #3180, #62350, #31800, #52686, #2865, #32111, #61406, #62668, #13134, #52381, #28230, #46602, #43028, #12186, #33073, #47845, #32434, #52063, #3803, #22484, #36951, #23103, #23426, #36630, #8002, #8318, #56578, #22799, #42079, #61721, #17950, #56262, #51747, #46920, #17650, #2546, #32753, #3489, #51433, #47539, #7376, #27605, #26983, #12499, #37574, #42707, #18272, #37266, #27917, #37898, #22161, #57528, #41757, #17329, #47237, #56893, #7689, #12813, #42392, #62033, #44599, #34631, #19203, #38817, #58458, #63286, #33378, #24673, #23740, #52993, #29798, #24992, #28859, #9559, #9245, #8933, #4732, #48166, #14381, #18588, #243, #39138, #19524, #34313, #29476, #9866, #19840, #58765, #38214, #54257, #14695, #39455, #53936, #59090, #49430, #57837, #14065, #48482, #24043, #28547, #49109, #5054, #10197, #44280, #13756, #29165, #4119, #18892, #15016, #5374, #43334, #4418, #62977, #38506, #58134, #33692, #53311, #43645, #48789, #34005, #53628, #24356, #43957, #63604, #21446, #31083, #30441, #50068, #6024, #25628, #15342, #40728, #49748, #59411, #26255, #1841, #15660, #20807, #59733, #34966, #15973, #54581, #45242, #559, #35921, #30768, #50389, #25945, #21121, #45560, #55550, #6337, #39764, #6649, #1518, #11461, #60375, #50706, #20168, #1210, #10503, #20492, #60049, #16299, #45878, #55224, #30118, #5693, #40410, #35600, #25308, #44929, #885, #11146, #40091, #10827, #35277, #54899, #28752, #14587, #58980, #44493, #58033, #34207, #54481, #9143, #34860, #14280, #14908, #48683, #30020, #10408, #24570, #20059, #54147, #44175 ),
 ( #10086, #49328, #58664, #48377, #455, #13963, #4319, #142, #39663, #34516, #19736, #23939, #39350, #29367, #59300, #29697, #43540, #5271, #24892, #15232, #49648, #53831, #58352, #33899, #5585, #25202, #44816, #778, #9760, #4623, #53522, #33590, #20385, #53209, #63184, #19095, #38713, #24248, #9450, #29059, #39037, #63498, #43852, #19423, #49000, #4947, #50285, #6232, #26159, #15563, #40630, #11041, #39985, #21023, #36131, #45778, #60273, #1737, #16191, #1424, #21340, #50925, #55753, #35818, #55442, #25842, #30980, #11357, #50604, #40940, #11992, #31289, #54801, #60590, #40317, #16510, #6545, #11670, #6866, #26481, #46095, #35183, #2055, #49962, #25521, #59955, #59630, #1103, #51254, #45459, #21663, #41254, #31619, #10729, #60901, #16824, #7189, #26797, #36443, #56072, #46417, #2366, #30336, #5914, #20712, #45139, #15878, #30664, #35498, #55116, #56398, #22294, #42213, #42845, #32246, #42528, #62165, #12943, #22617, #12324, #27419, #23231, #13585, #47983, #38027, #61858, #17775, #37394, #3000, #36768, #28052, #27114, #31935, #33204, #28362, #51876, #32567, #12629, #51563, #8134, #7502, #57029, #21975, #3624, #18085, #22934, #37708, #32886, #13262, #62488, #57345, #41567, #57659, #52514, #18406, #8449, #52819, #8756, #7816, #61220, #46727, #52189, #47672, #17144, #27737, #2672, #41893, #61538, #47050, #17471, #37092, #56711, #47366, #3314, #55053, #61160, #56011, #51189, #60523, #50218, #46353, #15813, #30597, #26414, #21910, #36381, #21599, #10977, #1994, #31231, #2307, #31556, #6168, #11924, #46031, #41193, #17083, #36068, #60206, #16130, #7121, #26737, #41507, #36703, #55697, #50544, #55377, #35429, #60838, #16764, #59893, #1361, #56337, #6488, #25785, #20965, #40880, #1671, #12257, #11292, #11611, #50861, #26098, #45719, #31871, #45396, #16449, #30918, #40565, #6805, #51504, #7442, #27050, #46668, #2613, #21273, #22231, #35752, #57599, #37643, #57286, #27675, #32824, #42460, #22868, #56651, #47915, #46989, #12567, #53064, #48231, #52132, #52453, #32500, #32180, #27989, #7753, #18021, #4188, #23492, #62425, #42780, #13526, #52760, #33145, #43094, #18343, #61475, #13828, #37965, #62735, #8689, #18657, #9004, #8074, #41832, #27356, #62103, #28302, #3873, #13202, #57904, #38279, #42153, #47302, #33447, #28616, #17409, #37024, #51811, #8387, #2938, #47608, #22551, #3562, #61789, #17716, #37330, #23170, #56963, #12882, #3256, #43715, #44349, #14450, #59486, #631, #54009, #29874, #63049, #15421, #20241, #19276, #48549, #49818, #312, #39524, #35043, #33760, #30190, #18959, #39843, #54655, #19597, #39209, #10578, #53695, #24116, #10270, #23802, #43404, #58833, #59162, #63360, #9939, #9627, #29235, #5126, #38575, #38891, #34072, #48860, #53379, #19910, #54336, #58206, #34711, #14133, #14763, #9312, #58526, #24745, #49504, #5443, #4804, #15094, #25061, #28926, #44671, #4488, #24428, #34381, #44030, #36964, #29554, #49188, #61085, #31794, #21840, #6416, #26025, #41436, #35678, #6095, #55935, #2236, #5763, #1599, #21523, #25708, #35995, #55306, #11222, #50787, #25381, #1287, #16050, #30845, #15735, #1918, #36311, #17007, #16692, #968, #60451, #20570, #45319, #6726, #11850, #31468, #50476, #26336, #41119, #35352, #60767, #45953, #51109, #16376, #45641, #59813, #21197, #7046, #36623, #45002, #56255, #40803, #55626, #11541, #31158, #40176, #26659, #10902, #54973, #12180, #30517, #46277, #50140, #60129, #20885, #40488, #17324, #27598, #57832, #33068, #8312, #52374, #3484, #62345, #42701, #52681, #27912, #7369, #23420, #47534, #8616, #23098, #28224, #18583, #61715, #13751, #36946, #32429, #18266, #37893, #47232, #3799, #57522, #51742, #56888, #13442, #47840, #38206, #51426, #43023, #52058, #62663, #22794, #22156, #7996, #26977, #46596, #2540, #3174, #41750, #61400, #56572, #7684, #12494, #42074, #32106, #27290, #17944, #46915, #2857, #22479, #17644, #37260, #12808, #42387, #62027, #37569, #57209, #13128, #32746, #8928, #29792, #24987, #29159, #48783, #48161, #10192, #53306, #53931, #24037, #5369, #49425, #63599, #39448, #28541, #44594, #554, #28854, #58129, #59404, #9860, #49103, #20163, #43329, #39759, #4114, #33373, #52987, #4726, #24351, #23734, #63281, #33685, #19835, #62970, #18887, #43951, #5049, #9240, #19519, #19198, #38811, #14690, #38501, #48476, #43640, #58453, #14060, #29471, #237, #4413, #44275, #14376, #39133, #34000, #53623, #34308, #59085, #15011, #9554, #24667, #34625, #58760, #54251, #36791, #56422, #7211, #16847, #5687, #21688, #17495, #7840, #42239, #32272, #36468, #56094, #12014, #60927, #30113, #22317, #20486, #49743, #27442, #22640, #26505, #26825, #6890, #25303, #2388, #44924, #31644, #15337, #61561, #12345, #17165, #31956, #27137, #7526, #37117, #51590, #34959, #51899, #46752, #56735, #2698, #12656, #47076, #46119, #54576, #879, #51278, #41919, #3024, #46442, #10498, #40085, #16534, #41279, #59728, #36157, #55778, #11694, #31314, #21998, #50949, #41593, #2084, #61243, #62819, #48319, #61881, #18429, #58301, #13912, #9092, #53154, #63134, #18736, #17797, #33848, #57986, #19046, #33539, #38662, #29006, #8470, #24195, #27761, #42866, #38360, #28699, #38050, #14221, #4269, #62192, #3648, #23887, #43489, #48632, #4571, #53466, #62512, #9396, #33225, #32591, #57682, #37422, #57056, #12966, #13608, #52216, #8161, #47388, #18111, #3339, #52536, #22955, #42551, #28388, #37733, #57367, #13288, #32913, #28078, #47695, #23261, #52844, #8778, #48008, #3961, #23581, #43177, #40263, #35437, #39611, #59248, #59904, #10032, #44118, #30284, #15824, #43801, #15178, #59577, #82, #10355, #29645, #49278, #25146, #63448, #39294, #54093, #5215, #53776, #39931, #10667, #55064, #54747, #38977, #34804, #58615, #19683, #44757, #49904, #5857, #24833, #719, #15510, #9710, #35131, #20329, #25465, #54426, #44440, #34154, #400, #45088, #10987, #6180, #30607, #20002, #29964, #49589, #5532, #14535, #1053, #48945, #29314, #50231, #19366, #20659, #4893, #34463, #24517, #58921, #14850, #2006, #32194, #7455, #46366, #26748, #50874, #11940, #36718, #41520, #21610, #41204, #11621, #16775, #60848, #36392, #31567, #61490, #17095, #40575, #51200, #26110, #7132, #56023, #2318, #6818, #26424, #46041, #1373, #21922, #35763, #11303, #45730, #45406, #50554, #37036, #55708, #61172, #56349, #17422, #20974, #46680, #12271, #56662, #12580, #31883, #51517, #27062, #2626, #41843, #22245, #6498, #51823, #25795, #16459, #60216, #1683, #16140, #21283, #55387, #30928, #36078, #40890, #60537, #31241, #42165, #38586, #28313, #3885, #18971, #62436, #23503, #27690, #2950, #9016, #43106, #62747, #8401, #61801, #57917, #27369, #17727, #37979, #33458, #47930, #33157, #22567, #13537, #42795, #13838, #18668, #37343, #38290, #57610, #52771, #28627, #47620, #8086, #47316, #53078, #48244, #4200, #23813, #3574, #62115, #3268, #47002, #8700, #43416, #7765, #12893, #63059, #18034, #56977, #32513, #52465, #13214, #58219, #22880, #23182, #18354, #37657, #57298, #14146, #52144, #28001, #42474, #32836, #33772, #49516, #39535, #34393, #15107, #54019, #25072, #10281, #29886, #44360, #9953, #43728, #58845, #54666, #45013, #15746, #5774, #29568, #49199, #5139, #24756, #4499, #59497, #58539, #24127, #979, #59825, #6, #323, #44041, #63374, #59173, #19288, #19921, #53392, #35054, #5454, #54351, #44682, #643, #20254, #10590, #39854, #9323, #25394, #15436, #30201, #49830, #20582, #40189, #19608, #28936, #38904, #34722, #48560, #14461, #34083, #53706, #9638, #29246, #14774, #48871, #4818, #24438, #39220, #2246, #36006, #21850, #6737, #6106, #55637, #36321, #41446, #35362, #11552, #31805, #50152, #12190, #55318, #55948, #26037, #7379, #51438, #1930, #61095, #10913, #26987, #46606, #30857, #60141, #61412, #11862, #51121, #2551, #45331, #41763, #30529, #22166, #54984, #31170, #50801, #25721, #1609, #35691, #17019, #1301, #20897, #26346, #7058, #11232, #21534, #21208, #40814, #16703, #40499, #50486, #45651, #60462, #16061, #31478, #36634, #6425, #46289, #16387, #45968, #41131, #60778, #26669, #56268, #28236, #47242, #37903, #33078, #27300, #18278, #13458, #57219, #33383, #47850, #17656, #22804, #52691, #3808, #4124, #23746, #23432, #17955, #43033, #52387, #51752, #37579, #57533, #62673, #17335, #13139, #13761, #32116, #57842, #37271, #8626, #8008, #52999, #8938, #47544, #18594, #56585, #28552, #48172, #12818, #42085, #43339, #38221, #36956, #12504, #46925, #7694, #2873, #22489, #61727, #32758, #8323, #56898, #3187, #32439, #52068, #27612, #42398, #27923, #62038, #3495, #23108, #42712, #62354, #9250, #62984, #14070, #33698, #53316, #38511, #28865, #48487, #24050, #4423, #18897, #58139, #50814, #12521, #12208, #36976, #61745, #2892, #46621, #2567, #36653, #41784, #22181, #61429, #56604, #22824, #42099, #1948, #32133, #51141, #51768, #27002, #7712, #31826, #51458, #7395, #26363, #17352, #60792, #36335, #7075, #6751, #11876, #62057, #17037, #27316, #46944, #42414, #45983, #8024, #22504, #17970, #37594, #17673, #37287, #56916, #12834, #3204, #32454, #31495, #52086, #13154, #41462, #27631, #26689, #21549, #46306, #47259, #57238, #16718, #41145, #55965, #2263, #21866, #61112, #56282, #38239, #34028, #24382, #58789, #48816, #33402, #53017, #8958, #13780, #47563, #38846, #37919, #3513, #43983, #39164, #43050, #23762, #23447, #23125, #18915, #62373, #28568, #32774, #14406, #53334, #33715, #48504, #43667, #24071, #53649, #9268, #52409, #4754, #28883, #9584, #4441, #29189, #63630, #62690, #8340, #18296, #48189, #63308, #19230, #4142, #19550, #58480, #33093, #57859, #27939, #42728, #57549, #13477, #52708, #43359, #8642, #63006, #28255, #38529, #47868, #3827, #18612, #58157, #14091, #29504, #55256, #34665, #35308, #5401, #50426, #11175, #44957, #20838, #53963, #6369, #30798, #10222, #39481, #40756, #54928, #30470, #25975, #24701, #21152, #9895, #45590, #1548, #10533, #30145, #14719, #44627, #15046, #1238, #34339, #49136, #49774, #50097, #54284, #917, #587, #20194, #59762, #5080, #29828, #25017, #39796, #44305, #10854, #45272, #269, #25659, #19867, #59117, #49461, #5720, #40440, #60082, #16004, #59442, #6051, #54609, #15371, #34994, #25335, #40121, #35628, #20522, #15688, #42028, #7002, #55578, #1870, #41390, #2191, #56528, #11804, #12127, #51382, #26611, #46228, #46551, #35950, #61038, #31419, #60405, #16962, #12449, #17602, #22747, #16330, #22110, #21795, #2494, #7637, #32060, #56203, #31750, #36573, #7324, #26934, #41703, #61351, #32384, #51696, #11496, #17274, #60719, #36898, #27242, #46866, #2810, #22431, #61669, #31112, #37218, #6678, #45908, #16642, #50734, #21475, #7950, #56844, #12761, #52009, #27552, #26285, #47184, #3126, #41073, #36264, #55890, #51058, #28496, #48115, #58404, #33327, #23055, #23987, #4676, #33019, #23375, #42660, #13080, #62299, #62617, #63234, #52635, #42345, #53261, #62922, #32700, #9500, #18837, #38455, #53573, #52946, #58083, #18221, #37524, #43592, #14014, #33641, #42975, #52330, #28808, #61983, #8265, #8882, #4370, #9196, #4067, #57165, #23686, #13705, #48427, #19148, #27867, #38765, #43286, #14332, #33953, #18541, #37847, #57480, #29110, #48733, #17902, #47487, #38160, #57785, #3440, #13396, #8569, #28180, #47796, #3753, #35550, #30718, #34571, #15288, #14963, #39084, #10453, #53885, #504, #50342, #5967, #44871, #25254, #40038, #35230, #15612, #25578, #834, #43902, #60003, #20439, #45191, #59680, #1158, #55175, #54202, #24298, #9810, #5323, #54849, #10782, #20111, #40363, #30392, #24619, #29747, #50014, #20757, #11094 ) ),
 .UNSPECIFIED., .F., .F., .F. ) 
 B_SPLINE_SURFACE_WITH_KNOTS ( ( 2, 2 ),
 ( 3, 2, 2, 2, 2, 2, 2, 2, 2, 2, 2, 2, 2, 2, 2, 2, 2, 2, 2, 2, 2, 2, 2, 2, 2, 2, 2, 2, 2, 2, 2, 2, 2, 2, 2, 2, 2, 2, 2, 2, 2, 2, 2, 2, 2, 2, 2, 2, 2, 2, 2, 2, 2, 2, 2, 2, 2, 2, 2, 2, 2, 2, 2, 2, 2, 2, 2, 2, 2, 2, 2, 2, 2, 2, 2, 2, 2, 2, 2, 2, 2, 2, 2, 2, 2, 2, 2, 2, 2, 2, 2, 2, 2, 2, 2, 2, 2, 2, 2, 2, 2, 2, 2, 2, 2, 2, 2, 2, 2, 2, 2, 2, 2, 2, 2, 2, 2, 2, 2, 2, 2, 2, 2, 2, 2, 2, 2, 2, 2, 2, 2, 2, 2, 2, 2, 2, 2, 2, 2, 2, 2, 2, 2, 2, 2, 2, 2, 2, 2, 2, 2, 2, 2, 2, 2, 2, 2, 2, 2, 2, 2, 2, 2, 2, 2, 2, 2, 2, 2, 2, 2, 2, 2, 2, 2, 2, 2, 2, 2, 2, 2, 2, 2, 2, 2, 2, 2, 2, 2, 2, 2, 2, 2, 2, 2, 2, 2, 2, 2, 2, 2, 2, 2, 2, 2, 2, 2, 2, 2, 2, 2, 2, 2, 2, 2, 2, 2, 2, 2, 2, 2, 2, 2, 2, 2, 2, 2, 2, 2, 2, 2, 2, 2, 2, 2, 2, 2, 2, 2, 2, 2, 2, 2, 2, 2, 2, 2, 2, 2, 2, 2, 2, 2, 2, 2, 2, 2, 2, 2, 2, 2, 2, 2, 2, 2, 2, 2, 2, 2, 2, 2, 2, 2, 2, 2, 2, 2, 2, 2, 2, 2, 2, 2, 2, 2, 2, 2, 2, 2, 2, 2, 2, 2, 2, 2, 2, 2, 2, 2, 2, 2, 2, 2, 2, 2, 2, 2, 2, 2, 2, 2, 2, 2, 2, 2, 2, 2, 2, 2, 2, 2, 2, 2, 2, 2, 2, 2, 2, 2, 2, 2, 2, 2, 2, 2, 2, 2, 2, 2, 2, 2, 2, 2, 2, 2, 2, 2, 2, 2, 2, 2, 2, 2, 2, 2, 2, 2, 2, 2, 2, 2, 2, 2, 2, 2, 2, 2, 2, 2, 2, 2, 2, 2, 2, 2, 2, 2, 2, 2, 2, 2, 2, 2, 2, 2, 2, 2, 2, 2, 2, 2, 2, 2, 2, 2, 2, 2, 2, 2, 2, 2, 2, 2, 2, 2, 2, 2, 2, 2, 2, 2, 2, 2, 2, 2, 2, 2, 2, 2, 2, 2, 2, 2, 2, 2, 2, 2, 2, 2, 2, 2, 2, 2, 2, 2, 2, 2, 2, 2, 2, 2, 2, 2, 2, 2, 2, 2, 2, 2, 2, 2, 2, 2, 2, 2, 2, 2, 2, 2, 2, 2, 2, 2, 2, 2, 2, 2, 2, 2, 2, 2, 2, 2, 2, 2, 2, 2, 2, 2, 2, 2, 2, 2, 2, 2, 2, 2, 2, 2, 2, 2, 2, 2, 2, 2, 2, 2, 2, 2, 2, 2, 2, 2, 2, 2, 2, 2, 2, 2, 2, 2, 2, 2, 2, 2, 2, 2, 2, 2, 2, 2, 2, 2, 2, 2, 2, 2, 2, 2, 2, 2, 2, 2, 2, 2, 2, 2, 2, 2, 2, 2, 2, 2, 2, 2, 2, 2, 2, 2, 2, 2, 2, 2, 2, 2, 2, 2, 2, 2, 2, 2, 2, 2, 2, 2, 2, 2, 2, 2, 2, 2, 2, 2, 2, 2, 2, 2, 2, 2, 2, 2, 2, 2, 2, 2, 2, 2, 2, 2, 2, 2, 2, 2, 2, 2, 2, 2, 2, 2, 2, 2, 2, 2, 2, 2, 2, 2, 2, 2, 2, 2, 2, 2, 2, 2, 2, 2, 2, 2, 2, 2, 2, 2, 2, 2, 2, 2, 2, 2, 2, 2, 2, 2, 2, 2, 2, 2, 2, 2, 2, 2, 2, 2, 2, 2, 2, 2, 2, 2, 2, 2, 2, 2, 2, 2, 2, 2, 2, 2, 2, 2, 2, 2, 2, 2, 2, 2, 2, 2, 2, 2, 2, 2, 2, 2, 2, 2, 2, 2, 2, 2, 2, 2, 2, 2, 2, 2, 2, 2, 2, 2, 2, 2, 2, 2, 2, 2, 2, 2, 2, 2, 2, 2, 2, 2, 2, 2, 2, 2, 2, 2, 2, 2, 2, 2, 2, 2, 2, 2, 2, 3 ),
 ( 0.000000000000000000, 1.000000000000000000 ),
 ( 0.000000000000000000, 0.001388888888888888942, 0.002777777777777777884, 0.004166666666666666609, 0.005555555555555555768, 0.006944444444444444059, 0.008333333333333333218, 0.009722222222222222376, 0.01111111111111111154, 0.01250000000000000069, 0.01388888888888888812, 0.01527777777777777728, 0.01666666666666666644, 0.01805555555555555386, 0.01944444444444444475, 0.02083333333333333218, 0.02222222222222222307, 0.02361111111111111049, 0.02500000000000000139, 0.02638888888888888881, 0.02777777777777777624, 0.02916666666666666713, 0.03055555555555555455, 0.03194444444444444198, 0.03333333333333333287, 0.03472222222222222376, 0.03611111111111110772, 0.03749999999999999861, 0.03888888888888888951, 0.04027777777777778040, 0.04166666666666666435, 0.04305555555555555525, 0.04444444444444444614, 0.04583333333333333010, 0.04722222222222222099, 0.04861111111111111188, 0.05000000000000000278, 0.05138888888888888673, 0.05277777777777777762, 0.05416666666666666852, 0.05555555555555555247, 0.05694444444444444337, 0.05833333333333333426, 0.05972222222222222515, 0.06111111111111110911, 0.06250000000000000000, 0.06388888888888888395, 0.06527777777777778179, 0.06666666666666666574, 0.06805555555555554970, 0.06944444444444444753, 0.07083333333333333148, 0.07222222222222221544, 0.07361111111111111327, 0.07499999999999999722, 0.07638888888888889506, 0.07777777777777777901, 0.07916666666666666297, 0.08055555555555556080, 0.08194444444444444475, 0.08333333333333332871, 0.08472222222222222654, 0.08611111111111111049, 0.08749999999999999445, 0.08888888888888889228, 0.09027777777777777624, 0.09166666666666666019, 0.09305555555555555802, 0.09444444444444444198, 0.09583333333333333981, 0.09722222222222222376, 0.09861111111111110772, 0.1000000000000000056, 0.1013888888888888895, 0.1027777777777777735, 0.1041666666666666713, 0.1055555555555555552, 0.1069444444444444392, 0.1083333333333333370, 0.1097222222222222210, 0.1111111111111111049, 0.1125000000000000028, 0.1138888888888888867, 0.1152777777777777846, 0.1166666666666666685, 0.1180555555555555525, 0.1194444444444444503, 0.1208333333333333343, 0.1222222222222222182, 0.1236111111111111160, 0.1250000000000000000, 0.1263888888888888840, 0.1277777777777777679, 0.1291666666666666796, 0.1305555555555555636, 0.1319444444444444475, 0.1333333333333333315, 0.1347222222222222154, 0.1361111111111110994, 0.1375000000000000111, 0.1388888888888888951, 0.1402777777777777790, 0.1416666666666666630, 0.1430555555555555469, 0.1444444444444444309, 0.1458333333333333426, 0.1472222222222222265, 0.1486111111111111105, 0.1499999999999999944, 0.1513888888888888784, 0.1527777777777777901, 0.1541666666666666741, 0.1555555555555555580, 0.1569444444444444420, 0.1583333333333333259, 0.1597222222222222099, 0.1611111111111111216, 0.1625000000000000056, 0.1638888888888888895, 0.1652777777777777735, 0.1666666666666666574, 0.1680555555555555691, 0.1694444444444444531, 0.1708333333333333370, 0.1722222222222222210, 0.1736111111111111049, 0.1749999999999999889, 0.1763888888888889006, 0.1777777777777777846, 0.1791666666666666685, 0.1805555555555555525, 0.1819444444444444364, 0.1833333333333333204, 0.1847222222222222321, 0.1861111111111111160, 0.1875000000000000000, 0.1888888888888888840, 0.1902777777777777679, 0.1916666666666666796, 0.1930555555555555636, 0.1944444444444444475, 0.1958333333333333315, 0.1972222222222222154, 0.1986111111111110994, 0.2000000000000000111, 0.2013888888888888951, 0.2027777777777777790, 0.2041666666666666630, 0.2055555555555555469, 0.2069444444444444309, 0.2083333333333333426, 0.2097222222222222265, 0.2111111111111111105, 0.2124999999999999944, 0.2138888888888888784, 0.2152777777777777901, 0.2166666666666666741, 0.2180555555555555580, 0.2194444444444444420, 0.2208333333333333259, 0.2222222222222222099, 0.2236111111111111216, 0.2250000000000000056, 0.2263888888888888895, 0.2277777777777777735, 0.2291666666666666574, 0.2305555555555555691, 0.2319444444444444531, 0.2333333333333333370, 0.2347222222222222210, 0.2361111111111111049, 0.2374999999999999889, 0.2388888888888889006, 0.2402777777777777846, 0.2416666666666666685, 0.2430555555555555525, 0.2444444444444444364, 0.2458333333333333204, 0.2472222222222222321, 0.2486111111111111160, 0.2500000000000000000, 0.2513888888888888840, 0.2527777777777777679, 0.2541666666666666519, 0.2555555555555555358, 0.2569444444444444198, 0.2583333333333333592, 0.2597222222222222432, 0.2611111111111111271, 0.2625000000000000111, 0.2638888888888888951, 0.2652777777777777790, 0.2666666666666666630, 0.2680555555555555469, 0.2694444444444444309, 0.2708333333333333148, 0.2722222222222221988, 0.2736111111111111382, 0.2750000000000000222, 0.2763888888888889062, 0.2777777777777777901, 0.2791666666666666741, 0.2805555555555555580, 0.2819444444444444420, 0.2833333333333333259, 0.2847222222222222099, 0.2861111111111110938, 0.2874999999999999778, 0.2888888888888888618, 0.2902777777777778012, 0.2916666666666666852, 0.2930555555555555691, 0.2944444444444444531, 0.2958333333333333370, 0.2972222222222222210, 0.2986111111111111049, 0.2999999999999999889, 0.3013888888888888729, 0.3027777777777777568, 0.3041666666666666408, 0.3055555555555555802, 0.3069444444444444642, 0.3083333333333333481, 0.3097222222222222321, 0.3111111111111111160, 0.3125000000000000000, 0.3138888888888888840, 0.3152777777777777679, 0.3166666666666666519, 0.3180555555555555358, 0.3194444444444444198, 0.3208333333333333592, 0.3222222222222222432, 0.3236111111111111271, 0.3250000000000000111, 0.3263888888888888951, 0.3277777777777777790, 0.3291666666666666630, 0.3305555555555555469, 0.3319444444444444309, 0.3333333333333333148, 0.3347222222222221988, 0.3361111111111111382, 0.3375000000000000222, 0.3388888888888889062, 0.3402777777777777901, 0.3416666666666666741, 0.3430555555555555580, 0.3444444444444444420, 0.3458333333333333259, 0.3472222222222222099, 0.3486111111111110938, 0.3499999999999999778, 0.3513888888888888618, 0.3527777777777778012, 0.3541666666666666852, 0.3555555555555555691, 0.3569444444444444531, 0.3583333333333333370, 0.3597222222222222210, 0.3611111111111111049, 0.3624999999999999889, 0.3638888888888888729, 0.3652777777777777568, 0.3666666666666666408, 0.3680555555555555802, 0.3694444444444444642, 0.3708333333333333481, 0.3722222222222222321, 0.3736111111111111160, 0.3750000000000000000, 0.3763888888888888840, 0.3777777777777777679, 0.3791666666666666519, 0.3805555555555555358, 0.3819444444444444198, 0.3833333333333333592, 0.3847222222222222432, 0.3861111111111111271, 0.3875000000000000111, 0.3888888888888888951, 0.3902777777777777790, 0.3916666666666666630, 0.3930555555555555469, 0.3944444444444444309, 0.3958333333333333148, 0.3972222222222221988, 0.3986111111111111382, 0.4000000000000000222, 0.4013888888888889062, 0.4027777777777777901, 0.4041666666666666741, 0.4055555555555555580, 0.4069444444444444420, 0.4083333333333333259, 0.4097222222222222099, 0.4111111111111110938, 0.4124999999999999778, 0.4138888888888888618, 0.4152777777777778012, 0.4166666666666666852, 0.4180555555555555691, 0.4194444444444444531, 0.4208333333333333370, 0.4222222222222222210, 0.4236111111111111049, 0.4249999999999999889, 0.4263888888888888729, 0.4277777777777777568, 0.4291666666666666408, 0.4305555555555555802, 0.4319444444444444642, 0.4333333333333333481, 0.4347222222222222321, 0.4361111111111111160, 0.4375000000000000000, 0.4388888888888888840, 0.4402777777777777679, 0.4416666666666666519, 0.4430555555555555358, 0.4444444444444444198, 0.4458333333333333592, 0.4472222222222222432, 0.4486111111111111271, 0.4500000000000000111, 0.4513888888888888951, 0.4527777777777777790, 0.4541666666666666630, 0.4555555555555555469, 0.4569444444444444309, 0.4583333333333333148, 0.4597222222222221988, 0.4611111111111111382, 0.4625000000000000222, 0.4638888888888889062, 0.4652777777777777901, 0.4666666666666666741, 0.4680555555555555580, 0.4694444444444444420, 0.4708333333333333259, 0.4722222222222222099, 0.4736111111111110938, 0.4749999999999999778, 0.4763888888888888618, 0.4777777777777778012, 0.4791666666666666852, 0.4805555555555555691, 0.4819444444444444531, 0.4833333333333333370, 0.4847222222222222210, 0.4861111111111111049, 0.4874999999999999889, 0.4888888888888888729, 0.4902777777777777568, 0.4916666666666666408, 0.4930555555555555802, 0.4944444444444444642, 0.4958333333333333481, 0.4972222222222222321, 0.4986111111111111160, 0.5000000000000000000, 0.5013888888888888840, 0.5027777777777777679, 0.5041666666666666519, 0.5055555555555555358, 0.5069444444444444198, 0.5083333333333333037, 0.5097222222222221877, 0.5111111111111110716, 0.5124999999999999556, 0.5138888888888888395, 0.5152777777777777235, 0.5166666666666667185, 0.5180555555555556024, 0.5194444444444444864, 0.5208333333333333703, 0.5222222222222222543, 0.5236111111111111382, 0.5250000000000000222, 0.5263888888888889062, 0.5277777777777777901, 0.5291666666666666741, 0.5305555555555555580, 0.5319444444444444420, 0.5333333333333333259, 0.5347222222222222099, 0.5361111111111110938, 0.5374999999999999778, 0.5388888888888888618, 0.5402777777777777457, 0.5416666666666666297, 0.5430555555555555136, 0.5444444444444443976, 0.5458333333333332815, 0.5472222222222222765, 0.5486111111111111605, 0.5500000000000000444, 0.5513888888888889284, 0.5527777777777778123, 0.5541666666666666963, 0.5555555555555555802, 0.5569444444444444642, 0.5583333333333333481, 0.5597222222222222321, 0.5611111111111111160, 0.5625000000000000000, 0.5638888888888888840, 0.5652777777777777679, 0.5666666666666666519, 0.5680555555555555358, 0.5694444444444444198, 0.5708333333333333037, 0.5722222222222221877, 0.5736111111111110716, 0.5749999999999999556, 0.5763888888888888395, 0.5777777777777777235, 0.5791666666666667185, 0.5805555555555556024, 0.5819444444444444864, 0.5833333333333333703, 0.5847222222222222543, 0.5861111111111111382, 0.5875000000000000222, 0.5888888888888889062, 0.5902777777777777901, 0.5916666666666666741, 0.5930555555555555580, 0.5944444444444444420, 0.5958333333333333259, 0.5972222222222222099, 0.5986111111111110938, 0.5999999999999999778, 0.6013888888888888618, 0.6027777777777777457, 0.6041666666666666297, 0.6055555555555555136, 0.6069444444444443976, 0.6083333333333332815, 0.6097222222222222765, 0.6111111111111111605, 0.6125000000000000444, 0.6138888888888889284, 0.6152777777777778123, 0.6166666666666666963, 0.6180555555555555802, 0.6194444444444444642, 0.6208333333333333481, 0.6222222222222222321, 0.6236111111111111160, 0.6250000000000000000, 0.6263888888888888840, 0.6277777777777777679, 0.6291666666666666519, 0.6305555555555555358, 0.6319444444444444198, 0.6333333333333333037, 0.6347222222222221877, 0.6361111111111110716, 0.6374999999999999556, 0.6388888888888888395, 0.6402777777777777235, 0.6416666666666667185, 0.6430555555555556024, 0.6444444444444444864, 0.6458333333333333703, 0.6472222222222222543, 0.6486111111111111382, 0.6500000000000000222, 0.6513888888888889062, 0.6527777777777777901, 0.6541666666666666741, 0.6555555555555555580, 0.6569444444444444420, 0.6583333333333333259, 0.6597222222222222099, 0.6611111111111110938, 0.6624999999999999778, 0.6638888888888888618, 0.6652777777777777457, 0.6666666666666666297, 0.6680555555555555136, 0.6694444444444443976, 0.6708333333333332815, 0.6722222222222222765, 0.6736111111111111605, 0.6750000000000000444, 0.6763888888888889284, 0.6777777777777778123, 0.6791666666666666963, 0.6805555555555555802, 0.6819444444444444642, 0.6833333333333333481, 0.6847222222222222321, 0.6861111111111111160, 0.6875000000000000000, 0.6888888888888888840, 0.6902777777777777679, 0.6916666666666666519, 0.6930555555555555358, 0.6944444444444444198, 0.6958333333333333037, 0.6972222222222221877, 0.6986111111111110716, 0.6999999999999999556, 0.7013888888888888395, 0.7027777777777777235, 0.7041666666666667185, 0.7055555555555556024, 0.7069444444444444864, 0.7083333333333333703, 0.7097222222222222543, 0.7111111111111111382, 0.7125000000000000222, 0.7138888888888889062, 0.7152777777777777901, 0.7166666666666666741, 0.7180555555555555580, 0.7194444444444444420, 0.7208333333333333259, 0.7222222222222222099, 0.7236111111111110938, 0.7249999999999999778, 0.7263888888888888618, 0.7277777777777777457, 0.7291666666666666297, 0.7305555555555555136, 0.7319444444444443976, 0.7333333333333332815, 0.7347222222222222765, 0.7361111111111111605, 0.7375000000000000444, 0.7388888888888889284, 0.7402777777777778123, 0.7416666666666666963, 0.7430555555555555802, 0.7444444444444444642, 0.7458333333333333481, 0.7472222222222222321, 0.7486111111111111160, 0.7500000000000000000, 0.7513888888888888840, 0.7527777777777777679, 0.7541666666666666519, 0.7555555555555555358, 0.7569444444444444198, 0.7583333333333333037, 0.7597222222222221877, 0.7611111111111110716, 0.7624999999999999556, 0.7638888888888888395, 0.7652777777777777235, 0.7666666666666667185, 0.7680555555555556024, 0.7694444444444444864, 0.7708333333333333703, 0.7722222222222222543, 0.7736111111111111382, 0.7750000000000000222, 0.7763888888888889062, 0.7777777777777777901, 0.7791666666666666741, 0.7805555555555555580, 0.7819444444444444420, 0.7833333333333333259, 0.7847222222222222099, 0.7861111111111110938, 0.7874999999999999778, 0.7888888888888888618, 0.7902777777777777457, 0.7916666666666666297, 0.7930555555555555136, 0.7944444444444443976, 0.7958333333333332815, 0.7972222222222222765, 0.7986111111111111605, 0.8000000000000000444, 0.8013888888888889284, 0.8027777777777778123, 0.8041666666666666963, 0.8055555555555555802, 0.8069444444444444642, 0.8083333333333333481, 0.8097222222222222321, 0.8111111111111111160, 0.8125000000000000000, 0.8138888888888888840, 0.8152777777777777679, 0.8166666666666666519, 0.8180555555555555358, 0.8194444444444444198, 0.8208333333333333037, 0.8222222222222221877, 0.8236111111111110716, 0.8249999999999999556, 0.8263888888888888395, 0.8277777777777777235, 0.8291666666666667185, 0.8305555555555556024, 0.8319444444444444864, 0.8333333333333333703, 0.8347222222222222543, 0.8361111111111111382, 0.8375000000000000222, 0.8388888888888889062, 0.8402777777777777901, 0.8416666666666666741, 0.8430555555555555580, 0.8444444444444444420, 0.8458333333333333259, 0.8472222222222222099, 0.8486111111111110938, 0.8499999999999999778, 0.8513888888888888618, 0.8527777777777777457, 0.8541666666666666297, 0.8555555555555555136, 0.8569444444444443976, 0.8583333333333332815, 0.8597222222222222765, 0.8611111111111111605, 0.8625000000000000444, 0.8638888888888889284, 0.8652777777777778123, 0.8666666666666666963, 0.8680555555555555802, 0.8694444444444444642, 0.8708333333333333481, 0.8722222222222222321, 0.8736111111111111160, 0.8750000000000000000, 0.8763888888888888840, 0.8777777777777777679, 0.8791666666666666519, 0.8805555555555555358, 0.8819444444444444198, 0.8833333333333333037, 0.8847222222222221877, 0.8861111111111110716, 0.8874999999999999556, 0.8888888888888888395, 0.8902777777777777235, 0.8916666666666667185, 0.8930555555555556024, 0.8944444444444444864, 0.8958333333333333703, 0.8972222222222222543, 0.8986111111111111382, 0.9000000000000000222, 0.9013888888888889062, 0.9027777777777777901, 0.9041666666666666741, 0.9055555555555555580, 0.9069444444444444420, 0.9083333333333333259, 0.9097222222222222099, 0.9111111111111110938, 0.9124999999999999778, 0.9138888888888888618, 0.9152777777777777457, 0.9166666666666666297, 0.9180555555555555136, 0.9194444444444443976, 0.9208333333333332815, 0.9222222222222222765, 0.9236111111111111605, 0.9250000000000000444, 0.9263888888888889284, 0.9277777777777778123, 0.9291666666666666963, 0.9305555555555555802, 0.9319444444444444642, 0.9333333333333333481, 0.9347222222222222321, 0.9361111111111111160, 0.9375000000000000000, 0.9388888888888888840, 0.9402777777777777679, 0.9416666666666666519, 0.9430555555555555358, 0.9444444444444444198, 0.9458333333333333037, 0.9472222222222221877, 0.9486111111111110716, 0.9499999999999999556, 0.9513888888888888395, 0.9527777777777777235, 0.9541666666666667185, 0.9555555555555556024, 0.9569444444444444864, 0.9583333333333333703, 0.9597222222222222543, 0.9611111111111111382, 0.9625000000000000222, 0.9638888888888889062, 0.9652777777777777901, 0.9666666666666666741, 0.9680555555555555580, 0.9694444444444444420, 0.9708333333333333259, 0.9722222222222222099, 0.9736111111111110938, 0.9749999999999999778, 0.9763888888888888618, 0.9777777777777777457, 0.9791666666666666297, 0.9805555555555555136, 0.9819444444444443976, 0.9833333333333332815, 0.9847222222222222765, 0.9861111111111111605, 0.9875000000000000444, 0.9888888888888889284, 0.9902777777777778123, 0.9916666666666666963, 0.9930555555555555802, 0.9944444444444444642, 0.9958333333333333481, 0.9972222222222222321, 0.9986111111111111160, 1.000000000000000000 ),
 .UNSPECIFIED. ) 
 GEOMETRIC_REPRESENTATION_ITEM ( )  RATIONAL_B_SPLINE_SURFACE ( (
 ( 1.000000000000000000, 0.8660254037844387076, 1.000000000000000000, 0.8660254037844387076, 1.000000000000000000, 0.8660254037844387076, 1.000000000000000000, 0.8660254037844387076, 1.000000000000000000, 0.8660254037844387076, 1.000000000000000000, 0.8660254037844387076, 1.000000000000000000, 0.8660254037844387076, 1.000000000000000000, 0.8660254037844387076, 1.000000000000000000, 0.8660254037844387076, 1.000000000000000000, 0.8660254037844387076, 1.000000000000000000, 0.8660254037844387076, 1.000000000000000000, 0.8660254037844387076, 1.000000000000000000, 0.8660254037844387076, 1.000000000000000000, 0.8660254037844387076, 1.000000000000000000, 0.8660254037844387076, 1.000000000000000000, 0.8660254037844387076, 1.000000000000000000, 0.8660254037844387076, 1.000000000000000000, 0.8660254037844387076, 1.000000000000000000, 0.8660254037844387076, 1.000000000000000000, 0.8660254037844387076, 1.000000000000000000, 0.8660254037844387076, 1.000000000000000000, 0.8660254037844387076, 1.000000000000000000, 0.8660254037844387076, 1.000000000000000000, 0.8660254037844387076, 1.000000000000000000, 0.8660254037844387076, 1.000000000000000000, 0.8660254037844387076, 1.000000000000000000, 0.8660254037844387076, 1.000000000000000000, 0.8660254037844387076, 1.000000000000000000, 0.8660254037844387076, 1.000000000000000000, 0.8660254037844387076, 1.000000000000000000, 0.8660254037844387076, 1.000000000000000000, 0.8660254037844387076, 1.000000000000000000, 0.8660254037844387076, 1.000000000000000000, 0.8660254037844387076, 1.000000000000000000, 0.8660254037844387076, 1.000000000000000000, 0.8660254037844387076, 1.000000000000000000, 0.8660254037844387076, 1.000000000000000000, 0.8660254037844387076, 1.000000000000000000, 0.8660254037844387076, 1.000000000000000000, 0.8660254037844387076, 1.000000000000000000, 0.8660254037844387076, 1.000000000000000000, 0.8660254037844387076, 1.000000000000000000, 0.8660254037844387076, 1.000000000000000000, 0.8660254037844387076, 1.000000000000000000, 0.8660254037844387076, 1.000000000000000000, 0.8660254037844387076, 1.000000000000000000, 0.8660254037844387076, 1.000000000000000000, 0.8660254037844387076, 1.000000000000000000, 0.8660254037844387076, 1.000000000000000000, 0.8660254037844387076, 1.000000000000000000, 0.8660254037844387076, 1.000000000000000000, 0.8660254037844387076, 1.000000000000000000, 0.8660254037844387076, 1.000000000000000000, 0.8660254037844387076, 1.000000000000000000, 0.8660254037844387076, 1.000000000000000000, 0.8660254037844387076, 1.000000000000000000, 0.8660254037844387076, 1.000000000000000000, 0.8660254037844387076, 1.000000000000000000, 0.8660254037844387076, 1.000000000000000000, 0.8660254037844387076, 1.000000000000000000, 0.8660254037844387076, 1.000000000000000000, 0.8660254037844387076, 1.000000000000000000, 0.8660254037844387076, 1.000000000000000000, 0.8660254037844387076, 1.000000000000000000, 0.8660254037844387076, 1.000000000000000000, 0.8660254037844387076, 1.000000000000000000, 0.8660254037844387076, 1.000000000000000000, 0.8660254037844387076, 1.000000000000000000, 0.8660254037844387076, 1.000000000000000000, 0.8660254037844387076, 1.000000000000000000, 0.8660254037844387076, 1.000000000000000000, 0.8660254037844387076, 1.000000000000000000, 0.8660254037844387076, 1.000000000000000000, 0.8660254037844387076, 1.000000000000000000, 0.8660254037844387076, 1.000000000000000000, 0.8660254037844387076, 1.000000000000000000, 0.8660254037844387076, 1.000000000000000000, 0.8660254037844387076, 1.000000000000000000, 0.8660254037844387076, 1.000000000000000000, 0.8660254037844387076, 1.000000000000000000, 0.8660254037844387076, 1.000000000000000000, 0.8660254037844387076, 1.000000000000000000, 0.8660254037844387076, 1.000000000000000000, 0.8660254037844387076, 1.000000000000000000, 0.8660254037844387076, 1.000000000000000000, 0.8660254037844387076, 1.000000000000000000, 0.8660254037844387076, 1.000000000000000000, 0.8660254037844387076, 1.000000000000000000, 0.8660254037844387076, 1.000000000000000000, 0.8660254037844387076, 1.000000000000000000, 0.8660254037844387076, 1.000000000000000000, 0.8660254037844387076, 1.000000000000000000, 0.8660254037844387076, 1.000000000000000000, 0.8660254037844387076, 1.000000000000000000, 0.8660254037844387076, 1.000000000000000000, 0.8660254037844387076, 1.000000000000000000, 0.8660254037844387076, 1.000000000000000000, 0.8660254037844387076, 1.000000000000000000, 0.8660254037844387076, 1.000000000000000000, 0.8660254037844387076, 1.000000000000000000, 0.8660254037844387076, 1.000000000000000000, 0.8660254037844387076, 1.000000000000000000, 0.8660254037844387076, 1.000000000000000000, 0.8660254037844387076, 1.000000000000000000, 0.8660254037844387076, 1.000000000000000000, 0.8660254037844387076, 1.000000000000000000, 0.8660254037844387076, 1.000000000000000000, 0.8660254037844387076, 1.000000000000000000, 0.8660254037844387076, 1.000000000000000000, 0.8660254037844387076, 1.000000000000000000, 0.8660254037844387076, 1.000000000000000000, 0.8660254037844387076, 1.000000000000000000, 0.8660254037844387076, 1.000000000000000000, 0.8660254037844387076, 1.000000000000000000, 0.8660254037844387076, 1.000000000000000000, 0.8660254037844387076, 1.000000000000000000, 0.8660254037844387076, 1.000000000000000000, 0.8660254037844387076, 1.000000000000000000, 0.8660254037844387076, 1.000000000000000000, 0.8660254037844387076, 1.000000000000000000, 0.8660254037844387076, 1.000000000000000000, 0.8660254037844387076, 1.000000000000000000, 0.8660254037844387076, 1.000000000000000000, 0.8660254037844387076, 1.000000000000000000, 0.8660254037844387076, 1.000000000000000000, 0.8660254037844387076, 1.000000000000000000, 0.8660254037844387076, 1.000000000000000000, 0.8660254037844387076, 1.000000000000000000, 0.8660254037844387076, 1.000000000000000000, 0.8660254037844387076, 1.000000000000000000, 0.8660254037844387076, 1.000000000000000000, 0.8660254037844387076, 1.000000000000000000, 0.8660254037844387076, 1.000000000000000000, 0.8660254037844387076, 1.000000000000000000, 0.8660254037844387076, 1.000000000000000000, 0.8660254037844387076, 1.000000000000000000, 0.8660254037844387076, 1.000000000000000000, 0.8660254037844387076, 1.000000000000000000, 0.8660254037844387076, 1.000000000000000000, 0.8660254037844387076, 1.000000000000000000, 0.8660254037844387076, 1.000000000000000000, 0.8660254037844387076, 1.000000000000000000, 0.8660254037844387076, 1.000000000000000000, 0.8660254037844387076, 1.000000000000000000, 0.8660254037844387076, 1.000000000000000000, 0.8660254037844387076, 1.000000000000000000, 0.8660254037844387076, 1.000000000000000000, 0.8660254037844387076, 1.000000000000000000, 0.8660254037844387076, 1.000000000000000000, 0.8660254037844387076, 1.000000000000000000, 0.8660254037844387076, 1.000000000000000000, 0.8660254037844387076, 1.000000000000000000, 0.8660254037844387076, 1.000000000000000000, 0.8660254037844387076, 1.000000000000000000, 0.8660254037844387076, 1.000000000000000000, 0.8660254037844387076, 1.000000000000000000, 0.8660254037844387076, 1.000000000000000000, 0.8660254037844387076, 1.000000000000000000, 0.8660254037844387076, 1.000000000000000000, 0.8660254037844387076, 1.000000000000000000, 0.8660254037844387076, 1.000000000000000000, 0.8660254037844387076, 1.000000000000000000, 0.8660254037844387076, 1.000000000000000000, 0.8660254037844387076, 1.000000000000000000, 0.8660254037844387076, 1.000000000000000000, 0.8660254037844387076, 1.000000000000000000, 0.8660254037844387076, 1.000000000000000000, 0.8660254037844387076, 1.000000000000000000, 0.8660254037844387076, 1.000000000000000000, 0.8660254037844387076, 1.000000000000000000, 0.8660254037844387076, 1.000000000000000000, 0.8660254037844387076, 1.000000000000000000, 0.8660254037844387076, 1.000000000000000000, 0.8660254037844387076, 1.000000000000000000, 0.8660254037844387076, 1.000000000000000000, 0.8660254037844387076, 1.000000000000000000, 0.8660254037844387076, 1.000000000000000000, 0.8660254037844387076, 1.000000000000000000, 0.8660254037844387076, 1.000000000000000000, 0.8660254037844387076, 1.000000000000000000, 0.8660254037844387076, 1.000000000000000000, 0.8660254037844387076, 1.000000000000000000, 0.8660254037844387076, 1.000000000000000000, 0.8660254037844387076, 1.000000000000000000, 0.8660254037844387076, 1.000000000000000000, 0.8660254037844387076, 1.000000000000000000, 0.8660254037844387076, 1.000000000000000000, 0.8660254037844387076, 1.000000000000000000, 0.8660254037844387076, 1.000000000000000000, 0.8660254037844387076, 1.000000000000000000, 0.8660254037844387076, 1.000000000000000000, 0.8660254037844387076, 1.000000000000000000, 0.8660254037844387076, 1.000000000000000000, 0.8660254037844387076, 1.000000000000000000, 0.8660254037844387076, 1.000000000000000000, 0.8660254037844387076, 1.000000000000000000, 0.8660254037844387076, 1.000000000000000000, 0.8660254037844387076, 1.000000000000000000, 0.8660254037844387076, 1.000000000000000000, 0.8660254037844387076, 1.000000000000000000, 0.8660254037844387076, 1.000000000000000000, 0.8660254037844387076, 1.000000000000000000, 0.8660254037844387076, 1.000000000000000000, 0.8660254037844387076, 1.000000000000000000, 0.8660254037844387076, 1.000000000000000000, 0.8660254037844387076, 1.000000000000000000, 0.8660254037844387076, 1.000000000000000000, 0.8660254037844387076, 1.000000000000000000, 0.8660254037844387076, 1.000000000000000000, 0.8660254037844387076, 1.000000000000000000, 0.8660254037844387076, 1.000000000000000000, 0.8660254037844387076, 1.000000000000000000, 0.8660254037844387076, 1.000000000000000000, 0.8660254037844387076, 1.000000000000000000, 0.8660254037844387076, 1.000000000000000000, 0.8660254037844387076, 1.000000000000000000, 0.8660254037844387076, 1.000000000000000000, 0.8660254037844387076, 1.000000000000000000, 0.8660254037844387076, 1.000000000000000000, 0.8660254037844387076, 1.000000000000000000, 0.8660254037844387076, 1.000000000000000000, 0.8660254037844387076, 1.000000000000000000, 0.8660254037844387076, 1.000000000000000000, 0.8660254037844387076, 1.000000000000000000, 0.8660254037844387076, 1.000000000000000000, 0.8660254037844387076, 1.000000000000000000, 0.8660254037844387076, 1.000000000000000000, 0.8660254037844387076, 1.000000000000000000, 0.8660254037844387076, 1.000000000000000000, 0.8660254037844387076, 1.000000000000000000, 0.8660254037844387076, 1.000000000000000000, 0.8660254037844387076, 1.000000000000000000, 0.8660254037844387076, 1.000000000000000000, 0.8660254037844387076, 1.000000000000000000, 0.8660254037844387076, 1.000000000000000000, 0.8660254037844387076, 1.000000000000000000, 0.8660254037844387076, 1.000000000000000000, 0.8660254037844387076, 1.000000000000000000, 0.8660254037844387076, 1.000000000000000000, 0.8660254037844387076, 1.000000000000000000, 0.8660254037844387076, 1.000000000000000000, 0.8660254037844387076, 1.000000000000000000, 0.8660254037844387076, 1.000000000000000000, 0.8660254037844387076, 1.000000000000000000, 0.8660254037844387076, 1.000000000000000000, 0.8660254037844387076, 1.000000000000000000, 0.8660254037844387076, 1.000000000000000000, 0.8660254037844387076, 1.000000000000000000, 0.8660254037844387076, 1.000000000000000000, 0.8660254037844387076, 1.000000000000000000, 0.8660254037844387076, 1.000000000000000000, 0.8660254037844387076, 1.000000000000000000, 0.8660254037844387076, 1.000000000000000000, 0.8660254037844387076, 1.000000000000000000, 0.8660254037844387076, 1.000000000000000000, 0.8660254037844387076, 1.000000000000000000, 0.8660254037844387076, 1.000000000000000000, 0.8660254037844387076, 1.000000000000000000, 0.8660254037844387076, 1.000000000000000000, 0.8660254037844387076, 1.000000000000000000, 0.8660254037844387076, 1.000000000000000000, 0.8660254037844387076, 1.000000000000000000, 0.8660254037844387076, 1.000000000000000000, 0.8660254037844387076, 1.000000000000000000, 0.8660254037844387076, 1.000000000000000000, 0.8660254037844387076, 1.000000000000000000, 0.8660254037844387076, 1.000000000000000000, 0.8660254037844387076, 1.000000000000000000, 0.8660254037844387076, 1.000000000000000000, 0.8660254037844387076, 1.000000000000000000, 0.8660254037844387076, 1.000000000000000000, 0.8660254037844387076, 1.000000000000000000, 0.8660254037844387076, 1.000000000000000000, 0.8660254037844387076, 1.000000000000000000, 0.8660254037844387076, 1.000000000000000000, 0.8660254037844387076, 1.000000000000000000, 0.8660254037844387076, 1.000000000000000000, 0.8660254037844387076, 1.000000000000000000, 0.8660254037844387076, 1.000000000000000000, 0.8660254037844387076, 1.000000000000000000, 0.8660254037844387076, 1.000000000000000000, 0.8660254037844387076, 1.000000000000000000, 0.8660254037844387076, 1.000000000000000000, 0.8660254037844387076, 1.000000000000000000, 0.8660254037844387076, 1.000000000000000000, 0.8660254037844387076, 1.000000000000000000, 0.8660254037844387076, 1.000000000000000000, 0.8660254037844387076, 1.000000000000000000, 0.8660254037844387076, 1.000000000000000000, 0.8660254037844387076, 1.000000000000000000, 0.8660254037844387076, 1.000000000000000000, 0.8660254037844387076, 1.000000000000000000, 0.8660254037844387076, 1.000000000000000000, 0.8660254037844387076, 1.000000000000000000, 0.8660254037844387076, 1.000000000000000000, 0.8660254037844387076, 1.000000000000000000, 0.8660254037844387076, 1.000000000000000000, 0.8660254037844387076, 1.000000000000000000, 0.8660254037844387076, 1.000000000000000000, 0.8660254037844387076, 1.000000000000000000, 0.8660254037844387076, 1.000000000000000000, 0.8660254037844387076, 1.000000000000000000, 0.8660254037844387076, 1.000000000000000000, 0.8660254037844387076, 1.000000000000000000, 0.8660254037844387076, 1.000000000000000000, 0.8660254037844387076, 1.000000000000000000, 0.8660254037844387076, 1.000000000000000000, 0.8660254037844387076, 1.000000000000000000, 0.8660254037844387076, 1.000000000000000000, 0.8660254037844387076, 1.000000000000000000, 0.8660254037844387076, 1.000000000000000000, 0.8660254037844387076, 1.000000000000000000, 0.8660254037844387076, 1.000000000000000000, 0.8660254037844387076, 1.000000000000000000, 0.8660254037844387076, 1.000000000000000000, 0.8660254037844387076, 1.000000000000000000, 0.8660254037844387076, 1.000000000000000000, 0.8660254037844387076, 1.000000000000000000, 0.8660254037844387076, 1.000000000000000000, 0.8660254037844387076, 1.000000000000000000, 0.8660254037844387076, 1.000000000000000000, 0.8660254037844387076, 1.000000000000000000, 0.8660254037844387076, 1.000000000000000000, 0.8660254037844387076, 1.000000000000000000, 0.8660254037844387076, 1.000000000000000000, 0.8660254037844387076, 1.000000000000000000, 0.8660254037844387076, 1.000000000000000000, 0.8660254037844387076, 1.000000000000000000, 0.8660254037844387076, 1.000000000000000000, 0.8660254037844387076, 1.000000000000000000, 0.8660254037844387076, 1.000000000000000000, 0.8660254037844387076, 1.000000000000000000, 0.8660254037844387076, 1.000000000000000000, 0.8660254037844387076, 1.000000000000000000, 0.8660254037844387076, 1.000000000000000000, 0.8660254037844387076, 1.000000000000000000, 0.8660254037844387076, 1.000000000000000000, 0.8660254037844387076, 1.000000000000000000, 0.8660254037844387076, 1.000000000000000000, 0.8660254037844387076, 1.000000000000000000, 0.8660254037844387076, 1.000000000000000000, 0.8660254037844387076, 1.000000000000000000, 0.8660254037844387076, 1.000000000000000000, 0.8660254037844387076, 1.000000000000000000, 0.8660254037844387076, 1.000000000000000000, 0.8660254037844387076, 1.000000000000000000, 0.8660254037844387076, 1.000000000000000000, 0.8660254037844387076, 1.000000000000000000, 0.8660254037844387076, 1.000000000000000000, 0.8660254037844387076, 1.000000000000000000, 0.8660254037844387076, 1.000000000000000000, 0.8660254037844387076, 1.000000000000000000, 0.8660254037844387076, 1.000000000000000000, 0.8660254037844387076, 1.000000000000000000, 0.8660254037844387076, 1.000000000000000000, 0.8660254037844387076, 1.000000000000000000, 0.8660254037844387076, 1.000000000000000000, 0.8660254037844387076, 1.000000000000000000, 0.8660254037844387076, 1.000000000000000000, 0.8660254037844387076, 1.000000000000000000, 0.8660254037844387076, 1.000000000000000000, 0.8660254037844387076, 1.000000000000000000, 0.8660254037844387076, 1.000000000000000000, 0.8660254037844387076, 1.000000000000000000, 0.8660254037844387076, 1.000000000000000000, 0.8660254037844387076, 1.000000000000000000, 0.8660254037844387076, 1.000000000000000000, 0.8660254037844387076, 1.000000000000000000, 0.8660254037844387076, 1.000000000000000000, 0.8660254037844387076, 1.000000000000000000, 0.8660254037844387076, 1.000000000000000000, 0.8660254037844387076, 1.000000000000000000, 0.8660254037844387076, 1.000000000000000000, 0.8660254037844387076, 1.000000000000000000, 0.8660254037844387076, 1.000000000000000000, 0.8660254037844387076, 1.000000000000000000, 0.8660254037844387076, 1.000000000000000000, 0.8660254037844387076, 1.000000000000000000, 0.8660254037844387076, 1.000000000000000000, 0.8660254037844387076, 1.000000000000000000, 0.8660254037844387076, 1.000000000000000000, 0.8660254037844387076, 1.000000000000000000, 0.8660254037844387076, 1.000000000000000000, 0.8660254037844387076, 1.000000000000000000, 0.8660254037844387076, 1.000000000000000000, 0.8660254037844387076, 1.000000000000000000, 0.8660254037844387076, 1.000000000000000000, 0.8660254037844387076, 1.000000000000000000, 0.8660254037844387076, 1.000000000000000000, 0.8660254037844387076, 1.000000000000000000, 0.8660254037844387076, 1.000000000000000000, 0.8660254037844387076, 1.000000000000000000, 0.8660254037844387076, 1.000000000000000000, 0.8660254037844387076, 1.000000000000000000, 0.8660254037844387076, 1.000000000000000000, 0.8660254037844387076, 1.000000000000000000, 0.8660254037844387076, 1.000000000000000000, 0.8660254037844387076, 1.000000000000000000, 0.8660254037844387076, 1.000000000000000000, 0.8660254037844387076, 1.000000000000000000, 0.8660254037844387076, 1.000000000000000000, 0.8660254037844387076, 1.000000000000000000, 0.8660254037844387076, 1.000000000000000000, 0.8660254037844387076, 1.000000000000000000, 0.8660254037844387076, 1.000000000000000000, 0.8660254037844387076, 1.000000000000000000, 0.8660254037844387076, 1.000000000000000000, 0.8660254037844387076, 1.000000000000000000, 0.8660254037844387076, 1.000000000000000000, 0.8660254037844387076, 1.000000000000000000, 0.8660254037844387076, 1.000000000000000000, 0.8660254037844387076, 1.000000000000000000, 0.8660254037844387076, 1.000000000000000000, 0.8660254037844387076, 1.000000000000000000, 0.8660254037844387076, 1.000000000000000000, 0.8660254037844387076, 1.000000000000000000, 0.8660254037844387076, 1.000000000000000000, 0.8660254037844387076, 1.000000000000000000, 0.8660254037844387076, 1.000000000000000000, 0.8660254037844387076, 1.000000000000000000, 0.8660254037844387076, 1.000000000000000000, 0.8660254037844387076, 1.000000000000000000, 0.8660254037844387076, 1.000000000000000000, 0.8660254037844387076, 1.000000000000000000, 0.8660254037844387076, 1.000000000000000000, 0.8660254037844387076, 1.000000000000000000, 0.8660254037844387076, 1.000000000000000000, 0.8660254037844387076, 1.000000000000000000, 0.8660254037844387076, 1.000000000000000000, 0.8660254037844387076, 1.000000000000000000, 0.8660254037844387076, 1.000000000000000000, 0.8660254037844387076, 1.000000000000000000, 0.8660254037844387076, 1.000000000000000000, 0.8660254037844387076, 1.000000000000000000, 0.8660254037844387076, 1.000000000000000000, 0.8660254037844387076, 1.000000000000000000, 0.8660254037844387076, 1.000000000000000000, 0.8660254037844387076, 1.000000000000000000, 0.8660254037844387076, 1.000000000000000000, 0.8660254037844387076, 1.000000000000000000, 0.8660254037844387076, 1.000000000000000000, 0.8660254037844387076, 1.000000000000000000, 0.8660254037844387076, 1.000000000000000000, 0.8660254037844387076, 1.000000000000000000, 0.8660254037844387076, 1.000000000000000000, 0.8660254037844387076, 1.000000000000000000, 0.8660254037844387076, 1.000000000000000000, 0.8660254037844387076, 1.000000000000000000, 0.8660254037844387076, 1.000000000000000000, 0.8660254037844387076, 1.000000000000000000, 0.8660254037844387076, 1.000000000000000000, 0.8660254037844387076, 1.000000000000000000, 0.8660254037844387076, 1.000000000000000000, 0.8660254037844387076, 1.000000000000000000, 0.8660254037844387076, 1.000000000000000000, 0.8660254037844387076, 1.000000000000000000, 0.8660254037844387076, 1.000000000000000000, 0.8660254037844387076, 1.000000000000000000, 0.8660254037844387076, 1.000000000000000000, 0.8660254037844387076, 1.000000000000000000, 0.8660254037844387076, 1.000000000000000000, 0.8660254037844387076, 1.000000000000000000, 0.8660254037844387076, 1.000000000000000000, 0.8660254037844387076, 1.000000000000000000, 0.8660254037844387076, 1.000000000000000000, 0.8660254037844387076, 1.000000000000000000, 0.8660254037844387076, 1.000000000000000000, 0.8660254037844387076, 1.000000000000000000, 0.8660254037844387076, 1.000000000000000000, 0.8660254037844387076, 1.000000000000000000, 0.8660254037844387076, 1.000000000000000000, 0.8660254037844387076, 1.000000000000000000, 0.8660254037844387076, 1.000000000000000000, 0.8660254037844387076, 1.000000000000000000, 0.8660254037844387076, 1.000000000000000000, 0.8660254037844387076, 1.000000000000000000, 0.8660254037844387076, 1.000000000000000000, 0.8660254037844387076, 1.000000000000000000, 0.8660254037844387076, 1.000000000000000000, 0.8660254037844387076, 1.000000000000000000, 0.8660254037844387076, 1.000000000000000000, 0.8660254037844387076, 1.000000000000000000, 0.8660254037844387076, 1.000000000000000000, 0.8660254037844387076, 1.000000000000000000, 0.8660254037844387076, 1.000000000000000000, 0.8660254037844387076, 1.000000000000000000, 0.8660254037844387076, 1.000000000000000000, 0.8660254037844387076, 1.000000000000000000, 0.8660254037844387076, 1.000000000000000000, 0.8660254037844387076, 1.000000000000000000, 0.8660254037844387076, 1.000000000000000000, 0.8660254037844387076, 1.000000000000000000, 0.8660254037844387076, 1.000000000000000000, 0.8660254037844387076, 1.000000000000000000, 0.8660254037844387076, 1.000000000000000000, 0.8660254037844387076, 1.000000000000000000, 0.8660254037844387076, 1.000000000000000000, 0.8660254037844387076, 1.000000000000000000, 0.8660254037844387076, 1.000000000000000000, 0.8660254037844387076, 1.000000000000000000, 0.8660254037844387076, 1.000000000000000000, 0.8660254037844387076, 1.000000000000000000, 0.8660254037844387076, 1.000000000000000000, 0.8660254037844387076, 1.000000000000000000, 0.8660254037844387076, 1.000000000000000000, 0.8660254037844387076, 1.000000000000000000, 0.8660254037844387076, 1.000000000000000000, 0.8660254037844387076, 1.000000000000000000, 0.8660254037844387076, 1.000000000000000000, 0.8660254037844387076, 1.000000000000000000, 0.8660254037844387076, 1.000000000000000000, 0.8660254037844387076, 1.000000000000000000, 0.8660254037844387076, 1.000000000000000000, 0.8660254037844387076, 1.000000000000000000, 0.8660254037844387076, 1.000000000000000000, 0.8660254037844387076, 1.000000000000000000, 0.8660254037844387076, 1.000000000000000000, 0.8660254037844387076, 1.000000000000000000, 0.8660254037844387076, 1.000000000000000000, 0.8660254037844387076, 1.000000000000000000, 0.8660254037844387076, 1.000000000000000000, 0.8660254037844387076, 1.000000000000000000, 0.8660254037844387076, 1.000000000000000000, 0.8660254037844387076, 1.000000000000000000, 0.8660254037844387076, 1.000000000000000000, 0.8660254037844387076, 1.000000000000000000, 0.8660254037844387076, 1.000000000000000000, 0.8660254037844387076, 1.000000000000000000, 0.8660254037844387076, 1.000000000000000000, 0.8660254037844387076, 1.000000000000000000, 0.8660254037844387076, 1.000000000000000000, 0.8660254037844387076, 1.000000000000000000, 0.8660254037844387076, 1.000000000000000000, 0.8660254037844387076, 1.000000000000000000, 0.8660254037844387076, 1.000000000000000000, 0.8660254037844387076, 1.000000000000000000, 0.8660254037844387076, 1.000000000000000000, 0.8660254037844387076, 1.000000000000000000, 0.8660254037844387076, 1.000000000000000000, 0.8660254037844387076, 1.000000000000000000, 0.8660254037844387076, 1.000000000000000000, 0.8660254037844387076, 1.000000000000000000, 0.8660254037844387076, 1.000000000000000000, 0.8660254037844387076, 1.000000000000000000, 0.8660254037844387076, 1.000000000000000000, 0.8660254037844387076, 1.000000000000000000, 0.8660254037844387076, 1.000000000000000000, 0.8660254037844387076, 1.000000000000000000, 0.8660254037844387076, 1.000000000000000000, 0.8660254037844387076, 1.000000000000000000, 0.8660254037844387076, 1.000000000000000000, 0.8660254037844387076, 1.000000000000000000, 0.8660254037844387076, 1.000000000000000000, 0.8660254037844387076, 1.000000000000000000, 0.8660254037844387076, 1.000000000000000000, 0.8660254037844387076, 1.000000000000000000, 0.8660254037844387076, 1.000000000000000000, 0.8660254037844387076, 1.000000000000000000, 0.8660254037844387076, 1.000000000000000000, 0.8660254037844387076, 1.000000000000000000, 0.8660254037844387076, 1.000000000000000000, 0.8660254037844387076, 1.000000000000000000, 0.8660254037844387076, 1.000000000000000000, 0.8660254037844387076, 1.000000000000000000, 0.8660254037844387076, 1.000000000000000000, 0.8660254037844387076, 1.000000000000000000, 0.8660254037844387076, 1.000000000000000000, 0.8660254037844387076, 1.000000000000000000, 0.8660254037844387076, 1.000000000000000000, 0.8660254037844387076, 1.000000000000000000, 0.8660254037844387076, 1.000000000000000000, 0.8660254037844387076, 1.000000000000000000, 0.8660254037844387076, 1.000000000000000000, 0.8660254037844387076, 1.000000000000000000, 0.8660254037844387076, 1.000000000000000000, 0.8660254037844387076, 1.000000000000000000, 0.8660254037844387076, 1.000000000000000000, 0.8660254037844387076, 1.000000000000000000, 0.8660254037844387076, 1.000000000000000000, 0.8660254037844387076, 1.000000000000000000, 0.8660254037844387076, 1.000000000000000000, 0.8660254037844387076, 1.000000000000000000, 0.8660254037844387076, 1.000000000000000000, 0.8660254037844387076, 1.000000000000000000, 0.8660254037844387076, 1.000000000000000000, 0.8660254037844387076, 1.000000000000000000, 0.8660254037844387076, 1.000000000000000000, 0.8660254037844387076, 1.000000000000000000, 0.8660254037844387076, 1.000000000000000000, 0.8660254037844387076, 1.000000000000000000, 0.8660254037844387076, 1.000000000000000000, 0.8660254037844387076, 1.000000000000000000, 0.8660254037844387076, 1.000000000000000000, 0.8660254037844387076, 1.000000000000000000, 0.8660254037844387076, 1.000000000000000000, 0.8660254037844387076, 1.000000000000000000, 0.8660254037844387076, 1.000000000000000000, 0.8660254037844387076, 1.000000000000000000, 0.8660254037844387076, 1.000000000000000000, 0.8660254037844387076, 1.000000000000000000, 0.8660254037844387076, 1.000000000000000000, 0.8660254037844387076, 1.000000000000000000, 0.8660254037844387076, 1.000000000000000000, 0.8660254037844387076, 1.000000000000000000, 0.8660254037844387076, 1.000000000000000000, 0.8660254037844387076, 1.000000000000000000, 0.8660254037844387076, 1.000000000000000000, 0.8660254037844387076, 1.000000000000000000, 0.8660254037844387076, 1.000000000000000000, 0.8660254037844387076, 1.000000000000000000, 0.8660254037844387076, 1.000000000000000000, 0.8660254037844387076, 1.000000000000000000, 0.8660254037844387076, 1.000000000000000000, 0.8660254037844387076, 1.000000000000000000, 0.8660254037844387076, 1.000000000000000000, 0.8660254037844387076, 1.000000000000000000, 0.8660254037844387076, 1.000000000000000000, 0.8660254037844387076, 1.000000000000000000, 0.8660254037844387076, 1.000000000000000000, 0.8660254037844387076, 1.000000000000000000, 0.8660254037844387076, 1.000000000000000000, 0.8660254037844387076, 1.000000000000000000, 0.8660254037844387076, 1.000000000000000000, 0.8660254037844387076, 1.000000000000000000, 0.8660254037844387076, 1.000000000000000000, 0.8660254037844387076, 1.000000000000000000, 0.8660254037844387076, 1.000000000000000000, 0.8660254037844387076, 1.000000000000000000, 0.8660254037844387076, 1.000000000000000000, 0.8660254037844387076, 1.000000000000000000, 0.8660254037844387076, 1.000000000000000000, 0.8660254037844387076, 1.000000000000000000, 0.8660254037844387076, 1.000000000000000000, 0.8660254037844387076, 1.000000000000000000, 0.8660254037844387076, 1.000000000000000000, 0.8660254037844387076, 1.000000000000000000, 0.8660254037844387076, 1.000000000000000000, 0.8660254037844387076, 1.000000000000000000, 0.8660254037844387076, 1.000000000000000000, 0.8660254037844387076, 1.000000000000000000, 0.8660254037844387076, 1.000000000000000000, 0.8660254037844387076, 1.000000000000000000, 0.8660254037844387076, 1.000000000000000000, 0.8660254037844387076, 1.000000000000000000, 0.8660254037844387076, 1.000000000000000000, 0.8660254037844387076, 1.000000000000000000, 0.8660254037844387076, 1.000000000000000000, 0.8660254037844387076, 1.000000000000000000, 0.8660254037844387076, 1.000000000000000000, 0.8660254037844387076, 1.000000000000000000, 0.8660254037844387076, 1.000000000000000000, 0.8660254037844387076, 1.000000000000000000, 0.8660254037844387076, 1.000000000000000000, 0.8660254037844387076, 1.000000000000000000, 0.8660254037844387076, 1.000000000000000000, 0.8660254037844387076, 1.000000000000000000, 0.8660254037844387076, 1.000000000000000000, 0.8660254037844387076, 1.000000000000000000, 0.8660254037844387076, 1.000000000000000000, 0.8660254037844387076, 1.000000000000000000, 0.8660254037844387076, 1.000000000000000000, 0.8660254037844387076, 1.000000000000000000, 0.8660254037844387076, 1.000000000000000000, 0.8660254037844387076, 1.000000000000000000, 0.8660254037844387076, 1.000000000000000000, 0.8660254037844387076, 1.000000000000000000, 0.8660254037844387076, 1.000000000000000000, 0.8660254037844387076, 1.000000000000000000, 0.8660254037844387076, 1.000000000000000000, 0.8660254037844387076, 1.000000000000000000, 0.8660254037844387076, 1.000000000000000000, 0.8660254037844387076, 1.000000000000000000, 0.8660254037844387076, 1.000000000000000000, 0.8660254037844387076, 1.000000000000000000, 0.8660254037844387076, 1.000000000000000000, 0.8660254037844387076, 1.000000000000000000, 0.8660254037844387076, 1.000000000000000000, 0.8660254037844387076, 1.000000000000000000, 0.8660254037844387076, 1.000000000000000000, 0.8660254037844387076, 1.000000000000000000, 0.8660254037844387076, 1.000000000000000000, 0.8660254037844387076, 1.000000000000000000, 0.8660254037844387076, 1.000000000000000000, 0.8660254037844387076, 1.000000000000000000, 0.8660254037844387076, 1.000000000000000000, 0.8660254037844387076, 1.000000000000000000, 0.8660254037844387076, 1.000000000000000000, 0.8660254037844387076, 1.000000000000000000, 0.8660254037844387076, 1.000000000000000000, 0.8660254037844387076, 1.000000000000000000, 0.8660254037844387076, 1.000000000000000000, 0.8660254037844387076, 1.000000000000000000, 0.8660254037844387076, 1.000000000000000000, 0.8660254037844387076, 1.000000000000000000, 0.8660254037844387076, 1.000000000000000000, 0.8660254037844387076, 1.000000000000000000, 0.8660254037844387076, 1.000000000000000000, 0.8660254037844387076, 1.000000000000000000, 0.8660254037844387076, 1.000000000000000000, 0.8660254037844387076, 1.000000000000000000, 0.8660254037844387076, 1.000000000000000000, 0.8660254037844387076, 1.000000000000000000, 0.8660254037844387076, 1.000000000000000000, 0.8660254037844387076, 1.000000000000000000, 0.8660254037844387076, 1.000000000000000000, 0.8660254037844387076, 1.000000000000000000, 0.8660254037844387076, 1.000000000000000000, 0.8660254037844387076, 1.000000000000000000, 0.8660254037844387076, 1.000000000000000000, 0.8660254037844387076, 1.000000000000000000, 0.8660254037844387076, 1.000000000000000000, 0.8660254037844387076, 1.000000000000000000, 0.8660254037844387076, 1.000000000000000000, 0.8660254037844387076, 1.000000000000000000, 0.8660254037844387076, 1.000000000000000000, 0.8660254037844387076, 1.000000000000000000, 0.8660254037844387076, 1.000000000000000000, 0.8660254037844387076, 1.000000000000000000, 0.8660254037844387076, 1.000000000000000000, 0.8660254037844387076, 1.000000000000000000),
 ( 1.000000000000000000, 0.8660254037844387076, 1.000000000000000000, 0.8660254037844387076, 1.000000000000000000, 0.8660254037844387076, 1.000000000000000000, 0.8660254037844387076, 1.000000000000000000, 0.8660254037844387076, 1.000000000000000000, 0.8660254037844387076, 1.000000000000000000, 0.8660254037844387076, 1.000000000000000000, 0.8660254037844387076, 1.000000000000000000, 0.8660254037844387076, 1.000000000000000000, 0.8660254037844387076, 1.000000000000000000, 0.8660254037844387076, 1.000000000000000000, 0.8660254037844387076, 1.000000000000000000, 0.8660254037844387076, 1.000000000000000000, 0.8660254037844387076, 1.000000000000000000, 0.8660254037844387076, 1.000000000000000000, 0.8660254037844387076, 1.000000000000000000, 0.8660254037844387076, 1.000000000000000000, 0.8660254037844387076, 1.000000000000000000, 0.8660254037844387076, 1.000000000000000000, 0.8660254037844387076, 1.000000000000000000, 0.8660254037844387076, 1.000000000000000000, 0.8660254037844387076, 1.000000000000000000, 0.8660254037844387076, 1.000000000000000000, 0.8660254037844387076, 1.000000000000000000, 0.8660254037844387076, 1.000000000000000000, 0.8660254037844387076, 1.000000000000000000, 0.8660254037844387076, 1.000000000000000000, 0.8660254037844387076, 1.000000000000000000, 0.8660254037844387076, 1.000000000000000000, 0.8660254037844387076, 1.000000000000000000, 0.8660254037844387076, 1.000000000000000000, 0.8660254037844387076, 1.000000000000000000, 0.8660254037844387076, 1.000000000000000000, 0.8660254037844387076, 1.000000000000000000, 0.8660254037844387076, 1.000000000000000000, 0.8660254037844387076, 1.000000000000000000, 0.8660254037844387076, 1.000000000000000000, 0.8660254037844387076, 1.000000000000000000, 0.8660254037844387076, 1.000000000000000000, 0.8660254037844387076, 1.000000000000000000, 0.8660254037844387076, 1.000000000000000000, 0.8660254037844387076, 1.000000000000000000, 0.8660254037844387076, 1.000000000000000000, 0.8660254037844387076, 1.000000000000000000, 0.8660254037844387076, 1.000000000000000000, 0.8660254037844387076, 1.000000000000000000, 0.8660254037844387076, 1.000000000000000000, 0.8660254037844387076, 1.000000000000000000, 0.8660254037844387076, 1.000000000000000000, 0.8660254037844387076, 1.000000000000000000, 0.8660254037844387076, 1.000000000000000000, 0.8660254037844387076, 1.000000000000000000, 0.8660254037844387076, 1.000000000000000000, 0.8660254037844387076, 1.000000000000000000, 0.8660254037844387076, 1.000000000000000000, 0.8660254037844387076, 1.000000000000000000, 0.8660254037844387076, 1.000000000000000000, 0.8660254037844387076, 1.000000000000000000, 0.8660254037844387076, 1.000000000000000000, 0.8660254037844387076, 1.000000000000000000, 0.8660254037844387076, 1.000000000000000000, 0.8660254037844387076, 1.000000000000000000, 0.8660254037844387076, 1.000000000000000000, 0.8660254037844387076, 1.000000000000000000, 0.8660254037844387076, 1.000000000000000000, 0.8660254037844387076, 1.000000000000000000, 0.8660254037844387076, 1.000000000000000000, 0.8660254037844387076, 1.000000000000000000, 0.8660254037844387076, 1.000000000000000000, 0.8660254037844387076, 1.000000000000000000, 0.8660254037844387076, 1.000000000000000000, 0.8660254037844387076, 1.000000000000000000, 0.8660254037844387076, 1.000000000000000000, 0.8660254037844387076, 1.000000000000000000, 0.8660254037844387076, 1.000000000000000000, 0.8660254037844387076, 1.000000000000000000, 0.8660254037844387076, 1.000000000000000000, 0.8660254037844387076, 1.000000000000000000, 0.8660254037844387076, 1.000000000000000000, 0.8660254037844387076, 1.000000000000000000, 0.8660254037844387076, 1.000000000000000000, 0.8660254037844387076, 1.000000000000000000, 0.8660254037844387076, 1.000000000000000000, 0.8660254037844387076, 1.000000000000000000, 0.8660254037844387076, 1.000000000000000000, 0.8660254037844387076, 1.000000000000000000, 0.8660254037844387076, 1.000000000000000000, 0.8660254037844387076, 1.000000000000000000, 0.8660254037844387076, 1.000000000000000000, 0.8660254037844387076, 1.000000000000000000, 0.8660254037844387076, 1.000000000000000000, 0.8660254037844387076, 1.000000000000000000, 0.8660254037844387076, 1.000000000000000000, 0.8660254037844387076, 1.000000000000000000, 0.8660254037844387076, 1.000000000000000000, 0.8660254037844387076, 1.000000000000000000, 0.8660254037844387076, 1.000000000000000000, 0.8660254037844387076, 1.000000000000000000, 0.8660254037844387076, 1.000000000000000000, 0.8660254037844387076, 1.000000000000000000, 0.8660254037844387076, 1.000000000000000000, 0.8660254037844387076, 1.000000000000000000, 0.8660254037844387076, 1.000000000000000000, 0.8660254037844387076, 1.000000000000000000, 0.8660254037844387076, 1.000000000000000000, 0.8660254037844387076, 1.000000000000000000, 0.8660254037844387076, 1.000000000000000000, 0.8660254037844387076, 1.000000000000000000, 0.8660254037844387076, 1.000000000000000000, 0.8660254037844387076, 1.000000000000000000, 0.8660254037844387076, 1.000000000000000000, 0.8660254037844387076, 1.000000000000000000, 0.8660254037844387076, 1.000000000000000000, 0.8660254037844387076, 1.000000000000000000, 0.8660254037844387076, 1.000000000000000000, 0.8660254037844387076, 1.000000000000000000, 0.8660254037844387076, 1.000000000000000000, 0.8660254037844387076, 1.000000000000000000, 0.8660254037844387076, 1.000000000000000000, 0.8660254037844387076, 1.000000000000000000, 0.8660254037844387076, 1.000000000000000000, 0.8660254037844387076, 1.000000000000000000, 0.8660254037844387076, 1.000000000000000000, 0.8660254037844387076, 1.000000000000000000, 0.8660254037844387076, 1.000000000000000000, 0.8660254037844387076, 1.000000000000000000, 0.8660254037844387076, 1.000000000000000000, 0.8660254037844387076, 1.000000000000000000, 0.8660254037844387076, 1.000000000000000000, 0.8660254037844387076, 1.000000000000000000, 0.8660254037844387076, 1.000000000000000000, 0.8660254037844387076, 1.000000000000000000, 0.8660254037844387076, 1.000000000000000000, 0.8660254037844387076, 1.000000000000000000, 0.8660254037844387076, 1.000000000000000000, 0.8660254037844387076, 1.000000000000000000, 0.8660254037844387076, 1.000000000000000000, 0.8660254037844387076, 1.000000000000000000, 0.8660254037844387076, 1.000000000000000000, 0.8660254037844387076, 1.000000000000000000, 0.8660254037844387076, 1.000000000000000000, 0.8660254037844387076, 1.000000000000000000, 0.8660254037844387076, 1.000000000000000000, 0.8660254037844387076, 1.000000000000000000, 0.8660254037844387076, 1.000000000000000000, 0.8660254037844387076, 1.000000000000000000, 0.8660254037844387076, 1.000000000000000000, 0.8660254037844387076, 1.000000000000000000, 0.8660254037844387076, 1.000000000000000000, 0.8660254037844387076, 1.000000000000000000, 0.8660254037844387076, 1.000000000000000000, 0.8660254037844387076, 1.000000000000000000, 0.8660254037844387076, 1.000000000000000000, 0.8660254037844387076, 1.000000000000000000, 0.8660254037844387076, 1.000000000000000000, 0.8660254037844387076, 1.000000000000000000, 0.8660254037844387076, 1.000000000000000000, 0.8660254037844387076, 1.000000000000000000, 0.8660254037844387076, 1.000000000000000000, 0.8660254037844387076, 1.000000000000000000, 0.8660254037844387076, 1.000000000000000000, 0.8660254037844387076, 1.000000000000000000, 0.8660254037844387076, 1.000000000000000000, 0.8660254037844387076, 1.000000000000000000, 0.8660254037844387076, 1.000000000000000000, 0.8660254037844387076, 1.000000000000000000, 0.8660254037844387076, 1.000000000000000000, 0.8660254037844387076, 1.000000000000000000, 0.8660254037844387076, 1.000000000000000000, 0.8660254037844387076, 1.000000000000000000, 0.8660254037844387076, 1.000000000000000000, 0.8660254037844387076, 1.000000000000000000, 0.8660254037844387076, 1.000000000000000000, 0.8660254037844387076, 1.000000000000000000, 0.8660254037844387076, 1.000000000000000000, 0.8660254037844387076, 1.000000000000000000, 0.8660254037844387076, 1.000000000000000000, 0.8660254037844387076, 1.000000000000000000, 0.8660254037844387076, 1.000000000000000000, 0.8660254037844387076, 1.000000000000000000, 0.8660254037844387076, 1.000000000000000000, 0.8660254037844387076, 1.000000000000000000, 0.8660254037844387076, 1.000000000000000000, 0.8660254037844387076, 1.000000000000000000, 0.8660254037844387076, 1.000000000000000000, 0.8660254037844387076, 1.000000000000000000, 0.8660254037844387076, 1.000000000000000000, 0.8660254037844387076, 1.000000000000000000, 0.8660254037844387076, 1.000000000000000000, 0.8660254037844387076, 1.000000000000000000, 0.8660254037844387076, 1.000000000000000000, 0.8660254037844387076, 1.000000000000000000, 0.8660254037844387076, 1.000000000000000000, 0.8660254037844387076, 1.000000000000000000, 0.8660254037844387076, 1.000000000000000000, 0.8660254037844387076, 1.000000000000000000, 0.8660254037844387076, 1.000000000000000000, 0.8660254037844387076, 1.000000000000000000, 0.8660254037844387076, 1.000000000000000000, 0.8660254037844387076, 1.000000000000000000, 0.8660254037844387076, 1.000000000000000000, 0.8660254037844387076, 1.000000000000000000, 0.8660254037844387076, 1.000000000000000000, 0.8660254037844387076, 1.000000000000000000, 0.8660254037844387076, 1.000000000000000000, 0.8660254037844387076, 1.000000000000000000, 0.8660254037844387076, 1.000000000000000000, 0.8660254037844387076, 1.000000000000000000, 0.8660254037844387076, 1.000000000000000000, 0.8660254037844387076, 1.000000000000000000, 0.8660254037844387076, 1.000000000000000000, 0.8660254037844387076, 1.000000000000000000, 0.8660254037844387076, 1.000000000000000000, 0.8660254037844387076, 1.000000000000000000, 0.8660254037844387076, 1.000000000000000000, 0.8660254037844387076, 1.000000000000000000, 0.8660254037844387076, 1.000000000000000000, 0.8660254037844387076, 1.000000000000000000, 0.8660254037844387076, 1.000000000000000000, 0.8660254037844387076, 1.000000000000000000, 0.8660254037844387076, 1.000000000000000000, 0.8660254037844387076, 1.000000000000000000, 0.8660254037844387076, 1.000000000000000000, 0.8660254037844387076, 1.000000000000000000, 0.8660254037844387076, 1.000000000000000000, 0.8660254037844387076, 1.000000000000000000, 0.8660254037844387076, 1.000000000000000000, 0.8660254037844387076, 1.000000000000000000, 0.8660254037844387076, 1.000000000000000000, 0.8660254037844387076, 1.000000000000000000, 0.8660254037844387076, 1.000000000000000000, 0.8660254037844387076, 1.000000000000000000, 0.8660254037844387076, 1.000000000000000000, 0.8660254037844387076, 1.000000000000000000, 0.8660254037844387076, 1.000000000000000000, 0.8660254037844387076, 1.000000000000000000, 0.8660254037844387076, 1.000000000000000000, 0.8660254037844387076, 1.000000000000000000, 0.8660254037844387076, 1.000000000000000000, 0.8660254037844387076, 1.000000000000000000, 0.8660254037844387076, 1.000000000000000000, 0.8660254037844387076, 1.000000000000000000, 0.8660254037844387076, 1.000000000000000000, 0.8660254037844387076, 1.000000000000000000, 0.8660254037844387076, 1.000000000000000000, 0.8660254037844387076, 1.000000000000000000, 0.8660254037844387076, 1.000000000000000000, 0.8660254037844387076, 1.000000000000000000, 0.8660254037844387076, 1.000000000000000000, 0.8660254037844387076, 1.000000000000000000, 0.8660254037844387076, 1.000000000000000000, 0.8660254037844387076, 1.000000000000000000, 0.8660254037844387076, 1.000000000000000000, 0.8660254037844387076, 1.000000000000000000, 0.8660254037844387076, 1.000000000000000000, 0.8660254037844387076, 1.000000000000000000, 0.8660254037844387076, 1.000000000000000000, 0.8660254037844387076, 1.000000000000000000, 0.8660254037844387076, 1.000000000000000000, 0.8660254037844387076, 1.000000000000000000, 0.8660254037844387076, 1.000000000000000000, 0.8660254037844387076, 1.000000000000000000, 0.8660254037844387076, 1.000000000000000000, 0.8660254037844387076, 1.000000000000000000, 0.8660254037844387076, 1.000000000000000000, 0.8660254037844387076, 1.000000000000000000, 0.8660254037844387076, 1.000000000000000000, 0.8660254037844387076, 1.000000000000000000, 0.8660254037844387076, 1.000000000000000000, 0.8660254037844387076, 1.000000000000000000, 0.8660254037844387076, 1.000000000000000000, 0.8660254037844387076, 1.000000000000000000, 0.8660254037844387076, 1.000000000000000000, 0.8660254037844387076, 1.000000000000000000, 0.8660254037844387076, 1.000000000000000000, 0.8660254037844387076, 1.000000000000000000, 0.8660254037844387076, 1.000000000000000000, 0.8660254037844387076, 1.000000000000000000, 0.8660254037844387076, 1.000000000000000000, 0.8660254037844387076, 1.000000000000000000, 0.8660254037844387076, 1.000000000000000000, 0.8660254037844387076, 1.000000000000000000, 0.8660254037844387076, 1.000000000000000000, 0.8660254037844387076, 1.000000000000000000, 0.8660254037844387076, 1.000000000000000000, 0.8660254037844387076, 1.000000000000000000, 0.8660254037844387076, 1.000000000000000000, 0.8660254037844387076, 1.000000000000000000, 0.8660254037844387076, 1.000000000000000000, 0.8660254037844387076, 1.000000000000000000, 0.8660254037844387076, 1.000000000000000000, 0.8660254037844387076, 1.000000000000000000, 0.8660254037844387076, 1.000000000000000000, 0.8660254037844387076, 1.000000000000000000, 0.8660254037844387076, 1.000000000000000000, 0.8660254037844387076, 1.000000000000000000, 0.8660254037844387076, 1.000000000000000000, 0.8660254037844387076, 1.000000000000000000, 0.8660254037844387076, 1.000000000000000000, 0.8660254037844387076, 1.000000000000000000, 0.8660254037844387076, 1.000000000000000000, 0.8660254037844387076, 1.000000000000000000, 0.8660254037844387076, 1.000000000000000000, 0.8660254037844387076, 1.000000000000000000, 0.8660254037844387076, 1.000000000000000000, 0.8660254037844387076, 1.000000000000000000, 0.8660254037844387076, 1.000000000000000000, 0.8660254037844387076, 1.000000000000000000, 0.8660254037844387076, 1.000000000000000000, 0.8660254037844387076, 1.000000000000000000, 0.8660254037844387076, 1.000000000000000000, 0.8660254037844387076, 1.000000000000000000, 0.8660254037844387076, 1.000000000000000000, 0.8660254037844387076, 1.000000000000000000, 0.8660254037844387076, 1.000000000000000000, 0.8660254037844387076, 1.000000000000000000, 0.8660254037844387076, 1.000000000000000000, 0.8660254037844387076, 1.000000000000000000, 0.8660254037844387076, 1.000000000000000000, 0.8660254037844387076, 1.000000000000000000, 0.8660254037844387076, 1.000000000000000000, 0.8660254037844387076, 1.000000000000000000, 0.8660254037844387076, 1.000000000000000000, 0.8660254037844387076, 1.000000000000000000, 0.8660254037844387076, 1.000000000000000000, 0.8660254037844387076, 1.000000000000000000, 0.8660254037844387076, 1.000000000000000000, 0.8660254037844387076, 1.000000000000000000, 0.8660254037844387076, 1.000000000000000000, 0.8660254037844387076, 1.000000000000000000, 0.8660254037844387076, 1.000000000000000000, 0.8660254037844387076, 1.000000000000000000, 0.8660254037844387076, 1.000000000000000000, 0.8660254037844387076, 1.000000000000000000, 0.8660254037844387076, 1.000000000000000000, 0.8660254037844387076, 1.000000000000000000, 0.8660254037844387076, 1.000000000000000000, 0.8660254037844387076, 1.000000000000000000, 0.8660254037844387076, 1.000000000000000000, 0.8660254037844387076, 1.000000000000000000, 0.8660254037844387076, 1.000000000000000000, 0.8660254037844387076, 1.000000000000000000, 0.8660254037844387076, 1.000000000000000000, 0.8660254037844387076, 1.000000000000000000, 0.8660254037844387076, 1.000000000000000000, 0.8660254037844387076, 1.000000000000000000, 0.8660254037844387076, 1.000000000000000000, 0.8660254037844387076, 1.000000000000000000, 0.8660254037844387076, 1.000000000000000000, 0.8660254037844387076, 1.000000000000000000, 0.8660254037844387076, 1.000000000000000000, 0.8660254037844387076, 1.000000000000000000, 0.8660254037844387076, 1.000000000000000000, 0.8660254037844387076, 1.000000000000000000, 0.8660254037844387076, 1.000000000000000000, 0.8660254037844387076, 1.000000000000000000, 0.8660254037844387076, 1.000000000000000000, 0.8660254037844387076, 1.000000000000000000, 0.8660254037844387076, 1.000000000000000000, 0.8660254037844387076, 1.000000000000000000, 0.8660254037844387076, 1.000000000000000000, 0.8660254037844387076, 1.000000000000000000, 0.8660254037844387076, 1.000000000000000000, 0.8660254037844387076, 1.000000000000000000, 0.8660254037844387076, 1.000000000000000000, 0.8660254037844387076, 1.000000000000000000, 0.8660254037844387076, 1.000000000000000000, 0.8660254037844387076, 1.000000000000000000, 0.8660254037844387076, 1.000000000000000000, 0.8660254037844387076, 1.000000000000000000, 0.8660254037844387076, 1.000000000000000000, 0.8660254037844387076, 1.000000000000000000, 0.8660254037844387076, 1.000000000000000000, 0.8660254037844387076, 1.000000000000000000, 0.8660254037844387076, 1.000000000000000000, 0.8660254037844387076, 1.000000000000000000, 0.8660254037844387076, 1.000000000000000000, 0.8660254037844387076, 1.000000000000000000, 0.8660254037844387076, 1.000000000000000000, 0.8660254037844387076, 1.000000000000000000, 0.8660254037844387076, 1.000000000000000000, 0.8660254037844387076, 1.000000000000000000, 0.8660254037844387076, 1.000000000000000000, 0.8660254037844387076, 1.000000000000000000, 0.8660254037844387076, 1.000000000000000000, 0.8660254037844387076, 1.000000000000000000, 0.8660254037844387076, 1.000000000000000000, 0.8660254037844387076, 1.000000000000000000, 0.8660254037844387076, 1.000000000000000000, 0.8660254037844387076, 1.000000000000000000, 0.8660254037844387076, 1.000000000000000000, 0.8660254037844387076, 1.000000000000000000, 0.8660254037844387076, 1.000000000000000000, 0.8660254037844387076, 1.000000000000000000, 0.8660254037844387076, 1.000000000000000000, 0.8660254037844387076, 1.000000000000000000, 0.8660254037844387076, 1.000000000000000000, 0.8660254037844387076, 1.000000000000000000, 0.8660254037844387076, 1.000000000000000000, 0.8660254037844387076, 1.000000000000000000, 0.8660254037844387076, 1.000000000000000000, 0.8660254037844387076, 1.000000000000000000, 0.8660254037844387076, 1.000000000000000000, 0.8660254037844387076, 1.000000000000000000, 0.8660254037844387076, 1.000000000000000000, 0.8660254037844387076, 1.000000000000000000, 0.8660254037844387076, 1.000000000000000000, 0.8660254037844387076, 1.000000000000000000, 0.8660254037844387076, 1.000000000000000000, 0.8660254037844387076, 1.000000000000000000, 0.8660254037844387076, 1.000000000000000000, 0.8660254037844387076, 1.000000000000000000, 0.8660254037844387076, 1.000000000000000000, 0.8660254037844387076, 1.000000000000000000, 0.8660254037844387076, 1.000000000000000000, 0.8660254037844387076, 1.000000000000000000, 0.8660254037844387076, 1.000000000000000000, 0.8660254037844387076, 1.000000000000000000, 0.8660254037844387076, 1.000000000000000000, 0.8660254037844387076, 1.000000000000000000, 0.8660254037844387076, 1.000000000000000000, 0.8660254037844387076, 1.000000000000000000, 0.8660254037844387076, 1.000000000000000000, 0.8660254037844387076, 1.000000000000000000, 0.8660254037844387076, 1.000000000000000000, 0.8660254037844387076, 1.000000000000000000, 0.8660254037844387076, 1.000000000000000000, 0.8660254037844387076, 1.000000000000000000, 0.8660254037844387076, 1.000000000000000000, 0.8660254037844387076, 1.000000000000000000, 0.8660254037844387076, 1.000000000000000000, 0.8660254037844387076, 1.000000000000000000, 0.8660254037844387076, 1.000000000000000000, 0.8660254037844387076, 1.000000000000000000, 0.8660254037844387076, 1.000000000000000000, 0.8660254037844387076, 1.000000000000000000, 0.8660254037844387076, 1.000000000000000000, 0.8660254037844387076, 1.000000000000000000, 0.8660254037844387076, 1.000000000000000000, 0.8660254037844387076, 1.000000000000000000, 0.8660254037844387076, 1.000000000000000000, 0.8660254037844387076, 1.000000000000000000, 0.8660254037844387076, 1.000000000000000000, 0.8660254037844387076, 1.000000000000000000, 0.8660254037844387076, 1.000000000000000000, 0.8660254037844387076, 1.000000000000000000, 0.8660254037844387076, 1.000000000000000000, 0.8660254037844387076, 1.000000000000000000, 0.8660254037844387076, 1.000000000000000000, 0.8660254037844387076, 1.000000000000000000, 0.8660254037844387076, 1.000000000000000000, 0.8660254037844387076, 1.000000000000000000, 0.8660254037844387076, 1.000000000000000000, 0.8660254037844387076, 1.000000000000000000, 0.8660254037844387076, 1.000000000000000000, 0.8660254037844387076, 1.000000000000000000, 0.8660254037844387076, 1.000000000000000000, 0.8660254037844387076, 1.000000000000000000, 0.8660254037844387076, 1.000000000000000000, 0.8660254037844387076, 1.000000000000000000, 0.8660254037844387076, 1.000000000000000000, 0.8660254037844387076, 1.000000000000000000, 0.8660254037844387076, 1.000000000000000000, 0.8660254037844387076, 1.000000000000000000, 0.8660254037844387076, 1.000000000000000000, 0.8660254037844387076, 1.000000000000000000, 0.8660254037844387076, 1.000000000000000000, 0.8660254037844387076, 1.000000000000000000, 0.8660254037844387076, 1.000000000000000000, 0.8660254037844387076, 1.000000000000000000, 0.8660254037844387076, 1.000000000000000000, 0.8660254037844387076, 1.000000000000000000, 0.8660254037844387076, 1.000000000000000000, 0.8660254037844387076, 1.000000000000000000, 0.8660254037844387076, 1.000000000000000000, 0.8660254037844387076, 1.000000000000000000, 0.8660254037844387076, 1.000000000000000000, 0.8660254037844387076, 1.000000000000000000, 0.8660254037844387076, 1.000000000000000000, 0.8660254037844387076, 1.000000000000000000, 0.8660254037844387076, 1.000000000000000000, 0.8660254037844387076, 1.000000000000000000, 0.8660254037844387076, 1.000000000000000000, 0.8660254037844387076, 1.000000000000000000, 0.8660254037844387076, 1.000000000000000000, 0.8660254037844387076, 1.000000000000000000, 0.8660254037844387076, 1.000000000000000000, 0.8660254037844387076, 1.000000000000000000, 0.8660254037844387076, 1.000000000000000000, 0.8660254037844387076, 1.000000000000000000, 0.8660254037844387076, 1.000000000000000000, 0.8660254037844387076, 1.000000000000000000, 0.8660254037844387076, 1.000000000000000000, 0.8660254037844387076, 1.000000000000000000, 0.8660254037844387076, 1.000000000000000000, 0.8660254037844387076, 1.000000000000000000, 0.8660254037844387076, 1.000000000000000000, 0.8660254037844387076, 1.000000000000000000, 0.8660254037844387076, 1.000000000000000000, 0.8660254037844387076, 1.000000000000000000, 0.8660254037844387076, 1.000000000000000000, 0.8660254037844387076, 1.000000000000000000, 0.8660254037844387076, 1.000000000000000000, 0.8660254037844387076, 1.000000000000000000, 0.8660254037844387076, 1.000000000000000000, 0.8660254037844387076, 1.000000000000000000, 0.8660254037844387076, 1.000000000000000000, 0.8660254037844387076, 1.000000000000000000, 0.8660254037844387076, 1.000000000000000000, 0.8660254037844387076, 1.000000000000000000, 0.8660254037844387076, 1.000000000000000000, 0.8660254037844387076, 1.000000000000000000, 0.8660254037844387076, 1.000000000000000000, 0.8660254037844387076, 1.000000000000000000, 0.8660254037844387076, 1.000000000000000000, 0.8660254037844387076, 1.000000000000000000, 0.8660254037844387076, 1.000000000000000000, 0.8660254037844387076, 1.000000000000000000, 0.8660254037844387076, 1.000000000000000000, 0.8660254037844387076, 1.000000000000000000, 0.8660254037844387076, 1.000000000000000000, 0.8660254037844387076, 1.000000000000000000, 0.8660254037844387076, 1.000000000000000000, 0.8660254037844387076, 1.000000000000000000, 0.8660254037844387076, 1.000000000000000000, 0.8660254037844387076, 1.000000000000000000, 0.8660254037844387076, 1.000000000000000000, 0.8660254037844387076, 1.000000000000000000, 0.8660254037844387076, 1.000000000000000000, 0.8660254037844387076, 1.000000000000000000, 0.8660254037844387076, 1.000000000000000000, 0.8660254037844387076, 1.000000000000000000, 0.8660254037844387076, 1.000000000000000000, 0.8660254037844387076, 1.000000000000000000, 0.8660254037844387076, 1.000000000000000000, 0.8660254037844387076, 1.000000000000000000, 0.8660254037844387076, 1.000000000000000000, 0.8660254037844387076, 1.000000000000000000, 0.8660254037844387076, 1.000000000000000000, 0.8660254037844387076, 1.000000000000000000, 0.8660254037844387076, 1.000000000000000000, 0.8660254037844387076, 1.000000000000000000, 0.8660254037844387076, 1.000000000000000000, 0.8660254037844387076, 1.000000000000000000, 0.8660254037844387076, 1.000000000000000000, 0.8660254037844387076, 1.000000000000000000, 0.8660254037844387076, 1.000000000000000000, 0.8660254037844387076, 1.000000000000000000, 0.8660254037844387076, 1.000000000000000000, 0.8660254037844387076, 1.000000000000000000, 0.8660254037844387076, 1.000000000000000000, 0.8660254037844387076, 1.000000000000000000, 0.8660254037844387076, 1.000000000000000000, 0.8660254037844387076, 1.000000000000000000, 0.8660254037844387076, 1.000000000000000000, 0.8660254037844387076, 1.000000000000000000, 0.8660254037844387076, 1.000000000000000000, 0.8660254037844387076, 1.000000000000000000, 0.8660254037844387076, 1.000000000000000000, 0.8660254037844387076, 1.000000000000000000, 0.8660254037844387076, 1.000000000000000000, 0.8660254037844387076, 1.000000000000000000, 0.8660254037844387076, 1.000000000000000000, 0.8660254037844387076, 1.000000000000000000, 0.8660254037844387076, 1.000000000000000000, 0.8660254037844387076, 1.000000000000000000, 0.8660254037844387076, 1.000000000000000000, 0.8660254037844387076, 1.000000000000000000, 0.8660254037844387076, 1.000000000000000000, 0.8660254037844387076, 1.000000000000000000, 0.8660254037844387076, 1.000000000000000000, 0.8660254037844387076, 1.000000000000000000, 0.8660254037844387076, 1.000000000000000000, 0.8660254037844387076, 1.000000000000000000, 0.8660254037844387076, 1.000000000000000000, 0.8660254037844387076, 1.000000000000000000, 0.8660254037844387076, 1.000000000000000000, 0.8660254037844387076, 1.000000000000000000, 0.8660254037844387076, 1.000000000000000000, 0.8660254037844387076, 1.000000000000000000, 0.8660254037844387076, 1.000000000000000000, 0.8660254037844387076, 1.000000000000000000, 0.8660254037844387076, 1.000000000000000000, 0.8660254037844387076, 1.000000000000000000, 0.8660254037844387076, 1.000000000000000000, 0.8660254037844387076, 1.000000000000000000, 0.8660254037844387076, 1.000000000000000000, 0.8660254037844387076, 1.000000000000000000, 0.8660254037844387076, 1.000000000000000000, 0.8660254037844387076, 1.000000000000000000, 0.8660254037844387076, 1.000000000000000000, 0.8660254037844387076, 1.000000000000000000, 0.8660254037844387076, 1.000000000000000000, 0.8660254037844387076, 1.000000000000000000, 0.8660254037844387076, 1.000000000000000000, 0.8660254037844387076, 1.000000000000000000, 0.8660254037844387076, 1.000000000000000000, 0.8660254037844387076, 1.000000000000000000, 0.8660254037844387076, 1.000000000000000000, 0.8660254037844387076, 1.000000000000000000, 0.8660254037844387076, 1.000000000000000000, 0.8660254037844387076, 1.000000000000000000, 0.8660254037844387076, 1.000000000000000000, 0.8660254037844387076, 1.000000000000000000, 0.8660254037844387076, 1.000000000000000000, 0.8660254037844387076, 1.000000000000000000, 0.8660254037844387076, 1.000000000000000000, 0.8660254037844387076, 1.000000000000000000, 0.8660254037844387076, 1.000000000000000000, 0.8660254037844387076, 1.000000000000000000, 0.8660254037844387076, 1.000000000000000000, 0.8660254037844387076, 1.000000000000000000, 0.8660254037844387076, 1.000000000000000000, 0.8660254037844387076, 1.000000000000000000, 0.8660254037844387076, 1.000000000000000000, 0.8660254037844387076, 1.000000000000000000, 0.8660254037844387076, 1.000000000000000000, 0.8660254037844387076, 1.000000000000000000, 0.8660254037844387076, 1.000000000000000000, 0.8660254037844387076, 1.000000000000000000, 0.8660254037844387076, 1.000000000000000000, 0.8660254037844387076, 1.000000000000000000, 0.8660254037844387076, 1.000000000000000000, 0.8660254037844387076, 1.000000000000000000, 0.8660254037844387076, 1.000000000000000000, 0.8660254037844387076, 1.000000000000000000, 0.8660254037844387076, 1.000000000000000000, 0.8660254037844387076, 1.000000000000000000, 0.8660254037844387076, 1.000000000000000000, 0.8660254037844387076, 1.000000000000000000, 0.8660254037844387076, 1.000000000000000000, 0.8660254037844387076, 1.000000000000000000, 0.8660254037844387076, 1.000000000000000000, 0.8660254037844387076, 1.000000000000000000, 0.8660254037844387076, 1.000000000000000000, 0.8660254037844387076, 1.000000000000000000, 0.8660254037844387076, 1.000000000000000000, 0.8660254037844387076, 1.000000000000000000, 0.8660254037844387076, 1.000000000000000000, 0.8660254037844387076, 1.000000000000000000, 0.8660254037844387076, 1.000000000000000000, 0.8660254037844387076, 1.000000000000000000, 0.8660254037844387076, 1.000000000000000000, 0.8660254037844387076, 1.000000000000000000, 0.8660254037844387076, 1.000000000000000000, 0.8660254037844387076, 1.000000000000000000, 0.8660254037844387076, 1.000000000000000000, 0.8660254037844387076, 1.000000000000000000, 0.8660254037844387076, 1.000000000000000000, 0.8660254037844387076, 1.000000000000000000, 0.8660254037844387076, 1.000000000000000000, 0.8660254037844387076, 1.000000000000000000, 0.8660254037844387076, 1.000000000000000000, 0.8660254037844387076, 1.000000000000000000, 0.8660254037844387076, 1.000000000000000000, 0.8660254037844387076, 1.000000000000000000, 0.8660254037844387076, 1.000000000000000000, 0.8660254037844387076, 1.000000000000000000, 0.8660254037844387076, 1.000000000000000000, 0.8660254037844387076, 1.000000000000000000, 0.8660254037844387076, 1.000000000000000000, 0.8660254037844387076, 1.000000000000000000, 0.8660254037844387076, 1.000000000000000000, 0.8660254037844387076, 1.000000000000000000, 0.8660254037844387076, 1.000000000000000000, 0.8660254037844387076, 1.000000000000000000, 0.8660254037844387076, 1.000000000000000000, 0.8660254037844387076, 1.000000000000000000, 0.8660254037844387076, 1.000000000000000000, 0.8660254037844387076, 1.000000000000000000, 0.8660254037844387076, 1.000000000000000000, 0.8660254037844387076, 1.000000000000000000, 0.8660254037844387076, 1.000000000000000000, 0.8660254037844387076, 1.000000000000000000, 0.8660254037844387076, 1.000000000000000000, 0.8660254037844387076, 1.000000000000000000, 0.8660254037844387076, 1.000000000000000000, 0.8660254037844387076, 1.000000000000000000, 0.8660254037844387076, 1.000000000000000000, 0.8660254037844387076, 1.000000000000000000, 0.8660254037844387076, 1.000000000000000000, 0.8660254037844387076, 1.000000000000000000, 0.8660254037844387076, 1.000000000000000000, 0.8660254037844387076, 1.000000000000000000, 0.8660254037844387076, 1.000000000000000000, 0.8660254037844387076, 1.000000000000000000, 0.8660254037844387076, 1.000000000000000000, 0.8660254037844387076, 1.000000000000000000, 0.8660254037844387076, 1.000000000000000000, 0.8660254037844387076, 1.000000000000000000, 0.8660254037844387076, 1.000000000000000000, 0.8660254037844387076, 1.000000000000000000, 0.8660254037844387076, 1.000000000000000000, 0.8660254037844387076, 1.000000000000000000, 0.8660254037844387076, 1.000000000000000000, 0.8660254037844387076, 1.000000000000000000, 0.8660254037844387076, 1.000000000000000000, 0.8660254037844387076, 1.000000000000000000, 0.8660254037844387076, 1.000000000000000000, 0.8660254037844387076, 1.000000000000000000, 0.8660254037844387076, 1.000000000000000000, 0.8660254037844387076, 1.000000000000000000, 0.8660254037844387076, 1.000000000000000000, 0.8660254037844387076, 1.000000000000000000, 0.8660254037844387076, 1.000000000000000000, 0.8660254037844387076, 1.000000000000000000, 0.8660254037844387076, 1.000000000000000000, 0.8660254037844387076, 1.000000000000000000, 0.8660254037844387076, 1.000000000000000000, 0.8660254037844387076, 1.000000000000000000, 0.8660254037844387076, 1.000000000000000000, 0.8660254037844387076, 1.000000000000000000, 0.8660254037844387076, 1.000000000000000000, 0.8660254037844387076, 1.000000000000000000, 0.8660254037844387076, 1.000000000000000000, 0.8660254037844387076, 1.000000000000000000, 0.8660254037844387076, 1.000000000000000000, 0.8660254037844387076, 1.000000000000000000, 0.8660254037844387076, 1.000000000000000000, 0.8660254037844387076, 1.000000000000000000) ) ) 
 REPRESENTATION_ITEM ( '' )  SURFACE ( )  );
#52305=AXIS2_PLACEMENT_3D ( 'NONE', #11385, #23268, #31650 ) ;
#52306=CARTESIAN_POINT ( 'NONE',  ( -4.458734124999998549, -35.47916666530107221, 2.574251347313722516 ) ) ;
#52307=CARTESIAN_POINT ( 'NONE',  ( -5.000000000000000000, -147.6250000027312126, -6.123233995736766282E-16 ) ) ;
#52312=CARTESIAN_POINT ( 'NONE',  ( 5.000000000000000000, -24.29166666393548368, -2.886751345948130876 ) ) ;
#52316=CARTESIAN_POINT ( 'NONE',  ( -2.229367062499996610, -88.39583333196773651, 3.861377020970582219 ) ) ;
#52318=CARTESIAN_POINT ( 'NONE',  ( 5.000000000000000888, 22.41666666666666785, 2.886751345948126879 ) ) ;
#52319=CARTESIAN_POINT ( 'NONE',  ( 4.458734124999997661, -139.7500000013655779, 1.846868145590737864 ) ) ;
#52328=CARTESIAN_POINT ( 'NONE',  ( -2.499999999999996447, -72.83333333333332860, 4.330127018922195425 ) ) ;
#52329=CARTESIAN_POINT ( 'NONE',  ( 1.975475456537005874E-15, -45.62499999726880873, 5.000000000000000000 ) ) ;
#52330=CARTESIAN_POINT ( 'NONE',  ( -4.458734124999999437, -84.64583333196773651, -2.574251347313719407 ) ) ;
#52333=ORIENTED_EDGE ( 'NONE', *, *, #42774, .T. ) ;
#52336=CARTESIAN_POINT ( 'NONE',  ( 5.000000000000000000, -164.1875000027312126, 2.071067811865478614 ) ) ;
#52338=CARTESIAN_POINT ( 'NONE',  ( 4.458734124999999437, 4.937500001365595637, -5.460374474430324690E-16 ) ) ;
#52339=CARTESIAN_POINT ( 'NONE',  ( -2.499999999999996447, -15.83333333333333037, 4.330127018922195425 ) ) ;
#52344=CARTESIAN_POINT ( 'NONE',  ( -1.049326080737009628E-13, -19.75000000000000000, 5.000000000000000000 ) ) ;
#52346=CARTESIAN_POINT ( 'NONE',  ( -4.458734124999999437, -9.312499998634406140, 0.000000000000000000 ) ) ;
#52348=CARTESIAN_POINT ( 'NONE',  ( -4.458734124999997661, -37.47916666530107221, 2.574251347313722516 ) ) ;
#52349=VECTOR ( 'NONE', #36053, 1000.000000000000000 ) ;
#52354=CARTESIAN_POINT ( 'NONE',  ( -4.458734124999998549, 12.77083333469892601, 2.574251347313722516 ) ) ;
#52355=CARTESIAN_POINT ( 'NONE',  ( -4.999999999999998224, -81.79166666393547303, 2.886751345948131764 ) ) ;
#52357=CARTESIAN_POINT ( 'NONE',  ( -4.458734124999999437, -82.56249999863440792, 0.000000000000000000 ) ) ;
#52360=CARTESIAN_POINT ( 'NONE',  ( -3.535250795749689387E-16, 18.87500000273118772, -5.773502691896257311 ) ) ;
#52361=VERTEX_POINT ( 'NONE', #46019 ) ;
#52362=CARTESIAN_POINT ( 'NONE',  ( 2.071067811865560326, -146.9375000027311842, -4.999999999999914735 ) ) ;
#52363=CARTESIAN_POINT ( 'NONE',  ( -1.339745962155601378, 15.79465819873851906, -5.000000000000007105 ) ) ;
#52365=CARTESIAN_POINT ( 'NONE',  ( 5.000000000000000000, -30.41666666666666785, -2.886751345948129988 ) ) ;
#52366=CARTESIAN_POINT ( 'NONE',  ( 4.458734125000001214, -33.89583333196773651, 2.574251347313718519 ) ) ;
#52367=CARTESIAN_POINT ( 'NONE',  ( -1.339745962155610925, -33.79465819873851729, 5.000000000000000000 ) ) ;
#52369=CARTESIAN_POINT ( 'NONE',  ( 2.499999999999998668, -30.20833333060214443, -4.330127018922193649 ) ) ;
#52371=CARTESIAN_POINT ( 'NONE',  ( 4.458734125000001214, -58.89583333196773651, 2.574251347313718519 ) ) ;
#52372=ORIENTED_EDGE ( 'NONE', *, *, #34552, .F. ) ;
#52373=CYLINDRICAL_SURFACE ( 'NONE', #59046, 5.000000000000000000 ) ;
#52374=CARTESIAN_POINT ( 'NONE',  ( -3.152548672688508926E-16, -6.812499998634404363, -5.148502694627439702 ) ) ;
#52377=CARTESIAN_POINT ( 'NONE',  ( 5.000000000000000888, -79.58333333333331439, 2.886751345948126879 ) ) ;
#52380=ADVANCED_FACE ( 'NONE', ( #55999 ), #6791, .T. ) ;
#52381=CARTESIAN_POINT ( 'NONE',  ( 5.000000000000000000, -75.37499999726880162, -6.123233995736766282E-16 ) ) ;
#52385=CARTESIAN_POINT ( 'NONE',  ( 4.458734124999999437, -22.06249999863440436, -5.460374474430324690E-16 ) ) ;
#52386=EDGE_CURVE ( 'NONE', #61565, #35439, #45726, .T. ) ;
#52387=CARTESIAN_POINT ( 'NONE',  ( 4.458734124999998549, -55.97916666530107932, -2.574251347313721627 ) ) ;
#52388=ORIENTED_EDGE ( 'NONE', *, *, #54329, .T. ) ;
#52389=( BOUNDED_CURVE ( )  B_SPLINE_CURVE ( 2, ( #34071, #23801, #38890, #4803, #53377, #29873, #5442, #58832, #14762 ),
 .UNSPECIFIED., .F., .F. ) 
 B_SPLINE_CURVE_WITH_KNOTS ( ( 3, 2, 2, 2, 3 ),
 ( 0.4729166666666666519, 0.4736111111111110938, 0.4749999999999999778, 0.4763888888888888618, 0.4770833333333333592 ),
 .UNSPECIFIED. ) 
 CURVE ( )  GEOMETRIC_REPRESENTATION_ITEM ( )  RATIONAL_B_SPLINE_CURVE ( ( 0.9330127018922194093, 0.9330127018922194093, 1.000000000000000000, 0.8660254037844387076, 1.000000000000000000, 0.8660254037844387076, 1.000000000000000000, 0.9330127018922167448, 0.9330127018922194093 ) ) 
 REPRESENTATION_ITEM ( '' )  );
#52391=CARTESIAN_POINT ( 'NONE',  ( 1.846868145590736310, -141.6250000013656631, 4.458734124999999437 ) ) ;
#52393=CARTESIAN_POINT ( 'NONE',  ( -5.000000000000000000, -167.6250000027312126, -6.123233995736766282E-16 ) ) ;
#52398=ORIENTED_EDGE ( 'NONE', *, *, #51583, .T. ) ;
#52399=EDGE_CURVE ( 'NONE', #24836, #54901, #25998, .T. ) ;
#52400=EDGE_CURVE ( 'NONE', #30240, #29389, #32812, .T. ) ;
#52404=( BOUNDED_CURVE ( )  B_SPLINE_CURVE ( 2, ( #43332, #42704, #38504, #53934, #18586, #28857, #62974, #33376, #33071 ),
 .UNSPECIFIED., .F., .F. ) 
 B_SPLINE_CURVE_WITH_KNOTS ( ( 3, 2, 2, 2, 3 ),
 ( 0.002083333333333333738, 0.002777777777777777884, 0.004166666666666666609, 0.005555555555555555768, 0.006250000000000000347 ),
 .UNSPECIFIED. ) 
 CURVE ( )  GEOMETRIC_REPRESENTATION_ITEM ( )  RATIONAL_B_SPLINE_CURVE ( ( 0.9330127018922194093, 0.9330127018922194093, 1.000000000000000000, 0.8660254037844387076, 1.000000000000000000, 0.8660254037844387076, 1.000000000000000000, 0.9330127018922192983, 0.9330127018922194093 ) ) 
 REPRESENTATION_ITEM ( '' )  );
#52405=CARTESIAN_POINT ( 'NONE',  ( 3.152801135295367541, -147.5625000013655779, -3.152801135295367541 ) ) ;
#52409=CARTESIAN_POINT ( 'NONE',  ( -4.458734124999999437, -68.64583333196773651, -2.574251347313719407 ) ) ;
#52412=CARTESIAN_POINT ( 'NONE',  ( 2.730187237215162345E-16, -140.1875000013656063, -4.458734124999999437 ) ) ;
#52415=CARTESIAN_POINT ( 'NONE',  ( -2.498395430326213474E-14, 16.24999999999999645, 5.000000000000000000 ) ) ;
#52418=CARTESIAN_POINT ( 'NONE',  ( -6.972266317189433020E-16, -80.24999999999998579, -5.000000000000000000 ) ) ;
#52420=CARTESIAN_POINT ( 'NONE',  ( -4.458734124999999437, 28.43750000136559208, 0.000000000000000000 ) ) ;
#52426=CARTESIAN_POINT ( 'NONE',  ( -4.458734124999999437, 6.687500001365593860, 0.000000000000000000 ) ) ;
#52428=CARTESIAN_POINT ( 'NONE',  ( -2.229367062499996610, -19.39583333196774007, 3.861377020970582219 ) ) ;
#52430=CARTESIAN_POINT ( 'NONE',  ( -4.458734124999999437, -157.9375000013655779, -5.460374474430324690E-16 ) ) ;
#52431=LINE ( 'NONE', #31849, #45913 ) ;
#52434=CARTESIAN_POINT ( 'NONE',  ( -4.458734124999999437, 29.60416666803225993, -2.574251347313719407 ) ) ;
#52435=CARTESIAN_POINT ( 'NONE',  ( 2.229367062500001939, -39.97916666530107221, 3.861377020970579999 ) ) ;
#52438=CARTESIAN_POINT ( 'NONE',  ( -2.229367062499996610, -66.39583333196773651, 3.861377020970582219 ) ) ;
#52442=CARTESIAN_POINT ( 'NONE',  ( -1.339745962155613812, -85.20534180126148271, -5.000000000000000000 ) ) ;
#52443=CARTESIAN_POINT ( 'NONE',  ( 5.000000000000000000, -144.1875000027312126, 2.071067811865478614 ) ) ;
#52444=CARTESIAN_POINT ( 'NONE',  ( -2.500000000000000444, -12.16666666666666607, -4.330127018922193649 ) ) ;
#52445=CARTESIAN_POINT ( 'NONE',  ( 4.458734125000001214, -15.89583333196773651, 2.574251347313718519 ) ) ;
#52446=VECTOR ( 'NONE', #57503, 1000.000000000000000 ) ;
#52447=CARTESIAN_POINT ( 'NONE',  ( -3.152548672688508926E-16, -79.56249999863440792, -5.148502694627439702 ) ) ;
#52449=CARTESIAN_POINT ( 'NONE',  ( 5.000000000000000000, -10.29166666393547835, -2.886751345948129988 ) ) ;
#52450=CARTESIAN_POINT ( 'NONE',  ( -2.229367062500000163, -43.47916666530106511, -3.861377020970580443 ) ) ;
#52451=ORIENTED_EDGE ( 'NONE', *, *, #55529, .F. ) ;
#52452=CARTESIAN_POINT ( 'NONE',  ( 2.499999999999998668, -41.33333333333333570, -4.330127018922193649 ) ) ;
#52453=CARTESIAN_POINT ( 'NONE',  ( -4.458734124999999437, 8.437500001365595637, 0.000000000000000000 ) ) ;
#52455=CARTESIAN_POINT ( 'NONE',  ( -9.184850993605147944E-16, -153.2500000000000000, 5.000000000000000000 ) ) ;
#52456=CARTESIAN_POINT ( 'NONE',  ( 5.000000000000000000, -63.50000000000000000, -6.123233995736766282E-16 ) ) ;
#52457=CARTESIAN_POINT ( 'NONE',  ( 4.458734124999999437, -161.6875000013655779, 0.000000000000000000 ) ) ;
#52459=CARTESIAN_POINT ( 'NONE',  ( -4.458734124999999437, -78.39583333196772230, -2.574251347313719407 ) ) ;
#52461=CARTESIAN_POINT ( 'NONE',  ( 5.000000000000000000, -166.0000000000000000, 0.000000000000000000 ) ) ;
#52462=CARTESIAN_POINT ( 'NONE',  ( 5.000000000000000888, -167.9375000000000284, -2.071067811865475505 ) ) ;
#52464=CARTESIAN_POINT ( 'NONE',  ( 2.229367062499998831, -5.895833331967740953, -3.861377020970580887 ) ) ;
#52465=CARTESIAN_POINT ( 'NONE',  ( -4.458734124999999437, -42.56249999863440081, 0.000000000000000000 ) ) ;
#52472=CARTESIAN_POINT ( 'NONE',  ( -4.458734124999999437, -70.64583333196773651, -2.574251347313719407 ) ) ;
#52473=CARTESIAN_POINT ( 'NONE',  ( -1.846868145590737420, -145.0000000013656063, 4.458734124999997661 ) ) ;
#52475=CARTESIAN_POINT ( 'NONE',  ( -2.071067811865604735, -150.4375000027312126, 4.999999999999872990 ) ) ;
#52476=EDGE_CURVE ( 'NONE', #19516, #4014, #23562, .T. ) ;
#52480=CARTESIAN_POINT ( 'NONE',  ( 4.458734124999998549, 0.2708333346989263979, -2.574251347313721627 ) ) ;
#52482=CARTESIAN_POINT ( 'NONE',  ( -4.458734124999999437, -158.0000000013656063, -1.846868145590735644 ) ) ;
#52483=( BOUNDED_CURVE ( )  B_SPLINE_CURVE ( 2, ( #28713, #14549, #39309, #39624, #38996, #43502, #15194, #20344, #58000 ),
 .UNSPECIFIED., .F., .F. ) 
 B_SPLINE_CURVE_WITH_KNOTS ( ( 3, 2, 2, 2, 3 ),
 ( 0.9249999999999998224, 0.9291666666666664742, 0.9333333333333331261, 0.9374999999999998890, 0.9416666666666665408 ),
 .UNSPECIFIED. ) 
 CURVE ( )  GEOMETRIC_REPRESENTATION_ITEM ( )  RATIONAL_B_SPLINE_CURVE ( ( 1.000000000000003997, 0.9238795325112826307, 1.000000000000000000, 0.9238795325112867385, 1.000000000000000000, 0.9238795325112867385, 1.000000000000000000, 0.9238795325112887369, 0.9999999999999980016 ) ) 
 REPRESENTATION_ITEM ( '' )  );
#52485=EDGE_LOOP ( 'NONE', ( #36287, #35932, #4758, #4489 ) ) ;
#52487=CARTESIAN_POINT ( 'NONE',  ( 1.975475456537005874E-15, -28.74999999999999645, 5.000000000000000000 ) ) ;
#52493=CARTESIAN_POINT ( 'NONE',  ( 0.000000000000000000, -170.0000000000000000, 0.000000000000000000 ) ) ;
#52497=CARTESIAN_POINT ( 'NONE',  ( 2.229367062500001939, 25.02083333469892779, 3.861377020970579999 ) ) ;
#52499=CARTESIAN_POINT ( 'NONE',  ( -3.152548672688508926E-16, -3.812499998634408360, -5.148502694627439702 ) ) ;
#52500=CARTESIAN_POINT ( 'NONE',  ( -5.000000000000000000, -33.87499999726880873, 0.000000000000000000 ) ) ;
#52502=CARTESIAN_POINT ( 'NONE',  ( 3.061616997868383141E-16, -139.8750000027312126, -5.000000000000000000 ) ) ;
#52510=CARTESIAN_POINT ( 'NONE',  ( 1.846868145590736310, -156.8750000013655779, 4.458734124999997661 ) ) ;
#52512=CARTESIAN_POINT ( 'NONE',  ( -3.535533905932737309, -147.6250000000000000, -3.535533905932738197 ) ) ;
#52514=CARTESIAN_POINT ( 'NONE',  ( 9.457646018065525792E-16, 16.68750000136559564, 5.148502694627439702 ) ) ;
#52520=CARTESIAN_POINT ( 'NONE',  ( -4.999999999999999112, 4.083333333333334814, 2.886751345948131764 ) ) ;
#52521=CARTESIAN_POINT ( 'NONE',  ( -2.229367062499996610, -63.14583333196774362, 3.861377020970582219 ) ) ;
#52522=CARTESIAN_POINT ( 'NONE',  ( 0.000000000000000000, -170.0000000000000000, 0.000000000000000000 ) ) ;
#52523=CARTESIAN_POINT ( 'NONE',  ( -4.458734124999998549, -27.22916666530107221, 2.574251347313722516 ) ) ;
#52524=CARTESIAN_POINT ( 'NONE',  ( -4.999999999999998224, -37.79166666393548724, 2.886751345948131764 ) ) ;
#52527=CARTESIAN_POINT ( 'NONE',  ( -2.500000000000000444, -46.16666666666666430, -4.330127018922193649 ) ) ;
#52528=DIRECTION ( 'NONE',  ( -0.000000000000000000, 1.000000000000000000, -0.000000000000000000 ) ) ;
#52532=CARTESIAN_POINT ( 'NONE',  ( 4.458734124999998549, -64.72916666530106511, -2.574251347313721627 ) ) ;
#52533=CARTESIAN_POINT ( 'NONE',  ( -4.458734125000000326, -147.2500000013656063, -1.846868145590735644 ) ) ;
#52534=CARTESIAN_POINT ( 'NONE',  ( 4.458734124999998549, -76.72916666530106511, -2.574251347313721627 ) ) ;
#52536=CARTESIAN_POINT ( 'NONE',  ( 9.457646018065525792E-16, -26.31249999863440792, 5.148502694627439702 ) ) ;
#52537=CARTESIAN_POINT ( 'NONE',  ( 2.500000000000002220, -68.54166666393547303, 4.330127018922192761 ) ) ;
#52539=LINE ( 'NONE', #28081, #42566 ) ;
#52543=CYLINDRICAL_SURFACE ( 'NONE', #25617, 5.000000000000000000 ) ;
#52545=CARTESIAN_POINT ( 'NONE',  ( -2.499999999999996447, -5.708333330602148870, 4.330127018922195425 ) ) ;
#52546=CARTESIAN_POINT ( 'NONE',  ( -6.972266317189433020E-16, 15.87500000273118417, -5.000000000000000000 ) ) ;
#52547=CARTESIAN_POINT ( 'NONE',  ( -4.458734124999999437, -51.56249999863440792, 0.000000000000000000 ) ) ;
#52552=CARTESIAN_POINT ( 'NONE',  ( 4.458734124999999437, 19.18750000136559564, -5.460374474430324690E-16 ) ) ;
#52555=CARTESIAN_POINT ( 'NONE',  ( 3.152801135295366208, -167.5625000013656063, 3.152801135295367985 ) ) ;
#52558=DIRECTION ( 'NONE',  ( 0.000000000000000000, 0.000000000000000000, 1.000000000000000000 ) ) ;
#52560=CARTESIAN_POINT ( 'NONE',  ( 5.000000000000000888, -140.0625000027312126, -2.071067811865475505 ) ) ;
#52563=LINE ( 'NONE', #53806, #24483 ) ;
#52567=DIRECTION ( 'NONE',  ( 0.000000000000000000, 0.000000000000000000, 1.000000000000000000 ) ) ;
#52570=CARTESIAN_POINT ( 'NONE',  ( 0.000000000000000000, -170.0000000000000000, 0.000000000000000000 ) ) ;
#52572=CARTESIAN_POINT ( 'NONE',  ( 2.071067811865476394, -152.3125000027312410, 5.000000000000000000 ) ) ;
#52573=ORIENTED_EDGE ( 'NONE', *, *, #14961, .F. ) ;
#52575=EDGE_CURVE ( 'NONE', #44494, #33925, #51920, .T. ) ;
#52579=( BOUNDED_CURVE ( )  B_SPLINE_CURVE ( 2, ( #52945, #39396, #43901, #44224, #48426, #58713, #38159, #29746, #5322 ),
 .UNSPECIFIED., .F., .F. ) 
 B_SPLINE_CURVE_WITH_KNOTS ( ( 3, 2, 2, 2, 3 ),
 ( 0.7979166666666667185, 0.7986111111111111605, 0.8000000000000000444, 0.8013888888888889284, 0.8020833333333333703 ),
 .UNSPECIFIED. ) 
 CURVE ( )  GEOMETRIC_REPRESENTATION_ITEM ( )  RATIONAL_B_SPLINE_CURVE ( ( 0.9330127018922194093, 0.9330127018922194093, 1.000000000000000000, 0.8660254037844387076, 1.000000000000000000, 0.8660254037844387076, 1.000000000000000000, 0.9330127018922194093, 0.9330127018922194093 ) ) 
 REPRESENTATION_ITEM ( '' )  );
#52580=CARTESIAN_POINT ( 'NONE',  ( -2.071067811865478170, -148.3125000000000000, 5.000000000000000000 ) ) ;
#52583=CARTESIAN_POINT ( 'NONE',  ( 2.500000000000002220, 22.45833333606451987, 4.330127018922192761 ) ) ;
#52584=CARTESIAN_POINT ( 'NONE',  ( 2.229367062499998831, -31.64583333196773651, -3.861377020970580887 ) ) ;
#52587=CARTESIAN_POINT ( 'NONE',  ( -8.190561711645485556E-16, -146.6875000013656063, 4.458734124999999437 ) ) ;
#52589=FACE_OUTER_BOUND ( 'NONE', #32245, .T. ) ;
#52590=CARTESIAN_POINT ( 'NONE',  ( -2.229367062499996610, -57.39583333196773651, 3.861377020970582219 ) ) ;
#52592=CARTESIAN_POINT ( 'NONE',  ( 5.000000000000000000, 21.50000000000000000, -6.123233995736766282E-16 ) ) ;
#52593=CARTESIAN_POINT ( 'NONE',  ( -1.339745962155613812, -37.08034179853029144, -5.000000000000000000 ) ) ;
#52594=CARTESIAN_POINT ( 'NONE',  ( -4.458734124999999437, 0.6875000013655957476, 0.000000000000000000 ) ) ;
#52596=FACE_OUTER_BOUND ( 'NONE', #56475, .T. ) ;
#52597=CARTESIAN_POINT ( 'NONE',  ( 4.458734125000001214, 11.85416666803225993, 2.574251347313718519 ) ) ;
#52598=ORIENTED_EDGE ( 'NONE', *, *, #45601, .T. ) ;
#52600=ORIENTED_EDGE ( 'NONE', *, *, #9817, .T. ) ;
#52601=CARTESIAN_POINT ( 'NONE',  ( -6.972266317189433020E-16, -7.124999997268814056, -5.000000000000000000 ) ) ;
#52602=CARTESIAN_POINT ( 'NONE',  ( 2.229367062499998831, -46.64583333196774362, -3.861377020970580887 ) ) ;
#52603=CARTESIAN_POINT ( 'NONE',  ( -1.846868145590737420, -161.0000000013656063, 4.458734124999999437 ) ) ;
#52604=CARTESIAN_POINT ( 'NONE',  ( -5.000000000000000000, -50.87499999726881583, 0.000000000000000000 ) ) ;
#52605=VERTEX_POINT ( 'NONE', #22220 ) ;
#52606=CARTESIAN_POINT ( 'NONE',  ( -4.458734124999998549, -22.22916666530107221, 2.574251347313722516 ) ) ;
#52609=CARTESIAN_POINT ( 'NONE',  ( 3.152801135295367541, -162.3125000013656063, -3.152801135295367541 ) ) ;
#52612=CARTESIAN_POINT ( 'NONE',  ( 9.457646018065525792E-16, -35.31249999863440792, 5.148502694627439702 ) ) ;
#52617=( BOUNDED_CURVE ( )  B_SPLINE_CURVE ( 2, ( #56904, #7062, #32121, #6742, #2251, #21855, #41450, #45972, #1937 ),
 .UNSPECIFIED., .F., .F. ) 
 B_SPLINE_CURVE_WITH_KNOTS ( ( 3, 2, 2, 2, 3 ),
 ( 0.3916666666666669960, 0.3958333333333336479, 0.4000000000000003553, 0.4041666666666670071, 0.4083333333333336590 ),
 .UNSPECIFIED. ) 
 CURVE ( )  GEOMETRIC_REPRESENTATION_ITEM ( )  RATIONAL_B_SPLINE_CURVE ( ( 0.9999999999999938938, 0.9238795325112928447, 1.000000000000000000, 0.9238795325112867385, 1.000000000000000000, 0.9238795325112867385, 1.000000000000000000, 0.9238795325112806323, 1.000000000000005995 ) ) 
 REPRESENTATION_ITEM ( '' )  );
#52620=CARTESIAN_POINT ( 'NONE',  ( 4.458734124999999437, -86.06249999863439371, -5.460374474430324690E-16 ) ) ;
#52624=( BOUNDED_CURVE ( )  B_SPLINE_CURVE ( 2, ( #30973, #26474, #12318, #2666, #41561, #31282, #61852, #7182, #55746 ),
 .UNSPECIFIED., .F., .F. ) 
 B_SPLINE_CURVE_WITH_KNOTS ( ( 3, 2, 2, 2, 3 ),
 ( 0.9812499999999999556, 0.9819444444444443976, 0.9833333333333332815, 0.9847222222222222765, 0.9854166666666667185 ),
 .UNSPECIFIED. ) 
 CURVE ( )  GEOMETRIC_REPRESENTATION_ITEM ( )  RATIONAL_B_SPLINE_CURVE ( ( 0.9330127018922194093, 0.9330127018922194093, 1.000000000000000000, 0.8660254037844387076, 1.000000000000000000, 0.8660254037844387076, 1.000000000000000000, 0.9330127018922194093, 0.9330127018922194093 ) ) 
 REPRESENTATION_ITEM ( '' )  );
#52625=CARTESIAN_POINT ( 'NONE',  ( 5.000000000000000000, -57.49999999999999289, -6.123233995736766282E-16 ) ) ;
#52627=CARTESIAN_POINT ( 'NONE',  ( 1.339745962155612702, -37.29465819873852439, -5.000000000000000000 ) ) ;
#52629=DIRECTION ( 'NONE',  ( -0.000000000000000000, 1.000000000000000000, -0.000000000000000000 ) ) ;
#52633=DIRECTION ( 'NONE',  ( 0.000000000000000000, 0.000000000000000000, 1.000000000000000000 ) ) ;
#52635=CARTESIAN_POINT ( 'NONE',  ( 2.229367062500001939, -83.22916666530106511, 3.861377020970579999 ) ) ;
#52638=EDGE_LOOP ( 'NONE', ( #7503, #9889, #57988, #15524 ) ) ;
#52639=CARTESIAN_POINT ( 'NONE',  ( -5.000000000000000000, 18.04166666939785557, -2.886751345948128211 ) ) ;
#52641=CARTESIAN_POINT ( 'NONE',  ( -5.000000000000000888, -166.6875000027311842, -2.071067811865475949 ) ) ;
#52650=CARTESIAN_POINT ( 'NONE',  ( 1.339745962155615144, -86.58034179853028434, 4.999999999999999112 ) ) ;
#52651=CARTESIAN_POINT ( 'NONE',  ( -3.535533905932738641, -152.3750000000000000, 3.535533905932737309 ) ) ;
#52652=CARTESIAN_POINT ( 'NONE',  ( -4.458734124999999437, -12.39583333196774184, -2.574251347313719407 ) ) ;
#52655=CARTESIAN_POINT ( 'NONE',  ( -2.229367062499996610, -39.39583333196773651, 3.861377020970582219 ) ) ;
#52656=CARTESIAN_POINT ( 'NONE',  ( 5.000000000000000000, -77.41666666666665719, -2.886751345948130876 ) ) ;
#52662=CARTESIAN_POINT ( 'NONE',  ( -3.152548672688508926E-16, 16.43750000136559564, -5.148502694627439702 ) ) ;
#52663=CARTESIAN_POINT ( 'NONE',  ( 1.975475456537005874E-15, -85.62499999726880162, 5.000000000000000000 ) ) ;
#52664=EDGE_CURVE ( 'NONE', #34612, #15531, #58484, .T. ) ;
#52665=CARTESIAN_POINT ( 'NONE',  ( 0.000000000000000000, -170.0000000000000000, 0.000000000000000000 ) ) ;
#52666=CARTESIAN_POINT ( 'NONE',  ( -2.229367062499996610, -82.39583333196773651, 3.861377020970582219 ) ) ;
#52668=CARTESIAN_POINT ( 'NONE',  ( -2.500000000000000444, 14.95833333606451809, -4.330127018922193649 ) ) ;
#52670=CARTESIAN_POINT ( 'NONE',  ( 2.500000000000002220, -35.66666666666666430, 4.330127018922192761 ) ) ;
#52674=CARTESIAN_POINT ( 'NONE',  ( 2.500000000000002220, -31.66666666666666075, 4.330127018922192761 ) ) ;
#52675=CARTESIAN_POINT ( 'NONE',  ( 9.457646018065525792E-16, -31.06249999863440436, 5.148502694627439702 ) ) ;
#52676=CARTESIAN_POINT ( 'NONE',  ( 0.000000000000000000, -170.0000000000000000, 0.000000000000000000 ) ) ;
#52677=CARTESIAN_POINT ( 'NONE',  ( 2.499999999999998668, -35.20833333060213732, -4.330127018922193649 ) ) ;
#52678=CARTESIAN_POINT ( 'NONE',  ( 2.229367062500001939, -60.97916666530106511, 3.861377020970579999 ) ) ;
#52679=VERTEX_POINT ( 'NONE', #57889 ) ;
#52681=CARTESIAN_POINT ( 'NONE',  ( 4.458734125000001214, -7.145833331967734736, 2.574251347313718519 ) ) ;
#52683=CARTESIAN_POINT ( 'NONE',  ( -4.999999999999999112, -76.91666666666667140, 2.886751345948131764 ) ) ;
#52686=CARTESIAN_POINT ( 'NONE',  ( -5.000000000000000000, -74.87499999726880162, 0.000000000000000000 ) ) ;
#52689=EDGE_CURVE ( 'NONE', #52296, #21524, #19027, .T. ) ;
#52690=CARTESIAN_POINT ( 'NONE',  ( -4.458734124999999437, -19.56249999863440081, 0.000000000000000000 ) ) ;
#52691=CARTESIAN_POINT ( 'NONE',  ( -2.229367062499996610, -55.39583333196773651, 3.861377020970582219 ) ) ;
#52692=ORIENTED_EDGE ( 'NONE', *, *, #25193, .F. ) ;
#52693=CARTESIAN_POINT ( 'NONE',  ( -1.846868145590737420, -168.0000000013655779, 4.458734124999999437 ) ) ;
#52696=ADVANCED_FACE ( 'NONE', ( #9298 ), #8676, .T. ) ;
#52697=ORIENTED_EDGE ( 'NONE', *, *, #39080, .T. ) ;
#52704=CARTESIAN_POINT ( 'NONE',  ( -3.152801135295367985, -146.0625000013655779, 3.152801135295367096 ) ) ;
#52708=CARTESIAN_POINT ( 'NONE',  ( -4.458734124999998549, -70.47916666530107932, 2.574251347313722516 ) ) ;
#52711=CARTESIAN_POINT ( 'NONE',  ( 4.458734124999997661, -139.5000000013655779, 1.846868145590737864 ) ) ;
#52718=CARTESIAN_POINT ( 'NONE',  ( 5.000000000000000888, -14.45833333060214976, 2.886751345948126879 ) ) ;
#52720=CARTESIAN_POINT ( 'NONE',  ( -4.458734124999999437, 22.35416666803225638, -2.574251347313719407 ) ) ;
#52723=ADVANCED_FACE ( 'NONE', ( #18944 ), #9614, .T. ) ;
#52729=EDGE_CURVE ( 'NONE', #3491, #12628, #43392, .T. ) ;
#52730=CARTESIAN_POINT ( 'NONE',  ( -2.229367062499996610, 7.854166668032260823, 3.861377020970582219 ) ) ;
#52732=CARTESIAN_POINT ( 'NONE',  ( 4.458734125000000326, -21.14583333196774362, 2.574251347313718519 ) ) ;
#52734=CARTESIAN_POINT ( 'NONE',  ( -1.846868145590734756, -157.1250000013656063, -4.458734125000000326 ) ) ;
#52735=CARTESIAN_POINT ( 'NONE',  ( 0.000000000000000000, -170.0000000000000000, 0.000000000000000000 ) ) ;
#52738=ADVANCED_FACE ( 'NONE', ( #19581 ), #52302, .T. ) ;
#52739=CARTESIAN_POINT ( 'NONE',  ( -4.458734124999998549, 28.77083333469892779, 2.574251347313722516 ) ) ;
#52740=CARTESIAN_POINT ( 'NONE',  ( -2.229367062499996610, -41.14583333196773651, 3.861377020970582219 ) ) ;
#52741=CARTESIAN_POINT ( 'NONE',  ( 1.975475456537005874E-15, -46.62499999726880873, 5.000000000000000000 ) ) ;
#52742=ADVANCED_FACE ( 'NONE', ( #15927 ), #34910, .T. ) ;
#52744=CARTESIAN_POINT ( 'NONE',  ( 4.458734125000000326, -69.14583333196773651, 2.574251347313718519 ) ) ;
#52746=CARTESIAN_POINT ( 'NONE',  ( 5.000000000000000888, -57.45833333060214443, 2.886751345948126879 ) ) ;
#52747=CARTESIAN_POINT ( 'NONE',  ( 2.071067811865603403, -156.3125000027311842, 4.999999999999872990 ) ) ;
#52750=CARTESIAN_POINT ( 'NONE',  ( 5.000000000000000000, -15.41666666666666963, -2.886751345948129988 ) ) ;
#52751=CARTESIAN_POINT ( 'NONE',  ( 4.458734125000001214, -17.89583333196774007, 2.574251347313718519 ) ) ;
#52753=CARTESIAN_POINT ( 'NONE',  ( 9.457646018065525792E-16, -77.06249999863440792, 5.148502694627439702 ) ) ;
#52754=( BOUNDED_CURVE ( )  B_SPLINE_CURVE ( 2, ( #10586, #5451, #59170, #34390, #25069, #45010, #59822, #5771, #1298 ),
 .UNSPECIFIED., .F., .F. ) 
 B_SPLINE_CURVE_WITH_KNOTS ( ( 3, 2, 2, 2, 3 ),
 ( 0.1812499999999999944, 0.1819444444444444364, 0.1833333333333333204, 0.1847222222222222321, 0.1854166666666666741 ),
 .UNSPECIFIED. ) 
 CURVE ( )  GEOMETRIC_REPRESENTATION_ITEM ( )  RATIONAL_B_SPLINE_CURVE ( ( 0.9330127018922194093, 0.9330127018922194093, 1.000000000000000000, 0.8660254037844387076, 1.000000000000000000, 0.8660254037844387076, 1.000000000000000000, 0.9330127018922194093, 0.9330127018922194093 ) ) 
 REPRESENTATION_ITEM ( '' )  );
#52755=CARTESIAN_POINT ( 'NONE',  ( 6.123233995736766282E-16, -170.0000000000000000, -5.000000000000000000 ) ) ;
#52756=CARTESIAN_POINT ( 'NONE',  ( -2.499999999999996447, -13.70833333060214976, 4.330127018922195425 ) ) ;
#52757=CARTESIAN_POINT ( 'NONE',  ( 4.458734124999999437, -46.81249999863440792, -5.460374474430324690E-16 ) ) ;
#52758=EDGE_LOOP ( 'NONE', ( #51659, #57498, #2498, #30518 ) ) ;
#52760=CARTESIAN_POINT ( 'NONE',  ( -4.458734124999998549, 7.520833334698926009, 2.574251347313722516 ) ) ;
#52761=ORIENTED_EDGE ( 'NONE', *, *, #2883, .T. ) ;
#52763=CARTESIAN_POINT ( 'NONE',  ( 2.499999999999998668, -59.33333333333333570, -4.330127018922193649 ) ) ;
#52764=CARTESIAN_POINT ( 'NONE',  ( -3.152801135295367985, -157.0625000013656063, 3.152801135295367096 ) ) ;
#52766=CARTESIAN_POINT ( 'NONE',  ( 1.339745962155612702, -14.29465819873851906, -5.000000000000000000 ) ) ;
#52767=CARTESIAN_POINT ( 'NONE',  ( 3.061616997868383141E-16, -166.7500000000000000, -5.000000000000000000 ) ) ;
#52768=CARTESIAN_POINT ( 'NONE',  ( 5.000000000000000000, -168.0625000000000000, 2.071067811865478614 ) ) ;
#52770=CARTESIAN_POINT ( 'NONE',  ( -2.229367062500000163, -7.729166665301073991, -3.861377020970580443 ) ) ;
#52771=CARTESIAN_POINT ( 'NONE',  ( -3.152548672688508926E-16, -40.81249999863440081, -5.148502694627439702 ) ) ;
#52772=AXIS2_PLACEMENT_3D ( 'NONE', #62754, #53089, #32843 ) ;
#52774=CARTESIAN_POINT ( 'NONE',  ( 1.846868145590736310, -152.6250000013655495, 4.458734124999999437 ) ) ;
#52776=CARTESIAN_POINT ( 'NONE',  ( 2.071067811865495045, -167.3125000027311842, 4.999999999999981348 ) ) ;
#52780=CARTESIAN_POINT ( 'NONE',  ( 4.458734124999998549, -67.97916666530107932, -2.574251347313721627 ) ) ;
#52781=CARTESIAN_POINT ( 'NONE',  ( 3.152801135295367541, -145.5625000013655779, -3.152801135295367541 ) ) ;
#52786=CARTESIAN_POINT ( 'NONE',  ( -4.458734124999998549, 3.770833334698929562, 2.574251347313722516 ) ) ;
#52788=CARTESIAN_POINT ( 'NONE',  ( 2.730187237215162345E-16, -153.1875000013656063, -4.458734124999999437 ) ) ;
#52790=EDGE_LOOP ( 'NONE', ( #59092, #49576, #41078, #28719 ) ) ;
#52795=CARTESIAN_POINT ( 'NONE',  ( -2.499999999999996447, 28.29166666939785202, 4.330127018922195425 ) ) ;
#52800=CARTESIAN_POINT ( 'NONE',  ( 6.123233995736766282E-16, -170.0000000000000000, -5.000000000000000000 ) ) ;
#52802=CARTESIAN_POINT ( 'NONE',  ( 4.458734124999999437, 24.18750000136559564, -5.460374474430324690E-16 ) ) ;
#52804=CARTESIAN_POINT ( 'NONE',  ( 9.457646018065525792E-16, -2.312499998634407028, 5.148502694627439702 ) ) ;
#52807=CARTESIAN_POINT ( 'NONE',  ( -5.000000000000000888, -142.6875000027311842, -2.071067811865475949 ) ) ;
#52812=VECTOR ( 'NONE', #59020, 1000.000000000000000 ) ;
#52815=CARTESIAN_POINT ( 'NONE',  ( 2.730187237215162345E-16, -158.4375000013655779, -4.458734124999999437 ) ) ;
#52819=CARTESIAN_POINT ( 'NONE',  ( -4.458734124999999437, 16.43750000136559564, 0.000000000000000000 ) ) ;
#52820=ORIENTED_EDGE ( 'NONE', *, *, #45714, .T. ) ;
#52824=( BOUNDED_CURVE ( )  B_SPLINE_CURVE ( 2, ( #48978, #29344, #34491, #38388, #14883, #29037, #4927, #34835, #43207 ),
 .UNSPECIFIED., .F., .F. ) 
 B_SPLINE_CURVE_WITH_KNOTS ( ( 3, 2, 2, 2, 3 ),
 ( 0.7604166666666666297, 0.7611111111111110716, 0.7624999999999999556, 0.7638888888888888395, 0.7645833333333332815 ),
 .UNSPECIFIED. ) 
 CURVE ( )  GEOMETRIC_REPRESENTATION_ITEM ( )  RATIONAL_B_SPLINE_CURVE ( ( 0.9330127018922194093, 0.9330127018922194093, 1.000000000000000000, 0.8660254037844387076, 1.000000000000000000, 0.8660254037844387076, 1.000000000000000000, 0.9330127018922194093, 0.9330127018922194093 ) ) 
 REPRESENTATION_ITEM ( '' )  );
#52825=CARTESIAN_POINT ( 'NONE',  ( 0.000000000000000000, -170.0000000000000000, 0.000000000000000000 ) ) ;
#52827=CARTESIAN_POINT ( 'NONE',  ( 2.500000000000002220, 4.333333333333331261, 4.330127018922192761 ) ) ;
#52828=CARTESIAN_POINT ( 'NONE',  ( 4.458734124999998549, -60.72916666530106511, -2.574251347313721627 ) ) ;
#52829=CARTESIAN_POINT ( 'NONE',  ( -2.500000000000000444, -53.04166666393548013, -4.330127018922193649 ) ) ;
#52830=EDGE_CURVE ( 'NONE', #21155, #59659, #4208, .T. ) ;
#52831=CARTESIAN_POINT ( 'NONE',  ( 2.499999999999998668, 2.791666669397851130, -4.330127018922193649 ) ) ;
#52832=CARTESIAN_POINT ( 'NONE',  ( 4.458734124999998549, -28.72916666530107221, -2.574251347313721627 ) ) ;
#52833=CARTESIAN_POINT ( 'NONE',  ( -5.000000000000000000, -42.08333333333333570, -2.886751345948128211 ) ) ;
#52834=CARTESIAN_POINT ( 'NONE',  ( 1.975475456537005874E-15, -56.75000000000000000, 5.000000000000000000 ) ) ;
#52835=DIRECTION ( 'NONE',  ( 0.000000000000000000, 0.000000000000000000, 1.000000000000000000 ) ) ;
#52836=CARTESIAN_POINT ( 'NONE',  ( 2.500000000000002220, -42.66666666666667140, 4.330127018922192761 ) ) ;
#52837=CARTESIAN_POINT ( 'NONE',  ( 2.500000000000002220, -26.54166666393547658, 4.330127018922192761 ) ) ;
#52839=CARTESIAN_POINT ( 'NONE',  ( -2.498395430326213474E-14, 14.37500000273118417, 5.000000000000000000 ) ) ;
#52840=CARTESIAN_POINT ( 'NONE',  ( 2.229367062500001939, -63.97916666530106511, 3.861377020970579999 ) ) ;
#52841=CARTESIAN_POINT ( 'NONE',  ( -3.152801135295367096, -146.3125000013655779, -3.152801135295367541 ) ) ;
#52842=CARTESIAN_POINT ( 'NONE',  ( -2.229367062500000163, -76.47916666530106511, -3.861377020970580443 ) ) ;
#52844=CARTESIAN_POINT ( 'NONE',  ( 2.229367062500001939, -27.22916666530106866, 3.861377020970579999 ) ) ;
#52845=CARTESIAN_POINT ( 'NONE',  ( 1.060575238724906964E-15, -64.62499999726881583, 5.773502691896257311 ) ) ;
#52847=CARTESIAN_POINT ( 'NONE',  ( 5.000000000000000000, -1.416666666666663410, -2.886751345948130876 ) ) ;
#52853=( BOUNDED_CURVE ( )  B_SPLINE_CURVE ( 2, ( #20672, #60233, #45420, #55720, #55078, #21299, #60862, #6193, #25807 ),
 .UNSPECIFIED., .F., .F. ) 
 B_SPLINE_CURVE_WITH_KNOTS ( ( 3, 2, 2, 2, 3 ),
 ( 0.1979166666666666574, 0.1986111111111110994, 0.2000000000000000111, 0.2013888888888888951, 0.2020833333333333370 ),
 .UNSPECIFIED. ) 
 CURVE ( )  GEOMETRIC_REPRESENTATION_ITEM ( )  RATIONAL_B_SPLINE_CURVE ( ( 0.9330127018922194093, 0.9330127018922194093, 1.000000000000000000, 0.8660254037844387076, 1.000000000000000000, 0.8660254037844387076, 1.000000000000000000, 0.9330127018922194093, 0.9330127018922194093 ) ) 
 REPRESENTATION_ITEM ( '' )  );
#52855=CARTESIAN_POINT ( 'NONE',  ( -4.458734124999999437, -53.56249999863439371, 0.000000000000000000 ) ) ;
#52857=ORIENTED_EDGE ( 'NONE', *, *, #11365, .T. ) ;
#52861=CARTESIAN_POINT ( 'NONE',  ( -4.458734124999998549, 19.77083333469892779, 2.574251347313722516 ) ) ;
#52864=CARTESIAN_POINT ( 'NONE',  ( -4.458734124999999437, -165.0000000013655779, -1.846868145590735644 ) ) ;
#52865=ORIENTED_EDGE ( 'NONE', *, *, #5603, .T. ) ;
#52867=CARTESIAN_POINT ( 'NONE',  ( 1.975475456537005874E-15, -85.62499999726880162, 5.000000000000000000 ) ) ;
#52870=DIRECTION ( 'NONE',  ( -0.000000000000000000, 1.000000000000000000, -0.000000000000000000 ) ) ;
#52873=CARTESIAN_POINT ( 'NONE',  ( 1.975475456537005874E-15, 6.249999999999998224, 5.000000000000000000 ) ) ;
#52875=DIRECTION ( 'NONE',  ( 0.000000000000000000, 0.000000000000000000, 1.000000000000000000 ) ) ;
#52881=CARTESIAN_POINT ( 'NONE',  ( -5.000000000000000888, -151.6875000027312126, -2.071067811865475949 ) ) ;
#52888=CARTESIAN_POINT ( 'NONE',  ( -5.000000000000000000, -143.5000000000000284, -6.123233995736766282E-16 ) ) ;
#52891=CARTESIAN_POINT ( 'NONE',  ( 0.000000000000000000, -170.0000000000000000, 5.000000000000000000 ) ) ;
#52892=CARTESIAN_POINT ( 'NONE',  ( -4.458734124999999437, -29.31249999863440436, 0.000000000000000000 ) ) ;
#52896=CARTESIAN_POINT ( 'NONE',  ( -1.846868145590734756, -146.1250000013655779, -4.458734125000000326 ) ) ;
#52899=CARTESIAN_POINT ( 'NONE',  ( 4.458734125000000326, -57.14583333196773651, 2.574251347313718519 ) ) ;
#52901=LINE ( 'NONE', #28450, #22701 ) ;
#52902=CARTESIAN_POINT ( 'NONE',  ( 1.060575238724906964E-15, 19.25000000000000000, 5.773502691896257311 ) ) ;
#52903=CARTESIAN_POINT ( 'NONE',  ( -2.500000000000000444, -89.16666666666665719, -4.330127018922193649 ) ) ;
#52904=CARTESIAN_POINT ( 'NONE',  ( 9.457646018065525792E-16, -2.062499998634407028, 5.148502694627439702 ) ) ;
#52905=CARTESIAN_POINT ( 'NONE',  ( -3.535533905932737309, -154.6250000000000000, -3.535533905932738197 ) ) ;
#52907=CARTESIAN_POINT ( 'NONE',  ( 2.229367062500001939, 7.770833334698926009, 3.861377020970579999 ) ) ;
#52909=EDGE_LOOP ( 'NONE', ( #1831, #49327, #50951, #23114 ) ) ;
#52910=CARTESIAN_POINT ( 'NONE',  ( -4.458734124999999437, -51.39583333196772941, -2.574251347313719407 ) ) ;
#52911=CARTESIAN_POINT ( 'NONE',  ( 4.458734124999999437, -160.7500000013655779, 1.846868145590737864 ) ) ;
#52912=CARTESIAN_POINT ( 'NONE',  ( 2.499999999999998668, -50.20833333060213732, -4.330127018922193649 ) ) ;
#52913=ORIENTED_EDGE ( 'NONE', *, *, #25746, .T. ) ;
#52914=CARTESIAN_POINT ( 'NONE',  ( 4.458734125000001214, -22.89583333196773651, 2.574251347313718519 ) ) ;
#52918=CARTESIAN_POINT ( 'NONE',  ( -4.458734125000000326, -160.0000000013656063, -1.846868145590735644 ) ) ;
#52920=CARTESIAN_POINT ( 'NONE',  ( 5.000000000000000888, -39.45833333060214443, 2.886751345948126879 ) ) ;
#52923=CARTESIAN_POINT ( 'NONE',  ( 4.458734124999999437, -37.06249999863440792, -5.460374474430324690E-16 ) ) ;
#52924=ORIENTED_EDGE ( 'NONE', *, *, #25556, .T. ) ;
#52929=ORIENTED_EDGE ( 'NONE', *, *, #1720, .T. ) ;
#52931=CARTESIAN_POINT ( 'NONE',  ( -3.152548672688508926E-16, -86.81249999863439371, -5.148502694627439702 ) ) ;
#52933=CARTESIAN_POINT ( 'NONE',  ( -1.339745962155614034, 25.33034180399266333, 4.999999999999999112 ) ) ;
#52940=AXIS2_PLACEMENT_3D ( 'NONE', #7386, #56273, #31177 ) ;
#52945=CARTESIAN_POINT ( 'NONE',  ( 1.975475456537005874E-15, -66.62499999726881583, 5.000000000000000000 ) ) ;
#52946=CARTESIAN_POINT ( 'NONE',  ( 4.458734124999998549, -83.97916666530107932, -2.574251347313721627 ) ) ;
#52949=ORIENTED_EDGE ( 'NONE', *, *, #51863, .T. ) ;
#52952=CARTESIAN_POINT ( 'NONE',  ( -3.535533905932737309, -165.7500000027312126, -3.535533905932738197 ) ) ;
#52961=CARTESIAN_POINT ( 'NONE',  ( 5.000000000000000888, 17.41666666666666430, 2.886751345948126879 ) ) ;
#52962=CARTESIAN_POINT ( 'NONE',  ( 4.458734124999999437, -13.81249999863440259, -5.460374474430324690E-16 ) ) ;
#52963=CARTESIAN_POINT ( 'NONE',  ( 1.339745962155612702, -71.29465819873850307, -5.000000000000000000 ) ) ;
#52964=ORIENTED_EDGE ( 'NONE', *, *, #13795, .T. ) ;
#52965=CARTESIAN_POINT ( 'NONE',  ( -4.458734124999999437, -41.56249999863440081, 0.000000000000000000 ) ) ;
#52966=CARTESIAN_POINT ( 'NONE',  ( -6.972266317189433020E-16, -77.25000000000000000, -5.000000000000000000 ) ) ;
#52971=CARTESIAN_POINT ( 'NONE',  ( -3.152548672688508926E-16, 14.43750000136559386, -5.148502694627439702 ) ) ;
#52972=CARTESIAN_POINT ( 'NONE',  ( -1.339745962155613812, -82.08034179853031276, -5.000000000000000000 ) ) ;
#52973=CARTESIAN_POINT ( 'NONE',  ( -6.972266317189433020E-16, -65.12499999726880162, -5.000000000000000000 ) ) ;
#52974=CARTESIAN_POINT ( 'NONE',  ( -4.458734124999997661, -87.47916666530107932, 2.574251347313722516 ) ) ;
#52976=CARTESIAN_POINT ( 'NONE',  ( -4.999999999999999112, 15.20833333606451987, 2.886751345948131764 ) ) ;
#52977=ORIENTED_EDGE ( 'NONE', *, *, #32193, .T. ) ;
#52978=CARTESIAN_POINT ( 'NONE',  ( -5.000000000000000000, -6.874999997268812280, 0.000000000000000000 ) ) ;
#52979=FACE_OUTER_BOUND ( 'NONE', #41035, .T. ) ;
#52981=CARTESIAN_POINT ( 'NONE',  ( -4.999999999999999112, -26.91666666666666075, 2.886751345948131764 ) ) ;
#52982=CARTESIAN_POINT ( 'NONE',  ( -3.152548672688508926E-16, -32.56249999863440792, -5.148502694627439702 ) ) ;
#52983=CARTESIAN_POINT ( 'NONE',  ( -3.535250795749689387E-16, -34.12499999726881583, -5.773502691896257311 ) ) ;
#52984=CARTESIAN_POINT ( 'NONE',  ( 4.458734124999999437, -62.81249999863440792, -5.460374474430324690E-16 ) ) ;
#52987=CARTESIAN_POINT ( 'NONE',  ( 4.458734124999998549, -13.97916666530107221, -2.574251347313721627 ) ) ;
#52989=CARTESIAN_POINT ( 'NONE',  ( 2.499999999999998668, -75.33333333333332860, -4.330127018922193649 ) ) ;
#52993=CARTESIAN_POINT ( 'NONE',  ( 5.000000000000000000, -80.37499999726881583, -6.123233995736766282E-16 ) ) ;
#52994=CARTESIAN_POINT ( 'NONE',  ( 5.000000000000000888, -65.45833333060213022, 2.886751345948126879 ) ) ;
#52997=ADVANCED_FACE ( 'NONE', ( #32863 ), #27088, .T. ) ;
#52998=CARTESIAN_POINT ( 'NONE',  ( 4.458734124999998549, -20.97916666530107221, -2.574251347313721627 ) ) ;
#52999=CARTESIAN_POINT ( 'NONE',  ( 4.458734124999999437, -57.06249999863440081, -5.460374474430324690E-16 ) ) ;
#53000=ORIENTED_EDGE ( 'NONE', *, *, #31152, .T. ) ;
#53001=CARTESIAN_POINT ( 'NONE',  ( -3.152801135295367096, -167.3125000013656063, -3.152801135295367541 ) ) ;
#53003=CARTESIAN_POINT ( 'NONE',  ( -1.339745962155610925, 18.20534180126147561, 5.000000000000000000 ) ) ;
#53004=VERTEX_POINT ( 'NONE', #46704 ) ;
#53012=CARTESIAN_POINT ( 'NONE',  ( -8.190561711645485556E-16, -142.9375000013656063, 4.458734124999999437 ) ) ;
#53014=EDGE_CURVE ( 'NONE', #21047, #61372, #30106, .T. ) ;
#53015=DIRECTION ( 'NONE',  ( -0.8660254037844410391, 0.4999999999999958367, 0.000000000000000000 ) ) ;
#53017=CARTESIAN_POINT ( 'NONE',  ( -4.458734124999999437, -66.56249999863440792, 0.000000000000000000 ) ) ;
#53020=CARTESIAN_POINT ( 'NONE',  ( 3.152801135295366208, -142.5625000013655779, 3.152801135295367985 ) ) ;
#53024=DIRECTION ( 'NONE',  ( -0.000000000000000000, 1.000000000000000000, -0.000000000000000000 ) ) ;
#53030=AXIS2_PLACEMENT_3D ( 'NONE', #10940, #11583, #6458 ) ;
#53031=CARTESIAN_POINT ( 'NONE',  ( -2.229367062499996610, 21.60416666803226349, 3.861377020970582219 ) ) ;
#53034=VECTOR ( 'NONE', #14330, 1000.000000000000000 ) ;
#53040=CARTESIAN_POINT ( 'NONE',  ( 2.229367062499998831, 1.354166668032261933, -3.861377020970580887 ) ) ;
#53041=CARTESIAN_POINT ( 'NONE',  ( 4.458734124999998549, -25.97916666530107221, -2.574251347313721627 ) ) ;
#53043=CARTESIAN_POINT ( 'NONE',  ( 1.846868145590735200, -156.2500000013656063, -4.458734125000000326 ) ) ;
#53046=CARTESIAN_POINT ( 'NONE',  ( -4.458734124999999437, 29.68750000136559208, 0.000000000000000000 ) ) ;
#53050=CARTESIAN_POINT ( 'NONE',  ( -3.152548672688508926E-16, -70.81249999863439371, -5.148502694627439702 ) ) ;
#53052=DIRECTION ( 'NONE',  ( 0.000000000000000000, 0.000000000000000000, 1.000000000000000000 ) ) ;
#53056=CARTESIAN_POINT ( 'NONE',  ( 5.000000000000000000, -10.50000000000000178, -6.123233995736766282E-16 ) ) ;
#53057=CARTESIAN_POINT ( 'NONE',  ( -3.152548672688508926E-16, -17.56249999863440792, -5.148502694627439702 ) ) ;
#53058=CARTESIAN_POINT ( 'NONE',  ( 9.457646018065525792E-16, -80.06249999863440792, 5.148502694627439702 ) ) ;
#53059=CARTESIAN_POINT ( 'NONE',  ( 4.458734125000000326, -168.6250000013655779, -1.846868145590734978 ) ) ;
#53060=CARTESIAN_POINT ( 'NONE',  ( 1.060575238724906964E-15, -17.62499999726881583, 5.773502691896257311 ) ) ;
#53061=CARTESIAN_POINT ( 'NONE',  ( 2.229367062499998831, -43.64583333196773651, -3.861377020970580887 ) ) ;
#53064=CARTESIAN_POINT ( 'NONE',  ( 9.457646018065525792E-16, 8.687500001365595637, 5.148502694627439702 ) ) ;
#53066=CARTESIAN_POINT ( 'NONE',  ( -5.000000000000000000, -86.95833333060214443, -2.886751345948128211 ) ) ;
#53067=CARTESIAN_POINT ( 'NONE',  ( -5.000000000000000000, -59.00000000000000000, 0.000000000000000000 ) ) ;
#53068=CARTESIAN_POINT ( 'NONE',  ( -3.152801135295367985, -155.0625000013656063, 3.152801135295367096 ) ) ;
#53070=CARTESIAN_POINT ( 'NONE',  ( -1.339745962155610925, -78.79465819873851729, 5.000000000000000000 ) ) ;
#53071=CARTESIAN_POINT ( 'NONE',  ( 5.000000000000000000, -164.0000000000000000, 0.000000000000000000 ) ) ;
#53072=CARTESIAN_POINT ( 'NONE',  ( 5.000000000000000000, 5.708333336064518981, -2.886751345948130876 ) ) ;
#53076=CARTESIAN_POINT ( 'NONE',  ( -2.229367062500000163, -4.729166665301071326, -3.861377020970580443 ) ) ;
#53078=CARTESIAN_POINT ( 'NONE',  ( 2.229367062500001939, -41.22916666530107932, 3.861377020970579999 ) ) ;
#53082=CARTESIAN_POINT ( 'NONE',  ( 1.846868145590736310, -147.6250000013655779, 4.458734124999999437 ) ) ;
#53085=DIRECTION ( 'NONE',  ( 0.000000000000000000, 0.000000000000000000, 1.000000000000000000 ) ) ;
#53089=DIRECTION ( 'NONE',  ( -0.000000000000000000, 1.000000000000000000, -0.000000000000000000 ) ) ;
#53090=CARTESIAN_POINT ( 'NONE',  ( -2.229367062499996610, -77.39583333196773651, 3.861377020970582219 ) ) ;
#53095=EDGE_CURVE ( 'NONE', #54241, #41751, #39109, .T. ) ;
#53097=CARTESIAN_POINT ( 'NONE',  ( 2.229367062499998831, 1.354166668032261933, -3.861377020970580887 ) ) ;
#53098=CYLINDRICAL_SURFACE ( 'NONE', #38769, 5.000000000000000000 ) ;
#53099=CARTESIAN_POINT ( 'NONE',  ( -1.846868145590734756, -154.1250000013655779, -4.458734124999999437 ) ) ;
#53101=ORIENTED_EDGE ( 'NONE', *, *, #38227, .F. ) ;
#53106=DIRECTION ( 'NONE',  ( -0.000000000000000000, 1.000000000000000000, -0.000000000000000000 ) ) ;
#53107=CARTESIAN_POINT ( 'NONE',  ( -5.000000000000000000, -13.08333333333333570, -2.886751345948128211 ) ) ;
#53112=CARTESIAN_POINT ( 'NONE',  ( 1.975475456537005874E-15, -44.74999999999999289, 5.000000000000000000 ) ) ;
#53113=CARTESIAN_POINT ( 'NONE',  ( -2.229367062500000163, 15.52083333469892779, -3.861377020970580443 ) ) ;
#53115=CARTESIAN_POINT ( 'NONE',  ( -4.458734124999997661, -11.47916666530107044, 2.574251347313722516 ) ) ;
#53117=CARTESIAN_POINT ( 'NONE',  ( -5.000000000000000000, -63.00000000000000000, 0.000000000000000000 ) ) ;
#53119=CARTESIAN_POINT ( 'NONE',  ( -1.846868145590734756, -169.1250000013656347, -4.458734125000000326 ) ) ;
#53120=DIRECTION ( 'NONE',  ( -0.000000000000000000, 1.000000000000000000, -0.000000000000000000 ) ) ;
#53126=CARTESIAN_POINT ( 'NONE',  ( 1.975475456537005874E-15, -45.62499999726880873, 5.000000000000000000 ) ) ;
#53130=CARTESIAN_POINT ( 'NONE',  ( 2.730187237215162345E-16, -157.4375000013655779, -4.458734124999999437 ) ) ;
#53138=CARTESIAN_POINT ( 'NONE',  ( -3.535250795749689387E-16, 2.749999999999999112, -5.773502691896257311 ) ) ;
#53139=CARTESIAN_POINT ( 'NONE',  ( -2.229367062499996610, -62.14583333196774362, 3.861377020970582219 ) ) ;
#53140=CARTESIAN_POINT ( 'NONE',  ( -2.500000000000000444, 19.83333333333333570, -4.330127018922193649 ) ) ;
#53141=CARTESIAN_POINT ( 'NONE',  ( 5.000000000000000888, -3.458333330602147093, 2.886751345948126879 ) ) ;
#53142=CARTESIAN_POINT ( 'NONE',  ( 2.229367062500001939, -27.97916666530107221, 3.861377020970579999 ) ) ;
#53146=CARTESIAN_POINT ( 'NONE',  ( 1.060575238724906964E-15, -46.75000000000000000, 5.773502691896257311 ) ) ;
#53149=CARTESIAN_POINT ( 'NONE',  ( -2.499999999999996447, 14.29166666939785202, 4.330127018922195425 ) ) ;
#53150=CARTESIAN_POINT ( 'NONE',  ( -4.458734124999998549, -70.22916666530107932, 2.574251347313722516 ) ) ;
#53151=CARTESIAN_POINT ( 'NONE',  ( -4.458734125000000326, -148.2500000013656063, -1.846868145590735644 ) ) ;
#53152=CARTESIAN_POINT ( 'NONE',  ( -4.458734124999999437, -76.39583333196775072, -2.574251347313719407 ) ) ;
#53154=CARTESIAN_POINT ( 'NONE',  ( 4.458734124999998549, -22.97916666530107221, -2.574251347313721627 ) ) ;
#53155=CARTESIAN_POINT ( 'NONE',  ( -2.500000000000000444, -66.04166666393547303, -4.330127018922193649 ) ) ;
#53156=EDGE_CURVE ( 'NONE', #46264, #18181, #1406, .T. ) ;
#53162=ORIENTED_EDGE ( 'NONE', *, *, #41247, .F. ) ;
#53163=ADVANCED_FACE ( 'NONE', ( #9217 ), #8592, .T. ) ;
#53164=VECTOR ( 'NONE', #25882, 1000.000000000000000 ) ;
#53165=DIRECTION ( 'NONE',  ( -0.000000000000000000, 1.000000000000000000, -0.000000000000000000 ) ) ;
#53166=CARTESIAN_POINT ( 'NONE',  ( -3.152548672688508926E-16, -56.81249999863439371, -5.148502694627439702 ) ) ;
#53169=VERTEX_POINT ( 'NONE', #63575 ) ;
#53172=EDGE_CURVE ( 'NONE', #63093, #12482, #7973, .T. ) ;
#53173=CARTESIAN_POINT ( 'NONE',  ( -2.229367062500000163, 17.52083333469892779, -3.861377020970580443 ) ) ;
#53175=CARTESIAN_POINT ( 'NONE',  ( -1.339745962155613812, -2.205341801261479162, -5.000000000000000000 ) ) ;
#53176=CARTESIAN_POINT ( 'NONE',  ( 3.152801135295367541, -163.3125000013656063, -3.152801135295367541 ) ) ;
#53177=ORIENTED_EDGE ( 'NONE', *, *, #43008, .F. ) ;
#53180=CARTESIAN_POINT ( 'NONE',  ( 5.000000000000000888, -39.58333333333333570, 2.886751345948126879 ) ) ;
#53182=EDGE_CURVE ( 'NONE', #45744, #43815, #50366, .T. ) ;
#53183=CARTESIAN_POINT ( 'NONE',  ( -1.339745962155613812, 1.794658198738520616, -5.000000000000000000 ) ) ;
#53188=CARTESIAN_POINT ( 'NONE',  ( -6.972266317189433020E-16, -18.12499999726881228, -5.000000000000000000 ) ) ;
#53192=( BOUNDED_CURVE ( )  B_SPLINE_CURVE ( 2, ( #58500, #33112, #23778, #13496, #48834, #19569, #47581, #44003, #13172 ),
 .UNSPECIFIED., .F., .F. ) 
 B_SPLINE_CURVE_WITH_KNOTS ( ( 3, 2, 2, 2, 3 ),
 ( 0.6020833333333333037, 0.6027777777777777457, 0.6041666666666666297, 0.6055555555555555136, 0.6062499999999999556 ),
 .UNSPECIFIED. ) 
 CURVE ( )  GEOMETRIC_REPRESENTATION_ITEM ( )  RATIONAL_B_SPLINE_CURVE ( ( 0.9330127018922194093, 0.9330127018922194093, 1.000000000000000000, 0.8660254037844387076, 1.000000000000000000, 0.8660254037844387076, 1.000000000000000000, 0.9330127018922194093, 0.9330127018922194093 ) ) 
 REPRESENTATION_ITEM ( '' )  );
#53193=DIRECTION ( 'NONE',  ( -0.000000000000000000, 1.000000000000000000, -0.000000000000000000 ) ) ;
#53195=CARTESIAN_POINT ( 'NONE',  ( 5.000000000000000888, -149.0625000027311842, -2.071067811865475505 ) ) ;
#53200=CARTESIAN_POINT ( 'NONE',  ( -5.000000000000000888, -142.5625000000000000, -2.071067811865475949 ) ) ;
#53202=CARTESIAN_POINT ( 'NONE',  ( -3.152801135295367096, -168.3125000013656063, -3.152801135295367541 ) ) ;
#53203=CARTESIAN_POINT ( 'NONE',  ( -4.458734124999999437, -30.39583333196773651, -2.574251347313719407 ) ) ;
#53204=CYLINDRICAL_SURFACE ( 'NONE', #58415, 5.000000000000000000 ) ;
#53207=CARTESIAN_POINT ( 'NONE',  ( 2.730187237215162345E-16, -146.1875000013656063, -4.458734124999999437 ) ) ;
#53209=CARTESIAN_POINT ( 'NONE',  ( 9.457646018065525792E-16, 26.68750000136559564, 5.148502694627439702 ) ) ;
#53211=CARTESIAN_POINT ( 'NONE',  ( -2.229367062499996610, -56.39583333196773651, 3.861377020970582219 ) ) ;
#53214=CARTESIAN_POINT ( 'NONE',  ( -3.535533905932737309, -162.6250000000000284, -3.535533905932738197 ) ) ;
#53215=CARTESIAN_POINT ( 'NONE',  ( -2.499999999999996447, 20.16666666666666430, 4.330127018922195425 ) ) ;
#53216=VECTOR ( 'NONE', #41174, 1000.000000000000000 ) ;
#53217=DIRECTION ( 'NONE',  ( -0.000000000000000000, 1.000000000000000000, -0.000000000000000000 ) ) ;
#53218=CARTESIAN_POINT ( 'NONE',  ( 4.458734124999999437, -5.812499998634403475, -5.460374474430324690E-16 ) ) ;
#53219=CARTESIAN_POINT ( 'NONE',  ( -3.535533905932738641, -154.3750000000000000, 3.535533905932737309 ) ) ;
#53221=CARTESIAN_POINT ( 'NONE',  ( -3.152548672688508926E-16, 9.187500001365593860, -5.148502694627439702 ) ) ;
#53223=ORIENTED_EDGE ( 'NONE', *, *, #15023, .F. ) ;
#53226=CARTESIAN_POINT ( 'NONE',  ( 4.458734124999998549, -56.72916666530107932, -2.574251347313721627 ) ) ;
#53227=CARTESIAN_POINT ( 'NONE',  ( -4.458734125000001214, -159.1250000013656063, 1.846868145590734089 ) ) ;
#53228=CARTESIAN_POINT ( 'NONE',  ( -5.000000000000000000, -48.95833333060213732, -2.886751345948128211 ) ) ;
#53229=ORIENTED_EDGE ( 'NONE', *, *, #61818, .T. ) ;
#53230=CARTESIAN_POINT ( 'NONE',  ( -4.458734124999999437, 4.437500001365595637, 0.000000000000000000 ) ) ;
#53233=CARTESIAN_POINT ( 'NONE',  ( -5.000000000000000888, -142.5625000027312410, 2.071067811865474617 ) ) ;
#53234=CARTESIAN_POINT ( 'NONE',  ( 1.846868145590735200, -160.2500000013656063, -4.458734125000000326 ) ) ;
#53239=CARTESIAN_POINT ( 'NONE',  ( 1.339745962155612702, -47.16965819600733312, -5.000000000000000000 ) ) ;
#53240=CARTESIAN_POINT ( 'NONE',  ( -2.229367062500000163, -37.72916666530107221, -3.861377020970580443 ) ) ;
#53244=CARTESIAN_POINT ( 'NONE',  ( 3.061616997868383141E-16, -156.8750000027311842, -5.000000000000000000 ) ) ;
#53246=CARTESIAN_POINT ( 'NONE',  ( 2.229367062499998831, -87.89583333196773651, -3.861377020970580887 ) ) ;
#53248=CARTESIAN_POINT ( 'NONE',  ( -2.499999999999996447, 25.29166666939785202, 4.330127018922195425 ) ) ;
#53250=CARTESIAN_POINT ( 'NONE',  ( -6.972266317189433020E-16, -45.12499999726880162, -5.000000000000000000 ) ) ;
#53252=CARTESIAN_POINT ( 'NONE',  ( -1.339745962155613812, -72.08034179853027013, -5.000000000000000000 ) ) ;
#53256=CARTESIAN_POINT ( 'NONE',  ( -5.000000000000000000, -82.00000000000000000, 0.000000000000000000 ) ) ;
#53260=LINE ( 'NONE', #14639, #57382 ) ;
#53261=CARTESIAN_POINT ( 'NONE',  ( -2.229367062499996610, -83.39583333196773651, 3.861377020970582219 ) ) ;
#53264=ORIENTED_EDGE ( 'NONE', *, *, #62495, .T. ) ;
#53265=CARTESIAN_POINT ( 'NONE',  ( 1.975475456537005874E-15, -80.74999999999998579, 5.000000000000000000 ) ) ;
#53267=CARTESIAN_POINT ( 'NONE',  ( -5.000000000000000888, -165.5625000027311842, 2.071067811865474617 ) ) ;
#53270=CYLINDRICAL_SURFACE ( 'NONE', #33561, 5.000000000000000000 ) ;
#53277=CARTESIAN_POINT ( 'NONE',  ( 4.458734124999998549, -15.72916666530107399, -2.574251347313721627 ) ) ;
#53278=FACE_OUTER_BOUND ( 'NONE', #15183, .T. ) ;
#53280=CARTESIAN_POINT ( 'NONE',  ( -3.152548672688508926E-16, -38.81249999863440081, -5.148502694627439702 ) ) ;
#53286=CARTESIAN_POINT ( 'NONE',  ( 2.229367062499998831, 9.354166668032261711, -3.861377020970580887 ) ) ;
#53289=CARTESIAN_POINT ( 'NONE',  ( 4.458734125000000326, -88.14583333196773651, 2.574251347313718519 ) ) ;
#53291=CARTESIAN_POINT ( 'NONE',  ( 2.500000000000002220, 13.45833333606451987, 4.330127018922192761 ) ) ;
#53292=ORIENTED_EDGE ( 'NONE', *, *, #36244, .T. ) ;
#53294=ORIENTED_EDGE ( 'NONE', *, *, #63342, .F. ) ;
#53295=VECTOR ( 'NONE', #21103, 1000.000000000000000 ) ;
#53296=CARTESIAN_POINT ( 'NONE',  ( -2.499999999999996447, 16.16666666666666430, 4.330127018922195425 ) ) ;
#53298=CARTESIAN_POINT ( 'NONE',  ( 5.000000000000000888, -28.58333333333333570, 2.886751345948126879 ) ) ;
#53299=CARTESIAN_POINT ( 'NONE',  ( 4.458734125000001214, -31.89583333196773651, 2.574251347313718519 ) ) ;
#53300=AXIS2_PLACEMENT_3D ( 'NONE', #17660, #26675, #12822 ) ;
#53302=CARTESIAN_POINT ( 'NONE',  ( 2.500000000000002220, -36.54166666393547303, 4.330127018922192761 ) ) ;
#53303=CARTESIAN_POINT ( 'NONE',  ( -3.152548672688508926E-16, -64.56249999863440792, -5.148502694627439702 ) ) ;
#53306=CARTESIAN_POINT ( 'NONE',  ( 9.457646018065525792E-16, -12.31249999863440259, 5.148502694627439702 ) ) ;
#53308=CARTESIAN_POINT ( 'NONE',  ( 2.500000000000002220, -74.66666666666665719, 4.330127018922192761 ) ) ;
#53311=CARTESIAN_POINT ( 'NONE',  ( 5.000000000000000000, -84.29166666393547303, -2.886751345948129988 ) ) ;
#53312=CARTESIAN_POINT ( 'NONE',  ( 1.975475456537005874E-15, -31.75000000000000000, 5.000000000000000000 ) ) ;
#53313=VERTEX_POINT ( 'NONE', #15952 ) ;
#53315=CARTESIAN_POINT ( 'NONE',  ( -2.229367062500000163, -23.72916666530107577, -3.861377020970580443 ) ) ;
#53316=CARTESIAN_POINT ( 'NONE',  ( 4.458734124999999437, -60.06249999863440081, -5.460374474430324690E-16 ) ) ;
#53320=CARTESIAN_POINT ( 'NONE',  ( 4.458734124999999437, -168.7500000013656063, 1.846868145590737864 ) ) ;
#53323=ORIENTED_EDGE ( 'NONE', *, *, #52213, .F. ) ;
#53330=CARTESIAN_POINT ( 'NONE',  ( 1.846868145590736310, -145.8750000013656063, 4.458734124999999437 ) ) ;
#53332=DIRECTION ( 'NONE',  ( -0.000000000000000000, 1.000000000000000000, -0.000000000000000000 ) ) ;
#53334=CARTESIAN_POINT ( 'NONE',  ( 4.458734124999999437, -68.06249999863440792, -5.460374474430324690E-16 ) ) ;
#53337=CARTESIAN_POINT ( 'NONE',  ( 1.846868145590735200, -142.2500000013656063, -4.458734124999999437 ) ) ;
#53339=VERTEX_POINT ( 'NONE', #40064 ) ;
#53343=CYLINDRICAL_SURFACE ( 'NONE', #27456, 5.000000000000000000 ) ;
#53345=CARTESIAN_POINT ( 'NONE',  ( 2.229367062499998831, 21.10416666803226349, -3.861377020970580887 ) ) ;
#53346=CARTESIAN_POINT ( 'NONE',  ( 0.000000000000000000, -170.0000000000000000, 0.000000000000000000 ) ) ;
#53351=CARTESIAN_POINT ( 'NONE',  ( 2.500000000000002220, -80.66666666666665719, 4.330127018922192761 ) ) ;
#53352=CARTESIAN_POINT ( 'NONE',  ( 4.458734124999998549, 3.270833334698929118, -2.574251347313721627 ) ) ;
#53353=CARTESIAN_POINT ( 'NONE',  ( 4.458734124999999437, -27.06249999863440081, -5.460374474430324690E-16 ) ) ;
#53354=CARTESIAN_POINT ( 'NONE',  ( 4.458734124999999437, -156.5000000013656347, 1.846868145590737864 ) ) ;
#53358=DIRECTION ( 'NONE',  ( -0.000000000000000000, 1.000000000000000000, -0.000000000000000000 ) ) ;
#53359=CARTESIAN_POINT ( 'NONE',  ( 0.000000000000000000, -170.0000000000000000, 0.000000000000000000 ) ) ;
#53361=CARTESIAN_POINT ( 'NONE',  ( 2.229367062500001939, -71.22916666530107932, 3.861377020970579999 ) ) ;
#53363=CARTESIAN_POINT ( 'NONE',  ( 5.000000000000000000, -73.41666666666665719, -2.886751345948130876 ) ) ;
#53364=CARTESIAN_POINT ( 'NONE',  ( 5.000000000000000888, -156.0625000027312126, -2.071067811865475505 ) ) ;
#53366=DIRECTION ( 'NONE',  ( -0.000000000000000000, 1.000000000000000000, -0.000000000000000000 ) ) ;
#53367=( BOUNDED_CURVE ( )  B_SPLINE_CURVE ( 2, ( #62089, #3240, #52116, #17069, #32487, #62407, #56948, #42447, #12244 ),
 .UNSPECIFIED., .F., .F. ) 
 B_SPLINE_CURVE_WITH_KNOTS ( ( 3, 2, 2, 2, 3 ),
 ( 0.5895833333333333481, 0.5902777777777777901, 0.5916666666666666741, 0.5930555555555555580, 0.5937500000000000000 ),
 .UNSPECIFIED. ) 
 CURVE ( )  GEOMETRIC_REPRESENTATION_ITEM ( )  RATIONAL_B_SPLINE_CURVE ( ( 0.9330127018922194093, 0.9330127018922194093, 1.000000000000000000, 0.8660254037844387076, 1.000000000000000000, 0.8660254037844387076, 1.000000000000000000, 0.9330127018922194093, 0.9330127018922194093 ) ) 
 REPRESENTATION_ITEM ( '' )  );
#53369=CARTESIAN_POINT ( 'NONE',  ( -4.999999999999999112, -14.91666666666666785, 2.886751345948131764 ) ) ;
#53370=CARTESIAN_POINT ( 'NONE',  ( -3.152548672688508926E-16, -19.56249999863440081, -5.148502694627439702 ) ) ;
#53371=CARTESIAN_POINT ( 'NONE',  ( 2.229367062500001939, -75.97916666530106511, 3.861377020970579999 ) ) ;
#53372=CARTESIAN_POINT ( 'NONE',  ( -3.152801135295367985, -168.0625000013656063, 3.152801135295367096 ) ) ;
#53373=ADVANCED_FACE ( 'NONE', ( #15638 ), #529, .T. ) ;
#53374=CARTESIAN_POINT ( 'NONE',  ( -2.499999999999996447, -19.70833333060214798, 4.330127018922195425 ) ) ;
#53375=CARTESIAN_POINT ( 'NONE',  ( -2.229367062500000163, -46.47916666530106511, -3.861377020970580443 ) ) ;
#53376=ORIENTED_EDGE ( 'NONE', *, *, #16124, .T. ) ;
#53377=CARTESIAN_POINT ( 'NONE',  ( -5.000000000000000000, -27.87499999726880873, 0.000000000000000000 ) ) ;
#53379=CARTESIAN_POINT ( 'NONE',  ( 4.458734124999999437, 0.9375000013655959696, -5.460374474430324690E-16 ) ) ;
#53380=ORIENTED_EDGE ( 'NONE', *, *, #16921, .F. ) ;
#53382=CARTESIAN_POINT ( 'NONE',  ( 5.000000000000000888, -63.58333333333332149, 2.886751345948126879 ) ) ;
#53383=CARTESIAN_POINT ( 'NONE',  ( -1.846868145590737420, -157.0000000013655779, 4.458734124999999437 ) ) ;
#53386=CARTESIAN_POINT ( 'NONE',  ( -2.499999999999996447, -55.83333333333332860, 4.330127018922195425 ) ) ;
#53387=CARTESIAN_POINT ( 'NONE',  ( 2.071067811865475505, -160.8125000000000284, -5.000000000000000888 ) ) ;
#53391=CARTESIAN_POINT ( 'NONE',  ( 2.229367062499998831, -7.895833331967735624, -3.861377020970580887 ) ) ;
#53392=CARTESIAN_POINT ( 'NONE',  ( -4.458734124999998549, -46.47916666530107221, 2.574251347313722516 ) ) ;
#53393=DIRECTION ( 'NONE',  ( -0.000000000000000000, 1.000000000000000000, -0.000000000000000000 ) ) ;
#53394=CARTESIAN_POINT ( 'NONE',  ( 4.458734125000000326, -147.3750000013656063, -1.846868145590734978 ) ) ;
#53400=CYLINDRICAL_SURFACE ( 'NONE', #52772, 5.000000000000000000 ) ;
#53401=EDGE_LOOP ( 'NONE', ( #49130, #17677, #7717, #22578 ) ) ;
#53402=CARTESIAN_POINT ( 'NONE',  ( 1.975475456537005874E-15, 12.37500000273118417, 5.000000000000000000 ) ) ;
#53406=CARTESIAN_POINT ( 'NONE',  ( 2.229367062499998831, -2.645833331967738289, -3.861377020970580887 ) ) ;
#53408=CARTESIAN_POINT ( 'NONE',  ( 4.458734124999999437, -154.4375000013655779, 0.000000000000000000 ) ) ;
#53423=CARTESIAN_POINT ( 'NONE',  ( -4.458734124999999437, 15.60416666803225993, -2.574251347313719407 ) ) ;
#53426=CARTESIAN_POINT ( 'NONE',  ( 9.457646018065525792E-16, -8.312499998634406140, 5.148502694627439702 ) ) ;
#53427=CARTESIAN_POINT ( 'NONE',  ( -4.999999999999998224, -33.79166666393547303, 2.886751345948131764 ) ) ;
#53429=CARTESIAN_POINT ( 'NONE',  ( -4.458734125000000326, -166.0000000013656063, -1.846868145590735644 ) ) ;
#53430=CARTESIAN_POINT ( 'NONE',  ( 1.339745962155612702, -88.29465819873851729, -5.000000000000000000 ) ) ;
#53434=EDGE_CURVE ( 'NONE', #48933, #45427, #3460, .T. ) ;
#53437=CARTESIAN_POINT ( 'NONE',  ( 0.000000000000000000, -170.0000000000000000, 5.000000000000000000 ) ) ;
#53439=CARTESIAN_POINT ( 'NONE',  ( 2.730187237215162345E-16, -152.4375000013655779, -4.458734124999999437 ) ) ;
#53443=VERTEX_POINT ( 'NONE', #24966 ) ;
#53446=CARTESIAN_POINT ( 'NONE',  ( 0.000000000000000000, -170.0000000000000000, 5.000000000000000000 ) ) ;
#53447=CARTESIAN_POINT ( 'NONE',  ( -5.000000000000000000, 1.916666666666667407, -2.886751345948128211 ) ) ;
#53449=CARTESIAN_POINT ( 'NONE',  ( -4.458734124999999437, -62.31249999863440792, 0.000000000000000000 ) ) ;
#53452=CARTESIAN_POINT ( 'NONE',  ( -2.500000000000000444, -1.041666663935479686, -4.330127018922193649 ) ) ;
#53453=CARTESIAN_POINT ( 'NONE',  ( -4.458734124999998549, -26.22916666530106866, 2.574251347313722516 ) ) ;
#53454=CARTESIAN_POINT ( 'NONE',  ( 5.000000000000000888, -156.9375000000000000, -2.071067811865475505 ) ) ;
#53455=EDGE_CURVE ( 'NONE', #61074, #35844, #30495, .T. ) ;
#53457=CARTESIAN_POINT ( 'NONE',  ( -5.000000000000000000, -47.00000000000000000, 0.000000000000000000 ) ) ;
#53458=EDGE_CURVE ( 'NONE', #11542, #141, #41200, .T. ) ;
#53462=CARTESIAN_POINT ( 'NONE',  ( 4.458734125000001214, -70.89583333196773651, 2.574251347313718519 ) ) ;
#53463=CARTESIAN_POINT ( 'NONE',  ( 4.458734125000000326, -145.6250000013655779, -1.846868145590734978 ) ) ;
#53464=CARTESIAN_POINT ( 'NONE',  ( -4.458734124999998549, -76.22916666530107932, 2.574251347313722516 ) ) ;
#53466=CARTESIAN_POINT ( 'NONE',  ( 4.458734124999999437, -25.06249999863440792, -5.460374474430324690E-16 ) ) ;
#53467=CARTESIAN_POINT ( 'NONE',  ( 5.000000000000000000, -64.29166666393547303, -2.886751345948129988 ) ) ;
#53468=ORIENTED_EDGE ( 'NONE', *, *, #34579, .T. ) ;
#53469=DIRECTION ( 'NONE',  ( -0.000000000000000000, 1.000000000000000000, -0.000000000000000000 ) ) ;
#53470=ORIENTED_EDGE ( 'NONE', *, *, #12141, .T. ) ;
#53472=CARTESIAN_POINT ( 'NONE',  ( 3.535533905932738197, -165.8750000000000284, -3.535533905932738197 ) ) ;
#53473=EDGE_LOOP ( 'NONE', ( #48547, #46697, #2768, #59801 ) ) ;
#53477=VECTOR ( 'NONE', #41185, 1000.000000000000000 ) ;
#53478=EDGE_CURVE ( 'NONE', #9545, #45336, #22377, .T. ) ;
#53479=CARTESIAN_POINT ( 'NONE',  ( -2.229367062500000163, -59.72916666530106511, -3.861377020970580443 ) ) ;
#53481=VERTEX_POINT ( 'NONE', #16591 ) ;
#53482=DIRECTION ( 'NONE',  ( 0.000000000000000000, 0.000000000000000000, 1.000000000000000000 ) ) ;
#53484=CARTESIAN_POINT ( 'NONE',  ( 9.457646018065525792E-16, 12.93750000136559386, 5.148502694627439702 ) ) ;
#53486=CARTESIAN_POINT ( 'NONE',  ( -1.846868145590737420, -166.7500000013655779, 4.458734124999997661 ) ) ;
#53491=( BOUNDED_CURVE ( )  B_SPLINE_CURVE ( 2, ( #12209, #11877, #21867, #1949, #21550, #61430, #17353, #41146, #36977 ),
 .UNSPECIFIED., .F., .F. ) 
 B_SPLINE_CURVE_WITH_KNOTS ( ( 3, 2, 2, 2, 3 ),
 ( 0.9395833333333333259, 0.9402777777777777679, 0.9416666666666666519, 0.9430555555555555358, 0.9437499999999999778 ),
 .UNSPECIFIED. ) 
 CURVE ( )  GEOMETRIC_REPRESENTATION_ITEM ( )  RATIONAL_B_SPLINE_CURVE ( ( 0.9330127018922194093, 0.9330127018922194093, 1.000000000000000000, 0.8660254037844387076, 1.000000000000000000, 0.8660254037844387076, 1.000000000000000000, 0.9330127018922194093, 0.9330127018922194093 ) ) 
 REPRESENTATION_ITEM ( '' )  );
#53492=CARTESIAN_POINT ( 'NONE',  ( 1.975475456537005874E-15, -19.62499999726881228, 5.000000000000000000 ) ) ;
#53502=CARTESIAN_POINT ( 'NONE',  ( 9.457646018065525792E-16, 7.687500001365596525, 5.148502694627439702 ) ) ;
#53505=CARTESIAN_POINT ( 'NONE',  ( -2.071067811865475061, -149.8125000027311842, -5.000000000000000888 ) ) ;
#53506=CARTESIAN_POINT ( 'NONE',  ( 2.788906526875773208E-15, 28.75000000000000000, -5.000000000000000000 ) ) ;
#53510=CARTESIAN_POINT ( 'NONE',  ( -9.184850993605147944E-16, -141.2500000000000284, 5.000000000000000000 ) ) ;
#53514=CARTESIAN_POINT ( 'NONE',  ( -1.846868145590734756, -166.3750000013656063, -4.458734124999999437 ) ) ;
#53515=CARTESIAN_POINT ( 'NONE',  ( 2.229367062500001939, -28.97916666530107221, 3.861377020970579999 ) ) ;
#53516=ADVANCED_FACE ( 'NONE', ( #37477 ), #56478, .T. ) ;
#53520=CARTESIAN_POINT ( 'NONE',  ( 4.458734124999999437, -142.4375000013656063, 0.000000000000000000 ) ) ;
#53522=CARTESIAN_POINT ( 'NONE',  ( 4.458734124999999437, 26.93750000136559564, -5.460374474430324690E-16 ) ) ;
#53524=CARTESIAN_POINT ( 'NONE',  ( 4.458734124999999437, -55.06249999863440081, -5.460374474430324690E-16 ) ) ;
#53526=CARTESIAN_POINT ( 'NONE',  ( -3.535533905932738641, -162.3750000000000284, 3.535533905932737309 ) ) ;
#53527=CARTESIAN_POINT ( 'NONE',  ( 1.060575238724906964E-15, 21.24999999999999645, 5.773502691896257311 ) ) ;
#53528=EDGE_CURVE ( 'NONE', #2442, #36547, #47772, .T. ) ;
#53529=CARTESIAN_POINT ( 'NONE',  ( -2.499999999999996447, -36.70833333060213732, 4.330127018922195425 ) ) ;
#53530=CARTESIAN_POINT ( 'NONE',  ( -3.152548672688508926E-16, -8.562499998634404363, -5.148502694627439702 ) ) ;
#53532=CARTESIAN_POINT ( 'NONE',  ( 3.535533905932738197, -165.0000000027312126, -3.535533905932738197 ) ) ;
#53539=CARTESIAN_POINT ( 'NONE',  ( -2.229367062500000163, -52.47916666530107221, -3.861377020970580443 ) ) ;
#53540=CARTESIAN_POINT ( 'NONE',  ( -4.458734125000001214, -155.1250000013655779, 1.846868145590734089 ) ) ;
#53541=ADVANCED_FACE ( 'NONE', ( #21743 ), #2756, .T. ) ;
#53542=CARTESIAN_POINT ( 'NONE',  ( -3.535250795749689387E-16, -49.12499999726881583, -5.773502691896257311 ) ) ;
#53543=ORIENTED_EDGE ( 'NONE', *, *, #2095, .T. ) ;
#53544=CARTESIAN_POINT ( 'NONE',  ( 4.458734124999998549, 6.020833334698928674, -2.574251347313721627 ) ) ;
#53546=( BOUNDED_CURVE ( )  B_SPLINE_CURVE ( 2, ( #3813, #23437, #57538, #27928, #58466, #34013, #62678, #18600, #33388 ),
 .UNSPECIFIED., .F., .F. ) 
 B_SPLINE_CURVE_WITH_KNOTS ( ( 3, 2, 2, 2, 3 ),
 ( 0.6604166666666666519, 0.6611111111111110938, 0.6624999999999999778, 0.6638888888888888618, 0.6645833333333333037 ),
 .UNSPECIFIED. ) 
 CURVE ( )  GEOMETRIC_REPRESENTATION_ITEM ( )  RATIONAL_B_SPLINE_CURVE ( ( 0.9330127018922194093, 0.9330127018922194093, 1.000000000000000000, 0.8660254037844387076, 1.000000000000000000, 0.8660254037844387076, 1.000000000000000000, 0.9330127018922194093, 0.9330127018922194093 ) ) 
 REPRESENTATION_ITEM ( '' )  );
#53549=CARTESIAN_POINT ( 'NONE',  ( -3.152801135295367096, -162.0625000013656063, -3.152801135295367541 ) ) ;
#53551=CARTESIAN_POINT ( 'NONE',  ( 5.000000000000000888, -87.45833333060214443, 2.886751345948126879 ) ) ;
#53553=CARTESIAN_POINT ( 'NONE',  ( 3.061616997868383141E-16, -149.7500000000000284, -5.000000000000000000 ) ) ;
#53554=CARTESIAN_POINT ( 'NONE',  ( -2.229367062499996610, -45.39583333196774362, 3.861377020970582219 ) ) ;
#53559=CARTESIAN_POINT ( 'NONE',  ( 4.458734125000001214, -88.14583333196773651, 2.574251347313718519 ) ) ;
#53561=CARTESIAN_POINT ( 'NONE',  ( 1.975475456537005874E-15, -86.75000000000001421, 5.000000000000000000 ) ) ;
#53566=AXIS2_PLACEMENT_3D ( 'NONE', #61120, #12528, #17044 ) ;
#53572=DIRECTION ( 'NONE',  ( 0.000000000000000000, 0.000000000000000000, 1.000000000000000000 ) ) ;
#53573=CARTESIAN_POINT ( 'NONE',  ( 2.229367062499998831, -83.89583333196773651, -3.861377020970580887 ) ) ;
#53578=CARTESIAN_POINT ( 'NONE',  ( -2.071067811865308972, -155.4375000027312126, 5.000000000000169642 ) ) ;
#53580=CARTESIAN_POINT ( 'NONE',  ( 2.071067811865475505, -162.9375000027312126, -5.000000000000000888 ) ) ;
#53591=CARTESIAN_POINT ( 'NONE',  ( -4.458734124999997661, -12.22916666530106866, 2.574251347313722516 ) ) ;
#53592=CARTESIAN_POINT ( 'NONE',  ( 6.123233995736766282E-16, -170.0000000000000000, -5.000000000000000000 ) ) ;
#53593=CARTESIAN_POINT ( 'NONE',  ( -5.000000000000000000, -154.5000000000000284, -6.123233995736766282E-16 ) ) ;
#53595=CARTESIAN_POINT ( 'NONE',  ( 9.457646018065525792E-16, -39.31249999863439371, 5.148502694627439702 ) ) ;
#53596=( BOUNDED_CURVE ( )  B_SPLINE_CURVE ( 2, ( #12436, #41692, #11789, #46539, #42331, #52318, #16629, #61339, #55877 ),
 .UNSPECIFIED., .F., .F. ) 
 B_SPLINE_CURVE_WITH_KNOTS ( ( 3, 2, 2, 2, 3 ),
 ( 0.06041666666666666713, 0.06111111111111110911, 0.06250000000000000000, 0.06388888888888888395, 0.06458333333333333981 ),
 .UNSPECIFIED. ) 
 CURVE ( )  GEOMETRIC_REPRESENTATION_ITEM ( )  RATIONAL_B_SPLINE_CURVE ( ( 0.9330127018922194093, 0.9330127018922194093, 1.000000000000000000, 0.8660254037844387076, 1.000000000000000000, 0.8660254037844387076, 1.000000000000000000, 0.9330127018922187432, 0.9330127018922194093 ) ) 
 REPRESENTATION_ITEM ( '' )  );
#53602=CARTESIAN_POINT ( 'NONE',  ( -2.229367062499996610, 8.854166668032261711, 3.861377020970582219 ) ) ;
#53605=CARTESIAN_POINT ( 'NONE',  ( 4.458734125000000326, -90.14583333196773651, 2.574251347313718519 ) ) ;
#53606=CARTESIAN_POINT ( 'NONE',  ( -4.458734124999998549, 22.52083333469892423, 2.574251347313722516 ) ) ;
#53608=CARTESIAN_POINT ( 'NONE',  ( -5.000000000000000000, 16.04166666939785202, -2.886751345948128211 ) ) ;
#53610=EDGE_LOOP ( 'NONE', ( #35138, #35133, #30474, #59015 ) ) ;
#53611=CARTESIAN_POINT ( 'NONE',  ( 1.975475456537005874E-15, -6.624999997268813168, 5.000000000000000000 ) ) ;
#53613=CYLINDRICAL_SURFACE ( 'NONE', #23472, 5.000000000000000000 ) ;
#53614=CARTESIAN_POINT ( 'NONE',  ( 5.000000000000000000, -34.41666666666666430, -2.886751345948129988 ) ) ;
#53615=CARTESIAN_POINT ( 'NONE',  ( 2.229367062499998831, -35.64583333196772941, -3.861377020970580887 ) ) ;
#53618=CARTESIAN_POINT ( 'NONE',  ( 5.000000000000000000, -32.29166666393548724, -2.886751345948129988 ) ) ;
#53619=CARTESIAN_POINT ( 'NONE',  ( 9.457646018065525792E-16, -65.06249999863440792, 5.148502694627439702 ) ) ;
#53620=EDGE_LOOP ( 'NONE', ( #56028, #22728, #34087, #21116 ) ) ;
#53622=CARTESIAN_POINT ( 'NONE',  ( 4.458734124999999437, -14.81249999863440436, -5.460374474430324690E-16 ) ) ;
#53623=CARTESIAN_POINT ( 'NONE',  ( 9.457646018065525792E-16, -16.31249999863440436, 5.148502694627439702 ) ) ;
#53624=ORIENTED_EDGE ( 'NONE', *, *, #6348, .F. ) ;
#53625=CARTESIAN_POINT ( 'NONE',  ( -2.500000000000000444, -83.16666666666667140, -4.330127018922193649 ) ) ;
#53628=CARTESIAN_POINT ( 'NONE',  ( 1.060575238724906964E-15, -84.62499999726880162, 5.773502691896257311 ) ) ;
#53629=CARTESIAN_POINT ( 'NONE',  ( -1.339745962155660663, -17.79465819873852439, 4.999999999999972466 ) ) ;
#53630=ORIENTED_EDGE ( 'NONE', *, *, #48718, .F. ) ;
#53632=CARTESIAN_POINT ( 'NONE',  ( -2.229367062499996610, -28.39583333196774007, 3.861377020970582219 ) ) ;
#53634=CARTESIAN_POINT ( 'NONE',  ( -1.846868145590737420, -166.0000000013656063, 4.458734124999999437 ) ) ;
#53636=VERTEX_POINT ( 'NONE', #30323 ) ;
#53645=CARTESIAN_POINT ( 'NONE',  ( -4.458734124999999437, -145.1875000013656063, -5.460374474430324690E-16 ) ) ;
#53649=CARTESIAN_POINT ( 'NONE',  ( -4.458734124999998549, -68.47916666530106511, 2.574251347313722516 ) ) ;
#53652=CARTESIAN_POINT ( 'NONE',  ( -3.152801135295367096, -140.0625000013655779, -3.152801135295367541 ) ) ;
#53654=ORIENTED_EDGE ( 'NONE', *, *, #35884, .T. ) ;
#53655=CARTESIAN_POINT ( 'NONE',  ( -2.500000000000000444, -50.04166666393547303, -4.330127018922193649 ) ) ;
#53661=CARTESIAN_POINT ( 'NONE',  ( 4.458734124999998549, 21.02083333469892779, -2.574251347313721627 ) ) ;
#53669=CARTESIAN_POINT ( 'NONE',  ( 4.458734124999998549, 2.270833334698928230, -2.574251347313721627 ) ) ;
#53670=EDGE_LOOP ( 'NONE', ( #32168, #40078, #43289, #5003 ) ) ;
#53671=CARTESIAN_POINT ( 'NONE',  ( 4.458734124999998549, -24.97916666530106511, -2.574251347313721627 ) ) ;
#53675=CARTESIAN_POINT ( 'NONE',  ( 4.458734125000001214, 28.10416666803225993, 2.574251347313718519 ) ) ;
#53676=CARTESIAN_POINT ( 'NONE',  ( 1.975475456537005874E-15, -11.62499999726881406, 5.000000000000000000 ) ) ;
#53678=CARTESIAN_POINT ( 'NONE',  ( 9.457646018065525792E-16, -74.31249999863440792, 5.148502694627439702 ) ) ;
#53683=DIRECTION ( 'NONE',  ( 0.000000000000000000, 0.000000000000000000, 1.000000000000000000 ) ) ;
#53685=CARTESIAN_POINT ( 'NONE',  ( -4.999999999999999112, -18.91666666666666430, 2.886751345948131764 ) ) ;
#53686=CARTESIAN_POINT ( 'NONE',  ( 4.458734124999999437, -24.81249999863440436, -5.460374474430324690E-16 ) ) ;
#53687=CARTESIAN_POINT ( 'NONE',  ( -4.458734124999997661, -80.22916666530107932, 2.574251347313722516 ) ) ;
#53688=( BOUNDED_CURVE ( )  B_SPLINE_CURVE ( 2, ( #34672, #40763, #54935, #25981, #50434, #25023, #29835, #10861, #30477 ),
 .UNSPECIFIED., .F., .F. ) 
 B_SPLINE_CURVE_WITH_KNOTS ( ( 3, 2, 2, 2, 3 ),
 ( 0.3770833333333333259, 0.3777777777777777679, 0.3791666666666666519, 0.3805555555555555358, 0.3812499999999999778 ),
 .UNSPECIFIED. ) 
 CURVE ( )  GEOMETRIC_REPRESENTATION_ITEM ( )  RATIONAL_B_SPLINE_CURVE ( ( 0.9330127018922194093, 0.9330127018922194093, 1.000000000000000000, 0.8660254037844387076, 1.000000000000000000, 0.8660254037844387076, 1.000000000000000000, 0.9330127018922194093, 0.9330127018922194093 ) ) 
 REPRESENTATION_ITEM ( '' )  );
#53689=CARTESIAN_POINT ( 'NONE',  ( 4.458734124999999437, -169.6875000013656063, 0.000000000000000000 ) ) ;
#53690=CARTESIAN_POINT ( 'NONE',  ( 5.000000000000000000, -16.37499999726881228, -6.123233995736766282E-16 ) ) ;
#53691=CARTESIAN_POINT ( 'NONE',  ( -3.152548672688508926E-16, -52.56249999863440792, -5.148502694627439702 ) ) ;
#53693=CARTESIAN_POINT ( 'NONE',  ( 1.975475456537005874E-15, -70.62499999726880162, 5.000000000000000000 ) ) ;
#53695=CARTESIAN_POINT ( 'NONE',  ( -2.229367062500000163, 2.270833334698928230, -3.861377020970580443 ) ) ;
#53696=VERTEX_POINT ( 'NONE', #19723 ) ;
#53698=CARTESIAN_POINT ( 'NONE',  ( -4.999999999999999112, -58.91666666666665719, 2.886751345948131764 ) ) ;
#53699=CARTESIAN_POINT ( 'NONE',  ( -4.458734125000000326, -156.2500000013656063, -1.846868145590735644 ) ) ;
#53701=CARTESIAN_POINT ( 'NONE',  ( -5.000000000000000000, -65.08333333333332860, -2.886751345948128211 ) ) ;
#53702=CARTESIAN_POINT ( 'NONE',  ( 3.061616997868383141E-16, -162.7500000000000000, -5.000000000000000000 ) ) ;
#53703=CARTESIAN_POINT ( 'NONE',  ( -5.000000000000000000, 10.91666666666666607, -2.886751345948128211 ) ) ;
#53705=CARTESIAN_POINT ( 'NONE',  ( -4.458734124999999437, -7.645833331967735624, -2.574251347313719407 ) ) ;
#53706=CARTESIAN_POINT ( 'NONE',  ( -2.229367062499996610, -48.39583333196772941, 3.861377020970582219 ) ) ;
#53708=CARTESIAN_POINT ( 'NONE',  ( 2.730187237215162345E-16, -147.1875000013656063, -4.458734124999999437 ) ) ;
#53710=CARTESIAN_POINT ( 'NONE',  ( 1.339745962155612702, 8.705341801261477386, -5.000000000000000000 ) ) ;
#53713=CARTESIAN_POINT ( 'NONE',  ( -1.049326080737009628E-13, -5.624999997268816720, 5.000000000000000000 ) ) ;
#53716=EDGE_CURVE ( 'NONE', #34465, #16762, #25186, .T. ) ;
#53720=CARTESIAN_POINT ( 'NONE',  ( -1.339745962155610925, -50.79465819873851018, 5.000000000000000000 ) ) ;
#53721=CARTESIAN_POINT ( 'NONE',  ( 4.458734124999998549, -1.729166665301068440, -2.574251347313721627 ) ) ;
#53722=CARTESIAN_POINT ( 'NONE',  ( 2.499999999999998668, -73.20833333060214443, -4.330127018922193649 ) ) ;
#53723=CARTESIAN_POINT ( 'NONE',  ( 3.152801135295366208, -153.5625000013656063, 3.152801135295367985 ) ) ;
#53728=CARTESIAN_POINT ( 'NONE',  ( 2.500000000000002220, -40.66666666666667140, 4.330127018922192761 ) ) ;
#53735=ORIENTED_EDGE ( 'NONE', *, *, #443, .F. ) ;
#53736=CARTESIAN_POINT ( 'NONE',  ( -2.229367062500000163, 17.52083333469892779, -3.861377020970580443 ) ) ;
#53738=CARTESIAN_POINT ( 'NONE',  ( 9.457646018065525792E-16, -7.312499998634403475, 5.148502694627439702 ) ) ;
#53742=CARTESIAN_POINT ( 'NONE',  ( 1.846868145590735200, -166.2500000013656347, -4.458734125000000326 ) ) ;
#53749=CARTESIAN_POINT ( 'NONE',  ( -8.190561711645485556E-16, -151.9375000013655779, 4.458734124999999437 ) ) ;
#53752=CARTESIAN_POINT ( 'NONE',  ( 1.975475456537005874E-15, -70.75000000000000000, 5.000000000000000000 ) ) ;
#53756=CARTESIAN_POINT ( 'NONE',  ( 5.000000000000000888, 4.416666666666666075, 2.886751345948126879 ) ) ;
#53757=CARTESIAN_POINT ( 'NONE',  ( -2.229367062499996610, -65.14583333196773651, 3.861377020970582219 ) ) ;
#53760=CARTESIAN_POINT ( 'NONE',  ( 2.500000000000002220, -3.541666663935478354, 4.330127018922192761 ) ) ;
#53761=CARTESIAN_POINT ( 'NONE',  ( 2.229367062500001939, -33.97916666530107221, 3.861377020970579999 ) ) ;
#53765=AXIS2_PLACEMENT_3D ( 'NONE', #31051, #50674, #60342 ) ;
#53766=CARTESIAN_POINT ( 'NONE',  ( 5.000000000000000000, 5.500000000000001776, -6.123233995736766282E-16 ) ) ;
#53767=CARTESIAN_POINT ( 'NONE',  ( 5.000000000000000000, -47.50000000000000000, -6.123233995736766282E-16 ) ) ;
#53768=( BOUNDED_CURVE ( )  B_SPLINE_CURVE ( 2, ( #21034, #59640, #16835, #45149, #16521, #36144, #15574, #25213, #60281 ),
 .UNSPECIFIED., .F., .F. ) 
 B_SPLINE_CURVE_WITH_KNOTS ( ( 3, 2, 2, 2, 3 ),
 ( 0.7729166666666666963, 0.7736111111111111382, 0.7750000000000000222, 0.7763888888888889062, 0.7770833333333333481 ),
 .UNSPECIFIED. ) 
 CURVE ( )  GEOMETRIC_REPRESENTATION_ITEM ( )  RATIONAL_B_SPLINE_CURVE ( ( 0.9330127018922194093, 0.9330127018922194093, 1.000000000000000000, 0.8660254037844387076, 1.000000000000000000, 0.8660254037844387076, 1.000000000000000000, 0.9330127018922194093, 0.9330127018922194093 ) ) 
 REPRESENTATION_ITEM ( '' )  );
#53772=CARTESIAN_POINT ( 'NONE',  ( -4.458734124999999437, -69.31249999863439371, 0.000000000000000000 ) ) ;
#53773=CARTESIAN_POINT ( 'NONE',  ( 2.730187237215162345E-16, -145.4375000013656063, -4.458734124999999437 ) ) ;
#53774=CARTESIAN_POINT ( 'NONE',  ( -2.229367062499996610, -74.14583333196773651, 3.861377020970582219 ) ) ;
#53776=CARTESIAN_POINT ( 'NONE',  ( -4.458734124999998549, -29.47916666530106866, 2.574251347313722516 ) ) ;
#53777=CARTESIAN_POINT ( 'NONE',  ( -5.000000000000000000, -70.87499999726880162, 0.000000000000000000 ) ) ;
#53778=ORIENTED_EDGE ( 'NONE', *, *, #1642, .F. ) ;
#53779=LINE ( 'NONE', #39614, #60813 ) ;
#53780=VERTEX_POINT ( 'NONE', #49945 ) ;
#53786=CARTESIAN_POINT ( 'NONE',  ( -6.972266317189433020E-16, -3.250000000000001332, -5.000000000000000000 ) ) ;
#53787=CARTESIAN_POINT ( 'NONE',  ( -2.229367062500000163, -61.72916666530106511, -3.861377020970580443 ) ) ;
#53790=ORIENTED_EDGE ( 'NONE', *, *, #31528, .T. ) ;
#53791=CARTESIAN_POINT ( 'NONE',  ( 0.000000000000000000, -170.0000000000000000, 5.000000000000000000 ) ) ;
#53792=CARTESIAN_POINT ( 'NONE',  ( -5.000000000000000000, -59.95833333060214443, -2.886751345948128211 ) ) ;
#53793=CARTESIAN_POINT ( 'NONE',  ( -4.458734124999999437, 15.68750000136559564, 0.000000000000000000 ) ) ;
#53796=CARTESIAN_POINT ( 'NONE',  ( -3.152801135295367985, -163.8125000013656063, 3.152801135295367096 ) ) ;
#53799=CARTESIAN_POINT ( 'NONE',  ( -2.499999999999996447, -51.70833333060213732, 4.330127018922195425 ) ) ;
#53806=CARTESIAN_POINT ( 'NONE',  ( 0.000000000000000000, -170.0000000000000000, 5.000000000000000000 ) ) ;
#53808=CARTESIAN_POINT ( 'NONE',  ( -6.972266317189433020E-16, -32.24999999999999289, -5.000000000000000000 ) ) ;
#53813=CARTESIAN_POINT ( 'NONE',  ( -2.229367062499996610, 4.604166668032261711, 3.861377020970582219 ) ) ;
#53814=CARTESIAN_POINT ( 'NONE',  ( 5.000000000000000000, -151.0000000000000284, 0.000000000000000000 ) ) ;
#53816=CARTESIAN_POINT ( 'NONE',  ( 3.061616997868383141E-16, -147.8750000027312126, -5.000000000000000000 ) ) ;
#53817=CARTESIAN_POINT ( 'NONE',  ( 0.000000000000000000, -170.0000000000000000, 5.000000000000000000 ) ) ;
#53820=EDGE_CURVE ( 'NONE', #40578, #62567, #56443, .T. ) ;
#53822=CARTESIAN_POINT ( 'NONE',  ( 2.071067811865475505, -141.8125000000000284, -5.000000000000000888 ) ) ;
#53824=CARTESIAN_POINT ( 'NONE',  ( 3.152801135295367541, -165.5625000013656063, -3.152801135295367541 ) ) ;
#53825=CARTESIAN_POINT ( 'NONE',  ( -4.458734124999999437, -32.39583333196773651, -2.574251347313719407 ) ) ;
#53829=CARTESIAN_POINT ( 'NONE',  ( -8.190561711645485556E-16, -143.6875000013656063, 4.458734124999999437 ) ) ;
#53830=VERTEX_POINT ( 'NONE', #9436 ) ;
#53831=CARTESIAN_POINT ( 'NONE',  ( 9.457646018065525792E-16, 27.68750000136559208, 5.148502694627439702 ) ) ;
#53833=CARTESIAN_POINT ( 'NONE',  ( 9.457646018065525792E-16, -56.31249999863440081, 5.148502694627439702 ) ) ;
#53836=CARTESIAN_POINT ( 'NONE',  ( 5.000000000000000000, 16.50000000000000000, -6.123233995736766282E-16 ) ) ;
#53838=CARTESIAN_POINT ( 'NONE',  ( -4.458734124999999437, -6.312499998634403475, 0.000000000000000000 ) ) ;
#53839=CARTESIAN_POINT ( 'NONE',  ( -3.535533905932738641, -168.3750000000000284, 3.535533905932737309 ) ) ;
#53841=CARTESIAN_POINT ( 'NONE',  ( -4.999999999999998224, -8.916666666666662522, 2.886751345948131764 ) ) ;
#53843=CARTESIAN_POINT ( 'NONE',  ( 1.339745962155612702, -53.16965819600733312, -5.000000000000000000 ) ) ;
#53844=CARTESIAN_POINT ( 'NONE',  ( 3.061616997868383141E-16, -142.8750000027312126, -5.000000000000000000 ) ) ;
#53847=CARTESIAN_POINT ( 'NONE',  ( -4.458734124999999437, -56.39583333196773651, -2.574251347313719407 ) ) ;
#53848=CARTESIAN_POINT ( 'NONE',  ( -8.190561711645485556E-16, -157.9375000013655779, 4.458734124999999437 ) ) ;
#53849=AXIS2_PLACEMENT_3D ( 'NONE', #46988, #12566, #7752 ) ;
#53850=CARTESIAN_POINT ( 'NONE',  ( 5.000000000000000000, -50.37499999726881583, -6.123233995736766282E-16 ) ) ;
#53852=CARTESIAN_POINT ( 'NONE',  ( 4.458734124999999437, 2.937500001365594304, -5.460374474430324690E-16 ) ) ;
#53854=CARTESIAN_POINT ( 'NONE',  ( 5.000000000000000888, -56.58333333333333570, 2.886751345948126879 ) ) ;
#53855=CARTESIAN_POINT ( 'NONE',  ( 4.458734124999999437, -157.4375000013655779, 0.000000000000000000 ) ) ;
#53859=CARTESIAN_POINT ( 'NONE',  ( -6.972266317189433020E-16, -47.12499999726880873, -5.000000000000000000 ) ) ;
#53860=CARTESIAN_POINT ( 'NONE',  ( -4.458734124999999437, -40.64583333196773651, -2.574251347313719407 ) ) ;
#53864=EDGE_CURVE ( 'NONE', #12680, #43260, #45125, .T. ) ;
#53865=EDGE_CURVE ( 'NONE', #13785, #26724, #34845, .T. ) ;
#53866=CARTESIAN_POINT ( 'NONE',  ( -2.500000000000000444, -46.16666666666666430, -4.330127018922193649 ) ) ;
#53870=CARTESIAN_POINT ( 'NONE',  ( -2.229367062500000163, 26.52083333469892779, -3.861377020970580443 ) ) ;
#53872=CARTESIAN_POINT ( 'NONE',  ( 0.000000000000000000, -170.0000000000000000, 0.000000000000000000 ) ) ;
#53878=ADVANCED_FACE ( 'NONE', ( #44801 ), #20372, .T. ) ;
#53884=CARTESIAN_POINT ( 'NONE',  ( -5.000000000000000000, -19.87499999726880873, 0.000000000000000000 ) ) ;
#53885=CARTESIAN_POINT ( 'NONE',  ( 4.458734124999998549, -87.97916666530107932, -2.574251347313721627 ) ) ;
#53889=CARTESIAN_POINT ( 'NONE',  ( -2.500000000000000444, -81.16666666666667140, -4.330127018922193649 ) ) ;
#53891=CARTESIAN_POINT ( 'NONE',  ( 2.071067811865475505, -159.9375000027312126, -5.000000000000000888 ) ) ;
#53901=CARTESIAN_POINT ( 'NONE',  ( 2.229367062500001939, -11.97916666530107044, 3.861377020970579999 ) ) ;
#53902=LINE ( 'NONE', #29439, #50405 ) ;
#53903=CARTESIAN_POINT ( 'NONE',  ( 5.000000000000000000, -157.0000000000000000, 0.000000000000000000 ) ) ;
#53906=CARTESIAN_POINT ( 'NONE',  ( 4.458734124999999437, -42.06249999863440081, -5.460374474430324690E-16 ) ) ;
#53912=CARTESIAN_POINT ( 'NONE',  ( 9.457646018065525792E-16, 7.937500001365594748, 5.148502694627439702 ) ) ;
#53915=CARTESIAN_POINT ( 'NONE',  ( 9.457646018065525792E-16, -87.31249999863440792, 5.148502694627439702 ) ) ;
#53916=CARTESIAN_POINT ( 'NONE',  ( 2.229367062500001939, 22.77083333469892423, 3.861377020970579999 ) ) ;
#53918=( BOUNDED_CURVE ( )  B_SPLINE_CURVE ( 2, ( #30128, #49757, #44938, #896, #20503, #40101, #59745, #15670, #22727 ),
 .UNSPECIFIED., .F., .F. ) 
 B_SPLINE_CURVE_WITH_KNOTS ( ( 3, 2, 2, 2, 3 ),
 ( 0.4583333333333337589, 0.4625000000000004663, 0.4666666666666671182, 0.4708333333333337700, 0.4750000000000004219 ),
 .UNSPECIFIED. ) 
 CURVE ( )  GEOMETRIC_REPRESENTATION_ITEM ( )  RATIONAL_B_SPLINE_CURVE ( ( 0.9999999999999918954, 0.9238795325112948431, 1.000000000000000000, 0.9238795325112867385, 1.000000000000000000, 0.9238795325112867385, 1.000000000000000000, 0.9238795325112786339, 1.000000000000008216 ) ) 
 REPRESENTATION_ITEM ( '' )  );
#53919=CARTESIAN_POINT ( 'NONE',  ( -5.000000000000000000, 13.04166666939785379, -2.886751345948128211 ) ) ;
#53922=ORIENTED_EDGE ( 'NONE', *, *, #51239, .F. ) ;
#53923=DIRECTION ( 'NONE',  ( 0.000000000000000000, 0.000000000000000000, 1.000000000000000000 ) ) ;
#53924=CARTESIAN_POINT ( 'NONE',  ( 1.060575238724906964E-15, -32.75000000000000711, 5.773502691896257311 ) ) ;
#53925=CARTESIAN_POINT ( 'NONE',  ( 4.458734125000001214, -39.89583333196772941, 2.574251347313718519 ) ) ;
#53926=CARTESIAN_POINT ( 'NONE',  ( 1.060575238724906964E-15, -32.62499999726880873, 5.773502691896257311 ) ) ;
#53927=CARTESIAN_POINT ( 'NONE',  ( 4.458734125000001214, -66.89583333196773651, 2.574251347313718519 ) ) ;
#53928=ORIENTED_EDGE ( 'NONE', *, *, #59061, .T. ) ;
#53930=CARTESIAN_POINT ( 'NONE',  ( -2.229367062499996610, -15.14583333196773474, 3.861377020970582219 ) ) ;
#53931=CARTESIAN_POINT ( 'NONE',  ( -2.229367062499996610, -12.39583333196774007, 3.861377020970582219 ) ) ;
#53932=VERTEX_POINT ( 'NONE', #30968 ) ;
#53933=CARTESIAN_POINT ( 'NONE',  ( -2.499999999999996447, -82.83333333333332860, 4.330127018922195425 ) ) ;
#53934=CARTESIAN_POINT ( 'NONE',  ( 5.000000000000000000, 28.70833333606451987, -2.886751345948130876 ) ) ;
#53936=CARTESIAN_POINT ( 'NONE',  ( 5.000000000000000000, -82.29166666393548724, -2.886751345948129988 ) ) ;
#53937=CARTESIAN_POINT ( 'NONE',  ( -1.339745962155613812, -32.20534180126148271, -5.000000000000000000 ) ) ;
#53940=CARTESIAN_POINT ( 'NONE',  ( 9.457646018065525792E-16, -29.31249999863440436, 5.148502694627439702 ) ) ;
#53941=VERTEX_POINT ( 'NONE', #36118 ) ;
#53942=AXIS2_PLACEMENT_3D ( 'NONE', #35209, #16229, #11074 ) ;
#53943=EDGE_CURVE ( 'NONE', #27774, #6544, #34230, .T. ) ;
#53945=CARTESIAN_POINT ( 'NONE',  ( 3.152801135295366208, -166.8125000013656063, 3.152801135295367985 ) ) ;
#53947=CARTESIAN_POINT ( 'NONE',  ( 2.499999999999998668, -55.20833333060214443, -4.330127018922193649 ) ) ;
#53952=CARTESIAN_POINT ( 'NONE',  ( 2.730187237215162345E-16, -146.4375000013656063, -4.458734124999999437 ) ) ;
#53957=ORIENTED_EDGE ( 'NONE', *, *, #49457, .T. ) ;
#53958=CARTESIAN_POINT ( 'NONE',  ( -4.458734125000000326, -143.2500000013655779, -1.846868145590735644 ) ) ;
#53961=CARTESIAN_POINT ( 'NONE',  ( 3.061616997868383141E-16, -140.8750000027312126, -5.000000000000000000 ) ) ;
#53963=CARTESIAN_POINT ( 'NONE',  ( 4.458734125000001214, -72.14583333196773651, 2.574251347313718519 ) ) ;
#53964=ADVANCED_FACE ( 'NONE', ( #46403 ), #36755, .T. ) ;
#53965=CARTESIAN_POINT ( 'NONE',  ( -3.535533905932737309, -144.7500000027311842, -3.535533905932738197 ) ) ;
#53978=CARTESIAN_POINT ( 'NONE',  ( -3.152548672688508926E-16, 23.18750000136559564, -5.148502694627439702 ) ) ;
#53979=CARTESIAN_POINT ( 'NONE',  ( -5.000000000000000000, 23.04166666939784847, -2.886751345948128211 ) ) ;
#53981=EDGE_CURVE ( 'NONE', #25633, #2707, #12311, .T. ) ;
#53986=CARTESIAN_POINT ( 'NONE',  ( 4.458734125000000326, 4.104166668032260823, 2.574251347313718519 ) ) ;
#53987=CARTESIAN_POINT ( 'NONE',  ( 4.458734124999999437, -25.06249999863440792, -5.460374474430324690E-16 ) ) ;
#53991=CARTESIAN_POINT ( 'NONE',  ( -4.458734124999999437, 24.68750000136559208, 0.000000000000000000 ) ) ;
#53994=CARTESIAN_POINT ( 'NONE',  ( 4.458734124999999437, -73.06249999863439371, -5.460374474430324690E-16 ) ) ;
#53997=ORIENTED_EDGE ( 'NONE', *, *, #34627, .T. ) ;
#53999=LINE ( 'NONE', #11212, #51482 ) ;
#54000=CARTESIAN_POINT ( 'NONE',  ( 5.000000000000000888, -20.58333333333333570, 2.886751345948126879 ) ) ;
#54001=CARTESIAN_POINT ( 'NONE',  ( -2.229367062499996610, -22.14583333196773651, 3.861377020970582219 ) ) ;
#54002=CARTESIAN_POINT ( 'NONE',  ( -2.229367062499996610, -85.14583333196773651, 3.861377020970582219 ) ) ;
#54003=CARTESIAN_POINT ( 'NONE',  ( 2.730187237215162345E-16, -167.4375000013655779, -4.458734124999999437 ) ) ;
#54004=CARTESIAN_POINT ( 'NONE',  ( -4.999999999999999112, -15.79166666393548191, 2.886751345948131764 ) ) ;
#54005=CARTESIAN_POINT ( 'NONE',  ( -2.229367062500000163, -49.47916666530107221, -3.861377020970580443 ) ) ;
#54008=DIRECTION ( 'NONE',  ( -0.000000000000000000, 1.000000000000000000, -0.000000000000000000 ) ) ;
#54009=CARTESIAN_POINT ( 'NONE',  ( 4.458734125000001214, 3.854166668032260823, 2.574251347313718519 ) ) ;
#54011=CARTESIAN_POINT ( 'NONE',  ( -1.339745962155610925, -86.66965819600733312, 5.000000000000000000 ) ) ;
#54012=CARTESIAN_POINT ( 'NONE',  ( -2.499999999999996447, -64.83333333333332860, 4.330127018922195425 ) ) ;
#54013=CARTESIAN_POINT ( 'NONE',  ( -1.846868145590737420, -156.0000000013656063, 4.458734124999999437 ) ) ;
#54015=CARTESIAN_POINT ( 'NONE',  ( -9.184850993605147944E-16, -163.2500000000000000, 5.000000000000000000 ) ) ;
#54018=CARTESIAN_POINT ( 'NONE',  ( -4.458734124999999437, -9.645833331967738289, -2.574251347313719407 ) ) ;
#54019=CARTESIAN_POINT ( 'NONE',  ( 4.458734124999999437, -44.06249999863440081, -5.460374474430324690E-16 ) ) ;
#54021=CARTESIAN_POINT ( 'NONE',  ( 1.846868145590736310, -146.6250000013655779, 4.458734124999999437 ) ) ;
#54024=ORIENTED_EDGE ( 'NONE', *, *, #57306, .F. ) ;
#54026=DIRECTION ( 'NONE',  ( -0.000000000000000000, 1.000000000000000000, -0.000000000000000000 ) ) ;
#54028=CARTESIAN_POINT ( 'NONE',  ( 2.500000000000002220, -30.66666666666666785, 4.330127018922192761 ) ) ;
#54029=ORIENTED_EDGE ( 'NONE', *, *, #6782, .T. ) ;
#54033=CARTESIAN_POINT ( 'NONE',  ( 6.123233995736766282E-16, -170.0000000000000000, -5.000000000000000000 ) ) ;
#54034=CARTESIAN_POINT ( 'NONE',  ( -4.458734124999999437, -3.395833331967739177, -2.574251347313719407 ) ) ;
#54036=CARTESIAN_POINT ( 'NONE',  ( -8.190561711645485556E-16, -150.6875000013656063, 4.458734124999999437 ) ) ;
#54044=CARTESIAN_POINT ( 'NONE',  ( 6.123233995736766282E-16, -170.0000000000000000, -5.000000000000000000 ) ) ;
#54045=( BOUNDED_CURVE ( )  B_SPLINE_CURVE ( 2, ( #51013, #6958, #36856, #12083, #56802, #26567, #51656, #51966, #46186 ),
 .UNSPECIFIED., .F., .F. ) 
 B_SPLINE_CURVE_WITH_KNOTS ( ( 3, 2, 2, 2, 3 ),
 ( 0.3104166666666666741, 0.3111111111111111160, 0.3125000000000000000, 0.3138888888888888840, 0.3145833333333333259 ),
 .UNSPECIFIED. ) 
 CURVE ( )  GEOMETRIC_REPRESENTATION_ITEM ( )  RATIONAL_B_SPLINE_CURVE ( ( 0.9330127018922194093, 0.9330127018922194093, 1.000000000000000000, 0.8660254037844387076, 1.000000000000000000, 0.8660254037844387076, 1.000000000000000000, 0.9330127018922194093, 0.9330127018922194093 ) ) 
 REPRESENTATION_ITEM ( '' )  );
#54050=CARTESIAN_POINT ( 'NONE',  ( 1.975475456537005874E-15, -71.75000000000000000, 5.000000000000000000 ) ) ;
#54052=CARTESIAN_POINT ( 'NONE',  ( -3.152548672688508926E-16, 17.43750000136559564, -5.148502694627439702 ) ) ;
#54054=VERTEX_POINT ( 'NONE', #40303 ) ;
#54055=CARTESIAN_POINT ( 'NONE',  ( -2.229367062500000163, -6.729166665301073103, -3.861377020970580443 ) ) ;
#54057=CARTESIAN_POINT ( 'NONE',  ( 4.458734125000000326, -168.3750000013655779, -1.846868145590734978 ) ) ;
#54058=CARTESIAN_POINT ( 'NONE',  ( 1.339745962155615144, -88.70534180126146850, 4.999999999999999112 ) ) ;
#54062=CARTESIAN_POINT ( 'NONE',  ( 1.339745962155615144, -38.70534180126146850, 4.999999999999999112 ) ) ;
#54066=CARTESIAN_POINT ( 'NONE',  ( 4.458734124999999437, -152.6250000013655495, -1.846868145590734978 ) ) ;
#54075=CARTESIAN_POINT ( 'NONE',  ( 1.060575238724906964E-15, 0.2500000000000002220, 5.773502691896257311 ) ) ;
#54077=CARTESIAN_POINT ( 'NONE',  ( -2.229367062500000163, -67.47916666530106511, -3.861377020970580443 ) ) ;
#54079=CARTESIAN_POINT ( 'NONE',  ( -1.339745962155613812, -31.08034179853029144, -5.000000000000000000 ) ) ;
#54080=CARTESIAN_POINT ( 'NONE',  ( -5.000000000000000000, -1.874999997268814944, 0.000000000000000000 ) ) ;
#54081=CARTESIAN_POINT ( 'NONE',  ( -2.229367062499996610, -32.14583333196773651, 3.861377020970582219 ) ) ;
#54083=CARTESIAN_POINT ( 'NONE',  ( -4.999999999999998224, -41.91666666666667140, 2.886751345948131764 ) ) ;
#54084=CARTESIAN_POINT ( 'NONE',  ( 0.000000000000000000, -170.0000000000000000, 0.000000000000000000 ) ) ;
#54086=CARTESIAN_POINT ( 'NONE',  ( 2.499999999999998668, -50.33333333333332860, -4.330127018922193649 ) ) ;
#54089=CARTESIAN_POINT ( 'NONE',  ( -4.458734124999999437, -69.39583333196773651, -2.574251347313719407 ) ) ;
#54090=CARTESIAN_POINT ( 'NONE',  ( -8.190561711645485556E-16, -142.9375000013656063, 4.458734124999999437 ) ) ;
#54091=CARTESIAN_POINT ( 'NONE',  ( 2.229367062500001939, -81.97916666530106511, 3.861377020970579999 ) ) ;
#54093=CARTESIAN_POINT ( 'NONE',  ( 9.457646018065525792E-16, -29.31249999863440436, 5.148502694627439702 ) ) ;
#54094=CARTESIAN_POINT ( 'NONE',  ( 5.000000000000000000, -70.37499999726880162, -6.123233995736766282E-16 ) ) ;
#54095=ORIENTED_EDGE ( 'NONE', *, *, #33623, .T. ) ;
#54101=ORIENTED_EDGE ( 'NONE', *, *, #34284, .F. ) ;
#54102=CARTESIAN_POINT ( 'NONE',  ( -6.972266317189433020E-16, -39.25000000000000000, -5.000000000000000000 ) ) ;
#54104=CARTESIAN_POINT ( 'NONE',  ( -4.458734124999999437, -56.56249999863440081, 0.000000000000000000 ) ) ;
#54106=EDGE_LOOP ( 'NONE', ( #59233, #18559, #7539, #33661 ) ) ;
#54109=CARTESIAN_POINT ( 'NONE',  ( 4.458734125000001214, 14.10416666803225993, 2.574251347313718519 ) ) ;
#54111=CARTESIAN_POINT ( 'NONE',  ( 5.000000000000000000, -24.41666666666666430, -2.886751345948130876 ) ) ;
#54112=CARTESIAN_POINT ( 'NONE',  ( 4.458734124999999437, -166.3750000013656063, -1.846868145590734978 ) ) ;
#54113=( BOUNDED_CURVE ( )  B_SPLINE_CURVE ( 2, ( #15890, #25217, #35509, #44828, #39997, #30680, #6246, #25856, #49339 ),
 .UNSPECIFIED., .F., .F. ) 
 B_SPLINE_CURVE_WITH_KNOTS ( ( 3, 2, 2, 2, 3 ),
 ( 0.7937499999999999556, 0.7944444444444443976, 0.7958333333333332815, 0.7972222222222222765, 0.7979166666666667185 ),
 .UNSPECIFIED. ) 
 CURVE ( )  GEOMETRIC_REPRESENTATION_ITEM ( )  RATIONAL_B_SPLINE_CURVE ( ( 0.9330127018922194093, 0.9330127018922194093, 1.000000000000000000, 0.8660254037844387076, 1.000000000000000000, 0.8660254037844387076, 1.000000000000000000, 0.9330127018922194093, 0.9330127018922194093 ) ) 
 REPRESENTATION_ITEM ( '' )  );
#54117=CARTESIAN_POINT ( 'NONE',  ( 2.500000000000002220, -39.66666666666667140, 4.330127018922192761 ) ) ;
#54123=CARTESIAN_POINT ( 'NONE',  ( 2.499999999999998668, 12.79166666939785379, -4.330127018922193649 ) ) ;
#54129=CARTESIAN_POINT ( 'NONE',  ( 4.458734124999999437, 5.937500001365593860, -5.460374474430324690E-16 ) ) ;
#54130=CARTESIAN_POINT ( 'NONE',  ( 3.061616997868383141E-16, -150.7500000000000284, -5.000000000000000000 ) ) ;
#54132=CARTESIAN_POINT ( 'NONE',  ( 5.000000000000000000, -150.1250000027312126, 0.000000000000000000 ) ) ;
#54137=CARTESIAN_POINT ( 'NONE',  ( 3.535533905932736864, -144.1250000000000000, 3.535533905932738641 ) ) ;
#54140=CARTESIAN_POINT ( 'NONE',  ( 2.730187237215162345E-16, -167.4375000013655779, -4.458734124999999437 ) ) ;
#54141=CARTESIAN_POINT ( 'NONE',  ( 4.458734124999999437, -36.81249999863440792, -5.460374474430324690E-16 ) ) ;
#54143=CARTESIAN_POINT ( 'NONE',  ( -6.972266317189433020E-16, -45.12499999726880162, -5.000000000000000000 ) ) ;
#54145=CARTESIAN_POINT ( 'NONE',  ( -1.846868145590734756, -142.1250000013656063, -4.458734125000000326 ) ) ;
#54146=ORIENTED_EDGE ( 'NONE', *, *, #42035, .T. ) ;
#54147=CARTESIAN_POINT ( 'NONE',  ( -4.999999999999999112, -90.79166666393545881, 2.886751345948131764 ) ) ;
#54148=ORIENTED_EDGE ( 'NONE', *, *, #12605, .T. ) ;
#54149=CARTESIAN_POINT ( 'NONE',  ( 4.458734125000000326, -62.14583333196774362, 2.574251347313718519 ) ) ;
#54152=CARTESIAN_POINT ( 'NONE',  ( 2.500000000000002220, 11.33333333333333393, 4.330127018922192761 ) ) ;
#54153=EDGE_CURVE ( 'NONE', #43336, #43748, #16605, .T. ) ;
#54154=CARTESIAN_POINT ( 'NONE',  ( -4.458734124999997661, -53.22916666530107932, 2.574251347313722516 ) ) ;
#54155=CARTESIAN_POINT ( 'NONE',  ( 4.458734125000001214, -5.895833331967740953, 2.574251347313718519 ) ) ;
#54156=DIRECTION ( 'NONE',  ( -0.000000000000000000, 1.000000000000000000, -0.000000000000000000 ) ) ;
#54157=CARTESIAN_POINT ( 'NONE',  ( 3.535533905932736864, -158.2500000027312126, 3.535533905932738641 ) ) ;
#54163=CARTESIAN_POINT ( 'NONE',  ( -4.458734124999999437, -53.31249999863439371, 0.000000000000000000 ) ) ;
#54164=CARTESIAN_POINT ( 'NONE',  ( -4.458734125000001214, -156.1250000013655779, 1.846868145590734089 ) ) ;
#54166=AXIS2_PLACEMENT_3D ( 'NONE', #14842, #39287, #58914 ) ;
#54168=CARTESIAN_POINT ( 'NONE',  ( -2.499999999999996447, -57.70833333060214443, 4.330127018922195425 ) ) ;
#54169=EDGE_LOOP ( 'NONE', ( #57210, #16604, #63348, #43641 ) ) ;
#54172=CARTESIAN_POINT ( 'NONE',  ( 4.458734124999999437, 5.937500001365593860, -5.460374474430324690E-16 ) ) ;
#54174=ORIENTED_EDGE ( 'NONE', *, *, #29384, .T. ) ;
#54175=CARTESIAN_POINT ( 'NONE',  ( -6.972266317189433020E-16, 21.87500000273118417, -5.000000000000000000 ) ) ;
#54176=CARTESIAN_POINT ( 'NONE',  ( 3.152801135295366208, -156.5625000013656063, 3.152801135295367985 ) ) ;
#54177=ORIENTED_EDGE ( 'NONE', *, *, #30575, .F. ) ;
#54180=CARTESIAN_POINT ( 'NONE',  ( -6.972266317189433020E-16, -59.12499999726880873, -5.000000000000000000 ) ) ;
#54181=CARTESIAN_POINT ( 'NONE',  ( 4.458734124999999437, -43.06249999863440081, -5.460374474430324690E-16 ) ) ;
#54182=ORIENTED_EDGE ( 'NONE', *, *, #25475, .F. ) ;
#54184=CARTESIAN_POINT ( 'NONE',  ( 5.000000000000000000, -143.1875000027312410, 2.071067811865478614 ) ) ;
#54188=CARTESIAN_POINT ( 'NONE',  ( -2.229367062500000163, 28.52083333469892779, -3.861377020970580443 ) ) ;
#54192=CARTESIAN_POINT ( 'NONE',  ( -1.127183054612291972E-14, 24.25000000000000000, 4.999999999999999112 ) ) ;
#54194=DIRECTION ( 'NONE',  ( 0.000000000000000000, 0.000000000000000000, 1.000000000000000000 ) ) ;
#54198=EDGE_CURVE ( 'NONE', #11102, #17248, #21111, .T. ) ;
#54200=CARTESIAN_POINT ( 'NONE',  ( 5.000000000000000888, -42.45833333060214443, 2.886751345948126879 ) ) ;
#54202=CARTESIAN_POINT ( 'NONE',  ( -4.458734124999998549, -89.47916666530106511, 2.574251347313722516 ) ) ;
#54207=CARTESIAN_POINT ( 'NONE',  ( 3.061616997868383141E-16, -143.8750000027312126, -5.000000000000000000 ) ) ;
#54209=CARTESIAN_POINT ( 'NONE',  ( -2.071067811865475061, -162.8125000027312126, -5.000000000000000888 ) ) ;
#54212=CARTESIAN_POINT ( 'NONE',  ( 5.000000000000000000, -19.29166666393548013, -2.886751345948130876 ) ) ;
#54214=CARTESIAN_POINT ( 'NONE',  ( 1.975475456537005874E-15, -66.74999999999998579, 5.000000000000000000 ) ) ;
#54220=CARTESIAN_POINT ( 'NONE',  ( -1.339745962155610925, -53.79465819873851018, 5.000000000000000000 ) ) ;
#54221=CARTESIAN_POINT ( 'NONE',  ( -2.229367062499996610, -17.14583333196773651, 3.861377020970582219 ) ) ;
#54222=CARTESIAN_POINT ( 'NONE',  ( 1.339745962155612702, -75.29465819873853150, -5.000000000000000000 ) ) ;
#54223=CARTESIAN_POINT ( 'NONE',  ( 3.535533905932736864, -156.1250000000000000, 3.535533905932738641 ) ) ;
#54225=ORIENTED_EDGE ( 'NONE', *, *, #23328, .F. ) ;
#54226=CARTESIAN_POINT ( 'NONE',  ( 9.457646018065525792E-16, -44.31249999863440081, 5.148502694627439702 ) ) ;
#54227=CARTESIAN_POINT ( 'NONE',  ( -5.000000000000000000, 26.00000000000000000, 0.000000000000000000 ) ) ;
#54233=CARTESIAN_POINT ( 'NONE',  ( -2.229367062500000163, 7.520833334698929562, -3.861377020970580443 ) ) ;
#54234=CARTESIAN_POINT ( 'NONE',  ( -3.535533905932738641, -165.5000000027312126, 3.535533905932737309 ) ) ;
#54235=CARTESIAN_POINT ( 'NONE',  ( 4.458734124999998549, -86.97916666530107932, -2.574251347313721627 ) ) ;
#54236=CARTESIAN_POINT ( 'NONE',  ( -4.458734124999999437, 20.35416666803225993, -2.574251347313719407 ) ) ;
#54238=CARTESIAN_POINT ( 'NONE',  ( -5.000000000000000000, 7.125000002731185944, 0.000000000000000000 ) ) ;
#54241=VERTEX_POINT ( 'NONE', #57015 ) ;
#54242=DIRECTION ( 'NONE',  ( -0.000000000000000000, 1.000000000000000000, -0.000000000000000000 ) ) ;
#54243=CARTESIAN_POINT ( 'NONE',  ( -5.000000000000000000, -33.00000000000000000, 0.000000000000000000 ) ) ;
#54244=CARTESIAN_POINT ( 'NONE',  ( -3.152548672688508926E-16, -38.56249999863439371, -5.148502694627439702 ) ) ;
#54245=( BOUNDED_CURVE ( )  B_SPLINE_CURVE ( 2, ( #1382, #59587, #49912, #29656, #35448, #10995, #14859, #10364, #39619 ),
 .UNSPECIFIED., .F., .F. ) 
 B_SPLINE_CURVE_WITH_KNOTS ( ( 3, 2, 2, 2, 3 ),
 ( 0.3520833333333333592, 0.3527777777777778012, 0.3541666666666666852, 0.3555555555555555691, 0.3562500000000000111 ),
 .UNSPECIFIED. ) 
 CURVE ( )  GEOMETRIC_REPRESENTATION_ITEM ( )  RATIONAL_B_SPLINE_CURVE ( ( 0.9330127018922194093, 0.9330127018922220739, 1.000000000000000000, 0.8660254037844387076, 1.000000000000000000, 0.8660254037844387076, 1.000000000000000000, 0.9330127018922194093, 0.9330127018922194093 ) ) 
 REPRESENTATION_ITEM ( '' )  );
#54246=CARTESIAN_POINT ( 'NONE',  ( -2.499999999999996447, -38.70833333060213732, 4.330127018922195425 ) ) ;
#54249=CARTESIAN_POINT ( 'NONE',  ( 9.457646018065525792E-16, -14.06249999863440259, 5.148502694627439702 ) ) ;
#54251=CARTESIAN_POINT ( 'NONE',  ( 4.458734124999998549, -16.97916666530107221, -2.574251347313721627 ) ) ;
#54252=ORIENTED_EDGE ( 'NONE', *, *, #48267, .F. ) ;
#54253=CARTESIAN_POINT ( 'NONE',  ( 2.499999999999998668, -84.33333333333332860, -4.330127018922193649 ) ) ;
#54257=CARTESIAN_POINT ( 'NONE',  ( -2.500000000000000444, -82.04166666393547303, -4.330127018922193649 ) ) ;
#54259=ORIENTED_EDGE ( 'NONE', *, *, #17388, .F. ) ;
#54262=CARTESIAN_POINT ( 'NONE',  ( 9.457646018065525792E-16, -25.31249999863440792, 5.148502694627439702 ) ) ;
#54263=CARTESIAN_POINT ( 'NONE',  ( 1.339745962155612702, -5.169658196007333117, -5.000000000000000000 ) ) ;
#54264=ORIENTED_EDGE ( 'NONE', *, *, #44076, .T. ) ;
#54265=CARTESIAN_POINT ( 'NONE',  ( 3.152801135295366208, -162.8125000013656063, 3.152801135295367985 ) ) ;
#54267=CARTESIAN_POINT ( 'NONE',  ( 5.000000000000000000, -148.0625000000000000, 2.071067811865478614 ) ) ;
#54270=CARTESIAN_POINT ( 'NONE',  ( -4.458734124999998549, -74.47916666530106511, 2.574251347313722516 ) ) ;
#54273=CARTESIAN_POINT ( 'NONE',  ( -3.152801135295367096, -144.3125000013655779, -3.152801135295367541 ) ) ;
#54274=CARTESIAN_POINT ( 'NONE',  ( 6.123233995736766282E-16, -170.0000000000000000, -5.000000000000000000 ) ) ;
#54275=CARTESIAN_POINT ( 'NONE',  ( 1.975475456537005874E-15, -47.62499999726880873, 5.000000000000000000 ) ) ;
#54279=CARTESIAN_POINT ( 'NONE',  ( 4.458734124999999437, -141.7500000013655779, 1.846868145590737864 ) ) ;
#54284=CARTESIAN_POINT ( 'NONE',  ( 4.458734125000001214, -74.14583333196773651, 2.574251347313718519 ) ) ;
#54287=CARTESIAN_POINT ( 'NONE',  ( 0.000000000000000000, -170.0000000000000000, 0.000000000000000000 ) ) ;
#54289=ORIENTED_EDGE ( 'NONE', *, *, #5516, .F. ) ;
#54290=CARTESIAN_POINT ( 'NONE',  ( 6.123233995736766282E-16, -170.0000000000000000, -5.000000000000000000 ) ) ;
#54291=CARTESIAN_POINT ( 'NONE',  ( -4.999999999999998224, -59.91666666666665719, 2.886751345948131764 ) ) ;
#54296=CARTESIAN_POINT ( 'NONE',  ( -3.152548672688508926E-16, 19.18750000136559208, -5.148502694627439702 ) ) ;
#54304=CARTESIAN_POINT ( 'NONE',  ( -3.152548672688508926E-16, 3.437500001365594748, -5.148502694627439702 ) ) ;
#54305=CARTESIAN_POINT ( 'NONE',  ( 4.458734125000000326, -28.14583333196774007, 2.574251347313718519 ) ) ;
#54306=( BOUNDED_CURVE ( )  B_SPLINE_CURVE ( 2, ( #47895, #43076, #56943, #23784, #47590, #37623, #3542, #13808, #62714 ),
 .UNSPECIFIED., .F., .F. ) 
 B_SPLINE_CURVE_WITH_KNOTS ( ( 3, 2, 2, 2, 3 ),
 ( 0.1187500000000000083, 0.1194444444444444503, 0.1208333333333333343, 0.1222222222222222182, 0.1229166666666666741 ),
 .UNSPECIFIED. ) 
 CURVE ( )  GEOMETRIC_REPRESENTATION_ITEM ( )  RATIONAL_B_SPLINE_CURVE ( ( 0.9330127018922194093, 0.9330127018922200755, 1.000000000000000000, 0.8660254037844387076, 1.000000000000000000, 0.8660254037844387076, 1.000000000000000000, 0.9330127018922187432, 0.9330127018922194093 ) ) 
 REPRESENTATION_ITEM ( '' )  );
#54311=CARTESIAN_POINT ( 'NONE',  ( 4.458734124999998549, 24.27083333469892779, -2.574251347313721627 ) ) ;
#54313=EDGE_CURVE ( 'NONE', #61372, #15636, #38327, .T. ) ;
#54316=CARTESIAN_POINT ( 'NONE',  ( -2.229367062499996610, -75.39583333196773651, 3.861377020970582219 ) ) ;
#54318=EDGE_CURVE ( 'NONE', #39123, #62091, #43630, .T. ) ;
#54320=CARTESIAN_POINT ( 'NONE',  ( -5.000000000000000000, 25.04166666939785557, -2.886751345948128211 ) ) ;
#54321=ORIENTED_EDGE ( 'NONE', *, *, #16921, .T. ) ;
#54324=CYLINDRICAL_SURFACE ( 'NONE', #47340, 5.000000000000000000 ) ;
#54325=CARTESIAN_POINT ( 'NONE',  ( -4.999999999999999112, -19.91666666666666785, 2.886751345948131764 ) ) ;
#54326=CARTESIAN_POINT ( 'NONE',  ( 4.458734124999998549, -24.72916666530106866, -2.574251347313721627 ) ) ;
#54327=ADVANCED_FACE ( 'NONE', ( #28041 ), #22281, .T. ) ;
#54328=CARTESIAN_POINT ( 'NONE',  ( -2.229367062499996610, -84.14583333196773651, 3.861377020970582219 ) ) ;
#54329=EDGE_CURVE ( 'NONE', #2707, #55393, #63010, .T. ) ;
#54331=CARTESIAN_POINT ( 'NONE',  ( -2.500000000000000444, -18.04166666393547658, -4.330127018922193649 ) ) ;
#54332=CARTESIAN_POINT ( 'NONE',  ( -2.229367062499996610, -51.14583333196772941, 3.861377020970582219 ) ) ;
#54333=VERTEX_POINT ( 'NONE', #5497 ) ;
#54334=CARTESIAN_POINT ( 'NONE',  ( -6.972266317189433020E-16, -71.12499999726878741, -5.000000000000000000 ) ) ;
#54336=CARTESIAN_POINT ( 'NONE',  ( 2.229367062500001939, 0.7708333346989268975, 3.861377020970579999 ) ) ;
#54337=VERTEX_POINT ( 'NONE', #4538 ) ;
#54340=CARTESIAN_POINT ( 'NONE',  ( 5.000000000000000000, -67.41666666666665719, -2.886751345948129988 ) ) ;
#54342=CARTESIAN_POINT ( 'NONE',  ( 4.458734125000000326, -152.6250000013655495, -1.846868145590734978 ) ) ;
#54344=CARTESIAN_POINT ( 'NONE',  ( -5.000000000000000000, -76.87499999726880162, 0.000000000000000000 ) ) ;
#54345=CARTESIAN_POINT ( 'NONE',  ( -9.184850993605147944E-16, -161.2500000000000000, 5.000000000000000000 ) ) ;
#54346=EDGE_CURVE ( 'NONE', #29467, #9545, #38740, .T. ) ;
#54347=EDGE_CURVE ( 'NONE', #25868, #10085, #19403, .T. ) ;
#54350=CARTESIAN_POINT ( 'NONE',  ( -4.458734124999998549, -11.47916666530107044, 2.574251347313722516 ) ) ;
#54351=CARTESIAN_POINT ( 'NONE',  ( -2.229367062500000163, -46.72916666530106511, -3.861377020970580443 ) ) ;
#54353=CARTESIAN_POINT ( 'NONE',  ( -3.152801135295367096, -148.0625000013655779, -3.152801135295367541 ) ) ;
#54356=ORIENTED_EDGE ( 'NONE', *, *, #61818, .F. ) ;
#54358=CARTESIAN_POINT ( 'NONE',  ( 2.229367062500001939, 28.77083333469892779, 3.861377020970579999 ) ) ;
#54361=( BOUNDED_CURVE ( )  B_SPLINE_CURVE ( 2, ( #26390, #31524, #35404, #26074, #40229, #1973, #50192, #41170, #51166 ),
 .UNSPECIFIED., .F., .F. ) 
 B_SPLINE_CURVE_WITH_KNOTS ( ( 3, 2, 2, 2, 3 ),
 ( 0.5645833333333333259, 0.5652777777777777679, 0.5666666666666666519, 0.5680555555555555358, 0.5687499999999999778 ),
 .UNSPECIFIED. ) 
 CURVE ( )  GEOMETRIC_REPRESENTATION_ITEM ( )  RATIONAL_B_SPLINE_CURVE ( ( 0.9330127018922194093, 0.9330127018922194093, 1.000000000000000000, 0.8660254037844387076, 1.000000000000000000, 0.8660254037844387076, 1.000000000000000000, 0.9330127018922194093, 0.9330127018922194093 ) ) 
 REPRESENTATION_ITEM ( '' )  );
#54362=CARTESIAN_POINT ( 'NONE',  ( -6.972266317189433020E-16, -30.25000000000000000, -5.000000000000000000 ) ) ;
#54366=CARTESIAN_POINT ( 'NONE',  ( 5.000000000000000000, -19.41666666666666785, -2.886751345948130876 ) ) ;
#54368=LINE ( 'NONE', #54033, #10702 ) ;
#54369=CARTESIAN_POINT ( 'NONE',  ( 4.458734124999998549, -4.729166665301071326, -2.574251347313721627 ) ) ;
#54370=CARTESIAN_POINT ( 'NONE',  ( 1.975475456537005874E-15, 1.250000000000000000, 5.000000000000000000 ) ) ;
#54371=CARTESIAN_POINT ( 'NONE',  ( 3.152801135295367541, -149.3125000013655779, -3.152801135295367541 ) ) ;
#54375=DIRECTION ( 'NONE',  ( -0.000000000000000000, 1.000000000000000000, -0.000000000000000000 ) ) ;
#54376=CARTESIAN_POINT ( 'NONE',  ( -6.972266317189433020E-16, -40.24999999999999289, -5.000000000000000000 ) ) ;
#54384=CARTESIAN_POINT ( 'NONE',  ( 1.975475456537005874E-15, -89.62499999726880162, 5.000000000000000000 ) ) ;
#54385=CYLINDRICAL_SURFACE ( 'NONE', #22288, 5.000000000000000000 ) ;
#54386=CARTESIAN_POINT ( 'NONE',  ( -4.458734124999999437, 16.68750000136559564, 0.000000000000000000 ) ) ;
#54388=ORIENTED_EDGE ( 'NONE', *, *, #51926, .F. ) ;
#54389=CARTESIAN_POINT ( 'NONE',  ( 2.229367062499998831, -8.895833331967736513, -3.861377020970580887 ) ) ;
#54391=CARTESIAN_POINT ( 'NONE',  ( 3.535533905932736864, -139.2500000027311842, 3.535533905932738641 ) ) ;
#54396=CARTESIAN_POINT ( 'NONE',  ( -4.458734124999999437, -90.56249999863440792, 0.000000000000000000 ) ) ;
#54398=CARTESIAN_POINT ( 'NONE',  ( -3.152801135295367096, -155.3125000013656063, -3.152801135295367541 ) ) ;
#54400=CARTESIAN_POINT ( 'NONE',  ( 5.000000000000000000, -46.41666666666666430, -2.886751345948130876 ) ) ;
#54405=CARTESIAN_POINT ( 'NONE',  ( 0.000000000000000000, -170.0000000000000000, 0.000000000000000000 ) ) ;
#54406=CARTESIAN_POINT ( 'NONE',  ( -4.999999999999999112, -3.916666666666665630, 2.886751345948131764 ) ) ;
#54408=CARTESIAN_POINT ( 'NONE',  ( -2.229367062500000163, -69.47916666530107932, -3.861377020970580443 ) ) ;
#54410=CARTESIAN_POINT ( 'NONE',  ( 1.060575238724906964E-15, -3.624999997268816276, 5.773502691896257311 ) ) ;
#54411=CARTESIAN_POINT ( 'NONE',  ( -4.458734124999998549, -35.22916666530107221, 2.574251347313722516 ) ) ;
#54415=VERTEX_POINT ( 'NONE', #19012 ) ;
#54416=CARTESIAN_POINT ( 'NONE',  ( -5.147856630858197489E-14, 3.249999999999997335, 5.000000000000000000 ) ) ;
#54417=CARTESIAN_POINT ( 'NONE',  ( -3.535250795749689387E-16, -51.25000000000000000, -5.773502691896257311 ) ) ;
#54419=CARTESIAN_POINT ( 'NONE',  ( 5.000000000000000000, -17.37499999726881583, -6.123233995736766282E-16 ) ) ;
#54421=CARTESIAN_POINT ( 'NONE',  ( -4.999999999999998224, -41.79166666393548013, 2.886751345948131764 ) ) ;
#54422=CARTESIAN_POINT ( 'NONE',  ( 4.458734125000001214, -72.89583333196775072, 2.574251347313718519 ) ) ;
#54423=CARTESIAN_POINT ( 'NONE',  ( 1.846868145590735200, -142.5000000013656347, -4.458734125000000326 ) ) ;
#54424=CARTESIAN_POINT ( 'NONE',  ( 2.229367062499998831, -81.64583333196773651, -3.861377020970580887 ) ) ;
#54426=CARTESIAN_POINT ( 'NONE',  ( 4.458734124999999437, -31.06249999863440436, -5.460374474430324690E-16 ) ) ;
#54427=CARTESIAN_POINT ( 'NONE',  ( 2.499999999999998668, -69.20833333060214443, -4.330127018922193649 ) ) ;
#54429=EDGE_LOOP ( 'NONE', ( #34594, #13620, #20094, #2777 ) ) ;
#54430=CARTESIAN_POINT ( 'NONE',  ( -1.127183054612291972E-14, 24.37500000273118417, 4.999999999999999112 ) ) ;
#54433=CARTESIAN_POINT ( 'NONE',  ( -6.972266317189433020E-16, -21.24999999999999289, -5.000000000000000000 ) ) ;
#54437=CARTESIAN_POINT ( 'NONE',  ( 0.000000000000000000, 30.00000000000000000, 0.000000000000000000 ) ) ;
#54438=CARTESIAN_POINT ( 'NONE',  ( 2.229367062500001939, -58.22916666530107932, 3.861377020970579999 ) ) ;
#54442=DIRECTION ( 'NONE',  ( -0.000000000000000000, 1.000000000000000000, -0.000000000000000000 ) ) ;
#54443=DIRECTION ( 'NONE',  ( -0.000000000000000000, 1.000000000000000000, -0.000000000000000000 ) ) ;
#54444=CARTESIAN_POINT ( 'NONE',  ( 2.229367062500001939, 12.02083333469892601, 3.861377020970579999 ) ) ;
#54447=CARTESIAN_POINT ( 'NONE',  ( 3.152801135295366208, -160.5625000013656063, 3.152801135295367985 ) ) ;
#54448=ORIENTED_EDGE ( 'NONE', *, *, #59868, .F. ) ;
#54450=LINE ( 'NONE', #10378, #6906 ) ;
#54455=CARTESIAN_POINT ( 'NONE',  ( 1.339745962155615144, 4.419658201469705894, 4.999999999999999112 ) ) ;
#54458=CARTESIAN_POINT ( 'NONE',  ( -1.339745962155613812, 5.794658198738519950, -5.000000000000000000 ) ) ;
#54464=CARTESIAN_POINT ( 'NONE',  ( 2.229367062500001939, 5.770833334698927786, 3.861377020970579999 ) ) ;
#54465=CARTESIAN_POINT ( 'NONE',  ( -6.972266317189433020E-16, -10.12499999726881406, -5.000000000000000000 ) ) ;
#54467=CARTESIAN_POINT ( 'NONE',  ( -2.071067811865475061, -148.8125000027312126, -5.000000000000000888 ) ) ;
#54475=CARTESIAN_POINT ( 'NONE',  ( -4.458734124999999437, -164.1875000013655779, -5.460374474430324690E-16 ) ) ;
#54476=CARTESIAN_POINT ( 'NONE',  ( -4.999999999999998224, -32.91666666666666430, 2.886751345948131764 ) ) ;
#54479=CARTESIAN_POINT ( 'NONE',  ( 2.730187237215162345E-16, -144.1875000013656063, -4.458734124999999437 ) ) ;
#54480=ORIENTED_EDGE ( 'NONE', *, *, #16043, .T. ) ;
#54481=CARTESIAN_POINT ( 'NONE',  ( -5.000000000000000000, -89.95833333060214443, -2.886751345948128211 ) ) ;
#54482=ORIENTED_EDGE ( 'NONE', *, *, #98, .F. ) ;
#54483=CARTESIAN_POINT ( 'NONE',  ( 4.458734124999999437, -63.06249999863440792, -5.460374474430324690E-16 ) ) ;
#54485=CYLINDRICAL_SURFACE ( 'NONE', #13453, 5.000000000000000000 ) ;
#54486=CARTESIAN_POINT ( 'NONE',  ( -2.499999999999996447, 16.16666666666666430, 4.330127018922195425 ) ) ;
#54487=CARTESIAN_POINT ( 'NONE',  ( 9.457646018065525792E-16, -49.06249999863440792, 5.148502694627439702 ) ) ;
#54488=CARTESIAN_POINT ( 'NONE',  ( 4.458734124999998549, -4.729166665301071326, -2.574251347313721627 ) ) ;
#54489=CARTESIAN_POINT ( 'NONE',  ( -9.184850993605147944E-16, -166.3750000027312126, 5.000000000000000000 ) ) ;
#54490=CARTESIAN_POINT ( 'NONE',  ( 3.535533905932736864, -165.2500000027312126, 3.535533905932738641 ) ) ;
#54491=CARTESIAN_POINT ( 'NONE',  ( 3.535533905932738197, -158.0000000027312126, -3.535533905932738197 ) ) ;
#54493=CARTESIAN_POINT ( 'NONE',  ( -5.000000000000000000, -10.00000000000000178, 0.000000000000000000 ) ) ;
#54498=CARTESIAN_POINT ( 'NONE',  ( 4.458734124999999437, -51.81249999863440792, -5.460374474430324690E-16 ) ) ;
#54499=CARTESIAN_POINT ( 'NONE',  ( -4.458734125000001214, -154.1250000013656063, 1.846868145590734089 ) ) ;
#54500=VECTOR ( 'NONE', #10954, 1000.000000000000000 ) ;
#54501=CARTESIAN_POINT ( 'NONE',  ( -4.999999999999999112, -54.79166666393547303, 2.886751345948131764 ) ) ;
#54504=CARTESIAN_POINT ( 'NONE',  ( -2.229367062500000163, 4.270833334698926897, -3.861377020970580443 ) ) ;
#54505=VERTEX_POINT ( 'NONE', #39576 ) ;
#54508=CARTESIAN_POINT ( 'NONE',  ( 4.458734125000000326, -157.3750000013656347, -1.846868145590734978 ) ) ;
#54509=ORIENTED_EDGE ( 'NONE', *, *, #1565, .F. ) ;
#54513=CARTESIAN_POINT ( 'NONE',  ( -6.972266317189433020E-16, -47.25000000000000000, -5.000000000000000000 ) ) ;
#54514=CARTESIAN_POINT ( 'NONE',  ( 9.457646018065525792E-16, -43.31249999863440792, 5.148502694627439702 ) ) ;
#54515=VERTEX_POINT ( 'NONE', #29283 ) ;
#54516=CARTESIAN_POINT ( 'NONE',  ( 5.275681513340003914E-14, 9.875000002731184168, -5.000000000000000000 ) ) ;
#54518=CARTESIAN_POINT ( 'NONE',  ( -3.152548672688508926E-16, 27.43750000136559564, -5.148502694627439702 ) ) ;
#54521=CARTESIAN_POINT ( 'NONE',  ( -5.000000000000000000, -35.95833333060213732, -2.886751345948128211 ) ) ;
#54527=CARTESIAN_POINT ( 'NONE',  ( -4.999999999999998224, 7.083333333333333925, 2.886751345948131764 ) ) ;
#54531=CYLINDRICAL_SURFACE ( 'NONE', #29613, 5.000000000000000000 ) ;
#54533=CARTESIAN_POINT ( 'NONE',  ( 0.000000000000000000, -170.0000000000000000, 0.000000000000000000 ) ) ;
#54538=CARTESIAN_POINT ( 'NONE',  ( 3.535533905932738197, -160.0000000027312126, -3.535533905932738197 ) ) ;
#54541=CARTESIAN_POINT ( 'NONE',  ( -4.999999999999998224, 22.08333333333333215, 2.886751345948131764 ) ) ;
#54548=CARTESIAN_POINT ( 'NONE',  ( -5.000000000000000000, -141.6250000027312126, -6.123233995736766282E-16 ) ) ;
#54549=CARTESIAN_POINT ( 'NONE',  ( -4.458734124999997661, -19.22916666530106866, 2.574251347313722516 ) ) ;
#54550=CYLINDRICAL_SURFACE ( 'NONE', #53765, 5.000000000000000000 ) ;
#54551=CARTESIAN_POINT ( 'NONE',  ( -3.535533905932737309, -156.6250000000000000, -3.535533905932738197 ) ) ;
#54553=CARTESIAN_POINT ( 'NONE',  ( -3.152801135295367985, -157.8125000013656063, 3.152801135295367096 ) ) ;
#54555=CARTESIAN_POINT ( 'NONE',  ( -4.458734124999999437, -44.56249999863440081, 0.000000000000000000 ) ) ;
#54556=CARTESIAN_POINT ( 'NONE',  ( 5.000000000000000000, -44.37499999726880873, -6.123233995736766282E-16 ) ) ;
#54558=CARTESIAN_POINT ( 'NONE',  ( 2.229367062499998831, -88.64583333196773651, -3.861377020970580887 ) ) ;
#54561=CARTESIAN_POINT ( 'NONE',  ( -3.152548672688508926E-16, 10.43750000136559386, -5.148502694627439702 ) ) ;
#54565=CARTESIAN_POINT ( 'NONE',  ( 4.458734124999998549, 20.02083333469892779, -2.574251347313721627 ) ) ;
#54567=CARTESIAN_POINT ( 'NONE',  ( 2.500000000000002220, 6.458333336064519870, 4.330127018922192761 ) ) ;
#54572=CARTESIAN_POINT ( 'NONE',  ( -3.152548672688508926E-16, -37.56249999863440792, -5.148502694627439702 ) ) ;
#54573=CARTESIAN_POINT ( 'NONE',  ( 5.000000000000000000, -38.29166666393548013, -2.886751345948129988 ) ) ;
#54575=CARTESIAN_POINT ( 'NONE',  ( -4.458734124999998549, -10.22916666530106866, 2.574251347313722516 ) ) ;
#54576=CARTESIAN_POINT ( 'NONE',  ( -2.229367062500000163, -20.72916666530107221, -3.861377020970580443 ) ) ;
#54577=ORIENTED_EDGE ( 'NONE', *, *, #31974, .T. ) ;
#54578=CARTESIAN_POINT ( 'NONE',  ( 5.000000000000000000, -84.49999999999998579, -6.123233995736766282E-16 ) ) ;
#54579=CARTESIAN_POINT ( 'NONE',  ( -3.152801135295367096, -169.0625000013656063, -3.152801135295367541 ) ) ;
#54581=CARTESIAN_POINT ( 'NONE',  ( 5.000000000000000000, -86.37499999726880162, -6.123233995736766282E-16 ) ) ;
#54582=CARTESIAN_POINT ( 'NONE',  ( -6.972266317189433020E-16, -18.25000000000000000, -5.000000000000000000 ) ) ;
#54584=VECTOR ( 'NONE', #43280, 1000.000000000000000 ) ;
#54586=CARTESIAN_POINT ( 'NONE',  ( 9.457646018065525792E-16, -27.31249999863440436, 5.148502694627439702 ) ) ;
#54587=CARTESIAN_POINT ( 'NONE',  ( 1.975475456537005874E-15, 7.375000002731185944, 5.000000000000000000 ) ) ;
#54590=CARTESIAN_POINT ( 'NONE',  ( 1.846868145590736310, -162.8750000013655779, 4.458734124999999437 ) ) ;
#54593=VERTEX_POINT ( 'NONE', #46328 ) ;
#54595=CARTESIAN_POINT ( 'NONE',  ( -4.458734124999998549, -73.47916666530106511, 2.574251347313722516 ) ) ;
#54598=CARTESIAN_POINT ( 'NONE',  ( -4.458734124999999437, -147.2500000013656063, -1.846868145590735644 ) ) ;
#54599=CARTESIAN_POINT ( 'NONE',  ( -5.000000000000000000, 23.00000000000000000, 0.000000000000000000 ) ) ;
#54604=CARTESIAN_POINT ( 'NONE',  ( 3.152801135295367541, -141.5625000013655779, -3.152801135295367541 ) ) ;
#54609=CARTESIAN_POINT ( 'NONE',  ( 4.458734124999999437, -76.06249999863440792, -5.460374474430324690E-16 ) ) ;
#54611=CARTESIAN_POINT ( 'NONE',  ( 3.061616997868383141E-16, -149.8750000027312126, -5.000000000000000000 ) ) ;
#54619=EDGE_CURVE ( 'NONE', #15810, #35184, #20622, .T. ) ;
#54622=CARTESIAN_POINT ( 'NONE',  ( 4.458734124999998549, 18.02083333469892779, -2.574251347313721627 ) ) ;
#54630=CARTESIAN_POINT ( 'NONE',  ( 2.229367062500001939, -5.979166665301072214, 3.861377020970579999 ) ) ;
#54631=CARTESIAN_POINT ( 'NONE',  ( -2.229367062499996610, -31.39583333196773651, 3.861377020970582219 ) ) ;
#54635=( BOUNDED_CURVE ( )  B_SPLINE_CURVE ( 2, ( #47029, #3294, #27717, #11646, #26775, #61835, #46394, #11966, #2342 ),
 .UNSPECIFIED., .F., .F. ) 
 B_SPLINE_CURVE_WITH_KNOTS ( ( 3, 2, 2, 2, 3 ),
 ( 0.9020833333333333481, 0.9027777777777777901, 0.9041666666666666741, 0.9055555555555555580, 0.9062500000000000000 ),
 .UNSPECIFIED. ) 
 CURVE ( )  GEOMETRIC_REPRESENTATION_ITEM ( )  RATIONAL_B_SPLINE_CURVE ( ( 0.9330127018922194093, 0.9330127018922194093, 1.000000000000000000, 0.8660254037844387076, 1.000000000000000000, 0.8660254037844387076, 1.000000000000000000, 0.9330127018922194093, 0.9330127018922194093 ) ) 
 REPRESENTATION_ITEM ( '' )  );
#54636=CARTESIAN_POINT ( 'NONE',  ( -4.458734124999999437, 23.60416666803225993, -2.574251347313719407 ) ) ;
#54638=DIRECTION ( 'NONE',  ( 0.000000000000000000, 0.000000000000000000, 1.000000000000000000 ) ) ;
#54639=CARTESIAN_POINT ( 'NONE',  ( 4.458734124999999437, -79.06249999863440792, -5.460374474430324690E-16 ) ) ;
#54642=CARTESIAN_POINT ( 'NONE',  ( -4.999999999999999112, 22.20833333606451987, 2.886751345948131764 ) ) ;
#54645=DIRECTION ( 'NONE',  ( 0.000000000000000000, 0.000000000000000000, 1.000000000000000000 ) ) ;
#54646=CARTESIAN_POINT ( 'NONE',  ( -5.000000000000000000, -19.99999999999999645, 0.000000000000000000 ) ) ;
#54647=CARTESIAN_POINT ( 'NONE',  ( 4.458734124999999437, -21.81249999863440436, -5.460374474430324690E-16 ) ) ;
#54648=CARTESIAN_POINT ( 'NONE',  ( 4.458734124999998549, -80.72916666530106511, -2.574251347313721627 ) ) ;
#54649=CARTESIAN_POINT ( 'NONE',  ( -2.500000000000000444, -24.04166666393548368, -4.330127018922193649 ) ) ;
#54651=CARTESIAN_POINT ( 'NONE',  ( 4.458734125000001214, -51.89583333196773651, 2.574251347313718519 ) ) ;
#54654=CYLINDRICAL_SURFACE ( 'NONE', #39518, 5.000000000000000000 ) ;
#54655=CARTESIAN_POINT ( 'NONE',  ( -2.229367062499996610, 2.604166668032259491, 3.861377020970582219 ) ) ;
#54658=CARTESIAN_POINT ( 'NONE',  ( -2.500000000000000444, -68.16666666666667140, -4.330127018922193649 ) ) ;
#54659=CARTESIAN_POINT ( 'NONE',  ( 2.730187237215162345E-16, -153.4375000013655779, -4.458734124999999437 ) ) ;
#54661=CARTESIAN_POINT ( 'NONE',  ( -6.972266317189433020E-16, -77.12499999726881583, -5.000000000000000000 ) ) ;
#54662=CARTESIAN_POINT ( 'NONE',  ( 2.071067811865476394, -158.1875000000000000, 5.000000000000000000 ) ) ;
#54665=CARTESIAN_POINT ( 'NONE',  ( 9.457646018065525792E-16, -11.31249999863440792, 5.148502694627439702 ) ) ;
#54666=CARTESIAN_POINT ( 'NONE',  ( -2.229367062500000163, -44.72916666530106511, -3.861377020970580443 ) ) ;
#54667=CARTESIAN_POINT ( 'NONE',  ( -1.339745962155610925, -7.669658196007332229, 5.000000000000000000 ) ) ;
#54668=CARTESIAN_POINT ( 'NONE',  ( 4.458734124999999437, -143.5000000013656063, 1.846868145590737864 ) ) ;
#54670=CARTESIAN_POINT ( 'NONE',  ( -9.184850993605147944E-16, -151.3750000027311842, 5.000000000000000000 ) ) ;
#54673=CARTESIAN_POINT ( 'NONE',  ( -4.458734124999998549, 28.52083333469892423, 2.574251347313722516 ) ) ;
#54675=CARTESIAN_POINT ( 'NONE',  ( 5.000000000000000000, -30.50000000000000000, -6.123233995736766282E-16 ) ) ;
#54676=VERTEX_POINT ( 'NONE', #12235 ) ;
#54679=EDGE_CURVE ( 'NONE', #6968, #60408, #23176, .T. ) ;
#54682=( BOUNDED_CURVE ( )  B_SPLINE_CURVE ( 2, ( #38285, #13532, #24122, #63674, #24434, #53701, #4494, #9318, #57605 ),
 .UNSPECIFIED., .F., .F. ) 
 B_SPLINE_CURVE_WITH_KNOTS ( ( 3, 2, 2, 2, 3 ),
 ( 0.7895833333333333037, 0.7902777777777777457, 0.7916666666666666297, 0.7930555555555555136, 0.7937499999999999556 ),
 .UNSPECIFIED. ) 
 CURVE ( )  GEOMETRIC_REPRESENTATION_ITEM ( )  RATIONAL_B_SPLINE_CURVE ( ( 0.9330127018922194093, 0.9330127018922194093, 1.000000000000000000, 0.8660254037844387076, 1.000000000000000000, 0.8660254037844387076, 1.000000000000000000, 0.9330127018922194093, 0.9330127018922194093 ) ) 
 REPRESENTATION_ITEM ( '' )  );
#54683=EDGE_CURVE ( 'NONE', #44005, #11078, #54361, .T. ) ;
#54684=CARTESIAN_POINT ( 'NONE',  ( -1.339745962155636017, 2.330341803992663774, 4.999999999999985789 ) ) ;
#54685=CARTESIAN_POINT ( 'NONE',  ( 2.229367062499998831, -1.645833331967737401, -3.861377020970580887 ) ) ;
#54686=CARTESIAN_POINT ( 'NONE',  ( 2.500000000000002220, -73.54166666393548724, 4.330127018922192761 ) ) ;
#54687=CARTESIAN_POINT ( 'NONE',  ( -3.152801135295367985, -150.8125000013655779, 3.152801135295367096 ) ) ;
#54688=( BOUNDED_CURVE ( )  B_SPLINE_CURVE ( 2, ( #6638, #50695, #31382, #61313, #56492, #23021, #32025, #18183, #12413 ),
 .UNSPECIFIED., .F., .F. ) 
 B_SPLINE_CURVE_WITH_KNOTS ( ( 3, 2, 2, 2, 3 ),
 ( 0.01041666666666666782, 0.01111111111111111154, 0.01250000000000000069, 0.01388888888888888812, 0.01458333333333333356 ),
 .UNSPECIFIED. ) 
 CURVE ( )  GEOMETRIC_REPRESENTATION_ITEM ( )  RATIONAL_B_SPLINE_CURVE ( ( 0.9330127018922192983, 0.9330127018922194093, 1.000000000000000000, 0.8660254037844387076, 1.000000000000000000, 0.8660254037844387076, 1.000000000000000000, 0.9330127018922191873, 0.9330127018922192983 ) ) 
 REPRESENTATION_ITEM ( '' )  );
#54703=EDGE_CURVE ( 'NONE', #9342, #29478, #60950, .T. ) ;
#54704=CARTESIAN_POINT ( 'NONE',  ( 1.975475456537005874E-15, 9.250000000000000000, 5.000000000000000000 ) ) ;
#54705=CARTESIAN_POINT ( 'NONE',  ( -4.458734124999999437, 11.68750000136559564, 0.000000000000000000 ) ) ;
#54708=CARTESIAN_POINT ( 'NONE',  ( -2.229367062500000163, -11.72916666530107044, -3.861377020970580443 ) ) ;
#54710=CARTESIAN_POINT ( 'NONE',  ( -3.152801135295367096, -163.0625000013656063, -3.152801135295367541 ) ) ;
#54712=EDGE_CURVE ( 'NONE', #26438, #24132, #37620, .T. ) ;
#54720=CARTESIAN_POINT ( 'NONE',  ( 4.458734124999999437, -154.6250000013655779, -1.846868145590734978 ) ) ;
#54727=CARTESIAN_POINT ( 'NONE',  ( -5.000000000000000000, -8.874999997268814056, 0.000000000000000000 ) ) ;
#54728=CARTESIAN_POINT ( 'NONE',  ( 2.500000000000002220, -2.666666666666664298, 4.330127018922192761 ) ) ;
#54729=CARTESIAN_POINT ( 'NONE',  ( -4.458734124999999437, -68.31249999863439371, 0.000000000000000000 ) ) ;
#54731=CARTESIAN_POINT ( 'NONE',  ( -5.000000000000000000, -5.874999997268811391, 0.000000000000000000 ) ) ;
#54732=CARTESIAN_POINT ( 'NONE',  ( 4.458734124999998549, -31.72916666530107577, -2.574251347313721627 ) ) ;
#54733=ORIENTED_EDGE ( 'NONE', *, *, #4797, .T. ) ;
#54736=EDGE_LOOP ( 'NONE', ( #55812, #13290, #56807, #32247 ) ) ;
#54738=CARTESIAN_POINT ( 'NONE',  ( -4.999999999999999112, -50.91666666666667140, 2.886751345948131764 ) ) ;
#54741=CARTESIAN_POINT ( 'NONE',  ( 1.975475456537005874E-15, -4.624999997268815832, 5.000000000000000000 ) ) ;
#54742=CARTESIAN_POINT ( 'NONE',  ( 4.458734125000001214, -74.89583333196773651, 2.574251347313718519 ) ) ;
#54743=( BOUNDED_CURVE ( )  B_SPLINE_CURVE ( 2, ( #42382, #52367, #60608, #35835, #11057, #55130, #6247, #1437, #45473 ),
 .UNSPECIFIED., .F., .F. ) 
 B_SPLINE_CURVE_WITH_KNOTS ( ( 3, 2, 2, 2, 3 ),
 ( 0.5312500000000000000, 0.5319444444444444420, 0.5333333333333333259, 0.5347222222222222099, 0.5354166666666666519 ),
 .UNSPECIFIED. ) 
 CURVE ( )  GEOMETRIC_REPRESENTATION_ITEM ( )  RATIONAL_B_SPLINE_CURVE ( ( 0.9330127018922194093, 0.9330127018922194093, 1.000000000000000000, 0.8660254037844387076, 1.000000000000000000, 0.8660254037844387076, 1.000000000000000000, 0.9330127018922194093, 0.9330127018922194093 ) ) 
 REPRESENTATION_ITEM ( '' )  );
#54744=CARTESIAN_POINT ( 'NONE',  ( 3.152801135295366208, -145.8125000013655779, 3.152801135295367985 ) ) ;
#54745=CARTESIAN_POINT ( 'NONE',  ( -2.229367062499996610, -84.14583333196773651, 3.861377020970582219 ) ) ;
#54747=CARTESIAN_POINT ( 'NONE',  ( -3.152548672688508926E-16, -29.81249999863440436, -5.148502694627439702 ) ) ;
#54749=DIRECTION ( 'NONE',  ( 0.000000000000000000, 0.000000000000000000, 1.000000000000000000 ) ) ;
#54750=ORIENTED_EDGE ( 'NONE', *, *, #27180, .F. ) ;
#54756=CARTESIAN_POINT ( 'NONE',  ( 9.457646018065525792E-16, -62.31249999863440792, 5.148502694627439702 ) ) ;
#54758=ORIENTED_EDGE ( 'NONE', *, *, #52004, .T. ) ;
#54759=EDGE_CURVE ( 'NONE', #46916, #59564, #52431, .T. ) ;
#54760=CARTESIAN_POINT ( 'NONE',  ( 1.339745962155615144, -62.70534180126146850, 4.999999999999999112 ) ) ;
#54762=CARTESIAN_POINT ( 'NONE',  ( 2.229367062500001939, 11.02083333469892956, 3.861377020970579999 ) ) ;
#54764=CARTESIAN_POINT ( 'NONE',  ( 1.339745962155615144, -24.70534180126147561, 4.999999999999999112 ) ) ;
#54765=CARTESIAN_POINT ( 'NONE',  ( 4.458734124999997661, -160.5000000013656347, 1.846868145590737864 ) ) ;
#54766=ORIENTED_EDGE ( 'NONE', *, *, #45686, .F. ) ;
#54770=CARTESIAN_POINT ( 'NONE',  ( 0.000000000000000000, -170.0000000000000000, 0.000000000000000000 ) ) ;
#54771=CARTESIAN_POINT ( 'NONE',  ( -6.972266317189433020E-16, -36.25000000000000000, -5.000000000000000000 ) ) ;
#54774=CARTESIAN_POINT ( 'NONE',  ( -5.000000000000000000, -72.95833333060214443, -2.886751345948128211 ) ) ;
#54778=EDGE_CURVE ( 'NONE', #6544, #22858, #10391, .T. ) ;
#54781=CARTESIAN_POINT ( 'NONE',  ( -4.458734124999997661, -0.4791666653010707710, 2.574251347313722516 ) ) ;
#54782=CARTESIAN_POINT ( 'NONE',  ( -5.000000000000000888, -161.6875000027311842, -2.071067811865475949 ) ) ;
#54784=EDGE_CURVE ( 'NONE', #35059, #13136, #36329, .T. ) ;
#54785=CARTESIAN_POINT ( 'NONE',  ( 3.535533905932736864, -145.2500000027311842, 3.535533905932738641 ) ) ;
#54795=CARTESIAN_POINT ( 'NONE',  ( 3.152801135295367541, -164.5625000013656063, -3.152801135295367541 ) ) ;
#54796=CARTESIAN_POINT ( 'NONE',  ( 1.975475456537005874E-15, -32.74999999999999289, 5.000000000000000000 ) ) ;
#54797=CARTESIAN_POINT ( 'NONE',  ( -3.535533905932738641, -159.5000000027312126, 3.535533905932737309 ) ) ;
#54799=CARTESIAN_POINT ( 'NONE',  ( 1.846868145590736310, -144.6250000013655779, 4.458734124999999437 ) ) ;
#54800=ORIENTED_EDGE ( 'NONE', *, *, #11135, .T. ) ;
#54801=CARTESIAN_POINT ( 'NONE',  ( -4.458734124999999437, 23.43750000136559564, 0.000000000000000000 ) ) ;
#54803=CARTESIAN_POINT ( 'NONE',  ( 2.229367062500001939, -64.22916666530106511, 3.861377020970579999 ) ) ;
#54805=DIRECTION ( 'NONE',  ( -0.000000000000000000, 1.000000000000000000, -0.000000000000000000 ) ) ;
#54806=CARTESIAN_POINT ( 'NONE',  ( 5.000000000000000888, 13.41666666666666607, 2.886751345948126879 ) ) ;
#54807=CARTESIAN_POINT ( 'NONE',  ( 4.458734124999998549, -49.72916666530107221, -2.574251347313721627 ) ) ;
#54808=CARTESIAN_POINT ( 'NONE',  ( -2.229367062499996610, -9.145833331967736513, 3.861377020970582219 ) ) ;
#54809=DIRECTION ( 'NONE',  ( 0.000000000000000000, 0.000000000000000000, 1.000000000000000000 ) ) ;
#54811=CARTESIAN_POINT ( 'NONE',  ( -1.339745962155610925, -9.794658198738520838, 5.000000000000000000 ) ) ;
#54814=CARTESIAN_POINT ( 'NONE',  ( 1.975475456537005874E-15, -31.62499999726880873, 5.000000000000000000 ) ) ;
#54815=CARTESIAN_POINT ( 'NONE',  ( -3.152548672688508926E-16, -58.56249999863440081, -5.148502694627439702 ) ) ;
#54816=CARTESIAN_POINT ( 'NONE',  ( -4.458734125000000326, -157.2500000013656063, -1.846868145590735644 ) ) ;
#54818=CARTESIAN_POINT ( 'NONE',  ( 2.500000000000002220, -56.54166666393548013, 4.330127018922192761 ) ) ;
#54819=EDGE_LOOP ( 'NONE', ( #37121, #17952, #59552, #25301 ) ) ;
#54820=DIRECTION ( 'NONE',  ( 0.000000000000000000, 0.000000000000000000, 1.000000000000000000 ) ) ;
#54821=CARTESIAN_POINT ( 'NONE',  ( -4.458734124999998549, 0.5208333346989265644, 2.574251347313722516 ) ) ;
#54825=CARTESIAN_POINT ( 'NONE',  ( 1.846868145590736310, -156.6250000013655779, 4.458734124999999437 ) ) ;
#54826=ORIENTED_EDGE ( 'NONE', *, *, #11108, .F. ) ;
#54827=CARTESIAN_POINT ( 'NONE',  ( -1.127183054612291972E-14, 25.24999999999999645, 4.999999999999999112 ) ) ;
#54829=CARTESIAN_POINT ( 'NONE',  ( 3.535533905932738197, -152.8750000000000000, -3.535533905932738197 ) ) ;
#54830=CARTESIAN_POINT ( 'NONE',  ( -3.152548672688508926E-16, -43.81249999863440081, -5.148502694627439702 ) ) ;
#54831=ORIENTED_EDGE ( 'NONE', *, *, #24849, .T. ) ;
#54832=ADVANCED_FACE ( 'NONE', ( #33118 ), #47281, .T. ) ;
#54833=( BOUNDED_CURVE ( )  B_SPLINE_CURVE ( 2, ( #16759, #11287, #1989, #25779, #26732, #20958, #6483, #35115, #16443 ),
 .UNSPECIFIED., .F., .F. ) 
 B_SPLINE_CURVE_WITH_KNOTS ( ( 3, 2, 2, 2, 3 ),
 ( 0.4270833333333333148, 0.4277777777777777568, 0.4291666666666666408, 0.4305555555555555802, 0.4312500000000000222 ),
 .UNSPECIFIED. ) 
 CURVE ( )  GEOMETRIC_REPRESENTATION_ITEM ( )  RATIONAL_B_SPLINE_CURVE ( ( 0.9330127018922194093, 0.9330127018922194093, 1.000000000000000000, 0.8660254037844387076, 1.000000000000000000, 0.8660254037844387076, 1.000000000000000000, 0.9330127018922194093, 0.9330127018922194093 ) ) 
 REPRESENTATION_ITEM ( '' )  );
#54834=CARTESIAN_POINT ( 'NONE',  ( -1.339745962155610925, -45.79465819873851729, 5.000000000000000000 ) ) ;
#54836=CARTESIAN_POINT ( 'NONE',  ( 2.229367062500001939, -90.22916666530106511, 3.861377020970579999 ) ) ;
#54839=CARTESIAN_POINT ( 'NONE',  ( -4.999999999999998224, -35.79166666393547303, 2.886751345948131764 ) ) ;
#54840=CARTESIAN_POINT ( 'NONE',  ( 3.061616997868383141E-16, -159.8750000027311842, -5.000000000000000000 ) ) ;
#54844=CARTESIAN_POINT ( 'NONE',  ( 0.000000000000000000, -170.0000000000000000, 0.000000000000000000 ) ) ;
#54845=CARTESIAN_POINT ( 'NONE',  ( -4.999999999999998224, -26.91666666666666430, 2.886751345948131764 ) ) ;
#54848=CARTESIAN_POINT ( 'NONE',  ( -5.000000000000000000, -19.95833333060214798, -2.886751345948128211 ) ) ;
#54849=CARTESIAN_POINT ( 'NONE',  ( -3.152548672688508926E-16, -89.81249999863439371, -5.148502694627439702 ) ) ;
#54852=ORIENTED_EDGE ( 'NONE', *, *, #18499, .F. ) ;
#54853=CARTESIAN_POINT ( 'NONE',  ( -5.000000000000000888, -169.5625000000000284, -2.071067811865475949 ) ) ;
#54855=CARTESIAN_POINT ( 'NONE',  ( 5.000000000000000000, -161.1875000027312126, 2.071067811865478614 ) ) ;
#54867=CARTESIAN_POINT ( 'NONE',  ( -2.229367062499996610, -20.14583333196774007, 3.861377020970582219 ) ) ;
#54869=CARTESIAN_POINT ( 'NONE',  ( 5.000000000000000000, -154.0625000000000284, 2.071067811865478614 ) ) ;
#54871=CARTESIAN_POINT ( 'NONE',  ( 3.152801135295366208, -154.5625000013656063, 3.152801135295367985 ) ) ;
#54873=CARTESIAN_POINT ( 'NONE',  ( -2.229367062500000163, -45.72916666530106511, -3.861377020970580443 ) ) ;
#54876=CARTESIAN_POINT ( 'NONE',  ( -5.000000000000000000, 29.91666666666666430, -2.886751345948128211 ) ) ;
#54878=CARTESIAN_POINT ( 'NONE',  ( 2.229367062500001939, 7.020833334698928674, 3.861377020970579999 ) ) ;
#54881=CARTESIAN_POINT ( 'NONE',  ( 1.339745962155565406, -17.70534180126147916, 5.000000000000028422 ) ) ;
#54882=CARTESIAN_POINT ( 'NONE',  ( 2.229367062499998831, 23.10416666803225993, -3.861377020970580887 ) ) ;
#54884=CARTESIAN_POINT ( 'NONE',  ( -5.000000000000000000, 6.041666669397850242, -2.886751345948128211 ) ) ;
#54886=LINE ( 'NONE', #20154, #62324 ) ;
#54888=( BOUNDED_CURVE ( )  B_SPLINE_CURVE ( 2, ( #46774, #32293, #56442, #13309, #51919, #22018, #17186, #22661, #52237 ),
 .UNSPECIFIED., .F., .F. ) 
 B_SPLINE_CURVE_WITH_KNOTS ( ( 3, 2, 2, 2, 3 ),
 ( 0.1583333333333334925, 0.1625000000000001721, 0.1666666666666668239, 0.1708333333333335036, 0.1750000000000001554 ),
 .UNSPECIFIED. ) 
 CURVE ( )  GEOMETRIC_REPRESENTATION_ITEM ( )  RATIONAL_B_SPLINE_CURVE ( ( 0.9999999999999970024, 0.9238795325112897361, 1.000000000000000000, 0.9238795325112867385, 1.000000000000000000, 0.9238795325112867385, 1.000000000000000000, 0.9238795325112837409, 1.000000000000003109 ) ) 
 REPRESENTATION_ITEM ( '' )  );
#54889=DIRECTION ( 'NONE',  ( -0.000000000000000000, 1.000000000000000000, -0.000000000000000000 ) ) ;
#54890=CARTESIAN_POINT ( 'NONE',  ( 9.457646018065525792E-16, -37.06249999863440792, 5.148502694627439702 ) ) ;
#54891=EDGE_CURVE ( 'NONE', #57597, #5493, #10770, .T. ) ;
#54892=CARTESIAN_POINT ( 'NONE',  ( 5.000000000000000000, -41.37499999726880162, -6.123233995736766282E-16 ) ) ;
#54894=CARTESIAN_POINT ( 'NONE',  ( 2.229367062500001939, -12.97916666530107221, 3.861377020970579999 ) ) ;
#54895=VERTEX_POINT ( 'NONE', #22848 ) ;
#54896=CARTESIAN_POINT ( 'NONE',  ( 5.000000000000000888, -84.58333333333332860, 2.886751345948126879 ) ) ;
#54897=CARTESIAN_POINT ( 'NONE',  ( 1.846868145590735200, -169.2500000013655779, -4.458734125000000326 ) ) ;
#54899=CARTESIAN_POINT ( 'NONE',  ( 5.000000000000000000, -89.37499999726880162, -6.123233995736766282E-16 ) ) ;
#54901=VERTEX_POINT ( 'NONE', #42438 ) ;
#54903=CARTESIAN_POINT ( 'NONE',  ( 4.458734125000001214, -26.14583333196774007, 2.574251347313718519 ) ) ;
#54904=CARTESIAN_POINT ( 'NONE',  ( -4.999999999999998224, -49.91666666666667140, 2.886751345948131764 ) ) ;
#54907=CARTESIAN_POINT ( 'NONE',  ( -1.846868145590734756, -162.3750000013655779, -4.458734125000000326 ) ) ;
#54909=CARTESIAN_POINT ( 'NONE',  ( 2.500000000000002220, -23.66666666666666785, 4.330127018922192761 ) ) ;
#54912=CARTESIAN_POINT ( 'NONE',  ( 4.458734124999999437, -77.06249999863440792, -5.460374474430324690E-16 ) ) ;
#54915=CARTESIAN_POINT ( 'NONE',  ( -1.846868145590734756, -142.3750000013656063, -4.458734124999999437 ) ) ;
#54916=( BOUNDED_CURVE ( )  B_SPLINE_CURVE ( 2, ( #59012, #14943, #34551, #2102, #41295, #1777, #60629, #16548, #45494 ),
 .UNSPECIFIED., .F., .F. ) 
 B_SPLINE_CURVE_WITH_KNOTS ( ( 3, 2, 2, 2, 3 ),
 ( 0.8083333333333331261, 0.8124999999999997780, 0.8166666666666664298, 0.8208333333333330817, 0.8249999999999997335 ),
 .UNSPECIFIED. ) 
 CURVE ( )  GEOMETRIC_REPRESENTATION_ITEM ( )  RATIONAL_B_SPLINE_CURVE ( ( 1.000000000000003997, 0.9238795325112826307, 1.000000000000000000, 0.9238795325112867385, 1.000000000000000000, 0.9238795325112867385, 1.000000000000000000, 0.9238795325112908463, 0.9999999999999958922 ) ) 
 REPRESENTATION_ITEM ( '' )  );
#54922=AXIS2_PLACEMENT_3D ( 'NONE', #30596, #6167, #36067 ) ;
#54923=CARTESIAN_POINT ( 'NONE',  ( -3.152801135295367096, -140.3125000013655779, -3.152801135295367541 ) ) ;
#54926=CARTESIAN_POINT ( 'NONE',  ( -6.972266317189433020E-16, -72.12499999726878741, -5.000000000000000000 ) ) ;
#54928=CARTESIAN_POINT ( 'NONE',  ( -4.458734124999999437, -72.64583333196773651, -2.574251347313719407 ) ) ;
#54929=CARTESIAN_POINT ( 'NONE',  ( -6.972266317189433020E-16, -65.24999999999998579, -5.000000000000000000 ) ) ;
#54931=DIRECTION ( 'NONE',  ( 0.000000000000000000, 0.000000000000000000, 1.000000000000000000 ) ) ;
#54934=DIRECTION ( 'NONE',  ( -0.000000000000000000, 1.000000000000000000, -0.000000000000000000 ) ) ;
#54935=CARTESIAN_POINT ( 'NONE',  ( 2.499999999999998668, -15.33333333333333037, -4.330127018922193649 ) ) ;
#54940=CARTESIAN_POINT ( 'NONE',  ( 2.229367062500001939, 15.77083333469892601, 3.861377020970579999 ) ) ;
#54947=CARTESIAN_POINT ( 'NONE',  ( -2.229367062499996610, -87.14583333196773651, 3.861377020970582219 ) ) ;
#54948=CARTESIAN_POINT ( 'NONE',  ( 4.458734124999999437, -2.812499998634407472, -5.460374474430324690E-16 ) ) ;
#54949=CARTESIAN_POINT ( 'NONE',  ( -2.229367062500000163, -27.72916666530107221, -3.861377020970580443 ) ) ;
#54953=CARTESIAN_POINT ( 'NONE',  ( -4.458734124999999437, 24.60416666803225993, -2.574251347313719407 ) ) ;
#54956=CARTESIAN_POINT ( 'NONE',  ( 2.229367062499998831, -76.89583333196773651, -3.861377020970580887 ) ) ;
#54959=CARTESIAN_POINT ( 'NONE',  ( -3.535250795749689387E-16, 24.87500000273118417, -5.773502691896257311 ) ) ;
#54963=DIRECTION ( 'NONE',  ( 0.000000000000000000, 0.000000000000000000, 1.000000000000000000 ) ) ;
#54964=CARTESIAN_POINT ( 'NONE',  ( -5.000000000000000000, -20.99999999999999645, 0.000000000000000000 ) ) ;
#54965=CARTESIAN_POINT ( 'NONE',  ( 4.458734124999998549, -21.72916666530107221, -2.574251347313721627 ) ) ;
#54966=EDGE_CURVE ( 'NONE', #20646, #61326, #37097, .T. ) ;
#54967=CARTESIAN_POINT ( 'NONE',  ( 4.458734124999999437, -84.81249999863439371, -5.460374474430324690E-16 ) ) ;
#54969=CARTESIAN_POINT ( 'NONE',  ( -2.499999999999996447, -24.70833333060214443, 4.330127018922195425 ) ) ;
#54970=CARTESIAN_POINT ( 'NONE',  ( -3.152548672688508926E-16, -47.56249999863440792, -5.148502694627439702 ) ) ;
#54973=CARTESIAN_POINT ( 'NONE',  ( -2.229367062500000163, -5.729166665301072214, -3.861377020970580443 ) ) ;
#54976=CARTESIAN_POINT ( 'NONE',  ( -2.500000000000000444, -65.16666666666667140, -4.330127018922193649 ) ) ;
#54977=CARTESIAN_POINT ( 'NONE',  ( -3.152801135295367985, -153.0625000013656063, 3.152801135295367096 ) ) ;
#54980=CARTESIAN_POINT ( 'NONE',  ( 5.000000000000000000, -160.0625000000000568, 2.071067811865478614 ) ) ;
#54983=CARTESIAN_POINT ( 'NONE',  ( 4.458734125000001214, -9.145833331967736513, 2.574251347313718519 ) ) ;
#54984=CARTESIAN_POINT ( 'NONE',  ( -3.152548672688508926E-16, -51.81249999863440792, -5.148502694627439702 ) ) ;
#54985=EDGE_CURVE ( 'NONE', #54333, #46250, #50226, .T. ) ;
#54987=CARTESIAN_POINT ( 'NONE',  ( -4.458734125000000326, -146.0000000013655779, -1.846868145590735644 ) ) ;
#54991=ORIENTED_EDGE ( 'NONE', *, *, #28640, .T. ) ;
#54992=LINE ( 'NONE', #29574, #20065 ) ;
#54993=CARTESIAN_POINT ( 'NONE',  ( -2.229367062500000163, 25.27083333469892779, -3.861377020970580443 ) ) ;
#55001=CARTESIAN_POINT ( 'NONE',  ( 2.229367062499998831, -7.645833331967735624, -3.861377020970580887 ) ) ;
#55003=CARTESIAN_POINT ( 'NONE',  ( 4.458734124999999437, -148.4375000013656063, 0.000000000000000000 ) ) ;
#55005=EDGE_LOOP ( 'NONE', ( #2020, #49297, #6838, #35279 ) ) ;
#55006=DIRECTION ( 'NONE',  ( 0.000000000000000000, 0.000000000000000000, 1.000000000000000000 ) ) ;
#55009=CARTESIAN_POINT ( 'NONE',  ( 1.339745962155615144, -25.58034179853029144, 4.999999999999999112 ) ) ;
#55016=CARTESIAN_POINT ( 'NONE',  ( 1.339745962155615144, -74.70534180126148271, 4.999999999999999112 ) ) ;
#55019=CYLINDRICAL_SURFACE ( 'NONE', #48974, 5.000000000000000000 ) ;
#55020=CARTESIAN_POINT ( 'NONE',  ( -3.152548672688508926E-16, 10.43750000136559386, -5.148502694627439702 ) ) ;
#55023=CARTESIAN_POINT ( 'NONE',  ( 4.458734124999999437, -16.06249999863440436, -5.460374474430324690E-16 ) ) ;
#55025=CARTESIAN_POINT ( 'NONE',  ( 4.458734125000000326, -165.3750000013656347, -1.846868145590734978 ) ) ;
#55031=CARTESIAN_POINT ( 'NONE',  ( 1.975475456537005874E-15, -27.74999999999999645, 5.000000000000000000 ) ) ;
#55034=CARTESIAN_POINT ( 'NONE',  ( 1.846868145590736310, -148.8750000013655779, 4.458734124999997661 ) ) ;
#55036=CARTESIAN_POINT ( 'NONE',  ( -2.499999999999996447, -57.70833333060214443, 4.330127018922195425 ) ) ;
#55040=CYLINDRICAL_SURFACE ( 'NONE', #45263, 5.000000000000000000 ) ;
#55041=CARTESIAN_POINT ( 'NONE',  ( -5.000000000000000000, -0.08333333333333457771, -2.886751345948128211 ) ) ;
#55043=EDGE_CURVE ( 'NONE', #61158, #52679, #41372, .T. ) ;
#55044=CARTESIAN_POINT ( 'NONE',  ( -2.229367062500000163, -64.47916666530106511, -3.861377020970580443 ) ) ;
#55048=CARTESIAN_POINT ( 'NONE',  ( -2.499999999999996447, -8.708333330602144429, 4.330127018922195425 ) ) ;
#55049=CARTESIAN_POINT ( 'NONE',  ( 4.458734125000001214, -34.89583333196772941, 2.574251347313718519 ) ) ;
#55053=CARTESIAN_POINT ( 'NONE',  ( 4.458734124999999437, 14.93750000136559386, -5.460374474430324690E-16 ) ) ;
#55056=CARTESIAN_POINT ( 'NONE',  ( 1.060575238724906964E-15, -48.75000000000000000, 5.773502691896257311 ) ) ;
#55058=CARTESIAN_POINT ( 'NONE',  ( -4.999999999999998224, -3.916666666666665630, 2.886751345948131764 ) ) ;
#55059=CARTESIAN_POINT ( 'NONE',  ( 2.229367062499998831, -74.64583333196773651, -3.861377020970580887 ) ) ;
#55060=CARTESIAN_POINT ( 'NONE',  ( -4.458734124999999437, -140.1875000013656063, -5.460374474430324690E-16 ) ) ;
#55061=CARTESIAN_POINT ( 'NONE',  ( -2.229367062500000163, -79.47916666530106511, -3.861377020970580443 ) ) ;
#55064=CARTESIAN_POINT ( 'NONE',  ( -2.229367062500000163, -29.72916666530107221, -3.861377020970580443 ) ) ;
#55065=VERTEX_POINT ( 'NONE', #22089 ) ;
#55068=EDGE_CURVE ( 'NONE', #35072, #1769, #23921, .T. ) ;
#55075=CARTESIAN_POINT ( 'NONE',  ( -4.458734124999999437, -63.56249999863440792, 0.000000000000000000 ) ) ;
#55077=EDGE_LOOP ( 'NONE', ( #30548, #28243, #30297, #30165 ) ) ;
#55078=CARTESIAN_POINT ( 'NONE',  ( -5.000000000000000000, 5.125000002731184168, 0.000000000000000000 ) ) ;
#55079=DIRECTION ( 'NONE',  ( -0.000000000000000000, 1.000000000000000000, -0.000000000000000000 ) ) ;
#55080=CARTESIAN_POINT ( 'NONE',  ( -2.229367062500000163, 6.520833334698928674, -3.861377020970580443 ) ) ;
#55082=CARTESIAN_POINT ( 'NONE',  ( 1.975475456537005874E-15, -0.6249999972688137229, 5.000000000000000000 ) ) ;
#55083=CARTESIAN_POINT ( 'NONE',  ( -4.458734125000000326, -159.8750000013655779, 1.846868145590734089 ) ) ;
#55088=CARTESIAN_POINT ( 'NONE',  ( -6.972266317189433020E-16, -69.12499999726880162, -5.000000000000000000 ) ) ;
#55089=CARTESIAN_POINT ( 'NONE',  ( 1.975475456537005874E-15, -39.62499999726880162, 5.000000000000000000 ) ) ;
#55092=CARTESIAN_POINT ( 'NONE',  ( -4.999999999999998224, -28.91666666666666430, 2.886751345948131764 ) ) ;
#55094=CARTESIAN_POINT ( 'NONE',  ( 2.229367062500001939, 28.02083333469892779, 3.861377020970579999 ) ) ;
#55097=CARTESIAN_POINT ( 'NONE',  ( -2.229367062499996610, 2.604166668032259491, 3.861377020970582219 ) ) ;
#55098=VECTOR ( 'NONE', #17553, 1000.000000000000000 ) ;
#55101=CARTESIAN_POINT ( 'NONE',  ( 3.535533905932738197, -146.0000000027311842, -3.535533905932738197 ) ) ;
#55102=DIRECTION ( 'NONE',  ( 0.000000000000000000, 0.000000000000000000, 1.000000000000000000 ) ) ;
#55108=CARTESIAN_POINT ( 'NONE',  ( -9.184850993605147944E-16, -140.2500000000000000, 5.000000000000000000 ) ) ;
#55110=CARTESIAN_POINT ( 'NONE',  ( 2.730187237215162345E-16, -162.4375000013655779, -4.458734124999999437 ) ) ;
#55114=CARTESIAN_POINT ( 'NONE',  ( -3.152801135295367096, -141.0625000013655779, -3.152801135295367541 ) ) ;
#55115=ORIENTED_EDGE ( 'NONE', *, *, #56305, .F. ) ;
#55116=CARTESIAN_POINT ( 'NONE',  ( -4.458734124999999437, 20.35416666803225993, -2.574251347313719407 ) ) ;
#55117=VERTEX_POINT ( 'NONE', #29022 ) ;
#55118=CARTESIAN_POINT ( 'NONE',  ( -2.229367062500000163, -62.72916666530106511, -3.861377020970580443 ) ) ;
#55121=CARTESIAN_POINT ( 'NONE',  ( 1.975475456537005874E-15, -2.624999997268813168, 5.000000000000000000 ) ) ;
#55122=CARTESIAN_POINT ( 'NONE',  ( 1.060575238724906964E-15, 15.25000000000000000, 5.773502691896257311 ) ) ;
#55123=CARTESIAN_POINT ( 'NONE',  ( -4.458734124999999437, -52.39583333196773651, -2.574251347313719407 ) ) ;
#55124=CARTESIAN_POINT ( 'NONE',  ( -4.458734124999999437, -13.31249999863440259, 0.000000000000000000 ) ) ;
#55125=DIRECTION ( 'NONE',  ( 0.000000000000000000, 0.000000000000000000, 1.000000000000000000 ) ) ;
#55126=ADVANCED_FACE ( 'NONE', ( #8249 ), #24211, .T. ) ;
#55129=CARTESIAN_POINT ( 'NONE',  ( 0.000000000000000000, -170.0000000000000000, 0.000000000000000000 ) ) ;
#55130=CARTESIAN_POINT ( 'NONE',  ( -5.000000000000000000, -34.08333333333332860, -2.886751345948128211 ) ) ;
#55134=CARTESIAN_POINT ( 'NONE',  ( -2.229367062500000163, -60.47916666530106511, -3.861377020970580443 ) ) ;
#55135=CARTESIAN_POINT ( 'NONE',  ( 2.730187237215162345E-16, -150.4375000013656063, -4.458734124999999437 ) ) ;
#55136=CARTESIAN_POINT ( 'NONE',  ( 2.229367062499998831, -66.64583333196773651, -3.861377020970580887 ) ) ;
#55139=CARTESIAN_POINT ( 'NONE',  ( -4.999999999999999112, -53.79166666393548013, 2.886751345948131764 ) ) ;
#55142=CARTESIAN_POINT ( 'NONE',  ( -4.458734124999998549, 1.520833334698927342, 2.574251347313722516 ) ) ;
#55145=LINE ( 'NONE', #11071, #40901 ) ;
#55146=CARTESIAN_POINT ( 'NONE',  ( -4.458734125000000326, -155.0000000013656063, -1.846868145590735644 ) ) ;
#55147=EDGE_CURVE ( 'NONE', #30611, #39890, #638, .T. ) ;
#55148=ORIENTED_EDGE ( 'NONE', *, *, #55043, .T. ) ;
#55149=AXIS2_PLACEMENT_3D ( 'NONE', #40279, #54443, #49608 ) ;
#55152=CARTESIAN_POINT ( 'NONE',  ( -6.972266317189433020E-16, -80.12499999726881583, -5.000000000000000000 ) ) ;
#55153=CARTESIAN_POINT ( 'NONE',  ( 4.458734124999999437, -51.06249999863440792, -5.460374474430324690E-16 ) ) ;
#55154=AXIS2_PLACEMENT_3D ( 'NONE', #34950, #6962, #872 ) ;
#55157=EDGE_CURVE ( 'NONE', #17838, #39270, #62262, .T. ) ;
#55162=CARTESIAN_POINT ( 'NONE',  ( 4.458734125000001214, 24.10416666803226349, 2.574251347313718519 ) ) ;
#55165=CARTESIAN_POINT ( 'NONE',  ( -6.972266317189433020E-16, 16.87500000273118417, -5.000000000000000000 ) ) ;
#55167=CARTESIAN_POINT ( 'NONE',  ( -6.972266317189433020E-16, 0.7499999999999996669, -5.000000000000000000 ) ) ;
#55175=CARTESIAN_POINT ( 'NONE',  ( -2.229367062499996610, -89.39583333196773651, 3.861377020970582219 ) ) ;
#55176=LINE ( 'NONE', #20440, #6991 ) ;
#55178=ORIENTED_EDGE ( 'NONE', *, *, #42218, .T. ) ;
#55180=CARTESIAN_POINT ( 'NONE',  ( -5.000000000000000888, -156.5625000027312126, 2.071067811865474617 ) ) ;
#55190=CARTESIAN_POINT ( 'NONE',  ( 1.975475456537005874E-15, -53.74999999999999289, 5.000000000000000000 ) ) ;
#55191=CARTESIAN_POINT ( 'NONE',  ( -3.152548672688508926E-16, -20.56249999863440081, -5.148502694627439702 ) ) ;
#55193=CARTESIAN_POINT ( 'NONE',  ( -3.535533905932738641, -149.3750000000000000, 3.535533905932737309 ) ) ;
#55195=CARTESIAN_POINT ( 'NONE',  ( 1.846868145590735200, -152.2500000013656347, -4.458734125000000326 ) ) ;
#55197=CARTESIAN_POINT ( 'NONE',  ( -2.229367062500000163, -43.72916666530106511, -3.861377020970580443 ) ) ;
#55201=CARTESIAN_POINT ( 'NONE',  ( 4.458734124999999437, -88.81249999863439371, -5.460374474430324690E-16 ) ) ;
#55205=CARTESIAN_POINT ( 'NONE',  ( 2.229367062500001939, 4.020833334698926009, 3.861377020970579999 ) ) ;
#55208=CARTESIAN_POINT ( 'NONE',  ( 2.499999999999998668, -82.33333333333332860, -4.330127018922193649 ) ) ;
#55209=CARTESIAN_POINT ( 'NONE',  ( -4.458734124999999437, 14.43750000136559386, 0.000000000000000000 ) ) ;
#55211=CARTESIAN_POINT ( 'NONE',  ( 1.060575238724906964E-15, 9.375000002731184168, 5.773502691896257311 ) ) ;
#55216=CARTESIAN_POINT ( 'NONE',  ( 4.458734124999998549, -41.72916666530107932, -2.574251347313721627 ) ) ;
#55217=CARTESIAN_POINT ( 'NONE',  ( 1.975475456537005874E-15, -59.62499999726880873, 5.000000000000000000 ) ) ;
#55218=CARTESIAN_POINT ( 'NONE',  ( -4.999999999999999112, -41.79166666393548013, 2.886751345948131764 ) ) ;
#55219=EDGE_LOOP ( 'NONE', ( #6983, #2614, #10890, #6020 ) ) ;
#55220=CARTESIAN_POINT ( 'NONE',  ( -2.229367062500000163, -20.47916666530107221, -3.861377020970580443 ) ) ;
#55221=ORIENTED_EDGE ( 'NONE', *, *, #36967, .T. ) ;
#55222=CARTESIAN_POINT ( 'NONE',  ( -2.500000000000000444, -87.16666666666667140, -4.330127018922193649 ) ) ;
#55224=CARTESIAN_POINT ( 'NONE',  ( 5.000000000000000000, -88.37499999726880162, -6.123233995736766282E-16 ) ) ;
#55225=CARTESIAN_POINT ( 'NONE',  ( -6.972266317189433020E-16, -20.12499999726881228, -5.000000000000000000 ) ) ;
#55228=CARTESIAN_POINT ( 'NONE',  ( -2.229367062500000163, -30.72916666530107221, -3.861377020970580443 ) ) ;
#55229=CARTESIAN_POINT ( 'NONE',  ( -2.500000000000000444, -50.16666666666666430, -4.330127018922193649 ) ) ;
#55230=VERTEX_POINT ( 'NONE', #49292 ) ;
#55231=ADVANCED_FACE ( 'NONE', ( #59263 ), #5232, .T. ) ;
#55235=CARTESIAN_POINT ( 'NONE',  ( 1.975475456537005874E-15, -23.75000000000000000, 5.000000000000000000 ) ) ;
#55237=CARTESIAN_POINT ( 'NONE',  ( -5.000000000000000000, -166.6250000027312126, -6.123233995736766282E-16 ) ) ;
#55239=CARTESIAN_POINT ( 'NONE',  ( -3.152548672688508926E-16, -76.81249999863440792, -5.148502694627439702 ) ) ;
#55242=CARTESIAN_POINT ( 'NONE',  ( -4.458734124999999437, -141.2500000013656063, -1.846868145590735644 ) ) ;
#55243=AXIS2_PLACEMENT_3D ( 'NONE', #46769, #8174, #22335 ) ;
#55244=CARTESIAN_POINT ( 'NONE',  ( 1.339745962155609149, 24.29465819873852084, 5.000000000000003553 ) ) ;
#55246=CARTESIAN_POINT ( 'NONE',  ( 2.229367062499998831, -44.64583333196774362, -3.861377020970580887 ) ) ;
#55248=AXIS2_PLACEMENT_3D ( 'NONE', #9297, #4475, #48846 ) ;
#55251=CARTESIAN_POINT ( 'NONE',  ( 4.458734125000000326, -141.6250000013656631, -1.846868145590734978 ) ) ;
#55256=CARTESIAN_POINT ( 'NONE',  ( -4.458734124999998549, -71.47916666530107932, 2.574251347313722516 ) ) ;
#55257=CARTESIAN_POINT ( 'NONE',  ( -2.071067811865507036, -166.6875000000000284, -4.999999999999968914 ) ) ;
#55259=VECTOR ( 'NONE', #53393, 1000.000000000000000 ) ;
#55268=CARTESIAN_POINT ( 'NONE',  ( -3.152548672688508926E-16, 20.18750000136559208, -5.148502694627439702 ) ) ;
#55275=CARTESIAN_POINT ( 'NONE',  ( 9.457646018065525792E-16, -86.06249999863439371, 5.148502694627439702 ) ) ;
#55276=CARTESIAN_POINT ( 'NONE',  ( -2.229367062500000163, -3.479166665301069994, -3.861377020970580443 ) ) ;
#55278=ORIENTED_EDGE ( 'NONE', *, *, #45607, .T. ) ;
#55279=CARTESIAN_POINT ( 'NONE',  ( 2.229367062499998831, -27.89583333196774007, -3.861377020970580887 ) ) ;
#55280=( BOUNDED_CURVE ( )  B_SPLINE_CURVE ( 2, ( #7093, #46322, #32150, #22204, #47275, #52102, #36671, #12229, #41803 ),
 .UNSPECIFIED., .F., .F. ) 
 B_SPLINE_CURVE_WITH_KNOTS ( ( 3, 2, 2, 2, 3 ),
 ( 0.06875000000000000555, 0.06944444444444444753, 0.07083333333333333148, 0.07222222222222221544, 0.07291666666666667129 ),
 .UNSPECIFIED. ) 
 CURVE ( )  GEOMETRIC_REPRESENTATION_ITEM ( )  RATIONAL_B_SPLINE_CURVE ( ( 0.9330127018922194093, 0.9330127018922200755, 1.000000000000000000, 0.8660254037844387076, 1.000000000000000000, 0.8660254037844387076, 1.000000000000000000, 0.9330127018922187432, 0.9330127018922194093 ) ) 
 REPRESENTATION_ITEM ( '' )  );
#55284=CARTESIAN_POINT ( 'NONE',  ( -4.458734124999999437, 22.68750000136559564, 0.000000000000000000 ) ) ;
#55286=CARTESIAN_POINT ( 'NONE',  ( 1.062108568985190270E-13, -26.12499999726881583, -4.999999999999999112 ) ) ;
#55287=CARTESIAN_POINT ( 'NONE',  ( 4.458734124999998549, -76.97916666530106511, -2.574251347313721627 ) ) ;
#55289=DIRECTION ( 'NONE',  ( -0.000000000000000000, 1.000000000000000000, -0.000000000000000000 ) ) ;
#55290=CARTESIAN_POINT ( 'NONE',  ( 5.000000000000000000, 23.70833333606451632, -2.886751345948129988 ) ) ;
#55291=ORIENTED_EDGE ( 'NONE', *, *, #2434, .F. ) ;
#55293=VECTOR ( 'NONE', #42880, 1000.000000000000000 ) ;
#55294=CARTESIAN_POINT ( 'NONE',  ( -2.499999999999996447, -56.70833333060214443, 4.330127018922195425 ) ) ;
#55295=CARTESIAN_POINT ( 'NONE',  ( 1.339745962155612702, -0.2946581987385212820, -5.000000000000000000 ) ) ;
#55296=CARTESIAN_POINT ( 'NONE',  ( -5.000000000000000000, -25.08333333333333215, -2.886751345948128211 ) ) ;
#55297=CARTESIAN_POINT ( 'NONE',  ( 9.457646018065525792E-16, -28.06249999863440081, 5.148502694627439702 ) ) ;
#55300=CARTESIAN_POINT ( 'NONE',  ( -4.458734124999997661, -90.22916666530106511, 2.574251347313722516 ) ) ;
#55301=CARTESIAN_POINT ( 'NONE',  ( 5.000000000000000888, -21.45833333060215153, 2.886751345948126879 ) ) ;
#55302=CARTESIAN_POINT ( 'NONE',  ( 4.458734125000001214, -55.89583333196773651, 2.574251347313718519 ) ) ;
#55304=CARTESIAN_POINT ( 'NONE',  ( -6.972266317189433020E-16, -65.24999999999998579, -5.000000000000000000 ) ) ;
#55305=CARTESIAN_POINT ( 'NONE',  ( 1.975475456537005874E-15, -74.62499999726880162, 5.000000000000000000 ) ) ;
#55306=CARTESIAN_POINT ( 'NONE',  ( 9.457646018065525792E-16, -2.312499998634407028, 5.148502694627439702 ) ) ;
#55307=ORIENTED_EDGE ( 'NONE', *, *, #53172, .F. ) ;
#55309=CARTESIAN_POINT ( 'NONE',  ( 2.499999999999998668, -67.33333333333332860, -4.330127018922193649 ) ) ;
#55310=CARTESIAN_POINT ( 'NONE',  ( -1.846868145590734756, -150.3750000013655779, -4.458734125000000326 ) ) ;
#55313=( BOUNDED_CURVE ( )  B_SPLINE_CURVE ( 2, ( #55968, #17354, #45351, #30874, #60479, #16404, #21552, #36022, #11568 ),
 .UNSPECIFIED., .F., .F. ) 
 B_SPLINE_CURVE_WITH_KNOTS ( ( 3, 2, 2, 2, 3 ),
 ( 0.1854166666666666741, 0.1861111111111111160, 0.1875000000000000000, 0.1888888888888888840, 0.1895833333333333259 ),
 .UNSPECIFIED. ) 
 CURVE ( )  GEOMETRIC_REPRESENTATION_ITEM ( )  RATIONAL_B_SPLINE_CURVE ( ( 0.9330127018922194093, 0.9330127018922194093, 1.000000000000000000, 0.8660254037844387076, 1.000000000000000000, 0.8660254037844387076, 1.000000000000000000, 0.9330127018922194093, 0.9330127018922194093 ) ) 
 REPRESENTATION_ITEM ( '' )  );
#55314=CARTESIAN_POINT ( 'NONE',  ( -3.535533905932738641, -159.3750000000000284, 3.535533905932737309 ) ) ;
#55315=DIRECTION ( 'NONE',  ( 0.000000000000000000, 0.000000000000000000, 1.000000000000000000 ) ) ;
#55317=CARTESIAN_POINT ( 'NONE',  ( -4.458734124999999437, -13.64583333196774007, -2.574251347313719407 ) ) ;
#55318=CARTESIAN_POINT ( 'NONE',  ( 4.458734125000001214, -50.14583333196773651, 2.574251347313718519 ) ) ;
#55320=CARTESIAN_POINT ( 'NONE',  ( 2.730187237215162345E-16, -143.1875000013656063, -4.458734124999999437 ) ) ;
#55322=CARTESIAN_POINT ( 'NONE',  ( 1.975475456537005874E-15, -87.62499999726880162, 5.000000000000000000 ) ) ;
#55323=ORIENTED_EDGE ( 'NONE', *, *, #31885, .T. ) ;
#55325=CARTESIAN_POINT ( 'NONE',  ( 4.458734125000001214, 27.85416666803225993, 2.574251347313718519 ) ) ;
#55329=CARTESIAN_POINT ( 'NONE',  ( -6.972266317189433020E-16, -19.25000000000000000, -5.000000000000000000 ) ) ;
#55331=CARTESIAN_POINT ( 'NONE',  ( -4.999999999999998224, 9.083333333333333925, 2.886751345948131764 ) ) ;
#55332=CARTESIAN_POINT ( 'NONE',  ( 2.229367062499998831, -5.645833331967740953, -3.861377020970580887 ) ) ;
#55334=CARTESIAN_POINT ( 'NONE',  ( -4.458734125000000326, -149.8750000013655779, 1.846868145590734089 ) ) ;
#55335=AXIS2_PLACEMENT_3D ( 'NONE', #28174, #1072, #6517 ) ;
#55337=VERTEX_POINT ( 'NONE', #20019 ) ;
#55338=CARTESIAN_POINT ( 'NONE',  ( -1.339745962155610925, -26.66965819600732956, 5.000000000000000000 ) ) ;
#55341=ADVANCED_FACE ( 'NONE', ( #35145 ), #45101, .T. ) ;
#55351=CARTESIAN_POINT ( 'NONE',  ( -4.458734124999999437, 11.60416666803225993, -2.574251347313719407 ) ) ;
#55353=CARTESIAN_POINT ( 'NONE',  ( -3.152548672688508926E-16, -13.81249999863440259, -5.148502694627439702 ) ) ;
#55355=CARTESIAN_POINT ( 'NONE',  ( 4.458734125000000326, -162.3750000013655779, -1.846868145590734978 ) ) ;
#55356=CARTESIAN_POINT ( 'NONE',  ( -4.999999999999998224, -40.79166666393548724, 2.886751345948131764 ) ) ;
#55363=CARTESIAN_POINT ( 'NONE',  ( 4.458734124999999437, -35.81249999863440792, -5.460374474430324690E-16 ) ) ;
#55369=DIRECTION ( 'NONE',  ( -0.000000000000000000, 1.000000000000000000, -0.000000000000000000 ) ) ;
#55370=CARTESIAN_POINT ( 'NONE',  ( -3.535250795749689387E-16, -4.249999999999996447, -5.773502691896257311 ) ) ;
#55371=CARTESIAN_POINT ( 'NONE',  ( 9.457646018065525792E-16, -72.06249999863439371, 5.148502694627439702 ) ) ;
#55373=CARTESIAN_POINT ( 'NONE',  ( 5.000000000000000888, -5.458333330602148870, 2.886751345948126879 ) ) ;
#55374=CARTESIAN_POINT ( 'NONE',  ( 2.229367062499998831, -39.64583333196773651, -3.861377020970580887 ) ) ;
#55377=CARTESIAN_POINT ( 'NONE',  ( -2.229367062500000163, 12.27083333469892601, -3.861377020970580443 ) ) ;
#55378=EDGE_LOOP ( 'NONE', ( #62302, #88, #24605, #22795 ) ) ;
#55379=CARTESIAN_POINT ( 'NONE',  ( 2.500000000000002220, -52.66666666666666430, 4.330127018922192761 ) ) ;
#55381=CARTESIAN_POINT ( 'NONE',  ( -2.499999999999996447, -3.833333333333334370, 4.330127018922195425 ) ) ;
#55382=CARTESIAN_POINT ( 'NONE',  ( -4.458734124999999437, -77.31249999863440792, 0.000000000000000000 ) ) ;
#55383=CARTESIAN_POINT ( 'NONE',  ( 4.458734124999999437, -140.7500000013655779, 1.846868145590737864 ) ) ;
#55384=CARTESIAN_POINT ( 'NONE',  ( 4.458734125000001214, -81.89583333196773651, 2.574251347313718519 ) ) ;
#55387=CARTESIAN_POINT ( 'NONE',  ( 2.229367062499998831, -37.89583333196773651, -3.861377020970580887 ) ) ;
#55393=VERTEX_POINT ( 'NONE', #25480 ) ;
#55396=CARTESIAN_POINT ( 'NONE',  ( -3.152548672688508926E-16, -63.81249999863440792, -5.148502694627439702 ) ) ;
#55399=CARTESIAN_POINT ( 'NONE',  ( 2.500000000000002220, 3.458333336064517205, 4.330127018922192761 ) ) ;
#55400=( BOUNDED_CURVE ( )  B_SPLINE_CURVE ( 2, ( #59124, #20844, #25668, #35635, #6375, #25341, #45596, #55583, #40447 ),
 .UNSPECIFIED., .F., .F. ) 
 B_SPLINE_CURVE_WITH_KNOTS ( ( 3, 2, 2, 2, 3 ),
 ( 0.04375000000000000416, 0.04444444444444444614, 0.04583333333333333010, 0.04722222222222222099, 0.04791666666666666990 ),
 .UNSPECIFIED. ) 
 CURVE ( )  GEOMETRIC_REPRESENTATION_ITEM ( )  RATIONAL_B_SPLINE_CURVE ( ( 0.9330127018922192983, 0.9330127018922196314, 1.000000000000000000, 0.8660254037844387076, 1.000000000000000000, 0.8660254037844387076, 1.000000000000000000, 0.9330127018922189652, 0.9330127018922192983 ) ) 
 REPRESENTATION_ITEM ( '' )  );
#55402=VERTEX_POINT ( 'NONE', #25808 ) ;
#55404=CARTESIAN_POINT ( 'NONE',  ( 4.458734125000001214, 9.104166668032261711, 2.574251347313718519 ) ) ;
#55405=CARTESIAN_POINT ( 'NONE',  ( -6.972266317189433020E-16, -78.24999999999998579, -5.000000000000000000 ) ) ;
#55406=CARTESIAN_POINT ( 'NONE',  ( 1.846868145590736310, -162.6250000013656063, 4.458734124999997661 ) ) ;
#55407=CARTESIAN_POINT ( 'NONE',  ( 1.975475456537005874E-15, 19.37500000273118772, 5.000000000000000000 ) ) ;
#55408=ORIENTED_EDGE ( 'NONE', *, *, #22394, .T. ) ;
#55413=DIRECTION ( 'NONE',  ( 0.000000000000000000, 0.000000000000000000, 1.000000000000000000 ) ) ;
#55417=CARTESIAN_POINT ( 'NONE',  ( -1.339745962155610925, -20.79465819873852084, 5.000000000000000000 ) ) ;
#55420=CARTESIAN_POINT ( 'NONE',  ( -3.152548672688508926E-16, 28.43750000136559564, -5.148502694627439702 ) ) ;
#55423=CARTESIAN_POINT ( 'NONE',  ( -2.229367062500000163, 3.270833334698929118, -3.861377020970580443 ) ) ;
#55424=STYLED_ITEM ( 'NONE', ( #2553 ), #3382 ) ;
#55425=CARTESIAN_POINT ( 'NONE',  ( 3.061616997868383141E-16, -149.8750000027312126, -5.000000000000000000 ) ) ;
#55427=CARTESIAN_POINT ( 'NONE',  ( -3.535533905932738641, -143.5000000027311842, 3.535533905932737309 ) ) ;
#55428=CARTESIAN_POINT ( 'NONE',  ( 2.071067811865370256, -158.8125000000000284, -5.000000000000105693 ) ) ;
#55433=CARTESIAN_POINT ( 'NONE',  ( 0.000000000000000000, -170.0000000000000000, 0.000000000000000000 ) ) ;
#55437=CARTESIAN_POINT ( 'NONE',  ( 1.846868145590735200, -161.5000000013656063, -4.458734124999999437 ) ) ;
#55440=CARTESIAN_POINT ( 'NONE',  ( -1.339745962155613812, -57.20534180126148271, -5.000000000000000000 ) ) ;
#55442=CARTESIAN_POINT ( 'NONE',  ( 2.229367062499998831, 24.10416666803225993, -3.861377020970580887 ) ) ;
#55443=EDGE_LOOP ( 'NONE', ( #29087, #50692, #6489, #19508 ) ) ;
#55445=CARTESIAN_POINT ( 'NONE',  ( -5.000000000000000000, -2.958333330602146649, -2.886751345948128211 ) ) ;
#55446=CARTESIAN_POINT ( 'NONE',  ( -3.535250795749689387E-16, 11.74999999999999822, -5.773502691896257311 ) ) ;
#55447=CARTESIAN_POINT ( 'NONE',  ( -4.458734124999999437, -48.31249999863440792, 0.000000000000000000 ) ) ;
#55448=CARTESIAN_POINT ( 'NONE',  ( -3.152548672688508926E-16, -11.56249999863440792, -5.148502694627439702 ) ) ;
#55451=DIRECTION ( 'NONE',  ( -0.000000000000000000, 1.000000000000000000, -0.000000000000000000 ) ) ;
#55452=CARTESIAN_POINT ( 'NONE',  ( 3.061616997868383141E-16, -153.8750000027311842, -5.000000000000000000 ) ) ;
#55454=CARTESIAN_POINT ( 'NONE',  ( 5.000000000000000000, -33.50000000000000000, -6.123233995736766282E-16 ) ) ;
#55455=CYLINDRICAL_SURFACE ( 'NONE', #7913, 5.000000000000000000 ) ;
#55456=CARTESIAN_POINT ( 'NONE',  ( -1.339745962155613812, -59.20534180126148271, -5.000000000000000000 ) ) ;
#55460=CARTESIAN_POINT ( 'NONE',  ( -3.152548672688508926E-16, -61.56249999863440792, -5.148502694627439702 ) ) ;
#55461=CARTESIAN_POINT ( 'NONE',  ( -4.458734125000001214, -151.1250000013655779, 1.846868145590734089 ) ) ;
#55462=ADVANCED_FACE ( 'NONE', ( #45421 ), #10370, .T. ) ;
#55463=CARTESIAN_POINT ( 'NONE',  ( 4.458734124999999437, -64.81249999863440792, -5.460374474430324690E-16 ) ) ;
#55465=CARTESIAN_POINT ( 'NONE',  ( 5.000000000000000888, -57.45833333060214443, 2.886751345948126879 ) ) ;
#55467=FACE_OUTER_BOUND ( 'NONE', #12107, .T. ) ;
#55469=CYLINDRICAL_SURFACE ( 'NONE', #52305, 5.000000000000000000 ) ;
#55471=CARTESIAN_POINT ( 'NONE',  ( 2.730187237215162345E-16, -152.1875000013656063, -4.458734124999999437 ) ) ;
#55472=ORIENTED_EDGE ( 'NONE', *, *, #45902, .F. ) ;
#55474=DIRECTION ( 'NONE',  ( -0.000000000000000000, 1.000000000000000000, -0.000000000000000000 ) ) ;
#55476=CARTESIAN_POINT ( 'NONE',  ( 5.000000000000000000, -153.0625000000000284, 2.071067811865478614 ) ) ;
#55477=AXIS2_PLACEMENT_3D ( 'NONE', #1823, #56483, #26565 ) ;
#55478=CARTESIAN_POINT ( 'NONE',  ( 9.457646018065525792E-16, -47.31249999863440792, 5.148502694627439702 ) ) ;
#55480=CARTESIAN_POINT ( 'NONE',  ( 1.975475456537005874E-15, 17.37500000273118417, 5.000000000000000000 ) ) ;
#55481=AXIS2_PLACEMENT_3D ( 'NONE', #56050, #36108, #42821 ) ;
#55483=CARTESIAN_POINT ( 'NONE',  ( -4.458734124999999437, 23.68750000136559564, 0.000000000000000000 ) ) ;
#55486=CARTESIAN_POINT ( 'NONE',  ( -6.972266317189433020E-16, -36.12499999726880162, -5.000000000000000000 ) ) ;
#55493=CARTESIAN_POINT ( 'NONE',  ( -6.972266317189433020E-16, -51.25000000000000000, -5.000000000000000000 ) ) ;
#55502=ORIENTED_EDGE ( 'NONE', *, *, #53014, .F. ) ;
#55504=CARTESIAN_POINT ( 'NONE',  ( -3.535533905932738641, -169.3750000000000284, 3.535533905932737309 ) ) ;
#55506=CARTESIAN_POINT ( 'NONE',  ( -3.535533905932737309, -155.7500000027312126, -3.535533905932738197 ) ) ;
#55507=ORIENTED_EDGE ( 'NONE', *, *, #20868, .F. ) ;
#55518=CARTESIAN_POINT ( 'NONE',  ( -4.458734124999997661, -17.22916666530106866, 2.574251347313722516 ) ) ;
#55520=CARTESIAN_POINT ( 'NONE',  ( 5.000000000000000000, -152.0000000000000284, 0.000000000000000000 ) ) ;
#55523=CARTESIAN_POINT ( 'NONE',  ( -8.190561711645485556E-16, -150.6875000013656063, 4.458734124999999437 ) ) ;
#55524=ORIENTED_EDGE ( 'NONE', *, *, #14231, .F. ) ;
#55526=CARTESIAN_POINT ( 'NONE',  ( 4.458734125000000326, -45.14583333196774362, 2.574251347313718519 ) ) ;
#55528=CARTESIAN_POINT ( 'NONE',  ( -6.972266317189433020E-16, -63.25000000000000000, -5.000000000000000000 ) ) ;
#55529=EDGE_CURVE ( 'NONE', #37570, #54241, #53596, .T. ) ;
#55530=CARTESIAN_POINT ( 'NONE',  ( 1.060575238724906964E-15, 28.24999999999999645, 5.773502691896257311 ) ) ;
#55531=VECTOR ( 'NONE', #31610, 1000.000000000000000 ) ;
#55532=CARTESIAN_POINT ( 'NONE',  ( 9.457646018065525792E-16, 2.937500001365594304, 5.148502694627439702 ) ) ;
#55534=FACE_OUTER_BOUND ( 'NONE', #30833, .T. ) ;
#55536=CARTESIAN_POINT ( 'NONE',  ( -2.229367062500000163, 13.27083333469892779, -3.861377020970580443 ) ) ;
#55538=CARTESIAN_POINT ( 'NONE',  ( -2.500000000000000444, 8.958333336064518093, -4.330127018922193649 ) ) ;
#55542=CARTESIAN_POINT ( 'NONE',  ( -3.152548672688508926E-16, -45.56249999863439371, -5.148502694627439702 ) ) ;
#55543=CARTESIAN_POINT ( 'NONE',  ( -4.458734125000001214, -163.1250000013656063, 1.846868145590734089 ) ) ;
#55544=CARTESIAN_POINT ( 'NONE',  ( -3.535250795749689387E-16, -42.12499999726880873, -5.773502691896257311 ) ) ;
#55546=CARTESIAN_POINT ( 'NONE',  ( 4.458734124999998549, -15.72916666530107399, -2.574251347313721627 ) ) ;
#55548=CARTESIAN_POINT ( 'NONE',  ( 5.000000000000000000, -87.50000000000000000, -6.123233995736766282E-16 ) ) ;
#55549=CARTESIAN_POINT ( 'NONE',  ( -3.152801135295367096, -163.0625000013656063, -3.152801135295367541 ) ) ;
#55550=CARTESIAN_POINT ( 'NONE',  ( -3.535250795749689387E-16, -87.12499999726880162, -5.773502691896257311 ) ) ;
#55551=CARTESIAN_POINT ( 'NONE',  ( 1.975475456537005874E-15, -60.62499999726880162, 5.000000000000000000 ) ) ;
#55552=ORIENTED_EDGE ( 'NONE', *, *, #36926, .F. ) ;
#55554=CARTESIAN_POINT ( 'NONE',  ( -2.229367062500000163, -31.72916666530107577, -3.861377020970580443 ) ) ;
#55562=VECTOR ( 'NONE', #16176, 1000.000000000000000 ) ;
#55563=CARTESIAN_POINT ( 'NONE',  ( 2.229367062500001939, -82.22916666530106511, 3.861377020970579999 ) ) ;
#55566=CARTESIAN_POINT ( 'NONE',  ( -3.152801135295367096, -143.3125000013655779, -3.152801135295367541 ) ) ;
#55569=CARTESIAN_POINT ( 'NONE',  ( -3.152548672688508926E-16, -45.56249999863439371, -5.148502694627439702 ) ) ;
#55570=VECTOR ( 'NONE', #47677, 1000.000000000000000 ) ;
#55571=CARTESIAN_POINT ( 'NONE',  ( 1.255007937094098239E-14, 22.87500000273118772, -4.999999999999999112 ) ) ;
#55574=DIRECTION ( 'NONE',  ( 0.000000000000000000, 1.000000000000000000, 0.000000000000000000 ) ) ;
#55578=CARTESIAN_POINT ( 'NONE',  ( 2.229367062499998831, -76.89583333196773651, -3.861377020970580887 ) ) ;
#55582=ORIENTED_EDGE ( 'NONE', *, *, #57567, .T. ) ;
#55583=CARTESIAN_POINT ( 'NONE',  ( 1.339745962155609149, 23.41965820146970856, 5.000000000000003553 ) ) ;
#55585=CARTESIAN_POINT ( 'NONE',  ( 3.061616997868383141E-16, -168.8750000027312126, -5.000000000000000000 ) ) ;
#55587=CARTESIAN_POINT ( 'NONE',  ( -2.229367062499996610, 17.60416666803225993, 3.861377020970582219 ) ) ;
#55594=CARTESIAN_POINT ( 'NONE',  ( -2.499999999999996447, -15.70833333060214443, 4.330127018922195425 ) ) ;
#55595=CARTESIAN_POINT ( 'NONE',  ( -4.458734124999999437, -83.39583333196772230, -2.574251347313719407 ) ) ;
#55596=CARTESIAN_POINT ( 'NONE',  ( 9.457646018065525792E-16, -4.062499998634408804, 5.148502694627439702 ) ) ;
#55598=EDGE_CURVE ( 'NONE', #8450, #38824, #4745, .T. ) ;
#55600=CARTESIAN_POINT ( 'NONE',  ( 2.229367062499998831, -31.89583333196773651, -3.861377020970580887 ) ) ;
#55602=ADVANCED_FACE ( 'NONE', ( #61022 ), #51994, .T. ) ;
#55605=CARTESIAN_POINT ( 'NONE',  ( 4.458734124999998549, 20.27083333469892779, -2.574251347313721627 ) ) ;
#55608=CARTESIAN_POINT ( 'NONE',  ( 5.000000000000000000, -28.49999999999999645, -6.123233995736766282E-16 ) ) ;
#55609=CARTESIAN_POINT ( 'NONE',  ( -2.229367062500000163, -75.72916666530106511, -3.861377020970580443 ) ) ;
#55612=CARTESIAN_POINT ( 'NONE',  ( -2.499999999999996447, 22.29166666939785202, 4.330127018922195425 ) ) ;
#55613=ORIENTED_EDGE ( 'NONE', *, *, #46945, .F. ) ;
#55614=CARTESIAN_POINT ( 'NONE',  ( 0.000000000000000000, -170.0000000000000000, 0.000000000000000000 ) ) ;
#55616=CARTESIAN_POINT ( 'NONE',  ( 5.000000000000000000, -0.5000000000000004441, -6.123233995736766282E-16 ) ) ;
#55617=CARTESIAN_POINT ( 'NONE',  ( -2.500000000000000444, -24.16666666666666430, -4.330127018922193649 ) ) ;
#55618=CARTESIAN_POINT ( 'NONE',  ( -2.229367062500000163, -27.47916666530107221, -3.861377020970580443 ) ) ;
#55619=AXIS2_PLACEMENT_3D ( 'NONE', #1517, #35599, #34963 ) ;
#55620=CARTESIAN_POINT ( 'NONE',  ( 4.458734125000000326, -86.89583333196773651, 2.574251347313718519 ) ) ;
#55621=CARTESIAN_POINT ( 'NONE',  ( -5.000000000000000000, -22.95833333060214798, -2.886751345948128211 ) ) ;
#55622=CARTESIAN_POINT ( 'NONE',  ( 4.458734124999999437, -55.81249999863440081, -5.460374474430324690E-16 ) ) ;
#55624=CARTESIAN_POINT ( 'NONE',  ( -6.972266317189433020E-16, -49.24999999999999289, -5.000000000000000000 ) ) ;
#55626=CARTESIAN_POINT ( 'NONE',  ( 2.229367062500001939, -5.229166665301071326, 3.861377020970579999 ) ) ;
#55628=CARTESIAN_POINT ( 'NONE',  ( -4.999999999999999112, -72.91666666666665719, 2.886751345948131764 ) ) ;
#55629=CARTESIAN_POINT ( 'NONE',  ( -1.846868145590737420, -154.0000000013655779, 4.458734124999999437 ) ) ;
#55632=CARTESIAN_POINT ( 'NONE',  ( -2.071067811865475061, -159.6875000000000000, -5.000000000000000888 ) ) ;
#55633=CARTESIAN_POINT ( 'NONE',  ( 2.499999999999998668, -72.20833333060214443, -4.330127018922193649 ) ) ;
#55634=CARTESIAN_POINT ( 'NONE',  ( -5.000000000000000000, -53.87499999726880162, 0.000000000000000000 ) ) ;
#55636=CARTESIAN_POINT ( 'NONE',  ( -4.458734124999998549, -15.47916666530107399, 2.574251347313722516 ) ) ;
#55637=CARTESIAN_POINT ( 'NONE',  ( -4.458734124999998549, -49.47916666530106511, 2.574251347313722516 ) ) ;
#55639=CARTESIAN_POINT ( 'NONE',  ( -4.458734125000001214, -144.8750000013655779, 1.846868145590734089 ) ) ;
#55642=( BOUNDED_CURVE ( )  B_SPLINE_CURVE ( 2, ( #61649, #17583, #26916, #46533, #2474, #36879, #37200, #56826, #21456 ),
 .UNSPECIFIED., .F., .F. ) 
 B_SPLINE_CURVE_WITH_KNOTS ( ( 3, 2, 2, 2, 3 ),
 ( 0.03541666666666666574, 0.03611111111111110772, 0.03749999999999999861, 0.03888888888888888951, 0.03958333333333333842 ),
 .UNSPECIFIED. ) 
 CURVE ( )  GEOMETRIC_REPRESENTATION_ITEM ( )  RATIONAL_B_SPLINE_CURVE ( ( 0.9330127018922194093, 0.9330127018922194093, 1.000000000000000000, 0.8660254037844387076, 1.000000000000000000, 0.8660254037844387076, 1.000000000000000000, 0.9330127018922189652, 0.9330127018922192983 ) ) 
 REPRESENTATION_ITEM ( '' )  );
#55645=CARTESIAN_POINT ( 'NONE',  ( -3.152548672688508926E-16, 26.18750000136559564, -5.148502694627439702 ) ) ;
#55653=CARTESIAN_POINT ( 'NONE',  ( -3.152548672688508926E-16, -8.562499998634404363, -5.148502694627439702 ) ) ;
#55655=CARTESIAN_POINT ( 'NONE',  ( -4.458734124999999437, -144.0000000013655779, -1.846868145590735644 ) ) ;
#55657=ORIENTED_EDGE ( 'NONE', *, *, #23348, .T. ) ;
#55658=CARTESIAN_POINT ( 'NONE',  ( -5.000000000000000000, -62.95833333060215153, -2.886751345948128211 ) ) ;
#55664=CARTESIAN_POINT ( 'NONE',  ( 3.061616997868383141E-16, -146.8750000027312126, -5.000000000000000000 ) ) ;
#55667=CARTESIAN_POINT ( 'NONE',  ( 2.071067811865644703, -149.9375000027312126, -4.999999999999831246 ) ) ;
#55670=CARTESIAN_POINT ( 'NONE',  ( -2.229367062499996610, 11.85416666803225993, 3.861377020970582219 ) ) ;
#55672=CARTESIAN_POINT ( 'NONE',  ( 2.229367062499998831, -16.89583333196773651, -3.861377020970580887 ) ) ;
#55674=CARTESIAN_POINT ( 'NONE',  ( 4.458734124999999437, -162.5000000013655779, 1.846868145590737864 ) ) ;
#55679=CARTESIAN_POINT ( 'NONE',  ( -4.999999999999998224, -35.91666666666666430, 2.886751345948131764 ) ) ;
#55680=CARTESIAN_POINT ( 'NONE',  ( 9.457646018065525792E-16, -38.06249999863440792, 5.148502694627439702 ) ) ;
#55681=CARTESIAN_POINT ( 'NONE',  ( 5.000000000000000888, -51.45833333060214443, 2.886751345948126879 ) ) ;
#55690=CARTESIAN_POINT ( 'NONE',  ( -3.535250795749689387E-16, -10.25000000000000355, -5.773502691896257311 ) ) ;
#55691=CARTESIAN_POINT ( 'NONE',  ( 4.458734124999998549, -73.72916666530106511, -2.574251347313721627 ) ) ;
#55692=CARTESIAN_POINT ( 'NONE',  ( -6.972266317189433020E-16, -17.25000000000000000, -5.000000000000000000 ) ) ;
#55693=CARTESIAN_POINT ( 'NONE',  ( 5.000000000000000000, -8.291666663935481907, -2.886751345948129988 ) ) ;
#55694=CARTESIAN_POINT ( 'NONE',  ( 9.457646018065525792E-16, -38.06249999863441502, 5.148502694627439702 ) ) ;
#55696=CARTESIAN_POINT ( 'NONE',  ( 0.000000000000000000, -170.0000000000000000, 0.000000000000000000 ) ) ;
#55697=CARTESIAN_POINT ( 'NONE',  ( -4.458734124999999437, 12.43750000136559564, 0.000000000000000000 ) ) ;
#55698=ORIENTED_EDGE ( 'NONE', *, *, #16894, .T. ) ;
#55699=CARTESIAN_POINT ( 'NONE',  ( 0.000000000000000000, -170.0000000000000000, 5.000000000000000000 ) ) ;
#55700=CARTESIAN_POINT ( 'NONE',  ( -2.499999999999996447, -56.83333333333333570, 4.330127018922195425 ) ) ;
#55702=CARTESIAN_POINT ( 'NONE',  ( -6.972266317189433020E-16, -32.12499999726880873, -5.000000000000000000 ) ) ;
#55703=CARTESIAN_POINT ( 'NONE',  ( -3.152548672688508926E-16, -75.56249999863439371, -5.148502694627439702 ) ) ;
#55704=CARTESIAN_POINT ( 'NONE',  ( -3.535533905932738641, -169.3750000000000284, 3.535533905932737309 ) ) ;
#55705=CARTESIAN_POINT ( 'NONE',  ( 4.458734125000001214, -85.89583333196773651, 2.574251347313718519 ) ) ;
#55708=CARTESIAN_POINT ( 'NONE',  ( 4.458734124999998549, -35.97916666530107221, -2.574251347313721627 ) ) ;
#55709=CARTESIAN_POINT ( 'NONE',  ( 1.339745962155615144, -72.70534180126148271, 4.999999999999999112 ) ) ;
#55715=CARTESIAN_POINT ( 'NONE',  ( -4.999999999999998224, -18.79166666393547658, 2.886751345948131764 ) ) ;
#55716=CARTESIAN_POINT ( 'NONE',  ( 9.457646018065525792E-16, -65.31249999863440792, 5.148502694627439702 ) ) ;
#55720=CARTESIAN_POINT ( 'NONE',  ( -4.999999999999998224, 5.208333336064518981, 2.886751345948131764 ) ) ;
#55721=ORIENTED_EDGE ( 'NONE', *, *, #31450, .F. ) ;
#55723=CARTESIAN_POINT ( 'NONE',  ( 4.458734124999998549, 9.270833334698927786, -2.574251347313721627 ) ) ;
#55724=CARTESIAN_POINT ( 'NONE',  ( -8.190561711645485556E-16, -162.6875000013655779, 4.458734124999999437 ) ) ;
#55725=EDGE_LOOP ( 'NONE', ( #28702, #11219, #27736, #11612 ) ) ;
#55729=FACE_OUTER_BOUND ( 'NONE', #25150, .T. ) ;
#55734=CARTESIAN_POINT ( 'NONE',  ( -2.229367062499996610, 25.85416666803225993, 3.861377020970582219 ) ) ;
#55737=CARTESIAN_POINT ( 'NONE',  ( -2.229367062500000163, 4.270833334698926897, -3.861377020970580443 ) ) ;
#55738=CARTESIAN_POINT ( 'NONE',  ( 5.000000000000000000, -160.1875000027311842, 2.071067811865478614 ) ) ;
#55740=CARTESIAN_POINT ( 'NONE',  ( 3.535533905932736864, -147.2500000027311842, 3.535533905932738641 ) ) ;
#55746=CARTESIAN_POINT ( 'NONE',  ( -6.972266317189433020E-16, -88.25000000000000000, -5.000000000000000000 ) ) ;
#55748=CARTESIAN_POINT ( 'NONE',  ( -1.846868145590734756, -161.3750000013656063, -4.458734124999999437 ) ) ;
#55753=CARTESIAN_POINT ( 'NONE',  ( -2.229367062500000163, 24.27083333469892779, -3.861377020970580443 ) ) ;
#55758=CARTESIAN_POINT ( 'NONE',  ( 0.000000000000000000, -170.0000000000000000, 0.000000000000000000 ) ) ;
#55759=CARTESIAN_POINT ( 'NONE',  ( -4.999999999999999112, 10.08333333333333393, 2.886751345948131764 ) ) ;
#55760=( BOUNDED_CURVE ( )  B_SPLINE_CURVE ( 2, ( #45879, #41047, #60694, #11147, #31084, #51031, #25629, #45561, #6338 ),
 .UNSPECIFIED., .F., .F. ) 
 B_SPLINE_CURVE_WITH_KNOTS ( ( 3, 2, 2, 2, 3 ),
 ( 0.5312500000000000000, 0.5319444444444444420, 0.5333333333333333259, 0.5347222222222222099, 0.5354166666666666519 ),
 .UNSPECIFIED. ) 
 CURVE ( )  GEOMETRIC_REPRESENTATION_ITEM ( )  RATIONAL_B_SPLINE_CURVE ( ( 0.9330127018922194093, 0.9330127018922194093, 1.000000000000000000, 0.8660254037844387076, 1.000000000000000000, 0.8660254037844387076, 1.000000000000000000, 0.9330127018922194093, 0.9330127018922194093 ) ) 
 REPRESENTATION_ITEM ( '' )  );
#55761=CARTESIAN_POINT ( 'NONE',  ( 2.229367062499998831, -55.64583333196773651, -3.861377020970580887 ) ) ;
#55762=CARTESIAN_POINT ( 'NONE',  ( -4.458734124999999437, -11.31249999863440792, 0.000000000000000000 ) ) ;
#55763=CARTESIAN_POINT ( 'NONE',  ( 0.000000000000000000, -170.0000000000000000, 0.000000000000000000 ) ) ;
#55768=CARTESIAN_POINT ( 'NONE',  ( -3.535250795749689387E-16, -33.25000000000000000, -5.773502691896257311 ) ) ;
#55769=DIRECTION ( 'NONE',  ( -0.000000000000000000, 1.000000000000000000, -0.000000000000000000 ) ) ;
#55772=CARTESIAN_POINT ( 'NONE',  ( -2.071067811865432873, -140.8125000027312126, -5.000000000000041744 ) ) ;
#55773=CARTESIAN_POINT ( 'NONE',  ( -2.229367062499996610, -62.14583333196774362, 3.861377020970582219 ) ) ;
#55774=CARTESIAN_POINT ( 'NONE',  ( 3.152801135295367541, -151.5625000013655779, -3.152801135295367541 ) ) ;
#55775=CARTESIAN_POINT ( 'NONE',  ( -4.458734124999999437, -71.31249999863439371, 0.000000000000000000 ) ) ;
#55776=EDGE_CURVE ( 'NONE', #44127, #54337, #15844, .T. ) ;
#55778=CARTESIAN_POINT ( 'NONE',  ( -2.229367062500000163, -21.72916666530107221, -3.861377020970580443 ) ) ;
#55779=( BOUNDED_CURVE ( )  B_SPLINE_CURVE ( 2, ( #19236, #6685, #35315, #54291, #6058, #45278, #20530, #35958, #1244 ),
 .UNSPECIFIED., .F., .F. ) 
 B_SPLINE_CURVE_WITH_KNOTS ( ( 3, 2, 2, 2, 3 ),
 ( 0.7479166666666666741, 0.7486111111111111160, 0.7500000000000000000, 0.7513888888888888840, 0.7520833333333333259 ),
 .UNSPECIFIED. ) 
 CURVE ( )  GEOMETRIC_REPRESENTATION_ITEM ( )  RATIONAL_B_SPLINE_CURVE ( ( 0.9330127018922194093, 0.9330127018922194093, 1.000000000000000000, 0.8660254037844387076, 1.000000000000000000, 0.8660254037844387076, 1.000000000000000000, 0.9330127018922194093, 0.9330127018922194093 ) ) 
 REPRESENTATION_ITEM ( '' )  );
#55780=CARTESIAN_POINT ( 'NONE',  ( -4.999999999999999112, -61.79166666393546592, 2.886751345948131764 ) ) ;
#55782=CARTESIAN_POINT ( 'NONE',  ( -4.999999999999998224, -48.91666666666666430, 2.886751345948131764 ) ) ;
#55785=CARTESIAN_POINT ( 'NONE',  ( 3.152801135295366208, -153.5625000013656063, 3.152801135295367985 ) ) ;
#55786=VERTEX_POINT ( 'NONE', #28485 ) ;
#55787=DIRECTION ( 'NONE',  ( -0.000000000000000000, 1.000000000000000000, -0.000000000000000000 ) ) ;
#55790=CARTESIAN_POINT ( 'NONE',  ( 4.458734124999999437, -48.06249999863440792, -5.460374474430324690E-16 ) ) ;
#55791=VERTEX_POINT ( 'NONE', #53561 ) ;
#55792=EDGE_CURVE ( 'NONE', #28361, #13218, #31422, .T. ) ;
#55796=CARTESIAN_POINT ( 'NONE',  ( -2.229367062500000163, 25.52083333469892779, -3.861377020970580443 ) ) ;
#55799=CARTESIAN_POINT ( 'NONE',  ( -5.000000000000000000, -35.87499999726881583, 0.000000000000000000 ) ) ;
#55809=CYLINDRICAL_SURFACE ( 'NONE', #1929, 5.000000000000000000 ) ;
#55812=ORIENTED_EDGE ( 'NONE', *, *, #9817, .F. ) ;
#55815=CARTESIAN_POINT ( 'NONE',  ( -9.184850993605147944E-16, -157.3750000027311842, 5.000000000000000000 ) ) ;
#55816=ORIENTED_EDGE ( 'NONE', *, *, #5933, .T. ) ;
#55826=CARTESIAN_POINT ( 'NONE',  ( -4.458734124999997661, -27.22916666530107221, 2.574251347313722516 ) ) ;
#55828=CARTESIAN_POINT ( 'NONE',  ( -3.535533905932738641, -150.3750000000000000, 3.535533905932737309 ) ) ;
#55830=CARTESIAN_POINT ( 'NONE',  ( -3.152801135295367096, -151.0625000013655779, -3.152801135295367541 ) ) ;
#55831=ORIENTED_EDGE ( 'NONE', *, *, #1366, .T. ) ;
#55832=CARTESIAN_POINT ( 'NONE',  ( -4.458734124999999437, -51.64583333196773651, -2.574251347313719407 ) ) ;
#55834=DIRECTION ( 'NONE',  ( -0.000000000000000000, 1.000000000000000000, -0.000000000000000000 ) ) ;
#55836=CARTESIAN_POINT ( 'NONE',  ( -3.535250795749689387E-16, 28.74999999999999645, -5.773502691896257311 ) ) ;
#55838=CARTESIAN_POINT ( 'NONE',  ( 4.458734124999999437, 5.187500001365596525, -5.460374474430324690E-16 ) ) ;
#55839=CARTESIAN_POINT ( 'NONE',  ( -3.535533905932738641, -142.3750000000000000, 3.535533905932737309 ) ) ;
#55841=CARTESIAN_POINT ( 'NONE',  ( 5.000000000000000000, -82.41666666666667140, -2.886751345948130876 ) ) ;
#55842=CARTESIAN_POINT ( 'NONE',  ( -2.229367062500000163, 14.27083333469892601, -3.861377020970580443 ) ) ;
#55843=CARTESIAN_POINT ( 'NONE',  ( -5.000000000000000000, 1.041666669397853129, -2.886751345948128211 ) ) ;
#55845=FACE_OUTER_BOUND ( 'NONE', #63047, .T. ) ;
#55846=ORIENTED_EDGE ( 'NONE', *, *, #13302, .F. ) ;
#55848=CARTESIAN_POINT ( 'NONE',  ( -4.458734124999998549, -44.22916666530106511, 2.574251347313722516 ) ) ;
#55849=CARTESIAN_POINT ( 'NONE',  ( -4.458734125000000326, -162.2500000013656347, -1.846868145590735644 ) ) ;
#55850=ADVANCED_FACE ( 'NONE', ( #63537 ), #58702, .T. ) ;
#55853=CARTESIAN_POINT ( 'NONE',  ( -5.000000000000000000, -46.95833333060215153, -2.886751345948128211 ) ) ;
#55855=ORIENTED_EDGE ( 'NONE', *, *, #19301, .F. ) ;
#55856=CARTESIAN_POINT ( 'NONE',  ( 2.229367062499998831, -17.64583333196773651, -3.861377020970580887 ) ) ;
#55858=CARTESIAN_POINT ( 'NONE',  ( -5.000000000000000000, -88.08333333333332860, -2.886751345948128211 ) ) ;
#55859=CARTESIAN_POINT ( 'NONE',  ( -4.458734125000001214, -165.8750000013656063, 1.846868145590734089 ) ) ;
#55862=ORIENTED_EDGE ( 'NONE', *, *, #52729, .T. ) ;
#55864=CARTESIAN_POINT ( 'NONE',  ( -3.152548672688508926E-16, -30.81249999863440436, -5.148502694627439702 ) ) ;
#55865=CARTESIAN_POINT ( 'NONE',  ( 0.000000000000000000, -170.0000000000000000, 0.000000000000000000 ) ) ;
#55875=CARTESIAN_POINT ( 'NONE',  ( 4.458734124999999437, -82.06249999863440792, -5.460374474430324690E-16 ) ) ;
#55877=CARTESIAN_POINT ( 'NONE',  ( -2.498395430326213474E-14, 22.25000000000000000, 5.000000000000000000 ) ) ;
#55878=CARTESIAN_POINT ( 'NONE',  ( 1.846868145590735200, -142.5000000013656063, -4.458734124999999437 ) ) ;
#55879=( BOUNDED_CURVE ( )  B_SPLINE_CURVE ( 2, ( #39078, #19140, #44541, #24612, #4990, #34902, #24291, #40030, #4360 ),
 .UNSPECIFIED., .F., .F. ) 
 B_SPLINE_CURVE_WITH_KNOTS ( ( 3, 2, 2, 2, 3 ),
 ( 0.1562500000000000000, 0.1569444444444444420, 0.1583333333333333259, 0.1597222222222222099, 0.1604166666666666796 ),
 .UNSPECIFIED. ) 
 CURVE ( )  GEOMETRIC_REPRESENTATION_ITEM ( )  RATIONAL_B_SPLINE_CURVE ( ( 0.9330127018922194093, 0.9330127018922194093, 1.000000000000000000, 0.8660254037844387076, 1.000000000000000000, 0.8660254037844387076, 1.000000000000000000, 0.9330127018922180770, 0.9330127018922194093 ) ) 
 REPRESENTATION_ITEM ( '' )  );
#55880=CARTESIAN_POINT ( 'NONE',  ( -6.972266317189433020E-16, -58.24999999999999289, -5.000000000000000000 ) ) ;
#55882=CARTESIAN_POINT ( 'NONE',  ( -3.152548672688508926E-16, -46.56249999863440792, -5.148502694627439702 ) ) ;
#55885=CARTESIAN_POINT ( 'NONE',  ( -6.972266317189433020E-16, -3.250000000000001332, -5.000000000000000000 ) ) ;
#55888=CARTESIAN_POINT ( 'NONE',  ( -2.071067811865308972, -153.4375000027312410, 5.000000000000169642 ) ) ;
#55890=CARTESIAN_POINT ( 'NONE',  ( 2.229367062499998831, -81.89583333196773651, -3.861377020970580887 ) ) ;
#55894=ORIENTED_EDGE ( 'NONE', *, *, #24846, .F. ) ;
#55896=CARTESIAN_POINT ( 'NONE',  ( 0.000000000000000000, -170.0000000000000000, 0.000000000000000000 ) ) ;
#55900=CARTESIAN_POINT ( 'NONE',  ( -4.458734124999997661, 14.52083333469892779, 2.574251347313722516 ) ) ;
#55901=CARTESIAN_POINT ( 'NONE',  ( -6.972266317189433020E-16, -77.12499999726881583, -5.000000000000000000 ) ) ;
#55907=CARTESIAN_POINT ( 'NONE',  ( -5.000000000000000888, -163.5625000000000284, -2.071067811865475949 ) ) ;
#55908=CARTESIAN_POINT ( 'NONE',  ( 2.229367062500001939, -82.97916666530106511, 3.861377020970579999 ) ) ;
#55909=CARTESIAN_POINT ( 'NONE',  ( 2.229367062499998831, -4.645833331967740065, -3.861377020970580887 ) ) ;
#55910=ORIENTED_EDGE ( 'NONE', *, *, #36622, .T. ) ;
#55911=CARTESIAN_POINT ( 'NONE',  ( 4.458734124999998549, -33.97916666530107221, -2.574251347313721627 ) ) ;
#55915=CARTESIAN_POINT ( 'NONE',  ( -3.152548672688508926E-16, 18.43750000136559564, -5.148502694627439702 ) ) ;
#55918=CARTESIAN_POINT ( 'NONE',  ( 2.229367062500001939, -77.22916666530106511, 3.861377020970579999 ) ) ;
#55921=CARTESIAN_POINT ( 'NONE',  ( 5.000000000000000000, 19.70833333606451987, -2.886751345948129988 ) ) ;
#55923=CARTESIAN_POINT ( 'NONE',  ( 5.000000000000000000, -1.291666663935479908, -2.886751345948130876 ) ) ;
#55925=LINE ( 'NONE', #11532, #41040 ) ;
#55926=CARTESIAN_POINT ( 'NONE',  ( 5.000000000000000888, -23.58333333333333215, 2.886751345948126879 ) ) ;
#55927=CARTESIAN_POINT ( 'NONE',  ( 9.457646018065525792E-16, -25.06249999863440792, 5.148502694627439702 ) ) ;
#55928=CARTESIAN_POINT ( 'NONE',  ( -3.152548672688508926E-16, -86.56249999863440792, -5.148502694627439702 ) ) ;
#55930=CARTESIAN_POINT ( 'NONE',  ( -5.000000000000000000, -25.87499999726881583, 0.000000000000000000 ) ) ;
#55931=CARTESIAN_POINT ( 'NONE',  ( -4.458734124999999437, -57.39583333196773651, -2.574251347313719407 ) ) ;
#55934=DIRECTION ( 'NONE',  ( 0.000000000000000000, 0.000000000000000000, 1.000000000000000000 ) ) ;
#55935=CARTESIAN_POINT ( 'NONE',  ( -2.229367062500000163, -1.729166665301071992, -3.861377020970580443 ) ) ;
#55937=CARTESIAN_POINT ( 'NONE',  ( 5.000000000000000000, -72.41666666666667140, -2.886751345948129988 ) ) ;
#55941=EDGE_CURVE ( 'NONE', #28941, #11293, #10443, .T. ) ;
#55942=CARTESIAN_POINT ( 'NONE',  ( -2.071067811865475061, -158.6875000000000568, -5.000000000000000888 ) ) ;
#55943=CARTESIAN_POINT ( 'NONE',  ( 5.000000000000000000, -73.29166666393548724, -2.886751345948129988 ) ) ;
#55944=CARTESIAN_POINT ( 'NONE',  ( -5.000000000000000000, -53.95833333060214443, -2.886751345948128211 ) ) ;
#55946=EDGE_CURVE ( 'NONE', #62883, #2464, #16227, .T. ) ;
#55947=CARTESIAN_POINT ( 'NONE',  ( 9.457646018065525792E-16, -18.31249999863440436, 5.148502694627439702 ) ) ;
#55948=CARTESIAN_POINT ( 'NONE',  ( 2.229367062500001939, -50.22916666530107221, 3.861377020970579999 ) ) ;
#55949=CARTESIAN_POINT ( 'NONE',  ( -3.152801135295367985, -144.8125000013655779, 3.152801135295367096 ) ) ;
#55951=CARTESIAN_POINT ( 'NONE',  ( 3.535533905932736864, -148.2500000027311842, 3.535533905932738641 ) ) ;
#55952=EDGE_LOOP ( 'NONE', ( #34356, #35764, #18814, #58162 ) ) ;
#55953=EDGE_CURVE ( 'NONE', #3670, #44687, #15600, .T. ) ;
#55955=CARTESIAN_POINT ( 'NONE',  ( -2.229367062500000163, 24.27083333469892779, -3.861377020970580443 ) ) ;
#55963=CARTESIAN_POINT ( 'NONE',  ( -3.152801135295367985, -150.0625000013655779, 3.152801135295367096 ) ) ;
#55965=CARTESIAN_POINT ( 'NONE',  ( -4.458734124999999437, -65.64583333196773651, -2.574251347313719407 ) ) ;
#55966=DIRECTION ( 'NONE',  ( -0.000000000000000000, 1.000000000000000000, -0.000000000000000000 ) ) ;
#55967=CARTESIAN_POINT ( 'NONE',  ( -4.458734124999999437, -9.395833331967736513, -2.574251347313719407 ) ) ;
#55968=CARTESIAN_POINT ( 'NONE',  ( -6.972266317189433020E-16, 6.875000002731185944, -5.000000000000000000 ) ) ;
#55969=CARTESIAN_POINT ( 'NONE',  ( -8.190561711645485556E-16, -144.6875000013656063, 4.458734124999999437 ) ) ;
#55972=CARTESIAN_POINT ( 'NONE',  ( -1.339745962155613812, -27.08034179853029499, -5.000000000000000000 ) ) ;
#55976=CARTESIAN_POINT ( 'NONE',  ( -3.152548672688508926E-16, 26.18750000136560274, -5.148502694627439702 ) ) ;
#55977=CARTESIAN_POINT ( 'NONE',  ( 1.975475456537005874E-15, -5.750000000000000000, 5.000000000000000000 ) ) ;
#55984=CARTESIAN_POINT ( 'NONE',  ( -4.458734124999997661, 11.77083333469892601, 2.574251347313722516 ) ) ;
#55986=CARTESIAN_POINT ( 'NONE',  ( -4.458734124999999437, -15.64583333196773829, -2.574251347313719407 ) ) ;
#55988=CARTESIAN_POINT ( 'NONE',  ( 1.846868145590736310, -165.6250000013656063, 4.458734124999999437 ) ) ;
#55989=CARTESIAN_POINT ( 'NONE',  ( -2.500000000000000444, -41.04166666393548013, -4.330127018922193649 ) ) ;
#55993=CARTESIAN_POINT ( 'NONE',  ( -1.339745962155610925, 10.20534180126147739, 5.000000000000000000 ) ) ;
#55995=CARTESIAN_POINT ( 'NONE',  ( -4.458734124999999437, -36.39583333196773651, -2.574251347313719407 ) ) ;
#55999=FACE_OUTER_BOUND ( 'NONE', #20016, .T. ) ;
#56000=ORIENTED_EDGE ( 'NONE', *, *, #4580, .F. ) ;
#56004=CARTESIAN_POINT ( 'NONE',  ( -5.000000000000000000, -10.00000000000000178, 0.000000000000000000 ) ) ;
#56005=CARTESIAN_POINT ( 'NONE',  ( 2.229367062500001939, -73.97916666530106511, 3.861377020970579999 ) ) ;
#56006=CARTESIAN_POINT ( 'NONE',  ( -1.339745962155613812, -17.20534180126147916, -5.000000000000000000 ) ) ;
#56007=CARTESIAN_POINT ( 'NONE',  ( -5.000000000000000000, -7.874999997268813168, 0.000000000000000000 ) ) ;
#56008=CARTESIAN_POINT ( 'NONE',  ( 4.458734124999999437, -37.81249999863440792, -5.460374474430324690E-16 ) ) ;
#56009=ORIENTED_EDGE ( 'NONE', *, *, #57810, .T. ) ;
#56011=CARTESIAN_POINT ( 'NONE',  ( 2.229367062500001939, 14.77083333469892779, 3.861377020970579999 ) ) ;
#56014=DIRECTION ( 'NONE',  ( -0.000000000000000000, 1.000000000000000000, -0.000000000000000000 ) ) ;
#56015=CARTESIAN_POINT ( 'NONE',  ( 5.000000000000000000, -53.41666666666667140, -2.886751345948129988 ) ) ;
#56016=CARTESIAN_POINT ( 'NONE',  ( 4.458734124999999437, -160.7500000013655779, 1.846868145590737864 ) ) ;
#56018=CARTESIAN_POINT ( 'NONE',  ( 1.975475456537005874E-15, -53.74999999999999289, 5.000000000000000000 ) ) ;
#56019=CARTESIAN_POINT ( 'NONE',  ( -3.152548672688508926E-16, -74.56249999863440792, -5.148502694627439702 ) ) ;
#56020=CARTESIAN_POINT ( 'NONE',  ( -4.458734124999999437, -141.1875000013656063, -5.460374474430324690E-16 ) ) ;
#56021=CARTESIAN_POINT ( 'NONE',  ( 2.229367062500001939, -84.97916666530107932, 3.861377020970579999 ) ) ;
#56023=CARTESIAN_POINT ( 'NONE',  ( 2.229367062499998831, -34.89583333196772941, -3.861377020970580887 ) ) ;
#56028=ORIENTED_EDGE ( 'NONE', *, *, #2870, .F. ) ;
#56029=CARTESIAN_POINT ( 'NONE',  ( -2.500000000000000444, -4.041666663935479242, -4.330127018922193649 ) ) ;
#56030=CARTESIAN_POINT ( 'NONE',  ( 6.123233995736766282E-16, -170.0000000000000000, -5.000000000000000000 ) ) ;
#56031=CARTESIAN_POINT ( 'NONE',  ( 9.457646018065525792E-16, -66.31249999863440792, 5.148502694627439702 ) ) ;
#56036=CARTESIAN_POINT ( 'NONE',  ( 5.000000000000000000, -62.41666666666666430, -2.886751345948130876 ) ) ;
#56037=ORIENTED_EDGE ( 'NONE', *, *, #37679, .F. ) ;
#56040=CARTESIAN_POINT ( 'NONE',  ( -2.229367062500000163, 7.520833334698929562, -3.861377020970580443 ) ) ;
#56041=CARTESIAN_POINT ( 'NONE',  ( 5.000000000000000000, -154.0000000000000284, 0.000000000000000000 ) ) ;
#56042=CARTESIAN_POINT ( 'NONE',  ( -3.152801135295367096, -156.0625000013656063, -3.152801135295367541 ) ) ;
#56044=ORIENTED_EDGE ( 'NONE', *, *, #59724, .T. ) ;
#56048=CARTESIAN_POINT ( 'NONE',  ( 5.000000000000000000, -71.37499999726880162, -6.123233995736766282E-16 ) ) ;
#56050=CARTESIAN_POINT ( 'NONE',  ( 0.000000000000000000, -170.0000000000000000, 0.000000000000000000 ) ) ;
#56053=CARTESIAN_POINT ( 'NONE',  ( 4.458734124999998549, 28.27083333469892779, -2.574251347313721627 ) ) ;
#56056=CARTESIAN_POINT ( 'NONE',  ( 2.229367062499998831, 0.1041666680322607397, -3.861377020970580887 ) ) ;
#56060=CARTESIAN_POINT ( 'NONE',  ( -5.000000000000000000, -144.6250000027312126, -6.123233995736766282E-16 ) ) ;
#56061=CARTESIAN_POINT ( 'NONE',  ( -6.972266317189433020E-16, -75.12499999726880162, -5.000000000000000000 ) ) ;
#56065=LINE ( 'NONE', #37698, #42146 ) ;
#56066=CARTESIAN_POINT ( 'NONE',  ( 5.000000000000000000, -22.50000000000000000, -6.123233995736766282E-16 ) ) ;
#56068=CARTESIAN_POINT ( 'NONE',  ( -8.190561711645485556E-16, -159.9375000013655779, 4.458734124999999437 ) ) ;
#56071=ORIENTED_EDGE ( 'NONE', *, *, #35372, .T. ) ;
#56072=CARTESIAN_POINT ( 'NONE',  ( -3.152548672688508926E-16, 21.18750000136559208, -5.148502694627439702 ) ) ;
#56073=ORIENTED_EDGE ( 'NONE', *, *, #49967, .T. ) ;
#56078=CARTESIAN_POINT ( 'NONE',  ( -5.000000000000000000, 9.916666666666667851, -2.886751345948128211 ) ) ;
#56079=CARTESIAN_POINT ( 'NONE',  ( 4.458734124999998549, -58.72916666530106511, -2.574251347313721627 ) ) ;
#56083=CARTESIAN_POINT ( 'NONE',  ( -2.500000000000000444, -37.16666666666666430, -4.330127018922193649 ) ) ;
#56085=CARTESIAN_POINT ( 'NONE',  ( -5.000000000000000000, -40.08333333333332860, -2.886751345948128211 ) ) ;
#56086=CARTESIAN_POINT ( 'NONE',  ( 5.000000000000000000, -149.0625000000000000, 2.071067811865478614 ) ) ;
#56087=CARTESIAN_POINT ( 'NONE',  ( -1.339745962155613812, 14.79465819873851906, -5.000000000000000000 ) ) ;
#56090=CARTESIAN_POINT ( 'NONE',  ( 2.229367062500001939, -59.97916666530106511, 3.861377020970579999 ) ) ;
#56091=CARTESIAN_POINT ( 'NONE',  ( 4.458734124999999437, -152.6875000013656063, 0.000000000000000000 ) ) ;
#56092=CARTESIAN_POINT ( 'NONE',  ( -2.229367062500000163, -71.47916666530107932, -3.861377020970580443 ) ) ;
#56094=CARTESIAN_POINT ( 'NONE',  ( 4.458734124999998549, -17.97916666530106866, -2.574251347313721627 ) ) ;
#56095=CARTESIAN_POINT ( 'NONE',  ( -3.535250795749689387E-16, -59.12499999726880873, -5.773502691896257311 ) ) ;
#56097=CARTESIAN_POINT ( 'NONE',  ( 6.123233995736766282E-16, -170.0000000000000000, -5.000000000000000000 ) ) ;
#56102=CARTESIAN_POINT ( 'NONE',  ( 4.458734125000000326, -153.3750000013656347, -1.846868145590734978 ) ) ;
#56104=CARTESIAN_POINT ( 'NONE',  ( 2.499999999999998668, 25.66666666666666430, -4.330127018922193649 ) ) ;
#56106=FACE_OUTER_BOUND ( 'NONE', #39461, .T. ) ;
#56107=CARTESIAN_POINT ( 'NONE',  ( 2.229367062500001939, -48.22916666530106511, 3.861377020970579999 ) ) ;
#56109=CARTESIAN_POINT ( 'NONE',  ( -5.000000000000000000, 17.12500000273118417, 0.000000000000000000 ) ) ;
#56111=CARTESIAN_POINT ( 'NONE',  ( -2.229367062499996610, 25.85416666803225993, 3.861377020970582219 ) ) ;
#56114=CARTESIAN_POINT ( 'NONE',  ( 4.458734124999999437, -167.3750000013656347, -1.846868145590734978 ) ) ;
#56120=AXIS2_PLACEMENT_3D ( 'NONE', #2905, #36989, #51781 ) ;
#56133=CARTESIAN_POINT ( 'NONE',  ( 2.071067811865476394, -156.3125000027312410, 5.000000000000000000 ) ) ;
#56134=VERTEX_POINT ( 'NONE', #40350 ) ;
#56139=( BOUNDED_CURVE ( )  B_SPLINE_CURVE ( 2, ( #39765, #29477, #59412, #30119, #24674, #49110, #5694, #886, #35278 ),
 .UNSPECIFIED., .F., .F. ) 
 B_SPLINE_CURVE_WITH_KNOTS ( ( 3, 2, 2, 2, 3 ),
 ( 0.6479166666666666963, 0.6486111111111111382, 0.6500000000000000222, 0.6513888888888889062, 0.6520833333333333481 ),
 .UNSPECIFIED. ) 
 CURVE ( )  GEOMETRIC_REPRESENTATION_ITEM ( )  RATIONAL_B_SPLINE_CURVE ( ( 0.9330127018922194093, 0.9330127018922194093, 1.000000000000000000, 0.8660254037844387076, 1.000000000000000000, 0.8660254037844387076, 1.000000000000000000, 0.9330127018922194093, 0.9330127018922194093 ) ) 
 REPRESENTATION_ITEM ( '' )  );
#56141=CARTESIAN_POINT ( 'NONE',  ( 2.071067811865475505, -147.8125000000000284, -5.000000000000000888 ) ) ;
#56145=CARTESIAN_POINT ( 'NONE',  ( -2.229367062500000163, -27.47916666530107221, -3.861377020970580443 ) ) ;
#56146=CARTESIAN_POINT ( 'NONE',  ( -9.184850993605147944E-16, -151.2500000000000284, 5.000000000000000000 ) ) ;
#56148=CARTESIAN_POINT ( 'NONE',  ( -4.458734124999999437, -150.9375000013656063, -5.460374474430324690E-16 ) ) ;
#56149=ORIENTED_EDGE ( 'NONE', *, *, #17370, .F. ) ;
#56150=CARTESIAN_POINT ( 'NONE',  ( 4.458734124999999437, -52.06249999863440792, -5.460374474430324690E-16 ) ) ;
#56151=DIRECTION ( 'NONE',  ( 0.000000000000000000, 0.000000000000000000, 1.000000000000000000 ) ) ;
#56153=CARTESIAN_POINT ( 'NONE',  ( -5.000000000000000000, 23.00000000000000000, 0.000000000000000000 ) ) ;
#56155=CARTESIAN_POINT ( 'NONE',  ( 4.458734124999998549, 2.270833334698928230, -2.574251347313721627 ) ) ;
#56158=CARTESIAN_POINT ( 'NONE',  ( -5.000000000000000888, -142.5625000000000000, -2.071067811865475949 ) ) ;
#56159=EDGE_CURVE ( 'NONE', #8173, #10657, #47035, .T. ) ;
#56160=CARTESIAN_POINT ( 'NONE',  ( 1.975475456537005874E-15, -37.62499999726880873, 5.000000000000000000 ) ) ;
#56161=CYLINDRICAL_SURFACE ( 'NONE', #49903, 5.000000000000000000 ) ;
#56162=CARTESIAN_POINT ( 'NONE',  ( 4.458734124999999437, 17.93750000136559208, -5.460374474430324690E-16 ) ) ;
#56163=CARTESIAN_POINT ( 'NONE',  ( -3.535250795749689387E-16, 4.875000002731184168, -5.773502691896257311 ) ) ;
#56165=ORIENTED_EDGE ( 'NONE', *, *, #13377, .T. ) ;
#56167=CARTESIAN_POINT ( 'NONE',  ( -1.339745962155610925, -70.79465819873850307, 5.000000000000000000 ) ) ;
#56168=CARTESIAN_POINT ( 'NONE',  ( 2.229367062499998831, -41.64583333196773651, -3.861377020970580887 ) ) ;
#56169=CARTESIAN_POINT ( 'NONE',  ( -3.152801135295367985, -162.0625000013656063, 3.152801135295367096 ) ) ;
#56172=CARTESIAN_POINT ( 'NONE',  ( -3.535250795749689387E-16, -47.12499999726880873, -5.773502691896257311 ) ) ;
#56174=CARTESIAN_POINT ( 'NONE',  ( -2.229367062500000163, -19.47916666530106866, -3.861377020970580443 ) ) ;
#56175=ORIENTED_EDGE ( 'NONE', *, *, #8811, .T. ) ;
#56176=CARTESIAN_POINT ( 'NONE',  ( 5.000000000000000888, -89.58333333333334281, 2.886751345948126879 ) ) ;
#56177=CARTESIAN_POINT ( 'NONE',  ( -8.190561711645485556E-16, -165.6875000013655779, 4.458734124999999437 ) ) ;
#56181=CARTESIAN_POINT ( 'NONE',  ( 4.458734124999999437, -33.06249999863440792, -5.460374474430324690E-16 ) ) ;
#56186=CARTESIAN_POINT ( 'NONE',  ( -1.339745962155610925, -28.66965819600733312, 5.000000000000000000 ) ) ;
#56188=CARTESIAN_POINT ( 'NONE',  ( -5.000000000000000000, -161.5000000000000000, -6.123233995736766282E-16 ) ) ;
#56190=CARTESIAN_POINT ( 'NONE',  ( -3.152548672688508926E-16, -80.81249999863440792, -5.148502694627439702 ) ) ;
#56193=CARTESIAN_POINT ( 'NONE',  ( -1.846868145590734756, -143.3750000013656063, -4.458734124999999437 ) ) ;
#56194=CARTESIAN_POINT ( 'NONE',  ( 1.339745962155612702, -84.16965819600731891, -5.000000000000000000 ) ) ;
#56196=CARTESIAN_POINT ( 'NONE',  ( 4.458734124999998549, -45.72916666530106511, -2.574251347313721627 ) ) ;
#56199=CARTESIAN_POINT ( 'NONE',  ( -2.500000000000000444, 3.833333333333334370, -4.330127018922193649 ) ) ;
#56202=LINE ( 'NONE', #37523, #56373 ) ;
#56203=CARTESIAN_POINT ( 'NONE',  ( 4.458734124999998549, -78.97916666530106511, -2.574251347313721627 ) ) ;
#56208=ORIENTED_EDGE ( 'NONE', *, *, #26033, .T. ) ;
#56210=CARTESIAN_POINT ( 'NONE',  ( -6.972266317189433020E-16, -47.12499999726880873, -5.000000000000000000 ) ) ;
#56213=CARTESIAN_POINT ( 'NONE',  ( -2.071067811865475061, -168.8125000027312126, -5.000000000000000888 ) ) ;
#56216=AXIS2_PLACEMENT_3D ( 'NONE', #39319, #29339, #48972 ) ;
#56217=CARTESIAN_POINT ( 'NONE',  ( 4.458734125000000326, 14.85416666803225993, 2.574251347313718519 ) ) ;
#56218=CARTESIAN_POINT ( 'NONE',  ( 1.975475456537005874E-15, -73.62499999726878741, 5.000000000000000000 ) ) ;
#56219=VECTOR ( 'NONE', #45277, 1000.000000000000000 ) ;
#56226=CARTESIAN_POINT ( 'NONE',  ( 4.458734124999998549, -85.72916666530106511, -2.574251347313721627 ) ) ;
#56227=CARTESIAN_POINT ( 'NONE',  ( -4.458734124999999437, -8.395833331967736513, -2.574251347313719407 ) ) ;
#56230=CARTESIAN_POINT ( 'NONE',  ( -4.458734124999999437, -34.64583333196772941, -2.574251347313719407 ) ) ;
#56234=CARTESIAN_POINT ( 'NONE',  ( 3.152801135295367541, -148.5625000013655779, -3.152801135295367541 ) ) ;
#56235=CARTESIAN_POINT ( 'NONE',  ( -2.229367062500000163, 21.52083333469892779, -3.861377020970580443 ) ) ;
#56238=CARTESIAN_POINT ( 'NONE',  ( 2.500000000000002220, 1.333333333333332149, 4.330127018922192761 ) ) ;
#56239=CARTESIAN_POINT ( 'NONE',  ( -3.152548672688508926E-16, -83.81249999863437949, -5.148502694627439702 ) ) ;
#56242=CARTESIAN_POINT ( 'NONE',  ( -2.499999999999996447, 17.29166666939785557, 4.330127018922195425 ) ) ;
#56243=ORIENTED_EDGE ( 'NONE', *, *, #14083, .T. ) ;
#56244=CARTESIAN_POINT ( 'NONE',  ( 5.000000000000000000, -147.1875000027312410, 2.071067811865478614 ) ) ;
#56248=CARTESIAN_POINT ( 'NONE',  ( 1.060575238724906964E-15, -21.75000000000000000, 5.773502691896257311 ) ) ;
#56249=CARTESIAN_POINT ( 'NONE',  ( 2.229367062500001939, -29.97916666530107221, 3.861377020970579999 ) ) ;
#56250=CARTESIAN_POINT ( 'NONE',  ( -3.152548672688508926E-16, -89.56249999863439371, -5.148502694627439702 ) ) ;
#56251=CARTESIAN_POINT ( 'NONE',  ( -5.000000000000000000, -27.87499999726880873, 0.000000000000000000 ) ) ;
#56252=CARTESIAN_POINT ( 'NONE',  ( 4.458734124999998549, -53.72916666530106511, -2.574251347313721627 ) ) ;
#56253=ORIENTED_EDGE ( 'NONE', *, *, #28252, .T. ) ;
#56255=CARTESIAN_POINT ( 'NONE',  ( 4.458734124999999437, -5.062499998634402587, -5.460374474430324690E-16 ) ) ;
#56256=ORIENTED_EDGE ( 'NONE', *, *, #39714, .T. ) ;
#56257=CARTESIAN_POINT ( 'NONE',  ( -3.535250795749689387E-16, -71.25000000000000000, -5.773502691896257311 ) ) ;
#56261=VECTOR ( 'NONE', #31584, 1000.000000000000000 ) ;
#56262=CARTESIAN_POINT ( 'NONE',  ( 2.499999999999998668, -77.20833333060214443, -4.330127018922193649 ) ) ;
#56263=CARTESIAN_POINT ( 'NONE',  ( -4.999999999999998224, -85.91666666666667140, 2.886751345948131764 ) ) ;
#56266=CARTESIAN_POINT ( 'NONE',  ( 4.458734124999999437, -18.06249999863440792, -5.460374474430324690E-16 ) ) ;
#56267=AXIS2_PLACEMENT_3D ( 'NONE', #62253, #38415, #58039 ) ;
#56268=CARTESIAN_POINT ( 'NONE',  ( 9.457646018065525792E-16, -54.31249999863440081, 5.148502694627439702 ) ) ;
#56269=CARTESIAN_POINT ( 'NONE',  ( 1.846868145590736310, -140.6250000013656063, 4.458734124999999437 ) ) ;
#56273=DIRECTION ( 'NONE',  ( -0.000000000000000000, 1.000000000000000000, -0.000000000000000000 ) ) ;
#56278=CARTESIAN_POINT ( 'NONE',  ( 4.458734125000000326, -147.6250000013655779, -1.846868145590734978 ) ) ;
#56282=CARTESIAN_POINT ( 'NONE',  ( 4.458734124999998549, -65.97916666530106511, -2.574251347313721627 ) ) ;
#56284=CARTESIAN_POINT ( 'NONE',  ( -6.972266317189433020E-16, -55.24999999999999289, -5.000000000000000000 ) ) ;
#56285=CARTESIAN_POINT ( 'NONE',  ( 1.846868145590735200, -144.2500000013656063, -4.458734124999999437 ) ) ;
#56291=CARTESIAN_POINT ( 'NONE',  ( 2.229367062500001939, 28.77083333469892779, 3.861377020970579999 ) ) ;
#56292=CARTESIAN_POINT ( 'NONE',  ( -1.339745962155613812, -18.08034179853029499, -5.000000000000000000 ) ) ;
#56301=EDGE_CURVE ( 'NONE', #50806, #11542, #11704, .T. ) ;
#56302=CARTESIAN_POINT ( 'NONE',  ( 2.229367062500001939, 9.020833334698927786, 3.861377020970579999 ) ) ;
#56304=CARTESIAN_POINT ( 'NONE',  ( -4.458734124999997661, -18.47916666530106511, 2.574251347313722516 ) ) ;
#56305=EDGE_CURVE ( 'NONE', #62567, #5493, #28408, .T. ) ;
#56308=CARTESIAN_POINT ( 'NONE',  ( 3.152801135295367541, -161.3125000013656063, -3.152801135295367541 ) ) ;
#56311=CIRCLE ( 'NONE', #36788, 5.000000000000000000 ) ;
#56312=EDGE_CURVE ( 'NONE', #5760, #47469, #3092, .T. ) ;
#56316=CARTESIAN_POINT ( 'NONE',  ( -4.458734124999997661, -33.22916666530106511, 2.574251347313722516 ) ) ;
#56319=CARTESIAN_POINT ( 'NONE',  ( -3.152548672688508926E-16, -69.81249999863439371, -5.148502694627439702 ) ) ;
#56322=EDGE_CURVE ( 'NONE', #62531, #25786, #23598, .T. ) ;
#56323=EDGE_LOOP ( 'NONE', ( #17749, #39662, #39513, #238 ) ) ;
#56326=DIRECTION ( 'NONE',  ( -0.000000000000000000, 1.000000000000000000, -0.000000000000000000 ) ) ;
#56328=CARTESIAN_POINT ( 'NONE',  ( 5.000000000000000000, -8.416666666666669627, -2.886751345948129988 ) ) ;
#56330=CARTESIAN_POINT ( 'NONE',  ( 4.458734124999999437, -70.81249999863439371, -5.460374474430324690E-16 ) ) ;
#56333=CARTESIAN_POINT ( 'NONE',  ( 5.000000000000000000, -13.29166666393548191, -2.886751345948129988 ) ) ;
#56334=CARTESIAN_POINT ( 'NONE',  ( 4.458734124999999437, -40.81249999863440081, -5.460374474430324690E-16 ) ) ;
#56335=VERTEX_POINT ( 'NONE', #62529 ) ;
#56336=CARTESIAN_POINT ( 'NONE',  ( 1.975475456537005874E-15, -41.74999999999999289, 5.000000000000000000 ) ) ;
#56337=CARTESIAN_POINT ( 'NONE',  ( 2.229367062500001939, 11.77083333469892601, 3.861377020970579999 ) ) ;
#56338=ORIENTED_EDGE ( 'NONE', *, *, #42224, .F. ) ;
#56339=CARTESIAN_POINT ( 'NONE',  ( -2.071067811865348496, -151.6875000000000000, -5.000000000000127898 ) ) ;
#56340=CARTESIAN_POINT ( 'NONE',  ( -4.999999999999999112, -57.91666666666665719, 2.886751345948131764 ) ) ;
#56341=CARTESIAN_POINT ( 'NONE',  ( -8.190561711645485556E-16, -160.9375000013655779, 4.458734124999999437 ) ) ;
#56343=LINE ( 'NONE', #22237, #22472 ) ;
#56344=CARTESIAN_POINT ( 'NONE',  ( 4.458734125000001214, -79.89583333196773651, 2.574251347313718519 ) ) ;
#56345=CARTESIAN_POINT ( 'NONE',  ( 3.535533905932738197, -169.8750000000000284, -3.535533905932738197 ) ) ;
#56346=CARTESIAN_POINT ( 'NONE',  ( 4.458734124999998549, -86.72916666530107932, -2.574251347313721627 ) ) ;
#56348=CARTESIAN_POINT ( 'NONE',  ( 9.457646018065525792E-16, -0.3124999986344051961, 5.148502694627439702 ) ) ;
#56349=CARTESIAN_POINT ( 'NONE',  ( 4.458734125000001214, -36.14583333196773651, 2.574251347313718519 ) ) ;
#56350=( BOUNDED_CURVE ( )  B_SPLINE_CURVE ( 2, ( #23504, #28002, #3577, #23183, #62437, #37980, #57611, #9324, #43731 ),
 .UNSPECIFIED., .F., .F. ) 
 B_SPLINE_CURVE_WITH_KNOTS ( ( 3, 2, 2, 2, 3 ),
 ( 0.8020833333333333703, 0.8027777777777778123, 0.8041666666666666963, 0.8055555555555555802, 0.8062500000000000222 ),
 .UNSPECIFIED. ) 
 CURVE ( )  GEOMETRIC_REPRESENTATION_ITEM ( )  RATIONAL_B_SPLINE_CURVE ( ( 0.9330127018922194093, 0.9330127018922194093, 1.000000000000000000, 0.8660254037844387076, 1.000000000000000000, 0.8660254037844387076, 1.000000000000000000, 0.9330127018922194093, 0.9330127018922194093 ) ) 
 REPRESENTATION_ITEM ( '' )  );
#56351=CARTESIAN_POINT ( 'NONE',  ( -6.972266317189433020E-16, -72.25000000000000000, -5.000000000000000000 ) ) ;
#56354=ORIENTED_EDGE ( 'NONE', *, *, #42929, .T. ) ;
#56357=LINE ( 'NONE', #32521, #46578 ) ;
#56358=CARTESIAN_POINT ( 'NONE',  ( 2.229367062499998831, -70.89583333196773651, -3.861377020970580887 ) ) ;
#56361=CARTESIAN_POINT ( 'NONE',  ( -3.535533905932738641, -150.5000000027312126, 3.535533905932737309 ) ) ;
#56364=CARTESIAN_POINT ( 'NONE',  ( 4.458734125000001214, 7.104166668032259047, 2.574251347313718519 ) ) ;
#56365=LINE ( 'NONE', #61188, #4855 ) ;
#56366=CARTESIAN_POINT ( 'NONE',  ( -3.152801135295367985, -158.8125000013656063, 3.152801135295367096 ) ) ;
#56368=ORIENTED_EDGE ( 'NONE', *, *, #15269, .F. ) ;
#56372=CARTESIAN_POINT ( 'NONE',  ( 2.071067811865434205, -140.1874999999999716, 5.000000000000041744 ) ) ;
#56373=VECTOR ( 'NONE', #57164, 1000.000000000000000 ) ;
#56378=CARTESIAN_POINT ( 'NONE',  ( -4.458734124999999437, 27.68750000136559208, 0.000000000000000000 ) ) ;
#56381=CARTESIAN_POINT ( 'NONE',  ( -4.458734124999997661, -3.479166665301069994, 2.574251347313722516 ) ) ;
#56382=CARTESIAN_POINT ( 'NONE',  ( 2.499999999999998668, -0.2083333306021478704, -4.330127018922193649 ) ) ;
#56384=CARTESIAN_POINT ( 'NONE',  ( 3.535533905932736864, -143.2500000027311842, 3.535533905932738641 ) ) ;
#56389=CARTESIAN_POINT ( 'NONE',  ( 0.000000000000000000, -170.0000000000000000, 5.000000000000000000 ) ) ;
#56392=CARTESIAN_POINT ( 'NONE',  ( -4.458734124999999437, -162.2500000013656063, -1.846868145590735644 ) ) ;
#56393=( BOUNDED_CURVE ( )  B_SPLINE_CURVE ( 2, ( #59492, #35049, #25715, #35684, #54344, #40183, #29880, #44355, #54661 ),
 .UNSPECIFIED., .F., .F. ) 
 B_SPLINE_CURVE_WITH_KNOTS ( ( 3, 2, 2, 2, 3 ),
 ( 0.8812499999999999778, 0.8819444444444444198, 0.8833333333333333037, 0.8847222222222221877, 0.8854166666666666297 ),
 .UNSPECIFIED. ) 
 CURVE ( )  GEOMETRIC_REPRESENTATION_ITEM ( )  RATIONAL_B_SPLINE_CURVE ( ( 0.9330127018922194093, 0.9330127018922194093, 1.000000000000000000, 0.8660254037844387076, 1.000000000000000000, 0.8660254037844387076, 1.000000000000000000, 0.9330127018922194093, 0.9330127018922194093 ) ) 
 REPRESENTATION_ITEM ( '' )  );
#56397=EDGE_CURVE ( 'NONE', #54515, #3670, #22433, .T. ) ;
#56398=CARTESIAN_POINT ( 'NONE',  ( -2.229367062500000163, 20.27083333469892779, -3.861377020970580443 ) ) ;
#56399=ORIENTED_EDGE ( 'NONE', *, *, #28053, .F. ) ;
#56405=CARTESIAN_POINT ( 'NONE',  ( -5.000000000000000000, 9.000000000000001776, 0.000000000000000000 ) ) ;
#56406=CARTESIAN_POINT ( 'NONE',  ( -2.229367062500000163, -54.47916666530107221, -3.861377020970580443 ) ) ;
#56408=EDGE_CURVE ( 'NONE', #2867, #5270, #35574, .T. ) ;
#56410=LINE ( 'NONE', #41904, #50223 ) ;
#56411=CARTESIAN_POINT ( 'NONE',  ( -2.500000000000000444, -64.16666666666665719, -4.330127018922193649 ) ) ;
#56413=CARTESIAN_POINT ( 'NONE',  ( 1.060575238724906964E-15, -39.75000000000000000, 5.773502691896257311 ) ) ;
#56414=CARTESIAN_POINT ( 'NONE',  ( -1.339745962155613812, 12.91965820146970678, -5.000000000000000000 ) ) ;
#56415=CARTESIAN_POINT ( 'NONE',  ( -4.999999999999998224, 15.08333333333333215, 2.886751345948131764 ) ) ;
#56417=CARTESIAN_POINT ( 'NONE',  ( -5.000000000000000000, 13.00000000000000178, 0.000000000000000000 ) ) ;
#56418=CARTESIAN_POINT ( 'NONE',  ( 9.457646018065525792E-16, -66.06249999863440792, 5.148502694627439702 ) ) ;
#56419=CARTESIAN_POINT ( 'NONE',  ( 3.152801135295367541, -152.5625000013655779, -3.152801135295367541 ) ) ;
#56420=CARTESIAN_POINT ( 'NONE',  ( -4.458734124999999437, -71.39583333196773651, -2.574251347313719407 ) ) ;
#56422=CARTESIAN_POINT ( 'NONE',  ( 4.458734125000001214, -17.14583333196773651, 2.574251347313718519 ) ) ;
#56423=CARTESIAN_POINT ( 'NONE',  ( 2.500000000000002220, -58.54166666393548013, 4.330127018922192761 ) ) ;
#56424=ORIENTED_EDGE ( 'NONE', *, *, #59779, .F. ) ;
#56430=CARTESIAN_POINT ( 'NONE',  ( -4.458734124999999437, -151.9375000013655779, -5.460374474430324690E-16 ) ) ;
#56432=CARTESIAN_POINT ( 'NONE',  ( 3.535533905932736864, -155.2500000027312126, 3.535533905932738641 ) ) ;
#56435=CARTESIAN_POINT ( 'NONE',  ( -2.229367062500000163, -50.72916666530107221, -3.861377020970580443 ) ) ;
#56439=CARTESIAN_POINT ( 'NONE',  ( 2.229367062500001939, 26.02083333469892779, 3.861377020970579999 ) ) ;
#56442=CARTESIAN_POINT ( 'NONE',  ( 3.535533905932736864, -165.1250000000000284, 3.535533905932738641 ) ) ;
#56443=( BOUNDED_CURVE ( )  B_SPLINE_CURVE ( 2, ( #33886, #14892, #29352, #14266, #34499, #30005, #35170, #20698, #53506 ),
 .UNSPECIFIED., .F., .F. ) 
 B_SPLINE_CURVE_WITH_KNOTS ( ( 3, 2, 2, 2, 3 ),
 ( 0.006250000000000000347, 0.006944444444444444059, 0.008333333333333333218, 0.009722222222222222376, 0.01041666666666666782 ),
 .UNSPECIFIED. ) 
 CURVE ( )  GEOMETRIC_REPRESENTATION_ITEM ( )  RATIONAL_B_SPLINE_CURVE ( ( 0.9330127018922194093, 0.9330127018922194093, 1.000000000000000000, 0.8660254037844387076, 1.000000000000000000, 0.8660254037844387076, 1.000000000000000000, 0.9330127018922191873, 0.9330127018922192983 ) ) 
 REPRESENTATION_ITEM ( '' )  );
#56448=VECTOR ( 'NONE', #6397, 1000.000000000000000 ) ;
#56454=CARTESIAN_POINT ( 'NONE',  ( -6.972266317189433020E-16, 18.74999999999999645, -5.000000000000000000 ) ) ;
#56458=DIRECTION ( 'NONE',  ( -0.000000000000000000, 1.000000000000000000, -0.000000000000000000 ) ) ;
#56460=CARTESIAN_POINT ( 'NONE',  ( -9.184850993605147944E-16, -155.3750000027311842, 5.000000000000000000 ) ) ;
#56461=ORIENTED_EDGE ( 'NONE', *, *, #25667, .F. ) ;
#56466=CARTESIAN_POINT ( 'NONE',  ( -2.071067811865478170, -146.3125000000000000, 5.000000000000000000 ) ) ;
#56469=CARTESIAN_POINT ( 'NONE',  ( -1.339745962155610925, -89.79465819873851729, 5.000000000000000000 ) ) ;
#56470=CARTESIAN_POINT ( 'NONE',  ( 4.458734124999998549, -25.72916666530107221, -2.574251347313721627 ) ) ;
#56474=CARTESIAN_POINT ( 'NONE',  ( -4.458734125000000326, -152.0000000013655779, -1.846868145590735644 ) ) ;
#56475=EDGE_LOOP ( 'NONE', ( #32626, #59844, #34469, #57346 ) ) ;
#56477=CARTESIAN_POINT ( 'NONE',  ( 2.229367062500001939, -53.22916666530107221, 3.861377020970579999 ) ) ;
#56478=CYLINDRICAL_SURFACE ( 'NONE', #12988, 5.000000000000000000 ) ;
#56480=CARTESIAN_POINT ( 'NONE',  ( -2.499999999999996447, 26.16666666666666430, 4.330127018922195425 ) ) ;
#56482=CARTESIAN_POINT ( 'NONE',  ( 9.457646018065525792E-16, 0.9375000013655959696, 5.148502694627439702 ) ) ;
#56483=DIRECTION ( 'NONE',  ( -0.000000000000000000, 0.000000000000000000, -1.000000000000000000 ) ) ;
#56484=CARTESIAN_POINT ( 'NONE',  ( -5.000000000000000888, -164.5625000000000000, -2.071067811865475949 ) ) ;
#56486=CARTESIAN_POINT ( 'NONE',  ( -4.458734124999999437, 15.43750000136559386, 0.000000000000000000 ) ) ;
#56487=CARTESIAN_POINT ( 'NONE',  ( 5.000000000000000888, 0.5416666693978527958, 2.886751345948126879 ) ) ;
#56488=VERTEX_POINT ( 'NONE', #55082 ) ;
#56489=CARTESIAN_POINT ( 'NONE',  ( 6.042630808230842148E-15, 26.75000000000000000, -4.999999999999999112 ) ) ;
#56490=ORIENTED_EDGE ( 'NONE', *, *, #27184, .F. ) ;
#56491=PRODUCT_DEFINITION_FORMATION_WITH_SPECIFIED_SOURCE ( 'ANY', '', #24548, .NOT_KNOWN. ) ;
#56492=CARTESIAN_POINT ( 'NONE',  ( 5.000000000000000000, 27.62500000273118417, -6.123233995736766282E-16 ) ) ;
#56493=CARTESIAN_POINT ( 'NONE',  ( -2.229367062499996610, -45.14583333196774362, 3.861377020970582219 ) ) ;
#56494=CARTESIAN_POINT ( 'NONE',  ( -3.152801135295367096, -165.3125000013656063, -3.152801135295367541 ) ) ;
#56495=CARTESIAN_POINT ( 'NONE',  ( -2.500000000000000444, -45.04166666393547303, -4.330127018922193649 ) ) ;
#56497=CARTESIAN_POINT ( 'NONE',  ( 2.229367062500001939, -19.97916666530107221, 3.861377020970579999 ) ) ;
#56499=CARTESIAN_POINT ( 'NONE',  ( -3.535250795749689387E-16, -89.25000000000000000, -5.773502691896257311 ) ) ;
#56500=CARTESIAN_POINT ( 'NONE',  ( 3.152801135295367541, -163.3125000013656063, -3.152801135295367541 ) ) ;
#56501=DIRECTION ( 'NONE',  ( -0.000000000000000000, 1.000000000000000000, -0.000000000000000000 ) ) ;
#56503=EDGE_CURVE ( 'NONE', #39231, #27765, #22813, .T. ) ;
#56504=CARTESIAN_POINT ( 'NONE',  ( 2.229367062499998831, -30.89583333196773651, -3.861377020970580887 ) ) ;
#56506=ORIENTED_EDGE ( 'NONE', *, *, #58695, .T. ) ;
#56513=CARTESIAN_POINT ( 'NONE',  ( 2.229367062499998831, -77.89583333196773651, -3.861377020970580887 ) ) ;
#56517=CARTESIAN_POINT ( 'NONE',  ( 2.500000000000002220, 24.33333333333333215, 4.330127018922192761 ) ) ;
#56519=CARTESIAN_POINT ( 'NONE',  ( 4.458734125000000326, -43.89583333196773651, 2.574251347313718519 ) ) ;
#56520=CARTESIAN_POINT ( 'NONE',  ( -6.972266317189433020E-16, 20.74999999999999645, -5.000000000000000000 ) ) ;
#56523=CARTESIAN_POINT ( 'NONE',  ( 2.071067811865582087, -159.3125000027311842, 4.999999999999894307 ) ) ;
#56528=CARTESIAN_POINT ( 'NONE',  ( 2.229367062500001939, -77.22916666530106511, 3.861377020970579999 ) ) ;
#56533=CARTESIAN_POINT ( 'NONE',  ( 5.000000000000000000, -47.41666666666666430, -2.886751345948130876 ) ) ;
#56535=CARTESIAN_POINT ( 'NONE',  ( 5.000000000000000888, -169.0625000027312126, -2.071067811865475505 ) ) ;
#56538=CARTESIAN_POINT ( 'NONE',  ( -4.458734124999997661, 10.52083333469892779, 2.574251347313722516 ) ) ;
#56546=CARTESIAN_POINT ( 'NONE',  ( 1.975475456537005874E-15, -21.62499999726880873, 5.000000000000000000 ) ) ;
#56547=CARTESIAN_POINT ( 'NONE',  ( -3.152548672688508926E-16, -11.56249999863440792, -5.148502694627439702 ) ) ;
#56549=CARTESIAN_POINT ( 'NONE',  ( 4.458734124999999437, -36.06249999863440792, -5.460374474430324690E-16 ) ) ;
#56551=LINE ( 'NONE', #22770, #52446 ) ;
#56554=CARTESIAN_POINT ( 'NONE',  ( 1.846868145590735200, -151.5000000013655779, -4.458734124999999437 ) ) ;
#56555=CARTESIAN_POINT ( 'NONE',  ( -4.458734124999999437, 20.60416666803225993, -2.574251347313719407 ) ) ;
#56557=CARTESIAN_POINT ( 'NONE',  ( -4.458734124999999437, -82.64583333196773651, -2.574251347313719407 ) ) ;
#56559=DIRECTION ( 'NONE',  ( -0.000000000000000000, 1.000000000000000000, -0.000000000000000000 ) ) ;
#56560=CARTESIAN_POINT ( 'NONE',  ( 2.499999999999998668, 17.79166666939785557, -4.330127018922193649 ) ) ;
#56564=FACE_OUTER_BOUND ( 'NONE', #47629, .T. ) ;
#56565=CARTESIAN_POINT ( 'NONE',  ( -2.500000000000000444, -25.16666666666666430, -4.330127018922193649 ) ) ;
#56566=CARTESIAN_POINT ( 'NONE',  ( -2.229367062499996610, -30.14583333196773651, 3.861377020970582219 ) ) ;
#56567=CARTESIAN_POINT ( 'NONE',  ( -4.458734124999999437, -87.31249999863439371, 0.000000000000000000 ) ) ;
#56568=CARTESIAN_POINT ( 'NONE',  ( 5.000000000000000000, -26.29166666393547658, -2.886751345948129988 ) ) ;
#56569=CARTESIAN_POINT ( 'NONE',  ( -2.229367062500000163, -60.47916666530106511, -3.861377020970580443 ) ) ;
#56570=ORIENTED_EDGE ( 'NONE', *, *, #19321, .F. ) ;
#56572=CARTESIAN_POINT ( 'NONE',  ( 4.458734125000001214, -10.14583333196773829, 2.574251347313718519 ) ) ;
#56573=EDGE_LOOP ( 'NONE', ( #51018, #22709, #51527, #33445 ) ) ;
#56574=CARTESIAN_POINT ( 'NONE',  ( 2.500000000000002220, -73.66666666666665719, 4.330127018922192761 ) ) ;
#56576=AXIS2_PLACEMENT_3D ( 'NONE', #52570, #18469, #8503 ) ;
#56578=CARTESIAN_POINT ( 'NONE',  ( -4.999999999999999112, -76.79166666393547303, 2.886751345948131764 ) ) ;
#56579=CARTESIAN_POINT ( 'NONE',  ( -6.972266317189433020E-16, -54.12499999726880162, -5.000000000000000000 ) ) ;
#56584=CARTESIAN_POINT ( 'NONE',  ( -3.152548672688508926E-16, -14.81249999863440436, -5.148502694627439702 ) ) ;
#56585=CARTESIAN_POINT ( 'NONE',  ( -2.229367062499996610, -57.39583333196773651, 3.861377020970582219 ) ) ;
#56586=CARTESIAN_POINT ( 'NONE',  ( -4.999999999999998224, -29.79166666393548013, 2.886751345948131764 ) ) ;
#56587=( NAMED_UNIT ( * ) SI_UNIT ( $, .STERADIAN. ) SOLID_ANGLE_UNIT ( ) );
#56588=CARTESIAN_POINT ( 'NONE',  ( 4.458734124999999437, -169.6875000013656063, 0.000000000000000000 ) ) ;
#56590=CARTESIAN_POINT ( 'NONE',  ( 5.000000000000000000, -148.1250000027312126, 0.000000000000000000 ) ) ;
#56591=VERTEX_POINT ( 'NONE', #34823 ) ;
#56594=( BOUNDED_CURVE ( )  B_SPLINE_CURVE ( 2, ( #56489, #41350, #26894, #16916, #22389, #18180, #2150, #61311, #46512 ),
 .UNSPECIFIED., .F., .F. ) 
 B_SPLINE_CURVE_WITH_KNOTS ( ( 3, 2, 2, 2, 3 ),
 ( 0.02708333333333333426, 0.02777777777777777624, 0.02916666666666666713, 0.03055555555555555455, 0.03125000000000000000 ),
 .UNSPECIFIED. ) 
 CURVE ( )  GEOMETRIC_REPRESENTATION_ITEM ( )  RATIONAL_B_SPLINE_CURVE ( ( 0.9330127018922194093, 0.9330127018922195203, 1.000000000000000000, 0.8660254037844387076, 1.000000000000000000, 0.8660254037844387076, 1.000000000000000000, 0.9330127018922191873, 0.9330127018922194093 ) ) 
 REPRESENTATION_ITEM ( '' )  );
#56599=CARTESIAN_POINT ( 'NONE',  ( -1.846868145590734756, -147.3750000013656063, -4.458734125000000326 ) ) ;
#56604=CARTESIAN_POINT ( 'NONE',  ( -2.229367062500000163, -61.72916666530106511, -3.861377020970580443 ) ) ;
#56605=CARTESIAN_POINT ( 'NONE',  ( -6.972266317189433020E-16, -50.12499999726881583, -5.000000000000000000 ) ) ;
#56607=CARTESIAN_POINT ( 'NONE',  ( -1.846868145590734756, -143.1250000013656063, -4.458734124999999437 ) ) ;
#56609=ORIENTED_EDGE ( 'NONE', *, *, #41756, .F. ) ;
#56614=DIRECTION ( 'NONE',  ( 0.000000000000000000, 0.000000000000000000, 1.000000000000000000 ) ) ;
#56617=CARTESIAN_POINT ( 'NONE',  ( -6.972266317189433020E-16, -76.12499999726880162, -5.000000000000000000 ) ) ;
#56624=CARTESIAN_POINT ( 'NONE',  ( 4.458734124999999437, 5.187500001365596525, -5.460374474430324690E-16 ) ) ;
#56626=CARTESIAN_POINT ( 'NONE',  ( 4.458734125000000326, -20.14583333196774007, 2.574251347313718519 ) ) ;
#56629=CARTESIAN_POINT ( 'NONE',  ( -3.152801135295367096, -159.0625000013656063, -3.152801135295367541 ) ) ;
#56630=CARTESIAN_POINT ( 'NONE',  ( -5.000000000000000888, -158.5625000000000284, -2.071067811865475949 ) ) ;
#56634=CARTESIAN_POINT ( 'NONE',  ( 2.229367062500001939, -38.97916666530107221, 3.861377020970579999 ) ) ;
#56635=EDGE_CURVE ( 'NONE', #19199, #15810, #28972, .T. ) ;
#56636=CARTESIAN_POINT ( 'NONE',  ( 6.123233995736766282E-16, -170.0000000000000000, -5.000000000000000000 ) ) ;
#56637=CARTESIAN_POINT ( 'NONE',  ( -2.229367062499996610, -65.39583333196773651, 3.861377020970582219 ) ) ;
#56641=ORIENTED_EDGE ( 'NONE', *, *, #56664, .F. ) ;
#56644=CARTESIAN_POINT ( 'NONE',  ( -2.500000000000000444, -8.166666666666669627, -4.330127018922193649 ) ) ;
#56645=CARTESIAN_POINT ( 'NONE',  ( -2.229367062500000163, -71.47916666530107932, -3.861377020970580443 ) ) ;
#56647=CARTESIAN_POINT ( 'NONE',  ( 5.000000000000000000, -10.37499999726881583, -6.123233995736766282E-16 ) ) ;
#56648=CARTESIAN_POINT ( 'NONE',  ( -3.152548672688508926E-16, -41.56249999863439371, -5.148502694627439702 ) ) ;
#56649=ORIENTED_EDGE ( 'NONE', *, *, #59560, .T. ) ;
#56650=CARTESIAN_POINT ( 'NONE',  ( -6.972266317189433020E-16, 14.74999999999999822, -5.000000000000000000 ) ) ;
#56651=CARTESIAN_POINT ( 'NONE',  ( 4.458734124999998549, 9.020833334698927786, -2.574251347313721627 ) ) ;
#56653=CARTESIAN_POINT ( 'NONE',  ( -5.000000000000000000, -57.99999999999999289, 0.000000000000000000 ) ) ;
#56654=CARTESIAN_POINT ( 'NONE',  ( 1.846868145590735200, -161.5000000013656063, -4.458734125000000326 ) ) ;
#56656=CARTESIAN_POINT ( 'NONE',  ( -4.999999999999998224, -34.91666666666666430, 2.886751345948131764 ) ) ;
#56657=CARTESIAN_POINT ( 'NONE',  ( -2.229367062499996610, -82.14583333196773651, 3.861377020970582219 ) ) ;
#56658=CARTESIAN_POINT ( 'NONE',  ( 3.061616997868383141E-16, -164.7500000000000000, -5.000000000000000000 ) ) ;
#56659=CARTESIAN_POINT ( 'NONE',  ( -4.458734124999999437, -89.31249999863440792, 0.000000000000000000 ) ) ;
#56661=CARTESIAN_POINT ( 'NONE',  ( 4.458734124999999437, 0.9375000013655959696, -5.460374474430324690E-16 ) ) ;
#56662=CARTESIAN_POINT ( 'NONE',  ( -4.458734124999999437, -36.56249999863440792, 0.000000000000000000 ) ) ;
#56663=ADVANCED_FACE ( 'NONE', ( #51218 ), #26127, .T. ) ;
#56664=EDGE_CURVE ( 'NONE', #28553, #10085, #7469, .T. ) ;
#56665=CARTESIAN_POINT ( 'NONE',  ( -5.000000000000000000, 24.04166666939785202, -2.886751345948128211 ) ) ;
#56667=CARTESIAN_POINT ( 'NONE',  ( 2.500000000000002220, -86.66666666666667140, 4.330127018922192761 ) ) ;
#56668=ORIENTED_EDGE ( 'NONE', *, *, #53820, .T. ) ;
#56670=CARTESIAN_POINT ( 'NONE',  ( 2.071067811865645591, -152.1875000000000000, 4.999999999999830358 ) ) ;
#56671=CARTESIAN_POINT ( 'NONE',  ( 4.458734124999999437, -72.06249999863439371, -5.460374474430324690E-16 ) ) ;
#56674=VERTEX_POINT ( 'NONE', #41220 ) ;
#56675=EDGE_CURVE ( 'NONE', #22477, #20545, #56365, .T. ) ;
#56676=CARTESIAN_POINT ( 'NONE',  ( -5.000000000000000888, -150.6875000027312126, -2.071067811865475949 ) ) ;
#56677=CARTESIAN_POINT ( 'NONE',  ( 5.000000000000000888, -3.458333330602147093, 2.886751345948126879 ) ) ;
#56679=EDGE_CURVE ( 'NONE', #43575, #1059, #42142, .T. ) ;
#56680=PLANE ( 'NONE',  #62051 ) ;
#56681=CARTESIAN_POINT ( 'NONE',  ( -2.229367062500000163, 2.520833334698928230, -3.861377020970580443 ) ) ;
#56682=DIRECTION ( 'NONE',  ( -0.000000000000000000, 1.000000000000000000, -0.000000000000000000 ) ) ;
#56683=CARTESIAN_POINT ( 'NONE',  ( 3.152801135295367541, -157.3125000013656063, -3.152801135295367541 ) ) ;
#56687=CARTESIAN_POINT ( 'NONE',  ( 3.061616997868383141E-16, -167.8750000027312126, -5.000000000000000000 ) ) ;
#56691=CARTESIAN_POINT ( 'NONE',  ( 2.500000000000002220, -67.66666666666667140, 4.330127018922192761 ) ) ;
#56696=CARTESIAN_POINT ( 'NONE',  ( 2.229367062499998831, 21.35416666803226349, -3.861377020970580887 ) ) ;
#56698=CARTESIAN_POINT ( 'NONE',  ( 9.457646018065525792E-16, -3.312499998634407916, 5.148502694627439702 ) ) ;
#56701=CARTESIAN_POINT ( 'NONE',  ( 5.000000000000000888, -141.0625000027312410, -2.071067811865475505 ) ) ;
#56705=CARTESIAN_POINT ( 'NONE',  ( 0.000000000000000000, -170.0000000000000000, 5.000000000000000000 ) ) ;
#56707=CARTESIAN_POINT ( 'NONE',  ( 3.152801135295366208, -158.8125000013656063, 3.152801135295367985 ) ) ;
#56709=CARTESIAN_POINT ( 'NONE',  ( 0.000000000000000000, -170.0000000000000000, 0.000000000000000000 ) ) ;
#56711=CARTESIAN_POINT ( 'NONE',  ( -3.152548672688508926E-16, 15.18750000136559386, -5.148502694627439702 ) ) ;
#56717=CARTESIAN_POINT ( 'NONE',  ( 5.000000000000000888, 8.416666666666666075, 2.886751345948126879 ) ) ;
#56718=CARTESIAN_POINT ( 'NONE',  ( -4.458734124999997661, -56.22916666530107221, 2.574251347313722516 ) ) ;
#56720=DIRECTION ( 'NONE',  ( -0.000000000000000000, 1.000000000000000000, -0.000000000000000000 ) ) ;
#56726=CARTESIAN_POINT ( 'NONE',  ( 5.000000000000000888, -40.58333333333333570, 2.886751345948126879 ) ) ;
#56727=DIRECTION ( 'NONE',  ( -0.000000000000000000, 1.000000000000000000, -0.000000000000000000 ) ) ;
#56728=CARTESIAN_POINT ( 'NONE',  ( -6.972266317189433020E-16, 14.74999999999999822, -5.000000000000000000 ) ) ;
#56730=CARTESIAN_POINT ( 'NONE',  ( 0.000000000000000000, -170.0000000000000000, 0.000000000000000000 ) ) ;
#56731=CARTESIAN_POINT ( 'NONE',  ( 4.458734124999998549, -65.72916666530106511, -2.574251347313721627 ) ) ;
#56732=CARTESIAN_POINT ( 'NONE',  ( -1.846868145590734756, -149.3750000013656347, -4.458734125000000326 ) ) ;
#56733=CARTESIAN_POINT ( 'NONE',  ( -4.458734124999999437, -73.31249999863439371, 0.000000000000000000 ) ) ;
#56735=CARTESIAN_POINT ( 'NONE',  ( 9.457646018065525792E-16, -20.31249999863440081, 5.148502694627439702 ) ) ;
#56736=CARTESIAN_POINT ( 'NONE',  ( -4.999999999999999112, -62.79166666393546592, 2.886751345948131764 ) ) ;
#56738=ORIENTED_EDGE ( 'NONE', *, *, #41773, .T. ) ;
#56740=EDGE_LOOP ( 'NONE', ( #60472, #61713, #44931, #57718 ) ) ;
#56742=CARTESIAN_POINT ( 'NONE',  ( 5.000000000000000888, -21.45833333060214798, 2.886751345948126879 ) ) ;
#56747=CARTESIAN_POINT ( 'NONE',  ( -1.339745962155613812, -75.08034179853029855, -5.000000000000000000 ) ) ;
#56748=CARTESIAN_POINT ( 'NONE',  ( -4.458734124999998549, -51.47916666530106511, 2.574251347313722516 ) ) ;
#56749=ORIENTED_EDGE ( 'NONE', *, *, #48630, .T. ) ;
#56750=CARTESIAN_POINT ( 'NONE',  ( -5.000000000000000000, -90.43749999863440792, 0.000000000000000000 ) ) ;
#56752=EDGE_CURVE ( 'NONE', #14934, #49037, #27078, .T. ) ;
#56753=CARTESIAN_POINT ( 'NONE',  ( -4.458734124999999437, 19.60416666803225993, -2.574251347313719407 ) ) ;
#56756=CARTESIAN_POINT ( 'NONE',  ( -3.152801135295367985, -168.8125000013656063, 3.152801135295367096 ) ) ;
#56757=ORIENTED_EDGE ( 'NONE', *, *, #5906, .F. ) ;
#56758=EDGE_CURVE ( 'NONE', #36444, #43336, #31815, .T. ) ;
#56762=EDGE_CURVE ( 'NONE', #38362, #24136, #42885, .T. ) ;
#56763=CARTESIAN_POINT ( 'NONE',  ( 2.071067811865517694, -139.9375000027311557, -4.999999999999958256 ) ) ;
#56769=( BOUNDED_CURVE ( )  B_SPLINE_CURVE ( 2, ( #47623, #31571, #22883, #41523, #12895, #36722, #3579, #22571, #41207 ),
 .UNSPECIFIED., .F., .F. ) 
 B_SPLINE_CURVE_WITH_KNOTS ( ( 3, 2, 2, 2, 3 ),
 ( 0.9520833333333332815, 0.9527777777777777235, 0.9541666666666667185, 0.9555555555555556024, 0.9562500000000000444 ),
 .UNSPECIFIED. ) 
 CURVE ( )  GEOMETRIC_REPRESENTATION_ITEM ( )  RATIONAL_B_SPLINE_CURVE ( ( 0.9330127018922194093, 0.9330127018922194093, 1.000000000000000000, 0.8660254037844387076, 1.000000000000000000, 0.8660254037844387076, 1.000000000000000000, 0.9330127018922194093, 0.9330127018922194093 ) ) 
 REPRESENTATION_ITEM ( '' )  );
#56774=ORIENTED_EDGE ( 'NONE', *, *, #7951, .F. ) ;
#56775=CARTESIAN_POINT ( 'NONE',  ( -5.000000000000000000, -4.958333330602148870, -2.886751345948128211 ) ) ;
#56777=CARTESIAN_POINT ( 'NONE',  ( 5.000000000000000000, -153.1875000027312410, 2.071067811865478614 ) ) ;
#56778=ORIENTED_EDGE ( 'NONE', *, *, #2870, .T. ) ;
#56783=CARTESIAN_POINT ( 'NONE',  ( -3.535533905932737309, -145.6250000000000000, -3.535533905932738197 ) ) ;
#56787=CARTESIAN_POINT ( 'NONE',  ( 2.229367062499998831, -25.64583333196773651, -3.861377020970580887 ) ) ;
#56788=DIRECTION ( 'NONE',  ( -0.000000000000000000, 1.000000000000000000, -0.000000000000000000 ) ) ;
#56789=CARTESIAN_POINT ( 'NONE',  ( 1.975475456537005874E-15, 18.37500000273118062, 5.000000000000000000 ) ) ;
#56791=CARTESIAN_POINT ( 'NONE',  ( -1.846868145590734756, -149.1250000013656063, -4.458734125000000326 ) ) ;
#56793=CARTESIAN_POINT ( 'NONE',  ( -9.184850993605147944E-16, -150.2500000000000284, 5.000000000000000000 ) ) ;
#56794=CARTESIAN_POINT ( 'NONE',  ( -3.152548672688508926E-16, -50.81249999863440792, -5.148502694627439702 ) ) ;
#56795=CARTESIAN_POINT ( 'NONE',  ( 5.000000000000000888, -58.45833333060214443, 2.886751345948126879 ) ) ;
#56797=CARTESIAN_POINT ( 'NONE',  ( -5.000000000000000000, 24.91666666666666430, -2.886751345948128211 ) ) ;
#56799=CARTESIAN_POINT ( 'NONE',  ( 2.229367062499998831, -1.645833331967737401, -3.861377020970580887 ) ) ;
#56801=CARTESIAN_POINT ( 'NONE',  ( 3.535533905932736864, -141.1250000000000000, 3.535533905932738641 ) ) ;
#56802=CARTESIAN_POINT ( 'NONE',  ( 5.000000000000000000, -7.500000000000000000, -6.123233995736766282E-16 ) ) ;
#56803=CARTESIAN_POINT ( 'NONE',  ( -2.229367062500000163, 12.27083333469892601, -3.861377020970580443 ) ) ;
#56805=ORIENTED_EDGE ( 'NONE', *, *, #35657, .F. ) ;
#56807=ORIENTED_EDGE ( 'NONE', *, *, #44054, .T. ) ;
#56808=CARTESIAN_POINT ( 'NONE',  ( 5.000000000000000000, -168.1875000027311842, 2.071067811865478614 ) ) ;
#56809=CARTESIAN_POINT ( 'NONE',  ( 4.458734124999998549, -47.72916666530106511, -2.574251347313721627 ) ) ;
#56810=CARTESIAN_POINT ( 'NONE',  ( 2.730187237215162345E-16, -163.4375000013655779, -4.458734124999999437 ) ) ;
#56811=CARTESIAN_POINT ( 'NONE',  ( -3.535250795749689387E-16, -44.12499999726880873, -5.773502691896257311 ) ) ;
#56812=ORIENTED_EDGE ( 'NONE', *, *, #54784, .F. ) ;
#56813=CARTESIAN_POINT ( 'NONE',  ( 2.229367062500001939, -21.97916666530107221, 3.861377020970579999 ) ) ;
#56816=CARTESIAN_POINT ( 'NONE',  ( -4.458734125000000326, -164.0000000013656063, -1.846868145590735644 ) ) ;
#56820=CARTESIAN_POINT ( 'NONE',  ( -4.458734124999998549, -39.47916666530107932, 2.574251347313722516 ) ) ;
#56821=FACE_OUTER_BOUND ( 'NONE', #58620, .T. ) ;
#56826=CARTESIAN_POINT ( 'NONE',  ( 1.339745962155609149, 24.41965820146970856, 5.000000000000003553 ) ) ;
#56828=CARTESIAN_POINT ( 'NONE',  ( -1.339745962155613812, -23.08034179853029144, -5.000000000000000000 ) ) ;
#56830=CARTESIAN_POINT ( 'NONE',  ( -2.229367062499996610, -78.39583333196773651, 3.861377020970582219 ) ) ;
#56834=DIRECTION ( 'NONE',  ( -0.000000000000000000, 1.000000000000000000, -0.000000000000000000 ) ) ;
#56837=CARTESIAN_POINT ( 'NONE',  ( -5.000000000000000000, 20.91666666666666785, -2.886751345948128211 ) ) ;
#56839=CARTESIAN_POINT ( 'NONE',  ( 2.071067811865370256, -158.9375000027311842, -5.000000000000105693 ) ) ;
#56842=CARTESIAN_POINT ( 'NONE',  ( -4.999999999999998224, -72.91666666666667140, 2.886751345948131764 ) ) ;
#56844=CARTESIAN_POINT ( 'NONE',  ( 4.458734125000001214, -81.14583333196773651, 2.574251347313718519 ) ) ;
#56847=ORIENTED_EDGE ( 'NONE', *, *, #52575, .F. ) ;
#56850=CARTESIAN_POINT ( 'NONE',  ( -5.000000000000000000, -164.6250000027311842, -6.123233995736766282E-16 ) ) ;
#56852=CARTESIAN_POINT ( 'NONE',  ( -2.229367062499996610, 12.60416666803226171, 3.861377020970582219 ) ) ;
#56853=DIRECTION ( 'NONE',  ( -0.000000000000000000, 1.000000000000000000, -0.000000000000000000 ) ) ;
#56858=CARTESIAN_POINT ( 'NONE',  ( -5.000000000000000888, -163.4375000000000000, 2.071067811865474617 ) ) ;
#56860=CARTESIAN_POINT ( 'NONE',  ( 2.229367062500001939, -8.979166665301075767, 3.861377020970579999 ) ) ;
#56863=CARTESIAN_POINT ( 'NONE',  ( 2.229367062500001939, -35.22916666530107221, 3.861377020970579999 ) ) ;
#56868=CARTESIAN_POINT ( 'NONE',  ( -8.190561711645485556E-16, -149.9375000013656063, 4.458734124999999437 ) ) ;
#56870=CARTESIAN_POINT ( 'NONE',  ( -3.152548672688508926E-16, 17.43750000136559564, -5.148502694627439702 ) ) ;
#56871=LINE ( 'NONE', #41419, #56448 ) ;
#56872=CARTESIAN_POINT ( 'NONE',  ( -9.184850993605147944E-16, -161.2500000000000000, 5.000000000000000000 ) ) ;
#56873=CARTESIAN_POINT ( 'NONE',  ( -2.229367062499996610, -83.39583333196773651, 3.861377020970582219 ) ) ;
#56876=CARTESIAN_POINT ( 'NONE',  ( -2.500000000000000444, 20.95833333606451987, -4.330127018922193649 ) ) ;
#56878=CARTESIAN_POINT ( 'NONE',  ( 1.339745962155612702, -79.29465819873851729, -5.000000000000000000 ) ) ;
#56880=CARTESIAN_POINT ( 'NONE',  ( 1.339745962155612702, -52.29465819873851729, -5.000000000000000000 ) ) ;
#56881=CARTESIAN_POINT ( 'NONE',  ( 1.060575238724906964E-15, -30.75000000000000000, 5.773502691896257311 ) ) ;
#56882=CARTESIAN_POINT ( 'NONE',  ( 4.458734124999998549, -34.72916666530107221, -2.574251347313721627 ) ) ;
#56884=CARTESIAN_POINT ( 'NONE',  ( -5.000000000000000000, -26.95833333060214798, -2.886751345948128211 ) ) ;
#56885=CARTESIAN_POINT ( 'NONE',  ( 9.457646018065525792E-16, -58.06249999863440081, 5.148502694627439702 ) ) ;
#56887=CARTESIAN_POINT ( 'NONE',  ( 5.000000000000000000, -62.37499999726880873, -6.123233995736766282E-16 ) ) ;
#56888=CARTESIAN_POINT ( 'NONE',  ( -2.229367062500000163, -8.729166665301073991, -3.861377020970580443 ) ) ;
#56890=CARTESIAN_POINT ( 'NONE',  ( 5.000000000000000888, -72.58333333333334281, 2.886751345948126879 ) ) ;
#56893=CARTESIAN_POINT ( 'NONE',  ( 2.499999999999998668, -79.20833333060213022, -4.330127018922193649 ) ) ;
#56895=VERTEX_POINT ( 'NONE', #55405 ) ;
#56897=CARTESIAN_POINT ( 'NONE',  ( 2.229367062500001939, -14.22916666530107221, 3.861377020970579999 ) ) ;
#56898=CARTESIAN_POINT ( 'NONE',  ( -2.229367062500000163, -58.72916666530106511, -3.861377020970580443 ) ) ;
#56900=CARTESIAN_POINT ( 'NONE',  ( -1.339745962155613812, -24.20534180126147206, -5.000000000000000000 ) ) ;
#56902=CARTESIAN_POINT ( 'NONE',  ( -4.458734125000000326, -141.0000000013656063, -1.846868145590735644 ) ) ;
#56904=CARTESIAN_POINT ( 'NONE',  ( -9.184850993605147944E-16, -158.2500000000000000, 5.000000000000000000 ) ) ;
#56908=CARTESIAN_POINT ( 'NONE',  ( 1.339745962155615144, 18.29465819873851729, 4.999999999999999112 ) ) ;
#56912=CARTESIAN_POINT ( 'NONE',  ( 1.846868145590735200, -146.5000000013656347, -4.458734125000000326 ) ) ;
#56914=DIRECTION ( 'NONE',  ( -0.000000000000000000, 1.000000000000000000, -0.000000000000000000 ) ) ;
#56916=CARTESIAN_POINT ( 'NONE',  ( 9.457646018065525792E-16, -64.31249999863440792, 5.148502694627439702 ) ) ;
#56919=CARTESIAN_POINT ( 'NONE',  ( 3.152801135295366208, -144.5625000013655779, 3.152801135295367985 ) ) ;
#56922=CARTESIAN_POINT ( 'NONE',  ( -5.000000000000000888, -164.6875000027311842, -2.071067811865475949 ) ) ;
#56928=CARTESIAN_POINT ( 'NONE',  ( -4.458734124999997661, 27.52083333469892779, 2.574251347313722516 ) ) ;
#56929=CARTESIAN_POINT ( 'NONE',  ( -4.999999999999998224, -17.79166666393547658, 2.886751345948131764 ) ) ;
#56933=CARTESIAN_POINT ( 'NONE',  ( -1.049326080737009628E-13, -2.750000000000003109, 5.000000000000000000 ) ) ;
#56934=CARTESIAN_POINT ( 'NONE',  ( 4.458734124999999437, 8.187500001365595637, -5.460374474430324690E-16 ) ) ;
#56936=CARTESIAN_POINT ( 'NONE',  ( 2.229367062500001939, -17.22916666530106866, 3.861377020970579999 ) ) ;
#56938=CARTESIAN_POINT ( 'NONE',  ( -4.458734125000000326, -158.0000000013655779, -1.846868145590735644 ) ) ;
#56939=CARTESIAN_POINT ( 'NONE',  ( -5.000000000000000000, 29.04166666939785557, -2.886751345948128211 ) ) ;
#56943=CARTESIAN_POINT ( 'NONE',  ( 2.499999999999998668, 15.66666666666666607, -4.330127018922193649 ) ) ;
#56944=CARTESIAN_POINT ( 'NONE',  ( -2.229367062500000163, -38.47916666530107221, -3.861377020970580443 ) ) ;
#56946=CARTESIAN_POINT ( 'NONE',  ( -3.152548672688508926E-16, -66.81249999863440792, -5.148502694627439702 ) ) ;
#56948=CARTESIAN_POINT ( 'NONE',  ( -2.500000000000000444, -41.16666666666667140, -4.330127018922193649 ) ) ;
#56949=CARTESIAN_POINT ( 'NONE',  ( 2.499999999999998668, -36.20833333060213732, -4.330127018922193649 ) ) ;
#56953=CARTESIAN_POINT ( 'NONE',  ( -3.535250795749689387E-16, -7.249999999999999112, -5.773502691896257311 ) ) ;
#56954=CARTESIAN_POINT ( 'NONE',  ( -4.458734124999998549, -13.22916666530107221, 2.574251347313722516 ) ) ;
#56955=CARTESIAN_POINT ( 'NONE',  ( -2.229367062499996610, -76.14583333196773651, 3.861377020970582219 ) ) ;
#56957=ADVANCED_FACE ( 'NONE', ( #28018 ), #53098, .T. ) ;
#56958=CARTESIAN_POINT ( 'NONE',  ( -2.500000000000000444, -13.04166666393548013, -4.330127018922193649 ) ) ;
#56959=CARTESIAN_POINT ( 'NONE',  ( 2.229367062500001939, -44.97916666530106511, 3.861377020970579999 ) ) ;
#56960=ORIENTED_EDGE ( 'NONE', *, *, #7496, .F. ) ;
#56962=EDGE_CURVE ( 'NONE', #12680, #7140, #33499, .T. ) ;
#56963=CARTESIAN_POINT ( 'NONE',  ( -4.458734124999998549, 4.520833334698926009, 2.574251347313722516 ) ) ;
#56964=VERTEX_POINT ( 'NONE', #33476 ) ;
#56966=CARTESIAN_POINT ( 'NONE',  ( -3.535250795749689387E-16, -53.24999999999999289, -5.773502691896257311 ) ) ;
#56967=CARTESIAN_POINT ( 'NONE',  ( 4.458734125000000326, -158.6250000013655779, -1.846868145590734978 ) ) ;
#56970=CARTESIAN_POINT ( 'NONE',  ( 4.458734124999999437, -79.81249999863440792, -5.460374474430324690E-16 ) ) ;
#56972=CARTESIAN_POINT ( 'NONE',  ( -2.071067811865475061, -166.6875000000000568, -5.000000000000000888 ) ) ;
#56973=CARTESIAN_POINT ( 'NONE',  ( 4.458734125000001214, -84.89583333196773651, 2.574251347313718519 ) ) ;
#56975=CARTESIAN_POINT ( 'NONE',  ( 9.457646018065525792E-16, -2.312499998634407028, 5.148502694627439702 ) ) ;
#56977=CARTESIAN_POINT ( 'NONE',  ( -2.229367062499996610, -42.39583333196773651, 3.861377020970582219 ) ) ;
#56979=CARTESIAN_POINT ( 'NONE',  ( 1.975475456537005874E-15, 16.37500000273118417, 5.000000000000000000 ) ) ;
#56982=CARTESIAN_POINT ( 'NONE',  ( 0.000000000000000000, -170.0000000000000000, 5.000000000000000000 ) ) ;
#56983=CARTESIAN_POINT ( 'NONE',  ( 4.458734124999999437, -71.06249999863439371, -5.460374474430324690E-16 ) ) ;
#56987=CARTESIAN_POINT ( 'NONE',  ( 0.000000000000000000, -170.0000000000000000, 0.000000000000000000 ) ) ;
#56989=EDGE_CURVE ( 'NONE', #21118, #34811, #9633, .T. ) ;
#56992=CARTESIAN_POINT ( 'NONE',  ( -4.458734124999999437, 0.6875000013655957476, 0.000000000000000000 ) ) ;
#56993=CARTESIAN_POINT ( 'NONE',  ( 1.975475456537005874E-15, -30.62499999726881583, 5.000000000000000000 ) ) ;
#56994=CARTESIAN_POINT ( 'NONE',  ( 2.730187237215162345E-16, -156.1875000013655779, -4.458734124999999437 ) ) ;
#56999=CYLINDRICAL_SURFACE ( 'NONE', #58269, 5.000000000000000000 ) ;
#57004=CARTESIAN_POINT ( 'NONE',  ( 1.339745962155612702, -67.29465819873851729, -5.000000000000000000 ) ) ;
#57006=CARTESIAN_POINT ( 'NONE',  ( 1.975475456537005874E-15, -29.62499999726881228, 5.000000000000000000 ) ) ;
#57009=CARTESIAN_POINT ( 'NONE',  ( 4.458734124999999437, 23.18750000136559564, -5.460374474430324690E-16 ) ) ;
#57011=CARTESIAN_POINT ( 'NONE',  ( 4.458734124999999437, -3.062499998634407472, -5.460374474430324690E-16 ) ) ;
#57014=CARTESIAN_POINT ( 'NONE',  ( 3.535533905932736864, -142.2500000027311842, 3.535533905932738641 ) ) ;
#57015=CARTESIAN_POINT ( 'NONE',  ( -2.498395430326213474E-14, 22.25000000000000000, 5.000000000000000000 ) ) ;
#57018=EDGE_CURVE ( 'NONE', #41628, #48755, #58105, .T. ) ;
#57025=CARTESIAN_POINT ( 'NONE',  ( 1.846868145590736310, -155.8750000013655779, 4.458734124999997661 ) ) ;
#57027=( NAMED_UNIT ( * ) SI_UNIT ( $, .STERADIAN. ) SOLID_ANGLE_UNIT ( ) );
#57029=CARTESIAN_POINT ( 'NONE',  ( 9.457646018065525792E-16, 17.68750000136559564, 5.148502694627439702 ) ) ;
#57035=CARTESIAN_POINT ( 'NONE',  ( -2.500000000000000444, 9.833333333333332149, -4.330127018922193649 ) ) ;
#57037=CARTESIAN_POINT ( 'NONE',  ( -4.458734124999999437, -56.31249999863440081, 0.000000000000000000 ) ) ;
#57038=CARTESIAN_POINT ( 'NONE',  ( -5.000000000000000000, -8.083333333333332149, -2.886751345948128211 ) ) ;
#57041=CARTESIAN_POINT ( 'NONE',  ( -4.458734124999999437, -29.31249999863440436, 0.000000000000000000 ) ) ;
#57042=CARTESIAN_POINT ( 'NONE',  ( 3.535533905932736864, -153.2500000027312126, 3.535533905932738641 ) ) ;
#57045=CARTESIAN_POINT ( 'NONE',  ( -5.000000000000000000, -151.6250000027312126, -6.123233995736766282E-16 ) ) ;
#57046=CARTESIAN_POINT ( 'NONE',  ( -5.000000000000000000, -41.99999999999999289, 0.000000000000000000 ) ) ;
#57051=CARTESIAN_POINT ( 'NONE',  ( 4.458734124999999437, -65.81249999863440792, -5.460374474430324690E-16 ) ) ;
#57052=CARTESIAN_POINT ( 'NONE',  ( -1.846868145590734756, -148.3750000013655779, -4.458734125000000326 ) ) ;
#57053=CARTESIAN_POINT ( 'NONE',  ( -2.229367062499996610, -69.14583333196773651, 3.861377020970582219 ) ) ;
#57055=VECTOR ( 'NONE', #55474, 1000.000000000000000 ) ;
#57056=CARTESIAN_POINT ( 'NONE',  ( -4.458734124999999437, -25.64583333196773651, -2.574251347313719407 ) ) ;
#57057=CARTESIAN_POINT ( 'NONE',  ( -2.499999999999996447, -59.70833333060214443, 4.330127018922195425 ) ) ;
#57058=ORIENTED_EDGE ( 'NONE', *, *, #39697, .F. ) ;
#57059=DIRECTION ( 'NONE',  ( 0.000000000000000000, 0.000000000000000000, 1.000000000000000000 ) ) ;
#57060=VERTEX_POINT ( 'NONE', #54370 ) ;
#57062=CARTESIAN_POINT ( 'NONE',  ( 6.123233995736766282E-16, -170.0000000000000000, -5.000000000000000000 ) ) ;
#57063=LINE ( 'NONE', #22324, #26632 ) ;
#57066=CYLINDRICAL_SURFACE ( 'NONE', #28275, 5.000000000000000000 ) ;
#57067=CARTESIAN_POINT ( 'NONE',  ( 2.229367062499998831, -55.89583333196773651, -3.861377020970580887 ) ) ;
#57068=ORIENTED_EDGE ( 'NONE', *, *, #4704, .F. ) ;
#57071=CARTESIAN_POINT ( 'NONE',  ( -2.229367062499996610, 19.85416666803225993, 3.861377020970582219 ) ) ;
#57074=CARTESIAN_POINT ( 'NONE',  ( -4.458734124999999437, -168.9375000013656063, -5.460374474430324690E-16 ) ) ;
#57075=EDGE_LOOP ( 'NONE', ( #35916, #59814, #45863, #40398 ) ) ;
#57077=CARTESIAN_POINT ( 'NONE',  ( -1.339745962155613812, -86.08034179853028434, -5.000000000000000000 ) ) ;
#57079=CARTESIAN_POINT ( 'NONE',  ( 1.975475456537005874E-15, -78.74999999999998579, 5.000000000000000000 ) ) ;
#57087=VERTEX_POINT ( 'NONE', #39552 ) ;
#57090=CARTESIAN_POINT ( 'NONE',  ( 5.000000000000000888, -154.0625000027312126, -2.071067811865475505 ) ) ;
#57096=( BOUNDED_CURVE ( )  B_SPLINE_CURVE ( 2, ( #30638, #21318, #30958, #55092, #6208, #15208, #5244, #59277, #40605 ),
 .UNSPECIFIED., .F., .F. ) 
 B_SPLINE_CURVE_WITH_KNOTS ( ( 3, 2, 2, 2, 3 ),
 ( 0.4895833333333333148, 0.4902777777777777568, 0.4916666666666666408, 0.4930555555555555802, 0.4937500000000000222 ),
 .UNSPECIFIED. ) 
 CURVE ( )  GEOMETRIC_REPRESENTATION_ITEM ( )  RATIONAL_B_SPLINE_CURVE ( ( 0.9330127018922194093, 0.9330127018922194093, 1.000000000000000000, 0.8660254037844387076, 1.000000000000000000, 0.8660254037844387076, 1.000000000000000000, 0.9330127018922194093, 0.9330127018922194093 ) ) 
 REPRESENTATION_ITEM ( '' )  );
#57097=CARTESIAN_POINT ( 'NONE',  ( 5.000000000000000888, -146.9375000000000284, -2.071067811865475505 ) ) ;
#57099=EDGE_CURVE ( 'NONE', #38204, #47541, #7600, .T. ) ;
#57102=LINE ( 'NONE', #52891, #22336 ) ;
#57103=CARTESIAN_POINT ( 'NONE',  ( 2.229367062499998831, -26.64583333196774007, -3.861377020970580887 ) ) ;
#57104=ADVANCED_FACE ( 'NONE', ( #19626 ), #9653, .T. ) ;
#57108=CARTESIAN_POINT ( 'NONE',  ( -8.190561711645485556E-16, -148.6875000013656063, 4.458734124999999437 ) ) ;
#57109=ORIENTED_EDGE ( 'NONE', *, *, #23403, .T. ) ;
#57111=CARTESIAN_POINT ( 'NONE',  ( 4.458734124999999437, -53.06249999863440792, -5.460374474430324690E-16 ) ) ;
#57112=CARTESIAN_POINT ( 'NONE',  ( 5.000000000000000888, -2.583333333333333481, 2.886751345948126879 ) ) ;
#57114=CARTESIAN_POINT ( 'NONE',  ( 2.500000000000002220, 23.33333333333333215, 4.330127018922192761 ) ) ;
#57116=EDGE_CURVE ( 'NONE', #34696, #21297, #39236, .T. ) ;
#57118=CARTESIAN_POINT ( 'NONE',  ( 4.458734124999998549, -2.729166665301069550, -2.574251347313721627 ) ) ;
#57119=CARTESIAN_POINT ( 'NONE',  ( -2.499999999999996447, -10.83333333333333393, 4.330127018922195425 ) ) ;
#57120=CARTESIAN_POINT ( 'NONE',  ( 5.000000000000000000, -141.0625000000000000, 2.071067811865478614 ) ) ;
#57122=CARTESIAN_POINT ( 'NONE',  ( -2.229367062499996610, 10.60416666803225993, 3.861377020970582219 ) ) ;
#57124=VERTEX_POINT ( 'NONE', #25089 ) ;
#57127=CARTESIAN_POINT ( 'NONE',  ( -6.972266317189433020E-16, -85.25000000000000000, -5.000000000000000000 ) ) ;
#57128=CARTESIAN_POINT ( 'NONE',  ( -4.458734124999998549, -49.22916666530106511, 2.574251347313722516 ) ) ;
#57130=CARTESIAN_POINT ( 'NONE',  ( -3.152801135295367096, -158.3125000013656063, -3.152801135295367541 ) ) ;
#57132=CARTESIAN_POINT ( 'NONE',  ( 1.060575238724906964E-15, -46.62499999726880873, 5.773502691896257311 ) ) ;
#57134=CARTESIAN_POINT ( 'NONE',  ( -3.152548672688508926E-16, -21.56249999863440081, -5.148502694627439702 ) ) ;
#57137=CARTESIAN_POINT ( 'NONE',  ( -1.846868145590734756, -161.1250000013656063, -4.458734125000000326 ) ) ;
#57139=CARTESIAN_POINT ( 'NONE',  ( 4.458734125000001214, -37.14583333196773651, 2.574251347313718519 ) ) ;
#57143=AXIS2_PLACEMENT_3D ( 'NONE', #32058, #3124, #37522 ) ;
#57147=ORIENTED_EDGE ( 'NONE', *, *, #47211, .F. ) ;
#57150=CARTESIAN_POINT ( 'NONE',  ( -2.229367062500000163, -87.72916666530107932, -3.861377020970580443 ) ) ;
#57153=CARTESIAN_POINT ( 'NONE',  ( -2.499999999999996447, -6.833333333333330373, 4.330127018922195425 ) ) ;
#57154=( BOUNDED_CURVE ( )  B_SPLINE_CURVE ( 2, ( #9680, #49245, #1342, #49873, #4865, #35099, #24485, #14504, #10637 ),
 .UNSPECIFIED., .F., .F. ) 
 B_SPLINE_CURVE_WITH_KNOTS ( ( 3, 2, 2, 2, 3 ),
 ( 0.6979166666666666297, 0.6986111111111110716, 0.6999999999999999556, 0.7013888888888888395, 0.7020833333333332815 ),
 .UNSPECIFIED. ) 
 CURVE ( )  GEOMETRIC_REPRESENTATION_ITEM ( )  RATIONAL_B_SPLINE_CURVE ( ( 0.9330127018922194093, 0.9330127018922194093, 1.000000000000000000, 0.8660254037844387076, 1.000000000000000000, 0.8660254037844387076, 1.000000000000000000, 0.9330127018922194093, 0.9330127018922194093 ) ) 
 REPRESENTATION_ITEM ( '' )  );
#57155=CARTESIAN_POINT ( 'NONE',  ( -1.339745962155613812, -47.08034179853029144, -5.000000000000000000 ) ) ;
#57160=CARTESIAN_POINT ( 'NONE',  ( 0.000000000000000000, -170.0000000000000000, 5.000000000000000000 ) ) ;
#57164=DIRECTION ( 'NONE',  ( -0.000000000000000000, 1.000000000000000000, -0.000000000000000000 ) ) ;
#57165=CARTESIAN_POINT ( 'NONE',  ( 9.457646018065525792E-16, -85.31249999863439371, 5.148502694627439702 ) ) ;
#57168=ORIENTED_EDGE ( 'NONE', *, *, #30730, .F. ) ;
#57169=FACE_OUTER_BOUND ( 'NONE', #8410, .T. ) ;
#57171=CARTESIAN_POINT ( 'NONE',  ( -5.000000000000000888, -164.5625000027312126, 2.071067811865474617 ) ) ;
#57173=CARTESIAN_POINT ( 'NONE',  ( -2.229367062500000163, 14.27083333469892601, -3.861377020970580443 ) ) ;
#57180=CARTESIAN_POINT ( 'NONE',  ( 4.458734124999998549, -9.729166665301068662, -2.574251347313721627 ) ) ;
#57183=CARTESIAN_POINT ( 'NONE',  ( -4.458734124999997661, -35.47916666530107221, 2.574251347313722516 ) ) ;
#57184=AXIS2_PLACEMENT_3D ( 'NONE', #41338, #36521, #56151 ) ;
#57189=AXIS2_PLACEMENT_3D ( 'NONE', #13090, #51707, #12770 ) ;
#57190=CARTESIAN_POINT ( 'NONE',  ( 4.458734124999998549, 13.27083333469892779, -2.574251347313721627 ) ) ;
#57191=CARTESIAN_POINT ( 'NONE',  ( -5.000000000000000000, -81.95833333060213022, -2.886751345948128211 ) ) ;
#57193=CARTESIAN_POINT ( 'NONE',  ( 4.458734124999998549, -83.97916666530106511, -2.574251347313721627 ) ) ;
#57196=CARTESIAN_POINT ( 'NONE',  ( -2.499999999999996447, 21.29166666939785202, 4.330127018922195425 ) ) ;
#57198=CARTESIAN_POINT ( 'NONE',  ( 3.061616997868383141E-16, -146.8750000027312126, -5.000000000000000000 ) ) ;
#57199=DIRECTION ( 'NONE',  ( 0.000000000000000000, 0.000000000000000000, 1.000000000000000000 ) ) ;
#57201=DIRECTION ( 'NONE',  ( -0.000000000000000000, 1.000000000000000000, -0.000000000000000000 ) ) ;
#57202=CARTESIAN_POINT ( 'NONE',  ( -5.000000000000000000, -28.99999999999999645, 0.000000000000000000 ) ) ;
#57203=CARTESIAN_POINT ( 'NONE',  ( -4.458734124999999437, -34.31249999863440792, 0.000000000000000000 ) ) ;
#57205=CARTESIAN_POINT ( 'NONE',  ( 5.000000000000000000, -29.29166666393547658, -2.886751345948129988 ) ) ;
#57206=CARTESIAN_POINT ( 'NONE',  ( -3.152548672688508926E-16, -58.56249999863440081, -5.148502694627439702 ) ) ;
#57209=CARTESIAN_POINT ( 'NONE',  ( -4.458734124999998549, -11.47916666530107044, 2.574251347313722516 ) ) ;
#57210=ORIENTED_EDGE ( 'NONE', *, *, #35281, .F. ) ;
#57211=CARTESIAN_POINT ( 'NONE',  ( 5.000000000000000888, -76.58333333333332860, 2.886751345948126879 ) ) ;
#57214=CARTESIAN_POINT ( 'NONE',  ( 5.000000000000000000, -74.29166666393547303, -2.886751345948129988 ) ) ;
#57216=ORIENTED_EDGE ( 'NONE', *, *, #41328, .F. ) ;
#57218=CARTESIAN_POINT ( 'NONE',  ( -4.458734124999999437, -21.64583333196774362, -2.574251347313719407 ) ) ;
#57219=CARTESIAN_POINT ( 'NONE',  ( 4.458734124999998549, -54.97916666530107221, -2.574251347313721627 ) ) ;
#57222=CARTESIAN_POINT ( 'NONE',  ( -1.846868145590734756, -141.1250000013655779, -4.458734125000000326 ) ) ;
#57224=CARTESIAN_POINT ( 'NONE',  ( 6.123233995736766282E-16, -170.0000000000000000, -5.000000000000000000 ) ) ;
#57233=CARTESIAN_POINT ( 'NONE',  ( 3.152801135295367541, -148.5625000013655779, -3.152801135295367541 ) ) ;
#57238=CARTESIAN_POINT ( 'NONE',  ( -2.229367062499996610, -65.39583333196773651, 3.861377020970582219 ) ) ;
#57241=CARTESIAN_POINT ( 'NONE',  ( -8.190561711645485556E-16, -141.6875000013656063, 4.458734124999999437 ) ) ;
#57244=CARTESIAN_POINT ( 'NONE',  ( 1.975475456537005874E-15, -49.62499999726880873, 5.000000000000000000 ) ) ;
#57245=CARTESIAN_POINT ( 'NONE',  ( 1.975475456537005874E-15, -6.624999997268813168, 5.000000000000000000 ) ) ;
#57250=CARTESIAN_POINT ( 'NONE',  ( 2.229367062499998831, 26.10416666803225993, -3.861377020970580887 ) ) ;
#57255=LINE ( 'NONE', #48522, #20211 ) ;
#57256=CARTESIAN_POINT ( 'NONE',  ( -4.458734124999999437, 8.687500001365595637, 0.000000000000000000 ) ) ;
#57258=CARTESIAN_POINT ( 'NONE',  ( 4.458734124999998549, -16.97916666530107577, -2.574251347313721627 ) ) ;
#57260=CARTESIAN_POINT ( 'NONE',  ( -1.846868145590734756, -160.1250000013655779, -4.458734125000000326 ) ) ;
#57261=CARTESIAN_POINT ( 'NONE',  ( 2.500000000000002220, 15.45833333606451987, 4.330127018922192761 ) ) ;
#57264=FACE_OUTER_BOUND ( 'NONE', #42175, .T. ) ;
#57265=CARTESIAN_POINT ( 'NONE',  ( 4.458734125000000326, -40.89583333196773651, 2.574251347313718519 ) ) ;
#57268=CARTESIAN_POINT ( 'NONE',  ( -2.229367062499996610, -67.39583333196773651, 3.861377020970582219 ) ) ;
#57270=CARTESIAN_POINT ( 'NONE',  ( 1.975475456537005874E-15, -57.62499999726880873, 5.000000000000000000 ) ) ;
#57273=CARTESIAN_POINT ( 'NONE',  ( -4.999999999999998224, 15.20833333606451987, 2.886751345948131764 ) ) ;
#57274=VECTOR ( 'NONE', #20913, 1000.000000000000000 ) ;
#57275=CARTESIAN_POINT ( 'NONE',  ( 5.000000000000000888, -13.58333333333333570, 2.886751345948126879 ) ) ;
#57276=CARTESIAN_POINT ( 'NONE',  ( 4.458734125000001214, -14.89583333196773474, 2.574251347313718519 ) ) ;
#57278=CARTESIAN_POINT ( 'NONE',  ( -2.229367062500000163, -75.47916666530106511, -3.861377020970580443 ) ) ;
#57279=AXIS2_PLACEMENT_3D ( 'NONE', #52676, #42696, #8609 ) ;
#57280=( BOUNDED_CURVE ( )  B_SPLINE_CURVE ( 2, ( #42334, #24289, #9801, #19138, #4358, #39389, #49042, #63223, #181 ),
 .UNSPECIFIED., .F., .F. ) 
 B_SPLINE_CURVE_WITH_KNOTS ( ( 3, 2, 2, 2, 3 ),
 ( 0.6770833333333333703, 0.6777777777777778123, 0.6791666666666666963, 0.6805555555555555802, 0.6812500000000000222 ),
 .UNSPECIFIED. ) 
 CURVE ( )  GEOMETRIC_REPRESENTATION_ITEM ( )  RATIONAL_B_SPLINE_CURVE ( ( 0.9330127018922194093, 0.9330127018922194093, 1.000000000000000000, 0.8660254037844387076, 1.000000000000000000, 0.8660254037844387076, 1.000000000000000000, 0.9330127018922194093, 0.9330127018922194093 ) ) 
 REPRESENTATION_ITEM ( '' )  );
#57282=CARTESIAN_POINT ( 'NONE',  ( -2.499999999999996447, -10.70833333060214621, 4.330127018922195425 ) ) ;
#57283=CARTESIAN_POINT ( 'NONE',  ( -4.458734124999999437, -45.39583333196773651, -2.574251347313719407 ) ) ;
#57285=CARTESIAN_POINT ( 'NONE',  ( 5.000000000000000888, -143.9375000000000000, -2.071067811865475505 ) ) ;
#57286=CARTESIAN_POINT ( 'NONE',  ( -4.458734124999999437, 9.437500001365593860, 0.000000000000000000 ) ) ;
#57287=ORIENTED_EDGE ( 'NONE', *, *, #9862, .T. ) ;
#57288=CARTESIAN_POINT ( 'NONE',  ( -6.972266317189433020E-16, -81.24999999999998579, -5.000000000000000000 ) ) ;
#57289=CARTESIAN_POINT ( 'NONE',  ( -3.535250795749689387E-16, -59.25000000000000000, -5.773502691896257311 ) ) ;
#57290=CARTESIAN_POINT ( 'NONE',  ( 1.846868145590736310, -160.8750000013655779, 4.458734124999999437 ) ) ;
#57292=CARTESIAN_POINT ( 'NONE',  ( 5.000000000000000000, -14.41666666666666785, -2.886751345948130876 ) ) ;
#57293=CARTESIAN_POINT ( 'NONE',  ( -4.458734124999998549, -81.22916666530106511, 2.574251347313722516 ) ) ;
#57294=CARTESIAN_POINT ( 'NONE',  ( -2.071067811865478170, -166.3125000000000000, 5.000000000000000000 ) ) ;
#57295=CARTESIAN_POINT ( 'NONE',  ( -4.458734124999999437, -90.31249999863440792, 0.000000000000000000 ) ) ;
#57297=CARTESIAN_POINT ( 'NONE',  ( -3.152548672688508926E-16, -5.812499998634404363, -5.148502694627439702 ) ) ;
#57298=CARTESIAN_POINT ( 'NONE',  ( 4.458734125000001214, -43.14583333196773651, 2.574251347313718519 ) ) ;
#57305=CARTESIAN_POINT ( 'NONE',  ( -2.229367062499996610, -67.39583333196773651, 3.861377020970582219 ) ) ;
#57306=EDGE_CURVE ( 'NONE', #45731, #14852, #36655, .T. ) ;
#57307=CARTESIAN_POINT ( 'NONE',  ( 4.458734124999997661, -146.7500000013656063, 1.846868145590737864 ) ) ;
#57309=CARTESIAN_POINT ( 'NONE',  ( 5.000000000000000000, -5.416666666666666963, -2.886751345948130876 ) ) ;
#57310=CARTESIAN_POINT ( 'NONE',  ( -2.071067811865391128, -146.8125000027312126, -5.000000000000086153 ) ) ;
#57312=CARTESIAN_POINT ( 'NONE',  ( -4.458734124999999437, 3.687500001365594748, 0.000000000000000000 ) ) ;
#57313=CARTESIAN_POINT ( 'NONE',  ( -1.846868145590734756, -155.1250000013656063, -4.458734124999999437 ) ) ;
#57314=VECTOR ( 'NONE', #43831, 1000.000000000000000 ) ;
#57316=ORIENTED_EDGE ( 'NONE', *, *, #31089, .T. ) ;
#57322=CYLINDRICAL_SURFACE ( 'NONE', #4631, 5.000000000000000000 ) ;
#57323=CARTESIAN_POINT ( 'NONE',  ( 5.000000000000000888, -23.45833333060214443, 2.886751345948126879 ) ) ;
#57329=CARTESIAN_POINT ( 'NONE',  ( -2.229367062500000163, 21.52083333469892779, -3.861377020970580443 ) ) ;
#57331=CARTESIAN_POINT ( 'NONE',  ( -3.152548672688508926E-16, -5.812499998634404363, -5.148502694627439702 ) ) ;
#57334=CARTESIAN_POINT ( 'NONE',  ( -3.535533905932738641, -141.5000000027311842, 3.535533905932737309 ) ) ;
#57335=CARTESIAN_POINT ( 'NONE',  ( 0.000000000000000000, -170.0000000000000000, 0.000000000000000000 ) ) ;
#57342=CARTESIAN_POINT ( 'NONE',  ( 4.458734124999999437, -155.6875000013655779, 0.000000000000000000 ) ) ;
#57345=CARTESIAN_POINT ( 'NONE',  ( 4.458734124999999437, 16.93750000136559564, -5.460374474430324690E-16 ) ) ;
#57346=ORIENTED_EDGE ( 'NONE', *, *, #8811, .F. ) ;
#57352=CARTESIAN_POINT ( 'NONE',  ( -2.500000000000000444, 1.833333333333332593, -4.330127018922193649 ) ) ;
#57353=CARTESIAN_POINT ( 'NONE',  ( 9.457646018065525792E-16, -63.06249999863440792, 5.148502694627439702 ) ) ;
#57355=CARTESIAN_POINT ( 'NONE',  ( -4.458734124999999437, -28.31249999863440081, 0.000000000000000000 ) ) ;
#57356=CARTESIAN_POINT ( 'NONE',  ( -2.499999999999996447, 26.29166666939785202, 4.330127018922195425 ) ) ;
#57357=CARTESIAN_POINT ( 'NONE',  ( 2.500000000000002220, -38.66666666666667140, 4.330127018922192761 ) ) ;
#57358=CARTESIAN_POINT ( 'NONE',  ( 2.499999999999998668, -70.20833333060214443, -4.330127018922193649 ) ) ;
#57359=CARTESIAN_POINT ( 'NONE',  ( 1.975475456537005874E-15, -14.74999999999999822, 5.000000000000000000 ) ) ;
#57361=CARTESIAN_POINT ( 'NONE',  ( -2.499999999999996447, 13.16666666666666607, 4.330127018922195425 ) ) ;
#57362=CARTESIAN_POINT ( 'NONE',  ( -2.229367062500000163, -64.47916666530106511, -3.861377020970580443 ) ) ;
#57363=CARTESIAN_POINT ( 'NONE',  ( 4.458734124999999437, -149.7500000013656063, 1.846868145590737864 ) ) ;
#57364=CARTESIAN_POINT ( 'NONE',  ( 2.229367062500001939, -75.97916666530106511, 3.861377020970579999 ) ) ;
#57365=AXIS2_PLACEMENT_3D ( 'NONE', #27968, #18323, #62401 ) ;
#57367=CARTESIAN_POINT ( 'NONE',  ( -2.229367062500000163, -26.72916666530106866, -3.861377020970580443 ) ) ;
#57368=CARTESIAN_POINT ( 'NONE',  ( 5.000000000000000000, -68.29166666393547303, -2.886751345948129988 ) ) ;
#57370=CARTESIAN_POINT ( 'NONE',  ( -6.972266317189433020E-16, -1.250000000000000000, -5.000000000000000000 ) ) ;
#57375=VERTEX_POINT ( 'NONE', #56284 ) ;
#57376=( BOUNDED_CURVE ( )  B_SPLINE_CURVE ( 2, ( #7352, #31451, #6080, #41103, #51092, #36606, #1899, #17303, #55286 ),
 .UNSPECIFIED., .F., .F. ) 
 B_SPLINE_CURVE_WITH_KNOTS ( ( 3, 2, 2, 2, 3 ),
 ( 0.4562499999999999889, 0.4569444444444444309, 0.4583333333333333148, 0.4597222222222221988, 0.4604166666666666963 ),
 .UNSPECIFIED. ) 
 CURVE ( )  GEOMETRIC_REPRESENTATION_ITEM ( )  RATIONAL_B_SPLINE_CURVE ( ( 0.9330127018922194093, 0.9330127018922194093, 1.000000000000000000, 0.8660254037844387076, 1.000000000000000000, 0.8660254037844387076, 1.000000000000000000, 0.9330127018922167448, 0.9330127018922194093 ) ) 
 REPRESENTATION_ITEM ( '' )  );
#57377=CARTESIAN_POINT ( 'NONE',  ( 4.458734124999998549, 28.02083333469892779, -2.574251347313721627 ) ) ;
#57378=CARTESIAN_POINT ( 'NONE',  ( -2.500000000000000444, -83.16666666666667140, -4.330127018922193649 ) ) ;
#57379=CARTESIAN_POINT ( 'NONE',  ( -2.229367062499996610, -54.39583333196773651, 3.861377020970582219 ) ) ;
#57382=VECTOR ( 'NONE', #4369, 1000.000000000000000 ) ;
#57385=CARTESIAN_POINT ( 'NONE',  ( 4.458734125000001214, 18.10416666803225638, 2.574251347313718519 ) ) ;
#57387=CARTESIAN_POINT ( 'NONE',  ( 1.975475456537005874E-15, -1.749999999999999334, 5.000000000000000000 ) ) ;
#57388=CARTESIAN_POINT ( 'NONE',  ( -3.152801135295367985, -167.8125000013656063, 3.152801135295367096 ) ) ;
#57391=EDGE_CURVE ( 'NONE', #29720, #19705, #55313, .T. ) ;
#57392=CARTESIAN_POINT ( 'NONE',  ( 0.000000000000000000, 30.00000000000000000, 0.000000000000000000 ) ) ;
#57394=CARTESIAN_POINT ( 'NONE',  ( 5.000000000000000000, -140.1250000027312126, 0.000000000000000000 ) ) ;
#57398=CARTESIAN_POINT ( 'NONE',  ( 1.339745962155590275, 4.294658198738519062, 5.000000000000013323 ) ) ;
#57402=FACE_OUTER_BOUND ( 'NONE', #47084, .T. ) ;
#57406=CARTESIAN_POINT ( 'NONE',  ( 5.275681513340003914E-14, 11.74999999999999645, -5.000000000000000000 ) ) ;
#57408=CARTESIAN_POINT ( 'NONE',  ( -5.000000000000000888, -152.6875000027311842, -2.071067811865475949 ) ) ;
#57414=CARTESIAN_POINT ( 'NONE',  ( -9.184850993605147944E-16, -146.2500000000000284, 5.000000000000000000 ) ) ;
#57417=CARTESIAN_POINT ( 'NONE',  ( 1.846868145590736310, -167.8750000013656063, 4.458734124999997661 ) ) ;
#57418=CARTESIAN_POINT ( 'NONE',  ( 4.458734124999998549, -27.72916666530107221, -2.574251347313721627 ) ) ;
#57419=FACE_OUTER_BOUND ( 'NONE', #55443, .T. ) ;
#57422=CARTESIAN_POINT ( 'NONE',  ( 1.846868145590736310, -148.6250000013655779, 4.458734124999999437 ) ) ;
#57424=CARTESIAN_POINT ( 'NONE',  ( -6.972266317189433020E-16, -0.2500000000000001665, -5.000000000000000000 ) ) ;
#57425=CARTESIAN_POINT ( 'NONE',  ( 9.457646018065525792E-16, -58.31249999863440792, 5.148502694627439702 ) ) ;
#57428=CARTESIAN_POINT ( 'NONE',  ( 1.060575238724906964E-15, 24.24999999999999645, 5.773502691896257311 ) ) ;
#57429=ADVANCED_FACE ( 'NONE', ( #3829 ), #32777, .T. ) ;
#57430=CARTESIAN_POINT ( 'NONE',  ( 1.975475456537005874E-15, -88.74999999999998579, 5.000000000000000000 ) ) ;
#57431=CARTESIAN_POINT ( 'NONE',  ( 4.458734124999998549, 0.2708333346989263979, -2.574251347313721627 ) ) ;
#57432=LINE ( 'NONE', #13352, #29775 ) ;
#57433=CARTESIAN_POINT ( 'NONE',  ( -9.184850993605147944E-16, -141.2500000000000284, 5.000000000000000000 ) ) ;
#57434=CARTESIAN_POINT ( 'NONE',  ( -4.458734124999998549, 10.52083333469892779, 2.574251347313722516 ) ) ;
#57436=CARTESIAN_POINT ( 'NONE',  ( 5.000000000000000000, -42.49999999999999289, -6.123233995736766282E-16 ) ) ;
#57438=CARTESIAN_POINT ( 'NONE',  ( -9.184850993605147944E-16, -168.3750000027312126, 5.000000000000000000 ) ) ;
#57439=CARTESIAN_POINT ( 'NONE',  ( 4.458734125000001214, -47.89583333196775072, 2.574251347313718519 ) ) ;
#57440=CARTESIAN_POINT ( 'NONE',  ( -4.458734124999999437, -158.1875000013655779, -5.460374474430324690E-16 ) ) ;
#57441=CARTESIAN_POINT ( 'NONE',  ( -2.500000000000000444, -49.04166666393547303, -4.330127018922193649 ) ) ;
#57443=CARTESIAN_POINT ( 'NONE',  ( 4.458734124999998549, -24.72916666530106866, -2.574251347313721627 ) ) ;
#57445=LINE ( 'NONE', #18510, #4993 ) ;
#57447=CARTESIAN_POINT ( 'NONE',  ( 3.152801135295367541, -161.3125000013656063, -3.152801135295367541 ) ) ;
#57451=CARTESIAN_POINT ( 'NONE',  ( -2.229367062499996610, -37.39583333196773651, 3.861377020970582219 ) ) ;
#57453=( BOUNDED_CURVE ( )  B_SPLINE_CURVE ( 2, ( #48106, #22737, #13388, #62608, #37516, #14006, #18531, #2801, #28801 ),
 .UNSPECIFIED., .F., .F. ) 
 B_SPLINE_CURVE_WITH_KNOTS ( ( 3, 2, 2, 2, 3 ),
 ( 0.9479166666666666297, 0.9486111111111110716, 0.9499999999999999556, 0.9513888888888888395, 0.9520833333333332815 ),
 .UNSPECIFIED. ) 
 CURVE ( )  GEOMETRIC_REPRESENTATION_ITEM ( )  RATIONAL_B_SPLINE_CURVE ( ( 0.9330127018922194093, 0.9330127018922194093, 1.000000000000000000, 0.8660254037844387076, 1.000000000000000000, 0.8660254037844387076, 1.000000000000000000, 0.9330127018922194093, 0.9330127018922194093 ) ) 
 REPRESENTATION_ITEM ( '' )  );
#57463=CARTESIAN_POINT ( 'NONE',  ( 9.457646018065525792E-16, -85.31249999863439371, 5.148502694627439702 ) ) ;
#57467=CARTESIAN_POINT ( 'NONE',  ( -6.972266317189433020E-16, -57.25000000000000000, -5.000000000000000000 ) ) ;
#57471=ADVANCED_FACE ( 'NONE', ( #51770 ), #2894, .T. ) ;
#57473=( BOUNDED_CURVE ( )  B_SPLINE_CURVE ( 2, ( #58882, #16024, #43764, #25995, #48910, #60740, #35971, #44401, #38941 ),
 .UNSPECIFIED., .F., .F. ) 
 B_SPLINE_CURVE_WITH_KNOTS ( ( 3, 2, 2, 2, 3 ),
 ( 0.5062499999999999778, 0.5069444444444444198, 0.5083333333333333037, 0.5097222222222221877, 0.5104166666666666297 ),
 .UNSPECIFIED. ) 
 CURVE ( )  GEOMETRIC_REPRESENTATION_ITEM ( )  RATIONAL_B_SPLINE_CURVE ( ( 0.9330127018922194093, 0.9330127018922194093, 1.000000000000000000, 0.8660254037844387076, 1.000000000000000000, 0.8660254037844387076, 1.000000000000000000, 0.9330127018922194093, 0.9330127018922194093 ) ) 
 REPRESENTATION_ITEM ( '' )  );
#57474=CARTESIAN_POINT ( 'NONE',  ( 1.975475456537005874E-15, -23.75000000000000000, 5.000000000000000000 ) ) ;
#57477=LINE ( 'NONE', #38763, #53034 ) ;
#57478=EDGE_CURVE ( 'NONE', #47300, #23480, #51180, .T. ) ;
#57480=CARTESIAN_POINT ( 'NONE',  ( 9.457646018065525792E-16, -86.31249999863440792, 5.148502694627439702 ) ) ;
#57484=CARTESIAN_POINT ( 'NONE',  ( 2.499999999999998668, -9.208333330602146205, -4.330127018922193649 ) ) ;
#57487=CARTESIAN_POINT ( 'NONE',  ( -2.071067811865475061, -166.8125000027312126, -5.000000000000000888 ) ) ;
#57494=CARTESIAN_POINT ( 'NONE',  ( 5.000000000000000888, -86.45833333060213022, 2.886751345948126879 ) ) ;
#57496=CARTESIAN_POINT ( 'NONE',  ( -4.458734124999999437, -11.31249999863440792, 0.000000000000000000 ) ) ;
#57498=ORIENTED_EDGE ( 'NONE', *, *, #33158, .F. ) ;
#57499=CARTESIAN_POINT ( 'NONE',  ( 4.458734124999998549, -38.97916666530107221, -2.574251347313721627 ) ) ;
#57502=CARTESIAN_POINT ( 'NONE',  ( 1.975475456537005874E-15, -77.75000000000000000, 5.000000000000000000 ) ) ;
#57503=DIRECTION ( 'NONE',  ( -0.000000000000000000, 1.000000000000000000, -0.000000000000000000 ) ) ;
#57504=CARTESIAN_POINT ( 'NONE',  ( -5.000000000000000000, -27.99999999999999645, 0.000000000000000000 ) ) ;
#57507=CARTESIAN_POINT ( 'NONE',  ( 4.458734125000001214, 15.10416666803225993, 2.574251347313718519 ) ) ;
#57510=CARTESIAN_POINT ( 'NONE',  ( 4.458734124999999437, -81.06249999863440792, -5.460374474430324690E-16 ) ) ;
#57512=CARTESIAN_POINT ( 'NONE',  ( 5.000000000000000000, 13.62500000273118417, -6.123233995736766282E-16 ) ) ;
#57516=CARTESIAN_POINT ( 'NONE',  ( 5.000000000000000888, -29.58333333333332504, 2.886751345948126879 ) ) ;
#57517=CARTESIAN_POINT ( 'NONE',  ( 4.458734125000001214, -34.89583333196772941, 2.574251347313718519 ) ) ;
#57518=FACE_OUTER_BOUND ( 'NONE', #61732, .T. ) ;
#57519=CARTESIAN_POINT ( 'NONE',  ( -5.000000000000000000, -28.95833333060215153, -2.886751345948128211 ) ) ;
#57520=CARTESIAN_POINT ( 'NONE',  ( 9.457646018065525792E-16, -60.06249999863440792, 5.148502694627439702 ) ) ;
#57522=CARTESIAN_POINT ( 'NONE',  ( -4.458734124999999437, -8.562499998634406140, 0.000000000000000000 ) ) ;
#57524=CARTESIAN_POINT ( 'NONE',  ( -3.535250795749689387E-16, -76.24999999999998579, -5.773502691896257311 ) ) ;
#57528=CARTESIAN_POINT ( 'NONE',  ( -5.000000000000000000, -78.87499999726881583, 0.000000000000000000 ) ) ;
#57532=CARTESIAN_POINT ( 'NONE',  ( 2.229367062500001939, -20.22916666530107221, 3.861377020970579999 ) ) ;
#57533=CARTESIAN_POINT ( 'NONE',  ( 2.229367062500001939, -56.22916666530107221, 3.861377020970579999 ) ) ;
#57536=CARTESIAN_POINT ( 'NONE',  ( 4.458734124999999437, -166.7500000013655779, 1.846868145590737864 ) ) ;
#57538=CARTESIAN_POINT ( 'NONE',  ( 2.499999999999998668, -50.20833333060213732, -4.330127018922193649 ) ) ;
#57539=EDGE_LOOP ( 'NONE', ( #3500, #36868, #23200, #12511 ) ) ;
#57545=CARTESIAN_POINT ( 'NONE',  ( -4.458734125000000326, -145.2500000013655779, -1.846868145590735644 ) ) ;
#57549=CARTESIAN_POINT ( 'NONE',  ( 9.457646018065525792E-16, -70.31249999863439371, 5.148502694627439702 ) ) ;
#57551=CARTESIAN_POINT ( 'NONE',  ( 5.000000000000000888, -43.58333333333333570, 2.886751345948126879 ) ) ;
#57552=EDGE_CURVE ( 'NONE', #57658, #55786, #34341, .T. ) ;
#57554=CARTESIAN_POINT ( 'NONE',  ( -8.190561711645485556E-16, -142.6875000013656063, 4.458734124999999437 ) ) ;
#57556=ORIENTED_EDGE ( 'NONE', *, *, #33015, .T. ) ;
#57557=CARTESIAN_POINT ( 'NONE',  ( -5.000000000000000000, -49.95833333060213022, -2.886751345948128211 ) ) ;
#57559=CARTESIAN_POINT ( 'NONE',  ( 3.535533905932736864, -160.1250000000000284, 3.535533905932738641 ) ) ;
#57562=CARTESIAN_POINT ( 'NONE',  ( -6.972266317189433020E-16, -54.12499999726880162, -5.000000000000000000 ) ) ;
#57564=CARTESIAN_POINT ( 'NONE',  ( -4.458734124999999437, 22.43750000136559564, 0.000000000000000000 ) ) ;
#57567=EDGE_CURVE ( 'NONE', #7190, #15348, #40063, .T. ) ;
#57571=CARTESIAN_POINT ( 'NONE',  ( -4.458734124999997661, 4.770833334698926009, 2.574251347313722516 ) ) ;
#57573=CARTESIAN_POINT ( 'NONE',  ( 9.457646018065525792E-16, -19.31249999863440792, 5.148502694627439702 ) ) ;
#57576=CARTESIAN_POINT ( 'NONE',  ( 4.458734124999999437, -154.5000000013656347, 1.846868145590737864 ) ) ;
#57580=CARTESIAN_POINT ( 'NONE',  ( 4.458734125000001214, 29.10416666803225993, 2.574251347313718519 ) ) ;
#57581=CARTESIAN_POINT ( 'NONE',  ( -2.229367062499996610, -39.14583333196773651, 3.861377020970582219 ) ) ;
#57584=CARTESIAN_POINT ( 'NONE',  ( 9.457646018065525792E-16, -67.31249999863440792, 5.148502694627439702 ) ) ;
#57586=CARTESIAN_POINT ( 'NONE',  ( 1.062108568985190270E-13, -13.12499999726881583, -4.999999999999999112 ) ) ;
#57587=DIRECTION ( 'NONE',  ( -0.000000000000000000, 1.000000000000000000, -0.000000000000000000 ) ) ;
#57588=ORIENTED_EDGE ( 'NONE', *, *, #28767, .F. ) ;
#57589=LINE ( 'NONE', #57891, #22242 ) ;
#57590=CARTESIAN_POINT ( 'NONE',  ( 2.500000000000002220, 2.458333336064519870, 4.330127018922192761 ) ) ;
#57591=CARTESIAN_POINT ( 'NONE',  ( 5.000000000000000888, -14.58333333333333037, 2.886751345948126879 ) ) ;
#57592=CARTESIAN_POINT ( 'NONE',  ( -4.458734124999999437, -14.31249999863440436, 0.000000000000000000 ) ) ;
#57593=CARTESIAN_POINT ( 'NONE',  ( 9.457646018065525792E-16, -78.06249999863440792, 5.148502694627439702 ) ) ;
#57595=CARTESIAN_POINT ( 'NONE',  ( -4.999999999999999112, -12.79166666393547835, 2.886751345948131764 ) ) ;
#57596=CARTESIAN_POINT ( 'NONE',  ( 4.458734125000001214, -43.89583333196775072, 2.574251347313718519 ) ) ;
#57597=VERTEX_POINT ( 'NONE', #44307 ) ;
#57598=CARTESIAN_POINT ( 'NONE',  ( -1.339745962155613368, 29.79465819873851729, -5.000000000000000000 ) ) ;
#57599=CARTESIAN_POINT ( 'NONE',  ( -2.229367062499996610, 9.604166668032261711, 3.861377020970582219 ) ) ;
#57600=ORIENTED_EDGE ( 'NONE', *, *, #52232, .F. ) ;
#57602=CARTESIAN_POINT ( 'NONE',  ( -2.499999999999996447, -58.83333333333333570, 4.330127018922195425 ) ) ;
#57603=CARTESIAN_POINT ( 'NONE',  ( 1.846868145590736310, -157.8750000013656063, 4.458734124999999437 ) ) ;
#57605=CARTESIAN_POINT ( 'NONE',  ( -6.972266317189433020E-16, -65.24999999999998579, -5.000000000000000000 ) ) ;
#57606=CARTESIAN_POINT ( 'NONE',  ( 3.535533905932738197, -165.8750000000000284, -3.535533905932738197 ) ) ;
#57607=CARTESIAN_POINT ( 'NONE',  ( 5.000000000000000000, -11.41666666666666607, -2.886751345948130876 ) ) ;
#57609=CARTESIAN_POINT ( 'NONE',  ( -2.229367062499996610, -4.395833331967740065, 3.861377020970582219 ) ) ;
#57610=CARTESIAN_POINT ( 'NONE',  ( -2.229367062500000163, -40.72916666530107221, -3.861377020970580443 ) ) ;
#57611=CARTESIAN_POINT ( 'NONE',  ( 2.500000000000002220, -67.54166666393547303, 4.330127018922192761 ) ) ;
#57612=CARTESIAN_POINT ( 'NONE',  ( -4.458734125000000326, -152.0000000013655779, -1.846868145590735644 ) ) ;
#57614=CARTESIAN_POINT ( 'NONE',  ( -9.184850993605147944E-16, -167.3750000027312126, 5.000000000000000000 ) ) ;
#57616=CARTESIAN_POINT ( 'NONE',  ( -5.000000000000000888, -148.5625000027311842, 2.071067811865474617 ) ) ;
#57618=CARTESIAN_POINT ( 'NONE',  ( 2.229367062499998831, -69.89583333196773651, -3.861377020970580887 ) ) ;
#57619=CARTESIAN_POINT ( 'NONE',  ( 2.730187237215162345E-16, -147.4375000013656063, -4.458734124999999437 ) ) ;
#57620=ORIENTED_EDGE ( 'NONE', *, *, #2512, .T. ) ;
#57624=CARTESIAN_POINT ( 'NONE',  ( -2.229367062499996610, -0.1458333319677394824, 3.861377020970582219 ) ) ;
#57625=CARTESIAN_POINT ( 'NONE',  ( 1.975475456537005874E-15, -79.74999999999998579, 5.000000000000000000 ) ) ;
#57626=CARTESIAN_POINT ( 'NONE',  ( -8.190561711645485556E-16, -151.6875000013656063, 4.458734124999999437 ) ) ;
#57628=VERTEX_POINT ( 'NONE', #54611 ) ;
#57630=DIRECTION ( 'NONE',  ( 0.000000000000000000, 0.000000000000000000, 1.000000000000000000 ) ) ;
#57633=VECTOR ( 'NONE', #9070, 1000.000000000000000 ) ;
#57634=DIRECTION ( 'NONE',  ( -0.000000000000000000, 1.000000000000000000, -0.000000000000000000 ) ) ;
#57636=CARTESIAN_POINT ( 'NONE',  ( 5.000000000000000888, -87.58333333333332860, 2.886751345948126879 ) ) ;
#57638=DIRECTION ( 'NONE',  ( -0.000000000000000000, 1.000000000000000000, -0.000000000000000000 ) ) ;
#57641=CARTESIAN_POINT ( 'NONE',  ( -4.458734124999999437, 22.68750000136559564, 0.000000000000000000 ) ) ;
#57643=CARTESIAN_POINT ( 'NONE',  ( -2.229367062500000163, -4.729166665301071326, -3.861377020970580443 ) ) ;
#57646=CARTESIAN_POINT ( 'NONE',  ( 5.000000000000000000, -142.1250000027312126, 0.000000000000000000 ) ) ;
#57647=CARTESIAN_POINT ( 'NONE',  ( 5.000000000000000000, -75.37499999726880162, -6.123233995736766282E-16 ) ) ;
#57652=CARTESIAN_POINT ( 'NONE',  ( 1.975475456537005874E-15, -42.74999999999999289, 5.000000000000000000 ) ) ;
#57655=CARTESIAN_POINT ( 'NONE',  ( -8.190561711645485556E-16, -158.9375000013655779, 4.458734124999999437 ) ) ;
#57658=VERTEX_POINT ( 'NONE', #33717 ) ;
#57659=CARTESIAN_POINT ( 'NONE',  ( 2.229367062500001939, 16.77083333469892779, 3.861377020970579999 ) ) ;
#57660=ORIENTED_EDGE ( 'NONE', *, *, #45686, .T. ) ;
#57664=CARTESIAN_POINT ( 'NONE',  ( 5.000000000000000000, -162.0000000000000000, 0.000000000000000000 ) ) ;
#57665=CARTESIAN_POINT ( 'NONE',  ( -5.000000000000000000, 5.000000000000000888, 0.000000000000000000 ) ) ;
#57666=ADVANCED_FACE ( 'NONE', ( #20196 ), #10535, .T. ) ;
#57667=CARTESIAN_POINT ( 'NONE',  ( 4.458734124999999437, -63.81249999863440792, -5.460374474430324690E-16 ) ) ;
#57668=CARTESIAN_POINT ( 'NONE',  ( 5.000000000000000888, 3.541666669397852019, 2.886751345948126879 ) ) ;
#57669=CARTESIAN_POINT ( 'NONE',  ( -4.458734124999999437, -30.31249999863440436, 0.000000000000000000 ) ) ;
#57671=CARTESIAN_POINT ( 'NONE',  ( -4.764381983412779477E-15, 26.37500000273118417, 5.000000000000000000 ) ) ;
#57672=CARTESIAN_POINT ( 'NONE',  ( 3.061616997868383141E-16, -151.8750000027311842, -5.000000000000000000 ) ) ;
#57673=CARTESIAN_POINT ( 'NONE',  ( 1.060575238724906964E-15, -44.74999999999999289, 5.773502691896257311 ) ) ;
#57674=CARTESIAN_POINT ( 'NONE',  ( 5.000000000000000000, -26.37499999726881583, -6.123233995736766282E-16 ) ) ;
#57676=CARTESIAN_POINT ( 'NONE',  ( 2.071067811865306751, -154.8125000000000000, -5.000000000000171418 ) ) ;
#57677=CARTESIAN_POINT ( 'NONE',  ( 9.457646018065525792E-16, -63.06249999863440081, 5.148502694627439702 ) ) ;
#57678=CARTESIAN_POINT ( 'NONE',  ( -4.458734124999999437, -148.1875000013656063, -5.460374474430324690E-16 ) ) ;
#57680=CARTESIAN_POINT ( 'NONE',  ( 9.457646018065525792E-16, -75.06249999863439371, 5.148502694627439702 ) ) ;
#57682=CARTESIAN_POINT ( 'NONE',  ( -4.458734124999998549, -25.47916666530106866, 2.574251347313722516 ) ) ;
#57683=CARTESIAN_POINT ( 'NONE',  ( 2.499999999999998668, -65.20833333060213022, -4.330127018922193649 ) ) ;
#57688=CARTESIAN_POINT ( 'NONE',  ( 5.000000000000000000, -21.29166666393548013, -2.886751345948130876 ) ) ;
#57691=CARTESIAN_POINT ( 'NONE',  ( 4.458734125000001214, -53.14583333196773651, 2.574251347313718519 ) ) ;
#57693=ORIENTED_EDGE ( 'NONE', *, *, #18173, .F. ) ;
#57697=CARTESIAN_POINT ( 'NONE',  ( 2.229367062499998831, 17.35416666803225993, -3.861377020970580887 ) ) ;
#57700=CARTESIAN_POINT ( 'NONE',  ( -1.846868145590734756, -165.1250000013656347, -4.458734124999999437 ) ) ;
#57703=CARTESIAN_POINT ( 'NONE',  ( 0.000000000000000000, -170.0000000000000000, 0.000000000000000000 ) ) ;
#57710=CYLINDRICAL_SURFACE ( 'NONE', #13093, 5.000000000000000000 ) ;
#57711=CARTESIAN_POINT ( 'NONE',  ( 6.123233995736766282E-16, -170.0000000000000000, -5.000000000000000000 ) ) ;
#57717=CARTESIAN_POINT ( 'NONE',  ( 2.071067811865475505, -151.9375000027312126, -5.000000000000000888 ) ) ;
#57718=ORIENTED_EDGE ( 'NONE', *, *, #43588, .F. ) ;
#57723=CARTESIAN_POINT ( 'NONE',  ( -3.535533905932738641, -142.3750000000000000, 3.535533905932737309 ) ) ;
#57726=CARTESIAN_POINT ( 'NONE',  ( 1.975475456537005874E-15, -7.750000000000000000, 5.000000000000000000 ) ) ;
#57727=CARTESIAN_POINT ( 'NONE',  ( -4.458734124999997661, -32.22916666530106511, 2.574251347313722516 ) ) ;
#57729=DIRECTION ( 'NONE',  ( -0.000000000000000000, 1.000000000000000000, -0.000000000000000000 ) ) ;
#57731=CARTESIAN_POINT ( 'NONE',  ( -3.152801135295367985, -147.8125000013655779, 3.152801135295367096 ) ) ;
#57734=CARTESIAN_POINT ( 'NONE',  ( -4.458734124999997661, -55.47916666530106511, 2.574251347313722516 ) ) ;
#57737=CARTESIAN_POINT ( 'NONE',  ( -3.535250795749689387E-16, 19.74999999999999645, -5.773502691896257311 ) ) ;
#57738=EDGE_CURVE ( 'NONE', #45744, #4902, #59820, .T. ) ;
#57740=CARTESIAN_POINT ( 'NONE',  ( 2.229367062500001939, -1.979166665301068662, 3.861377020970579999 ) ) ;
#57741=CARTESIAN_POINT ( 'NONE',  ( -5.000000000000000000, -11.08333333333333393, -2.886751345948128211 ) ) ;
#57743=CARTESIAN_POINT ( 'NONE',  ( 4.458734124999998549, 10.02083333469892779, -2.574251347313721627 ) ) ;
#57748=CARTESIAN_POINT ( 'NONE',  ( 4.458734125000001214, -50.89583333196772230, 2.574251347313718519 ) ) ;
#57749=CARTESIAN_POINT ( 'NONE',  ( 4.458734125000000326, -160.6250000013655779, -1.846868145590734978 ) ) ;
#57751=CARTESIAN_POINT ( 'NONE',  ( 5.000000000000000000, -51.37499999726881583, -6.123233995736766282E-16 ) ) ;
#57753=CARTESIAN_POINT ( 'NONE',  ( 4.458734125000001214, -20.89583333196774007, 2.574251347313718519 ) ) ;
#57754=EDGE_CURVE ( 'NONE', #56488, #35184, #62640, .T. ) ;
#57755=ORIENTED_EDGE ( 'NONE', *, *, #53864, .F. ) ;
#57758=CARTESIAN_POINT ( 'NONE',  ( -4.458734125000001214, -161.8750000013656063, 1.846868145590734089 ) ) ;
#57759=ORIENTED_EDGE ( 'NONE', *, *, #48740, .T. ) ;
#57760=CARTESIAN_POINT ( 'NONE',  ( 0.000000000000000000, -170.0000000000000000, 0.000000000000000000 ) ) ;
#57762=CARTESIAN_POINT ( 'NONE',  ( 2.229367062499998831, -36.89583333196773651, -3.861377020970580887 ) ) ;
#57763=ORIENTED_EDGE ( 'NONE', *, *, #37421, .F. ) ;
#57764=ADVANCED_FACE ( 'NONE', ( #48818 ), #24384, .T. ) ;
#57768=ORIENTED_EDGE ( 'NONE', *, *, #4296, .F. ) ;
#57770=CARTESIAN_POINT ( 'NONE',  ( -4.458734124999999437, -86.64583333196773651, -2.574251347313719407 ) ) ;
#57773=CYLINDRICAL_SURFACE ( 'NONE', #1824, 5.000000000000000000 ) ;
#57776=LINE ( 'NONE', #38447, #35643 ) ;
#57779=CARTESIAN_POINT ( 'NONE',  ( 1.975475456537005874E-15, 5.375000002731185944, 5.000000000000000000 ) ) ;
#57781=EDGE_CURVE ( 'NONE', #1040, #22477, #5509, .T. ) ;
#57784=CARTESIAN_POINT ( 'NONE',  ( -1.339745962155610925, -60.79465819873851729, 5.000000000000000000 ) ) ;
#57785=CARTESIAN_POINT ( 'NONE',  ( -3.152548672688508926E-16, -86.81249999863439371, -5.148502694627439702 ) ) ;
#57789=CARTESIAN_POINT ( 'NONE',  ( 1.975475456537005874E-15, 18.37500000273118062, 5.000000000000000000 ) ) ;
#57791=CARTESIAN_POINT ( 'NONE',  ( -5.000000000000000000, -166.6250000027312126, -6.123233995736766282E-16 ) ) ;
#57799=CARTESIAN_POINT ( 'NONE',  ( -6.972266317189433020E-16, 16.74999999999999645, -5.000000000000000000 ) ) ;
#57801=CARTESIAN_POINT ( 'NONE',  ( 4.458734125000000326, -14.89583333196773474, 2.574251347313718519 ) ) ;
#57804=CARTESIAN_POINT ( 'NONE',  ( -4.458734124999997661, -42.47916666530106511, 2.574251347313722516 ) ) ;
#57805=CARTESIAN_POINT ( 'NONE',  ( 1.339745962155615144, -77.70534180126146850, 4.999999999999999112 ) ) ;
#57810=EDGE_CURVE ( 'NONE', #1054, #17081, #16881, .T. ) ;
#57811=CARTESIAN_POINT ( 'NONE',  ( 2.229367062499998831, 14.35416666803226171, -3.861377020970580887 ) ) ;
#57815=CARTESIAN_POINT ( 'NONE',  ( -2.500000000000000444, -65.04166666393547303, -4.330127018922193649 ) ) ;
#57816=CARTESIAN_POINT ( 'NONE',  ( 2.229367062500001939, -87.22916666530107932, 3.861377020970579999 ) ) ;
#57818=CARTESIAN_POINT ( 'NONE',  ( -5.000000000000000000, 11.12500000273118594, 0.000000000000000000 ) ) ;
#57819=VERTEX_POINT ( 'NONE', #42269 ) ;
#57821=CARTESIAN_POINT ( 'NONE',  ( -4.999999999999998224, 16.08333333333333215, 2.886751345948131764 ) ) ;
#57822=CARTESIAN_POINT ( 'NONE',  ( 0.000000000000000000, -170.0000000000000000, 0.000000000000000000 ) ) ;
#57823=CARTESIAN_POINT ( 'NONE',  ( -2.499999999999996447, -27.83333333333333570, 4.330127018922195425 ) ) ;
#57824=CARTESIAN_POINT ( 'NONE',  ( 2.229367062499998831, -30.64583333196773651, -3.861377020970580887 ) ) ;
#57827=CARTESIAN_POINT ( 'NONE',  ( 2.500000000000002220, -34.54166666393547303, 4.330127018922192761 ) ) ;
#57828=CARTESIAN_POINT ( 'NONE',  ( 4.458734124999998549, -62.72916666530106511, -2.574251347313721627 ) ) ;
#57832=CARTESIAN_POINT ( 'NONE',  ( -4.458734124999999437, -6.562499998634403475, 0.000000000000000000 ) ) ;
#57834=CARTESIAN_POINT ( 'NONE',  ( -2.500000000000000444, -78.16666666666665719, -4.330127018922193649 ) ) ;
#57837=CARTESIAN_POINT ( 'NONE',  ( 2.500000000000002220, -82.54166666393547303, 4.330127018922192761 ) ) ;
#57838=CYLINDRICAL_SURFACE ( 'NONE', #17957, 5.000000000000000000 ) ;
#57841=CARTESIAN_POINT ( 'NONE',  ( 2.229367062499998831, -20.89583333196774007, -3.861377020970580887 ) ) ;
#57842=CARTESIAN_POINT ( 'NONE',  ( -2.229367062500000163, -56.72916666530107221, -3.861377020970580443 ) ) ;
#57843=VERTEX_POINT ( 'NONE', #2731 ) ;
#57846=CARTESIAN_POINT ( 'NONE',  ( -3.152801135295367985, -165.0625000013656063, 3.152801135295367096 ) ) ;
#57855=CARTESIAN_POINT ( 'NONE',  ( -4.458734125000001214, -143.1250000013656063, 1.846868145590734089 ) ) ;
#57857=CARTESIAN_POINT ( 'NONE',  ( -4.729367062499999719, 29.84375000068279604, 0.000000000000000000 ) ) ;
#57859=CARTESIAN_POINT ( 'NONE',  ( 4.458734124999999437, -70.06249999863439371, -5.460374474430324690E-16 ) ) ;
#57861=CARTESIAN_POINT ( 'NONE',  ( -4.458734124999999437, -141.9375000013656063, -5.460374474430324690E-16 ) ) ;
#57868=CARTESIAN_POINT ( 'NONE',  ( 1.339745962155612702, -14.16965819600733312, -5.000000000000000000 ) ) ;
#57870=CARTESIAN_POINT ( 'NONE',  ( -2.229367062500000163, 24.27083333469892779, -3.861377020970580443 ) ) ;
#57871=CARTESIAN_POINT ( 'NONE',  ( -1.127183054612291972E-14, 23.37500000273118772, 4.999999999999999112 ) ) ;
#57876=CARTESIAN_POINT ( 'NONE',  ( 1.339745962155615144, -60.58034179853027723, 4.999999999999999112 ) ) ;
#57877=CARTESIAN_POINT ( 'NONE',  ( -4.458734124999997661, 3.770833334698929562, 2.574251347313722516 ) ) ;
#57878=CARTESIAN_POINT ( 'NONE',  ( -2.229367062500000163, -23.72916666530107577, -3.861377020970580443 ) ) ;
#57879=CARTESIAN_POINT ( 'NONE',  ( 3.152801135295366208, -155.5625000013656063, 3.152801135295367985 ) ) ;
#57882=CARTESIAN_POINT ( 'NONE',  ( -4.458734124999999437, 28.60416666803226349, -2.574251347313719407 ) ) ;
#57886=CARTESIAN_POINT ( 'NONE',  ( 4.458734124999999437, -75.06249999863440792, -5.460374474430324690E-16 ) ) ;
#57888=CARTESIAN_POINT ( 'NONE',  ( 1.975475456537005874E-15, -65.62499999726881583, 5.000000000000000000 ) ) ;
#57889=CARTESIAN_POINT ( 'NONE',  ( -6.972266317189433020E-16, -10.12499999726881406, -5.000000000000000000 ) ) ;
#57890=ORIENTED_EDGE ( 'NONE', *, *, #60657, .T. ) ;
#57891=CARTESIAN_POINT ( 'NONE',  ( 6.123233995736766282E-16, -170.0000000000000000, -5.000000000000000000 ) ) ;
#57892=( BOUNDED_CURVE ( )  B_SPLINE_CURVE ( 2, ( #49302, #24541, #33562, #116, #59274, #39011, #62844, #53183, #44467 ),
 .UNSPECIFIED., .F., .F. ) 
 B_SPLINE_CURVE_WITH_KNOTS ( ( 3, 2, 2, 2, 3 ),
 ( 0.2312500000000000111, 0.2319444444444444531, 0.2333333333333333370, 0.2347222222222222210, 0.2354166666666666630 ),
 .UNSPECIFIED. ) 
 CURVE ( )  GEOMETRIC_REPRESENTATION_ITEM ( )  RATIONAL_B_SPLINE_CURVE ( ( 0.9330127018922194093, 0.9330127018922194093, 1.000000000000000000, 0.8660254037844387076, 1.000000000000000000, 0.8660254037844387076, 1.000000000000000000, 0.9330127018922194093, 0.9330127018922194093 ) ) 
 REPRESENTATION_ITEM ( '' )  );
#57893=EDGE_CURVE ( 'NONE', #61326, #53004, #18663, .T. ) ;
#57894=CARTESIAN_POINT ( 'NONE',  ( -5.000000000000000000, 12.12500000273118772, 0.000000000000000000 ) ) ;
#57895=CARTESIAN_POINT ( 'NONE',  ( 5.000000000000000000, -12.49999999999999645, -6.123233995736766282E-16 ) ) ;
#57896=CARTESIAN_POINT ( 'NONE',  ( -3.152548672688508926E-16, -16.56249999863440792, -5.148502694627439702 ) ) ;
#57898=CARTESIAN_POINT ( 'NONE',  ( -2.229367062499996610, -75.14583333196773651, 3.861377020970582219 ) ) ;
#57899=CARTESIAN_POINT ( 'NONE',  ( 4.458734124999999437, -167.6875000013655779, 0.000000000000000000 ) ) ;
#57900=CARTESIAN_POINT ( 'NONE',  ( -2.499999999999996447, -16.70833333060214443, 4.330127018922195425 ) ) ;
#57901=CARTESIAN_POINT ( 'NONE',  ( -3.152548672688508926E-16, -46.56249999863440792, -5.148502694627439702 ) ) ;
#57902=ORIENTED_EDGE ( 'NONE', *, *, #35467, .T. ) ;
#57903=DIRECTION ( 'NONE',  ( -0.000000000000000000, 1.000000000000000000, -0.000000000000000000 ) ) ;
#57904=CARTESIAN_POINT ( 'NONE',  ( 4.458734124999998549, 6.020833334698928674, -2.574251347313721627 ) ) ;
#57905=VERTEX_POINT ( 'NONE', #6923 ) ;
#57907=CARTESIAN_POINT ( 'NONE',  ( -3.535250795749689387E-16, -60.25000000000000000, -5.773502691896257311 ) ) ;
#57909=CARTESIAN_POINT ( 'NONE',  ( -4.458734124999999437, -155.1875000013655779, -5.460374474430324690E-16 ) ) ;
#57912=CARTESIAN_POINT ( 'NONE',  ( -5.000000000000000000, -165.5000000000000000, -6.123233995736766282E-16 ) ) ;
#57913=EDGE_CURVE ( 'NONE', #59810, #29588, #14140, .T. ) ;
#57914=CARTESIAN_POINT ( 'NONE',  ( -6.972266317189433020E-16, 5.875000002731184168, -5.000000000000000000 ) ) ;
#57916=CARTESIAN_POINT ( 'NONE',  ( -3.152548672688508926E-16, -3.812499998634408360, -5.148502694627439702 ) ) ;
#57917=CARTESIAN_POINT ( 'NONE',  ( -4.458734124999999437, -39.56249999863440081, 0.000000000000000000 ) ) ;
#57921=CARTESIAN_POINT ( 'NONE',  ( 3.152801135295366208, -149.5625000013655779, 3.152801135295367985 ) ) ;
#57927=CARTESIAN_POINT ( 'NONE',  ( 5.000000000000000000, -2.374999997268815388, -6.123233995736766282E-16 ) ) ;
#57928=CARTESIAN_POINT ( 'NONE',  ( 2.229367062499998831, -75.89583333196773651, -3.861377020970580887 ) ) ;
#57933=CARTESIAN_POINT ( 'NONE',  ( -4.458734124999998549, 0.7708333346989267865, 2.574251347313722516 ) ) ;
#57935=CARTESIAN_POINT ( 'NONE',  ( 2.730187237215162345E-16, -151.1875000013656063, -4.458734124999999437 ) ) ;
#57936=( BOUNDED_CURVE ( )  B_SPLINE_CURVE ( 2, ( #6453, #60803, #15774, #26062, #11577, #6131, #26700, #31197, #15460 ),
 .UNSPECIFIED., .F., .F. ) 
 B_SPLINE_CURVE_WITH_KNOTS ( ( 3, 2, 2, 2, 3 ),
 ( 0.9770833333333333037, 0.9777777777777777457, 0.9791666666666666297, 0.9805555555555555136, 0.9812499999999999556 ),
 .UNSPECIFIED. ) 
 CURVE ( )  GEOMETRIC_REPRESENTATION_ITEM ( )  RATIONAL_B_SPLINE_CURVE ( ( 0.9330127018922194093, 0.9330127018922194093, 1.000000000000000000, 0.8660254037844387076, 1.000000000000000000, 0.8660254037844387076, 1.000000000000000000, 0.9330127018922194093, 0.9330127018922194093 ) ) 
 REPRESENTATION_ITEM ( '' )  );
#57941=CARTESIAN_POINT ( 'NONE',  ( 1.339745962155612702, -12.16965819600733667, -5.000000000000000000 ) ) ;
#57947=CARTESIAN_POINT ( 'NONE',  ( 1.975475456537005874E-15, -64.62499999726880162, 5.000000000000000000 ) ) ;
#57949=CARTESIAN_POINT ( 'NONE',  ( 5.000000000000000888, -44.58333333333333570, 2.886751345948126879 ) ) ;
#57950=CARTESIAN_POINT ( 'NONE',  ( -2.229367062499996610, 21.85416666803226349, 3.861377020970582219 ) ) ;
#57952=CARTESIAN_POINT ( 'NONE',  ( -4.458734124999997661, -6.479166665301072214, 2.574251347313722516 ) ) ;
#57953=CARTESIAN_POINT ( 'NONE',  ( 0.000000000000000000, -170.0000000000000000, 0.000000000000000000 ) ) ;
#57955=CARTESIAN_POINT ( 'NONE',  ( 3.152801135295367541, -166.3125000013656063, -3.152801135295367541 ) ) ;
#57961=CYLINDRICAL_SURFACE ( 'NONE', #18276, 5.000000000000000000 ) ;
#57963=CARTESIAN_POINT ( 'NONE',  ( -3.152801135295367096, -156.3125000013656063, -3.152801135295367541 ) ) ;
#57966=ORIENTED_EDGE ( 'NONE', *, *, #6409, .F. ) ;
#57970=CARTESIAN_POINT ( 'NONE',  ( -6.972266317189433020E-16, -88.12499999726880162, -5.000000000000000000 ) ) ;
#57971=CARTESIAN_POINT ( 'NONE',  ( 5.000000000000000000, 1.500000000000001332, -6.123233995736766282E-16 ) ) ;
#57972=CARTESIAN_POINT ( 'NONE',  ( -4.458734124999999437, -60.39583333196774362, -2.574251347313719407 ) ) ;
#57973=CARTESIAN_POINT ( 'NONE',  ( -2.499999999999996447, 1.291666669397853351, 4.330127018922195425 ) ) ;
#57974=CARTESIAN_POINT ( 'NONE',  ( -4.458734124999999437, -29.39583333196773296, -2.574251347313719407 ) ) ;
#57978=CARTESIAN_POINT ( 'NONE',  ( -2.499999999999996447, -45.83333333333333570, 4.330127018922195425 ) ) ;
#57981=CARTESIAN_POINT ( 'NONE',  ( 5.000000000000000000, -155.0625000000000284, 2.071067811865478614 ) ) ;
#57982=CARTESIAN_POINT ( 'NONE',  ( 4.458734125000001214, -68.89583333196773651, 2.574251347313718519 ) ) ;
#57983=CARTESIAN_POINT ( 'NONE',  ( 2.730187237215162345E-16, -149.4375000013656063, -4.458734124999999437 ) ) ;
#57984=CARTESIAN_POINT ( 'NONE',  ( -4.458734124999999437, -74.31249999863440792, 0.000000000000000000 ) ) ;
#57986=CARTESIAN_POINT ( 'NONE',  ( -2.229367062499996610, -23.39583333196773651, 3.861377020970582219 ) ) ;
#57987=CARTESIAN_POINT ( 'NONE',  ( 5.000000000000000000, -65.29166666393548724, -2.886751345948129988 ) ) ;
#57988=ORIENTED_EDGE ( 'NONE', *, *, #20766, .T. ) ;
#57989=CARTESIAN_POINT ( 'NONE',  ( -5.000000000000000000, -152.6250000027312126, -6.123233995736766282E-16 ) ) ;
#57994=ORIENTED_EDGE ( 'NONE', *, *, #15760, .F. ) ;
#57995=CARTESIAN_POINT ( 'NONE',  ( -2.499999999999996447, -82.83333333333332860, 4.330127018922195425 ) ) ;
#57996=CARTESIAN_POINT ( 'NONE',  ( -4.458734124999999437, -52.56249999863440792, 0.000000000000000000 ) ) ;
#57998=ORIENTED_EDGE ( 'NONE', *, *, #17229, .T. ) ;
#57999=VECTOR ( 'NONE', #61246, 1000.000000000000000 ) ;
#58000=CARTESIAN_POINT ( 'NONE',  ( 3.061616997868383141E-16, -141.7500000000000284, -5.000000000000000000 ) ) ;
#58001=CARTESIAN_POINT ( 'NONE',  ( 4.458734124999999437, 20.18750000136559208, -5.460374474430324690E-16 ) ) ;
#58003=CARTESIAN_POINT ( 'NONE',  ( 6.123233995736766282E-16, -170.0000000000000000, -5.000000000000000000 ) ) ;
#58004=CARTESIAN_POINT ( 'NONE',  ( 4.458734124999999437, -166.4375000013655779, 0.000000000000000000 ) ) ;
#58005=ORIENTED_EDGE ( 'NONE', *, *, #48798, .F. ) ;
#58007=CARTESIAN_POINT ( 'NONE',  ( -5.000000000000000888, -153.5625000000000853, -2.071067811865475949 ) ) ;
#58009=( BOUNDED_CURVE ( )  B_SPLINE_CURVE ( 2, ( #24844, #25154, #58931, #23034, #39618, #58308, #15187, #34163, #33857 ),
 .UNSPECIFIED., .F., .F. ) 
 B_SPLINE_CURVE_WITH_KNOTS ( ( 3, 2, 2, 2, 3 ),
 ( 0.1062499999999999972, 0.1069444444444444392, 0.1083333333333333370, 0.1097222222222222210, 0.1104166666666666630 ),
 .UNSPECIFIED. ) 
 CURVE ( )  GEOMETRIC_REPRESENTATION_ITEM ( )  RATIONAL_B_SPLINE_CURVE ( ( 0.9330127018922194093, 0.9330127018922194093, 1.000000000000000000, 0.8660254037844387076, 1.000000000000000000, 0.8660254037844387076, 1.000000000000000000, 0.9330127018922194093, 0.9330127018922194093 ) ) 
 REPRESENTATION_ITEM ( '' )  );
#58010=LINE ( 'NONE', #13936, #14079 ) ;
#58013=CARTESIAN_POINT ( 'NONE',  ( 1.339745962155615144, -20.70534180126147916, 4.999999999999999112 ) ) ;
#58018=CARTESIAN_POINT ( 'NONE',  ( 2.499999999999998668, 11.66666666666666607, -4.330127018922193649 ) ) ;
#58020=CARTESIAN_POINT ( 'NONE',  ( -5.000000000000000888, -148.5625000027312126, 2.071067811865474617 ) ) ;
#58025=CARTESIAN_POINT ( 'NONE',  ( 3.535533905932738197, -144.8750000000000000, -3.535533905932738197 ) ) ;
#58027=CARTESIAN_POINT ( 'NONE',  ( -4.458734124999999437, -169.1875000013656063, -5.460374474430324690E-16 ) ) ;
#58028=CARTESIAN_POINT ( 'NONE',  ( 4.458734124999999437, -30.81249999863440436, -5.460374474430324690E-16 ) ) ;
#58031=CARTESIAN_POINT ( 'NONE',  ( -4.458734124999999437, -146.9375000013656063, -5.460374474430324690E-16 ) ) ;
#58032=EDGE_LOOP ( 'NONE', ( #30105, #29875, #32030, #46340 ) ) ;
#58033=CARTESIAN_POINT ( 'NONE',  ( -4.999999999999999112, -89.79166666393547303, 2.886751345948131764 ) ) ;
#58035=CARTESIAN_POINT ( 'NONE',  ( -3.152548672688508926E-16, -54.81249999863440081, -5.148502694627439702 ) ) ;
#58038=CARTESIAN_POINT ( 'NONE',  ( -2.500000000000000444, 20.83333333333333215, -4.330127018922193649 ) ) ;
#58039=DIRECTION ( 'NONE',  ( 0.000000000000000000, 0.000000000000000000, 1.000000000000000000 ) ) ;
#58040=AXIS2_PLACEMENT_3D ( 'NONE', #19929, #44689, #15114 ) ;
#58041=CARTESIAN_POINT ( 'NONE',  ( 2.229367062500001939, -7.979166665301073991, 3.861377020970579999 ) ) ;
#58042=CARTESIAN_POINT ( 'NONE',  ( 2.500000000000002220, -48.66666666666666430, 4.330127018922192761 ) ) ;
#58044=CARTESIAN_POINT ( 'NONE',  ( 2.229367062499998831, 12.10416666803226171, -3.861377020970580887 ) ) ;
#58045=CARTESIAN_POINT ( 'NONE',  ( 5.000000000000000888, -53.45833333060213732, 2.886751345948126879 ) ) ;
#58048=CARTESIAN_POINT ( 'NONE',  ( -4.458734124999998549, -50.22916666530107221, 2.574251347313722516 ) ) ;
#58049=CARTESIAN_POINT ( 'NONE',  ( -8.190561711645485556E-16, -161.9375000013655779, 4.458734124999999437 ) ) ;
#58050=CARTESIAN_POINT ( 'NONE',  ( -2.499999999999996447, -49.70833333060213732, 4.330127018922195425 ) ) ;
#58052=CARTESIAN_POINT ( 'NONE',  ( -2.229367062499996610, -24.14583333196773651, 3.861377020970582219 ) ) ;
#58054=( BOUNDED_CURVE ( )  B_SPLINE_CURVE ( 2, ( #17105, #42176, #22891, #57309, #61183, #51528, #2637, #27700, #3279 ),
 .UNSPECIFIED., .F., .F. ) 
 B_SPLINE_CURVE_WITH_KNOTS ( ( 3, 2, 2, 2, 3 ),
 ( 0.2937500000000000111, 0.2944444444444444531, 0.2958333333333333370, 0.2972222222222222210, 0.2979166666666666630 ),
 .UNSPECIFIED. ) 
 CURVE ( )  GEOMETRIC_REPRESENTATION_ITEM ( )  RATIONAL_B_SPLINE_CURVE ( ( 0.9330127018922194093, 0.9330127018922194093, 1.000000000000000000, 0.8660254037844387076, 1.000000000000000000, 0.8660254037844387076, 1.000000000000000000, 0.9330127018922194093, 0.9330127018922194093 ) ) 
 REPRESENTATION_ITEM ( '' )  );
#58055=CARTESIAN_POINT ( 'NONE',  ( 6.123233995736766282E-16, -170.0000000000000000, -5.000000000000000000 ) ) ;
#58057=CARTESIAN_POINT ( 'NONE',  ( -4.458734125000001214, -158.8750000013655779, 1.846868145590734089 ) ) ;
#58061=CARTESIAN_POINT ( 'NONE',  ( -6.972266317189433020E-16, -20.24999999999999645, -5.000000000000000000 ) ) ;
#58062=CARTESIAN_POINT ( 'NONE',  ( 4.458734124999999437, -38.06249999863440792, -5.460374474430324690E-16 ) ) ;
#58067=EDGE_LOOP ( 'NONE', ( #7907, #20980, #57216, #57763 ) ) ;
#58068=CARTESIAN_POINT ( 'NONE',  ( 2.229367062500001939, -85.22916666530107932, 3.861377020970579999 ) ) ;
#58072=CARTESIAN_POINT ( 'NONE',  ( -4.999999999999998224, -44.79166666393547303, 2.886751345948131764 ) ) ;
#58078=VECTOR ( 'NONE', #57634, 1000.000000000000000 ) ;
#58079=LINE ( 'NONE', #48728, #54584 ) ;
#58082=CARTESIAN_POINT ( 'NONE',  ( 1.975475456537005874E-15, -69.74999999999998579, 5.000000000000000000 ) ) ;
#58083=CARTESIAN_POINT ( 'NONE',  ( 4.458734124999999437, -84.06249999863439371, -5.460374474430324690E-16 ) ) ;
#58086=ORIENTED_EDGE ( 'NONE', *, *, #37086, .T. ) ;
#58087=CARTESIAN_POINT ( 'NONE',  ( -4.999999999999998224, 18.20833333606451632, 2.886751345948131764 ) ) ;
#58089=CARTESIAN_POINT ( 'NONE',  ( -3.535533905932738641, -163.5000000027312126, 3.535533905932737309 ) ) ;
#58092=CARTESIAN_POINT ( 'NONE',  ( -5.000000000000000000, -30.00000000000000000, 0.000000000000000000 ) ) ;
#58101=CARTESIAN_POINT ( 'NONE',  ( 9.457646018065525792E-16, -15.06249999863440259, 5.148502694627439702 ) ) ;
#58104=CARTESIAN_POINT ( 'NONE',  ( 4.458734125000000326, -39.14583333196773651, 2.574251347313718519 ) ) ;
#58105=( BOUNDED_CURVE ( )  B_SPLINE_CURVE ( 2, ( #62131, #42810, #43433, #32853, #3592, #38603, #33791, #61821, #56993 ),
 .UNSPECIFIED., .F., .F. ) 
 B_SPLINE_CURVE_WITH_KNOTS ( ( 3, 2, 2, 2, 3 ),
 ( 0.4937500000000000222, 0.4944444444444444642, 0.4958333333333333481, 0.4972222222222222321, 0.4979166666666666741 ),
 .UNSPECIFIED. ) 
 CURVE ( )  GEOMETRIC_REPRESENTATION_ITEM ( )  RATIONAL_B_SPLINE_CURVE ( ( 0.9330127018922194093, 0.9330127018922194093, 1.000000000000000000, 0.8660254037844387076, 1.000000000000000000, 0.8660254037844387076, 1.000000000000000000, 0.9330127018922194093, 0.9330127018922194093 ) ) 
 REPRESENTATION_ITEM ( '' )  );
#58106=CARTESIAN_POINT ( 'NONE',  ( 1.339745962155612702, -77.29465819873853150, -5.000000000000000000 ) ) ;
#58107=CARTESIAN_POINT ( 'NONE',  ( -5.000000000000000000, -12.08333333333333570, -2.886751345948128211 ) ) ;
#58111=CARTESIAN_POINT ( 'NONE',  ( -3.152548672688508926E-16, 9.437500001365593860, -5.148502694627439702 ) ) ;
#58112=CARTESIAN_POINT ( 'NONE',  ( -1.339745962155610925, -81.66965819600736154, 5.000000000000000000 ) ) ;
#58114=CARTESIAN_POINT ( 'NONE',  ( -4.458734124999999437, -90.56249999863440792, 0.000000000000000000 ) ) ;
#58116=CARTESIAN_POINT ( 'NONE',  ( -4.999999999999999112, 13.20833333606451809, 2.886751345948131764 ) ) ;
#58117=ORIENTED_EDGE ( 'NONE', *, *, #31908, .T. ) ;
#58120=CARTESIAN_POINT ( 'NONE',  ( 3.535533905932738197, -166.8750000000000284, -3.535533905932738197 ) ) ;
#58122=CARTESIAN_POINT ( 'NONE',  ( 2.500000000000002220, -28.66666666666666785, 4.330127018922192761 ) ) ;
#58123=CARTESIAN_POINT ( 'NONE',  ( 9.457646018065525792E-16, -34.06249999863440792, 5.148502694627439702 ) ) ;
#58124=CARTESIAN_POINT ( 'NONE',  ( 2.499999999999998668, -34.20833333060213732, -4.330127018922193649 ) ) ;
#58126=CARTESIAN_POINT ( 'NONE',  ( -3.152548672688508926E-16, -68.56249999863439371, -5.148502694627439702 ) ) ;
#58129=CARTESIAN_POINT ( 'NONE',  ( 2.229367062500001939, -13.22916666530107221, 3.861377020970579999 ) ) ;
#58130=ORIENTED_EDGE ( 'NONE', *, *, #27592, .T. ) ;
#58131=CARTESIAN_POINT ( 'NONE',  ( 2.499999999999998668, -78.33333333333332860, -4.330127018922193649 ) ) ;
#58134=CARTESIAN_POINT ( 'NONE',  ( -3.535250795749689387E-16, -84.12499999726880162, -5.773502691896257311 ) ) ;
#58135=CARTESIAN_POINT ( 'NONE',  ( 1.975475456537005874E-15, 10.37500000273118417, 5.000000000000000000 ) ) ;
#58138=CARTESIAN_POINT ( 'NONE',  ( -4.458734124999999437, -23.56249999863440436, 0.000000000000000000 ) ) ;
#58139=CARTESIAN_POINT ( 'NONE',  ( -4.458734124999999437, -60.64583333196774362, -2.574251347313719407 ) ) ;
#58140=EDGE_LOOP ( 'NONE', ( #32011, #28300, #59322, #10116 ) ) ;
#58142=CARTESIAN_POINT ( 'NONE',  ( -4.458734124999999437, -168.1875000013655779, -5.460374474430324690E-16 ) ) ;
#58145=ORIENTED_EDGE ( 'NONE', *, *, #60733, .F. ) ;
#58150=EDGE_CURVE ( 'NONE', #54054, #52029, #62542, .T. ) ;
#58153=CARTESIAN_POINT ( 'NONE',  ( 3.152801135295366208, -142.8125000013655779, 3.152801135295367985 ) ) ;
#58157=CARTESIAN_POINT ( 'NONE',  ( 2.229367062500001939, -71.22916666530107932, 3.861377020970579999 ) ) ;
#58159=CARTESIAN_POINT ( 'NONE',  ( 0.000000000000000000, -170.0000000000000000, 0.000000000000000000 ) ) ;
#58160=CARTESIAN_POINT ( 'NONE',  ( 2.730187237215162345E-16, -141.1875000013656063, -4.458734124999999437 ) ) ;
#58162=ORIENTED_EDGE ( 'NONE', *, *, #49598, .T. ) ;
#58164=CARTESIAN_POINT ( 'NONE',  ( 0.000000000000000000, -170.0000000000000000, 0.000000000000000000 ) ) ;
#58165=CARTESIAN_POINT ( 'NONE',  ( -9.184850993605147944E-16, -144.3750000027312126, 5.000000000000000000 ) ) ;
#58171=CARTESIAN_POINT ( 'NONE',  ( -4.458734124999997661, 22.52083333469892423, 2.574251347313722516 ) ) ;
#58172=FACE_OUTER_BOUND ( 'NONE', #42449, .T. ) ;
#58173=AXIS2_PLACEMENT_3D ( 'NONE', #42973, #3751, #52633 ) ;
#58180=CARTESIAN_POINT ( 'NONE',  ( 2.229367062499998831, -0.6458333319677399542, -3.861377020970580887 ) ) ;
#58182=CARTESIAN_POINT ( 'NONE',  ( 4.458734124999998549, -23.97916666530107577, -2.574251347313721627 ) ) ;
#58183=CARTESIAN_POINT ( 'NONE',  ( 4.458734124999999437, -155.4375000013655779, 0.000000000000000000 ) ) ;
#58187=DIRECTION ( 'NONE',  ( 0.000000000000000000, 0.000000000000000000, 1.000000000000000000 ) ) ;
#58189=CARTESIAN_POINT ( 'NONE',  ( 9.457646018065525792E-16, -72.31249999863439371, 5.148502694627439702 ) ) ;
#58191=CARTESIAN_POINT ( 'NONE',  ( -5.000000000000000000, -65.87499999726881583, 0.000000000000000000 ) ) ;
#58192=CARTESIAN_POINT ( 'NONE',  ( 1.060575238724906964E-15, 28.37500000273118417, 5.773502691896257311 ) ) ;
#58194=CARTESIAN_POINT ( 'NONE',  ( -5.000000000000000888, -140.5625000000000000, -2.071067811865475949 ) ) ;
#58196=CARTESIAN_POINT ( 'NONE',  ( -5.000000000000000000, -12.99999999999999822, 0.000000000000000000 ) ) ;
#58197=CARTESIAN_POINT ( 'NONE',  ( 2.229367062500001939, -17.97916666530106866, 3.861377020970579999 ) ) ;
#58199=CARTESIAN_POINT ( 'NONE',  ( 4.458734124999999437, -79.81249999863440792, -5.460374474430324690E-16 ) ) ;
#58200=( BOUNDED_CURVE ( )  B_SPLINE_CURVE ( 2, ( #63014, #48823, #57559, #33101, #48511, #13786, #43990, #33409, #18921 ),
 .UNSPECIFIED., .F., .F. ) 
 B_SPLINE_CURVE_WITH_KNOTS ( ( 3, 2, 2, 2, 3 ),
 ( 0.3250000000000002887, 0.3291666666666669405, 0.3333333333333335924, 0.3375000000000002998, 0.3416666666666669516 ),
 .UNSPECIFIED. ) 
 CURVE ( )  GEOMETRIC_REPRESENTATION_ITEM ( )  RATIONAL_B_SPLINE_CURVE ( ( 0.9999999999999948930, 0.9238795325112918455, 1.000000000000000000, 0.9238795325112867385, 1.000000000000000000, 0.9238795325112867385, 1.000000000000000000, 0.9238795325112816315, 1.000000000000005107 ) ) 
 REPRESENTATION_ITEM ( '' )  );
#58201=CARTESIAN_POINT ( 'NONE',  ( -8.190561711645485556E-16, -167.9375000013655779, 4.458734124999999437 ) ) ;
#58202=CARTESIAN_POINT ( 'NONE',  ( 2.500000000000002220, -20.54166666393548013, 4.330127018922192761 ) ) ;
#58203=CARTESIAN_POINT ( 'NONE',  ( 9.457646018065525792E-16, -45.06249999863440792, 5.148502694627439702 ) ) ;
#58206=CARTESIAN_POINT ( 'NONE',  ( 9.457646018065525792E-16, 0.6875000013655957476, 5.148502694627439702 ) ) ;
#58209=CARTESIAN_POINT ( 'NONE',  ( 2.499999999999998668, -63.33333333333332149, -4.330127018922193649 ) ) ;
#58210=CARTESIAN_POINT ( 'NONE',  ( 3.152801135295367541, -154.5625000013656063, -3.152801135295367541 ) ) ;
#58213=CARTESIAN_POINT ( 'NONE',  ( 5.000000000000000000, -163.0625000000000000, 2.071067811865478614 ) ) ;
#58214=FACE_OUTER_BOUND ( 'NONE', #18084, .T. ) ;
#58217=CARTESIAN_POINT ( 'NONE',  ( 2.229367062500001939, -3.229166665301069550, 3.861377020970579999 ) ) ;
#58219=CARTESIAN_POINT ( 'NONE',  ( -2.229367062500000163, -42.72916666530107932, -3.861377020970580443 ) ) ;
#58221=CARTESIAN_POINT ( 'NONE',  ( 1.846868145590736310, -148.6250000013655779, 4.458734124999999437 ) ) ;
#58229=EDGE_CURVE ( 'NONE', #14032, #39802, #46283, .T. ) ;
#58231=FACE_OUTER_BOUND ( 'NONE', #19374, .T. ) ;
#58233=EDGE_CURVE ( 'NONE', #44335, #41004, #44791, .T. ) ;
#58234=CARTESIAN_POINT ( 'NONE',  ( 5.000000000000000000, -79.29166666393547303, -2.886751345948130876 ) ) ;
#58235=CARTESIAN_POINT ( 'NONE',  ( -4.458734124999998549, -1.229166665301071326, 2.574251347313722516 ) ) ;
#58236=CARTESIAN_POINT ( 'NONE',  ( -2.499999999999996447, -79.83333333333332860, 4.330127018922195425 ) ) ;
#58237=CARTESIAN_POINT ( 'NONE',  ( 4.458734124999999437, -153.3750000013656063, -1.846868145590734978 ) ) ;
#58247=CARTESIAN_POINT ( 'NONE',  ( 2.500000000000002220, 8.458333336064518093, 4.330127018922192761 ) ) ;
#58252=CARTESIAN_POINT ( 'NONE',  ( 1.339745962155612702, -44.29465819873851729, -5.000000000000000000 ) ) ;
#58255=CARTESIAN_POINT ( 'NONE',  ( -4.458734124999999437, 15.68750000136559564, 0.000000000000000000 ) ) ;
#58256=EDGE_CURVE ( 'NONE', #45174, #55117, #55176, .T. ) ;
#58258=CARTESIAN_POINT ( 'NONE',  ( -4.458734124999997661, -9.479166665301068662, 2.574251347313722516 ) ) ;
#58259=( BOUNDED_CURVE ( )  B_SPLINE_CURVE ( 2, ( #10491, #11131, #20475, #15326, #25929, #6013, #45548, #21431, #30757 ),
 .UNSPECIFIED., .F., .F. ) 
 B_SPLINE_CURVE_WITH_KNOTS ( ( 3, 2, 2, 2, 3 ),
 ( 0.1812499999999999944, 0.1819444444444444364, 0.1833333333333333204, 0.1847222222222222321, 0.1854166666666666741 ),
 .UNSPECIFIED. ) 
 CURVE ( )  GEOMETRIC_REPRESENTATION_ITEM ( )  RATIONAL_B_SPLINE_CURVE ( ( 0.9330127018922194093, 0.9330127018922194093, 1.000000000000000000, 0.8660254037844387076, 1.000000000000000000, 0.8660254037844387076, 1.000000000000000000, 0.9330127018922194093, 0.9330127018922194093 ) ) 
 REPRESENTATION_ITEM ( '' )  );
#58263=CARTESIAN_POINT ( 'NONE',  ( 2.730187237215162345E-16, -168.1875000013655779, -4.458734124999999437 ) ) ;
#58265=ADVANCED_FACE ( 'NONE', ( #50015 ), #31034, .T. ) ;
#58269=AXIS2_PLACEMENT_3D ( 'NONE', #22266, #42187, #57630 ) ;
#58275=CARTESIAN_POINT ( 'NONE',  ( -1.846868145590734756, -153.3750000013656063, -4.458734124999999437 ) ) ;
#58277=CARTESIAN_POINT ( 'NONE',  ( 1.975475456537005874E-15, -56.62499999726880162, 5.000000000000000000 ) ) ;
#58278=FACE_OUTER_BOUND ( 'NONE', #28183, .T. ) ;
#58283=CARTESIAN_POINT ( 'NONE',  ( 2.071067811865561215, -162.1874999999999432, 4.999999999999913847 ) ) ;
#58284=CARTESIAN_POINT ( 'NONE',  ( 5.000000000000000000, 3.583333333333333925, -2.886751345948129988 ) ) ;
#58285=CARTESIAN_POINT ( 'NONE',  ( -2.229367062499996610, -60.14583333196774362, 3.861377020970582219 ) ) ;
#58287=CARTESIAN_POINT ( 'NONE',  ( 5.000000000000000000, -2.374999997268815388, -6.123233995736766282E-16 ) ) ;
#58288=CARTESIAN_POINT ( 'NONE',  ( -2.229367062499996610, -27.14583333196774007, 3.861377020970582219 ) ) ;
#58289=CARTESIAN_POINT ( 'NONE',  ( -1.339745962155610925, -41.79465819873852439, 5.000000000000000000 ) ) ;
#58290=CYLINDRICAL_SURFACE ( 'NONE', #4542, 5.000000000000000000 ) ;
#58291=CARTESIAN_POINT ( 'NONE',  ( 5.000000000000000888, 5.416666666666666963, 2.886751345948126879 ) ) ;
#58292=CARTESIAN_POINT ( 'NONE',  ( -2.499999999999996447, -42.83333333333333570, 4.330127018922195425 ) ) ;
#58293=( BOUNDED_CURVE ( )  B_SPLINE_CURVE ( 2, ( #35427, #25454, #49577, #25783, #15167, #10343, #10974, #25133, #45074 ),
 .UNSPECIFIED., .F., .F. ) 
 B_SPLINE_CURVE_WITH_KNOTS ( ( 3, 2, 2, 2, 3 ),
 ( 0.8979166666666666963, 0.8986111111111111382, 0.9000000000000000222, 0.9013888888888889062, 0.9020833333333333481 ),
 .UNSPECIFIED. ) 
 CURVE ( )  GEOMETRIC_REPRESENTATION_ITEM ( )  RATIONAL_B_SPLINE_CURVE ( ( 0.9330127018922194093, 0.9330127018922194093, 1.000000000000000000, 0.8660254037844387076, 1.000000000000000000, 0.8660254037844387076, 1.000000000000000000, 0.9330127018922194093, 0.9330127018922194093 ) ) 
 REPRESENTATION_ITEM ( '' )  );
#58296=CARTESIAN_POINT ( 'NONE',  ( 2.499999999999998668, -64.33333333333332860, -4.330127018922193649 ) ) ;
#58297=CARTESIAN_POINT ( 'NONE',  ( -3.152548672688508926E-16, -68.56249999863439371, -5.148502694627439702 ) ) ;
#58298=CARTESIAN_POINT ( 'NONE',  ( 1.846868145590736310, -143.8750000013656063, 4.458734124999999437 ) ) ;
#58299=CARTESIAN_POINT ( 'NONE',  ( -2.229367062500000163, -74.47916666530106511, -3.861377020970580443 ) ) ;
#58301=CARTESIAN_POINT ( 'NONE',  ( -2.229367062500000163, -22.72916666530107221, -3.861377020970580443 ) ) ;
#58302=CARTESIAN_POINT ( 'NONE',  ( -5.000000000000000000, -66.95833333060214443, -2.886751345948128211 ) ) ;
#58303=EDGE_LOOP ( 'NONE', ( #2101, #54831, #9022, #58757 ) ) ;
#58307=ORIENTED_EDGE ( 'NONE', *, *, #28314, .T. ) ;
#58308=CARTESIAN_POINT ( 'NONE',  ( -5.000000000000000000, 16.91666666666666785, -2.886751345948128211 ) ) ;
#58309=AXIS2_PLACEMENT_3D ( 'NONE', #43362, #23763, #62691 ) ;
#58310=CARTESIAN_POINT ( 'NONE',  ( -1.339745962155613812, -83.20534180126146850, -5.000000000000000000 ) ) ;
#58311=CARTESIAN_POINT ( 'NONE',  ( 9.457646018065525792E-16, -61.31249999863440792, 5.148502694627439702 ) ) ;
#58312=AXIS2_PLACEMENT_3D ( 'NONE', #27164, #41944, #27472 ) ;
#58316=CARTESIAN_POINT ( 'NONE',  ( 4.458734124999998549, 15.27083333469893134, -2.574251347313721627 ) ) ;
#58319=CARTESIAN_POINT ( 'NONE',  ( -3.152801135295367096, -165.0625000013656063, -3.152801135295367541 ) ) ;
#58322=CARTESIAN_POINT ( 'NONE',  ( -1.339745962155610925, -69.66965819600731891, 5.000000000000000000 ) ) ;
#58324=CARTESIAN_POINT ( 'NONE',  ( -3.535533905932738641, -162.5000000027312126, 3.535533905932737309 ) ) ;
#58327=CARTESIAN_POINT ( 'NONE',  ( 5.000000000000000000, -45.50000000000000000, -6.123233995736766282E-16 ) ) ;
#58328=CARTESIAN_POINT ( 'NONE',  ( 0.000000000000000000, -170.0000000000000000, 0.000000000000000000 ) ) ;
#58329=CARTESIAN_POINT ( 'NONE',  ( 5.000000000000000000, -18.37499999726881583, -6.123233995736766282E-16 ) ) ;
#58334=CARTESIAN_POINT ( 'NONE',  ( -3.152548672688508926E-16, 9.187500001365592084, -5.148502694627439702 ) ) ;
#58335=CARTESIAN_POINT ( 'NONE',  ( 0.000000000000000000, -170.0000000000000000, 0.000000000000000000 ) ) ;
#58337=CARTESIAN_POINT ( 'NONE',  ( -9.184850993605147944E-16, -151.3750000027311842, 5.000000000000000000 ) ) ;
#58342=CARTESIAN_POINT ( 'NONE',  ( -3.535533905932738641, -141.3750000000000000, 3.535533905932737309 ) ) ;
#58345=CARTESIAN_POINT ( 'NONE',  ( 3.152801135295366208, -164.8125000013656063, 3.152801135295367985 ) ) ;
#58346=CARTESIAN_POINT ( 'NONE',  ( -3.152548672688508926E-16, -31.56249999863440436, -5.148502694627439702 ) ) ;
#58348=DIRECTION ( 'NONE',  ( -0.000000000000000000, 1.000000000000000000, -0.000000000000000000 ) ) ;
#58350=CARTESIAN_POINT ( 'NONE',  ( 3.152801135295367541, -142.3125000013655779, -3.152801135295367541 ) ) ;
#58352=CARTESIAN_POINT ( 'NONE',  ( -2.229367062499996610, 27.60416666803225993, 3.861377020970582219 ) ) ;
#58354=CARTESIAN_POINT ( 'NONE',  ( -4.458734124999999437, -54.56249999863440081, 0.000000000000000000 ) ) ;
#58357=DIRECTION ( 'NONE',  ( -0.000000000000000000, 1.000000000000000000, -0.000000000000000000 ) ) ;
#58358=CARTESIAN_POINT ( 'NONE',  ( 2.500000000000002220, 21.33333333333333215, 4.330127018922192761 ) ) ;
#58359=AXIS2_PLACEMENT_3D ( 'NONE', #19762, #58686, #20411 ) ;
#58360=CARTESIAN_POINT ( 'NONE',  ( -2.500000000000000444, -37.04166666393548013, -4.330127018922193649 ) ) ;
#58361=CARTESIAN_POINT ( 'NONE',  ( -2.229367062500000163, -8.479166665301073991, -3.861377020970580443 ) ) ;
#58362=CARTESIAN_POINT ( 'NONE',  ( -9.184850993605147944E-16, -168.2500000000000000, 5.000000000000000000 ) ) ;
#58364=CYLINDRICAL_SURFACE ( 'NONE', #41544, 5.000000000000000000 ) ;
#58365=CARTESIAN_POINT ( 'NONE',  ( 1.339745962155615144, -53.58034179853029144, 4.999999999999999112 ) ) ;
#58367=CARTESIAN_POINT ( 'NONE',  ( 9.457646018065525792E-16, -56.06249999863440792, 5.148502694627439702 ) ) ;
#58368=CARTESIAN_POINT ( 'NONE',  ( -4.458734124999999437, -160.1875000013655779, -5.460374474430324690E-16 ) ) ;
#58370=CARTESIAN_POINT ( 'NONE',  ( -3.535250795749689387E-16, -48.12499999726880873, -5.773502691896257311 ) ) ;
#58371=ORIENTED_EDGE ( 'NONE', *, *, #54966, .T. ) ;
#58372=CARTESIAN_POINT ( 'NONE',  ( 4.458734124999999437, 4.937500001365595637, -5.460374474430324690E-16 ) ) ;
#58376=CARTESIAN_POINT ( 'NONE',  ( 1.846868145590735200, -161.2500000013655779, -4.458734125000000326 ) ) ;
#58377=VERTEX_POINT ( 'NONE', #16567 ) ;
#58378=UNCERTAINTY_MEASURE_WITH_UNIT (LENGTH_MEASURE( 1.000000000000000082E-05 ), #17021, 'distance_accuracy_value', 'NONE');
#58379=CARTESIAN_POINT ( 'NONE',  ( 1.975475456537005874E-15, -17.62499999726881583, 5.000000000000000000 ) ) ;
#58381=CARTESIAN_POINT ( 'NONE',  ( 5.000000000000000000, -47.37499999726880873, -6.123233995736766282E-16 ) ) ;
#58382=CARTESIAN_POINT ( 'NONE',  ( 9.457646018065525792E-16, -45.31249999863440081, 5.148502694627439702 ) ) ;
#58385=ADVANCED_FACE ( 'NONE', ( #44873 ), #11726, .T. ) ;
#58388=CARTESIAN_POINT ( 'NONE',  ( 5.000000000000000000, -24.37499999726881228, -6.123233995736766282E-16 ) ) ;
#58390=CARTESIAN_POINT ( 'NONE',  ( 4.458734124999998549, -87.97916666530107932, -2.574251347313721627 ) ) ;
#58392=CARTESIAN_POINT ( 'NONE',  ( -2.500000000000000444, 24.95833333606451987, -4.330127018922193649 ) ) ;
#58393=CARTESIAN_POINT ( 'NONE',  ( 5.000000000000000000, -169.0625000000000000, 2.071067811865478614 ) ) ;
#58395=CARTESIAN_POINT ( 'NONE',  ( 1.975475456537005874E-15, -61.62499999726880873, 5.000000000000000000 ) ) ;
#58402=CARTESIAN_POINT ( 'NONE',  ( 6.123233995736766282E-16, -170.0000000000000000, -5.000000000000000000 ) ) ;
#58404=CARTESIAN_POINT ( 'NONE',  ( 2.229367062500001939, -82.22916666530106511, 3.861377020970579999 ) ) ;
#58407=VERTEX_POINT ( 'NONE', #11095 ) ;
#58408=CARTESIAN_POINT ( 'NONE',  ( 3.061616997868383141E-16, -155.8750000027311842, -5.000000000000000000 ) ) ;
#58410=CARTESIAN_POINT ( 'NONE',  ( 2.071067811865475505, -160.9375000027312126, -5.000000000000000888 ) ) ;
#58412=CARTESIAN_POINT ( 'NONE',  ( -6.972266317189433020E-16, -49.12499999726880162, -5.000000000000000000 ) ) ;
#58415=AXIS2_PLACEMENT_3D ( 'NONE', #19418, #42605, #48678 ) ;
#58421=CARTESIAN_POINT ( 'NONE',  ( 3.061616997868383141E-16, -139.8750000027312126, -5.000000000000000000 ) ) ;
#58422=CARTESIAN_POINT ( 'NONE',  ( -2.229367062499996610, -16.14583333196773651, 3.861377020970582219 ) ) ;
#58423=CARTESIAN_POINT ( 'NONE',  ( 5.000000000000000000, -71.41666666666667140, -2.886751345948130876 ) ) ;
#58424=CARTESIAN_POINT ( 'NONE',  ( -3.535533905932738641, -155.3750000000000000, 3.535533905932737309 ) ) ;
#58426=CARTESIAN_POINT ( 'NONE',  ( 2.229367062500001939, -43.22916666530107932, 3.861377020970579999 ) ) ;
#58431=CARTESIAN_POINT ( 'NONE',  ( 4.458734124999998549, 10.27083333469892779, -2.574251347313721627 ) ) ;
#58433=CARTESIAN_POINT ( 'NONE',  ( -1.339745962155613812, -69.20534180126148271, -5.000000000000000000 ) ) ;
#58434=CARTESIAN_POINT ( 'NONE',  ( -4.458734124999997661, -86.47916666530107932, 2.574251347313722516 ) ) ;
#58437=CARTESIAN_POINT ( 'NONE',  ( -3.535250795749689387E-16, 14.87500000273118594, -5.773502691896257311 ) ) ;
#58441=CARTESIAN_POINT ( 'NONE',  ( 0.000000000000000000, -170.0000000000000000, 0.000000000000000000 ) ) ;
#58442=CYLINDRICAL_SURFACE ( 'NONE', #49163, 5.000000000000000000 ) ;
#58443=CARTESIAN_POINT ( 'NONE',  ( 5.000000000000000000, -34.50000000000000000, -6.123233995736766282E-16 ) ) ;
#58444=CARTESIAN_POINT ( 'NONE',  ( -2.229367062499996610, -37.14583333196773651, 3.861377020970582219 ) ) ;
#58445=ADVANCED_FACE ( 'NONE', ( #31342 ), #40364, .T. ) ;
#58446=VECTOR ( 'NONE', #33855, 1000.000000000000000 ) ;
#58447=CARTESIAN_POINT ( 'NONE',  ( -2.499999999999996447, -36.70833333060213732, 4.330127018922195425 ) ) ;
#58449=CARTESIAN_POINT ( 'NONE',  ( 2.229367062500001939, -66.97916666530106511, 3.861377020970579999 ) ) ;
#58450=ORIENTED_EDGE ( 'NONE', *, *, #9177, .T. ) ;
#58452=CARTESIAN_POINT ( 'NONE',  ( -3.152548672688508926E-16, -14.56249999863440436, -5.148502694627439702 ) ) ;
#58453=CARTESIAN_POINT ( 'NONE',  ( -4.458734124999999437, -15.56249999863440436, 0.000000000000000000 ) ) ;
#58454=ORIENTED_EDGE ( 'NONE', *, *, #28756, .F. ) ;
#58455=CARTESIAN_POINT ( 'NONE',  ( -2.500000000000000444, -75.16666666666665719, -4.330127018922193649 ) ) ;
#58458=CARTESIAN_POINT ( 'NONE',  ( -5.000000000000000000, -79.95833333060213022, -2.886751345948128211 ) ) ;
#58462=CARTESIAN_POINT ( 'NONE',  ( -2.229367062499996610, -24.39583333196773651, 3.861377020970582219 ) ) ;
#58463=EDGE_LOOP ( 'NONE', ( #32719, #2237, #3182, #21926 ) ) ;
#58464=CARTESIAN_POINT ( 'NONE',  ( -4.458734124999999437, -166.1875000013655779, -5.460374474430324690E-16 ) ) ;
#58466=CARTESIAN_POINT ( 'NONE',  ( 5.000000000000000000, -50.37499999726881583, -6.123233995736766282E-16 ) ) ;
#58472=CARTESIAN_POINT ( 'NONE',  ( -3.535533905932738641, -146.5000000027311842, 3.535533905932737309 ) ) ;
#58476=CARTESIAN_POINT ( 'NONE',  ( 2.730187237215162345E-16, -142.4375000013656063, -4.458734124999999437 ) ) ;
#58480=CARTESIAN_POINT ( 'NONE',  ( 2.229367062499998831, -69.89583333196773651, -3.861377020970580887 ) ) ;
#58483=CARTESIAN_POINT ( 'NONE',  ( 4.458734124999999437, -141.4375000013656063, 0.000000000000000000 ) ) ;
#58484=( BOUNDED_CURVE ( )  B_SPLINE_CURVE ( 2, ( #61777, #19261, #49173, #4789, #5113, #39512, #29536, #14121, #33747 ),
 .UNSPECIFIED., .F., .F. ) 
 B_SPLINE_CURVE_WITH_KNOTS ( ( 3, 2, 2, 2, 3 ),
 ( 0.3312499999999999889, 0.3319444444444444309, 0.3333333333333333148, 0.3347222222222221988, 0.3354166666666666963 ),
 .UNSPECIFIED. ) 
 CURVE ( )  GEOMETRIC_REPRESENTATION_ITEM ( )  RATIONAL_B_SPLINE_CURVE ( ( 0.9330127018922194093, 0.9330127018922194093, 1.000000000000000000, 0.8660254037844387076, 1.000000000000000000, 0.8660254037844387076, 1.000000000000000000, 0.9330127018922167448, 0.9330127018922194093 ) ) 
 REPRESENTATION_ITEM ( '' )  );
#58486=ORIENTED_EDGE ( 'NONE', *, *, #12665, .T. ) ;
#58488=DIRECTION ( 'NONE',  ( 0.000000000000000000, 0.000000000000000000, 1.000000000000000000 ) ) ;
#58493=VECTOR ( 'NONE', #40478, 1000.000000000000000 ) ;
#58494=CARTESIAN_POINT ( 'NONE',  ( 4.458734124999998549, 23.02083333469892423, -2.574251347313721627 ) ) ;
#58500=CARTESIAN_POINT ( 'NONE',  ( -6.972266317189433020E-16, -43.12499999726880873, -5.000000000000000000 ) ) ;
#58501=CARTESIAN_POINT ( 'NONE',  ( 2.229367062500001939, -0.9791666653010712151, 3.861377020970579999 ) ) ;
#58503=CARTESIAN_POINT ( 'NONE',  ( -2.229367062499996610, -23.39583333196773651, 3.861377020970582219 ) ) ;
#58506=CARTESIAN_POINT ( 'NONE',  ( 9.457646018065525792E-16, 25.93750000136559564, 5.148502694627439702 ) ) ;
#58509=CARTESIAN_POINT ( 'NONE',  ( -4.458734124999999437, -71.64583333196773651, -2.574251347313719407 ) ) ;
#58512=DIRECTION ( 'NONE',  ( -0.000000000000000000, 1.000000000000000000, -0.000000000000000000 ) ) ;
#58513=ORIENTED_EDGE ( 'NONE', *, *, #45176, .F. ) ;
#58515=CARTESIAN_POINT ( 'NONE',  ( 5.000000000000000000, -6.374999997268812280, -6.123233995736766282E-16 ) ) ;
#58516=CARTESIAN_POINT ( 'NONE',  ( 2.500000000000002220, -14.66666666666666785, 4.330127018922192761 ) ) ;
#58517=CARTESIAN_POINT ( 'NONE',  ( 2.229367062499998831, -17.64583333196773651, -3.861377020970580887 ) ) ;
#58518=EDGE_CURVE ( 'NONE', #41205, #1843, #22054, .T. ) ;
#58519=CARTESIAN_POINT ( 'NONE',  ( 4.458734124999999437, -80.81249999863440792, -5.460374474430324690E-16 ) ) ;
#58520=CARTESIAN_POINT ( 'NONE',  ( 4.458734124999999437, -166.7500000013655779, 1.846868145590737864 ) ) ;
#58521=CARTESIAN_POINT ( 'NONE',  ( -2.500000000000000444, -16.04166666393548368, -4.330127018922193649 ) ) ;
#58522=CARTESIAN_POINT ( 'NONE',  ( -4.458734124999999437, -52.31249999863440792, 0.000000000000000000 ) ) ;
#58524=CARTESIAN_POINT ( 'NONE',  ( 5.000000000000000000, -70.29166666393547303, -2.886751345948130876 ) ) ;
#58525=CARTESIAN_POINT ( 'NONE',  ( -9.184850993605147944E-16, -168.3750000027312126, 5.000000000000000000 ) ) ;
#58526=CARTESIAN_POINT ( 'NONE',  ( -2.229367062500000163, 0.2708333346989263979, -3.861377020970580443 ) ) ;
#58527=ORIENTED_EDGE ( 'NONE', *, *, #19247, .T. ) ;
#58529=CARTESIAN_POINT ( 'NONE',  ( -5.000000000000000000, -61.00000000000000000, 0.000000000000000000 ) ) ;
#58530=CARTESIAN_POINT ( 'NONE',  ( -3.152801135295367096, -157.3125000013656063, -3.152801135295367541 ) ) ;
#58533=CARTESIAN_POINT ( 'NONE',  ( -3.535533905932737309, -160.6250000000000284, -3.535533905932738197 ) ) ;
#58535=CARTESIAN_POINT ( 'NONE',  ( -2.499999999999996447, 11.16666666666666430, 4.330127018922195425 ) ) ;
#58536=VECTOR ( 'NONE', #59639, 1000.000000000000000 ) ;
#58538=CARTESIAN_POINT ( 'NONE',  ( 4.458734124999999437, -6.062499998634403475, -5.460374474430324690E-16 ) ) ;
#58539=CARTESIAN_POINT ( 'NONE',  ( -4.458734124999999437, -45.56249999863440081, 0.000000000000000000 ) ) ;
#58541=CARTESIAN_POINT ( 'NONE',  ( 1.846868145590735200, -147.2500000013656063, -4.458734125000000326 ) ) ;
#58542=EDGE_CURVE ( 'NONE', #32095, #58407, #20758, .T. ) ;
#58545=ORIENTED_EDGE ( 'NONE', *, *, #46136, .F. ) ;
#58551=EDGE_CURVE ( 'NONE', #50889, #38824, #13003, .T. ) ;
#58552=DIRECTION ( 'NONE',  ( 0.000000000000000000, 0.000000000000000000, 1.000000000000000000 ) ) ;
#58555=CARTESIAN_POINT ( 'NONE',  ( 2.229367062499998831, -3.645833331967739177, -3.861377020970580887 ) ) ;
#58557=CARTESIAN_POINT ( 'NONE',  ( -4.458734124999999437, -154.0000000013656063, -1.846868145590735644 ) ) ;
#58559=ORIENTED_EDGE ( 'NONE', *, *, #33927, .F. ) ;
#58561=LINE ( 'NONE', #24460, #50046 ) ;
#58562=CARTESIAN_POINT ( 'NONE',  ( 5.000000000000000888, -40.58333333333334281, 2.886751345948126879 ) ) ;
#58564=CARTESIAN_POINT ( 'NONE',  ( -5.000000000000000000, 28.12500000273118417, 0.000000000000000000 ) ) ;
#58566=( BOUNDED_CURVE ( )  B_SPLINE_CURVE ( 2, ( #57671, #42540, #57356, #13276, #43167, #47997, #32900, #3949, #62806 ),
 .UNSPECIFIED., .F., .F. ) 
 B_SPLINE_CURVE_WITH_KNOTS ( ( 3, 2, 2, 2, 3 ),
 ( 0.02291666666666666852, 0.02361111111111111049, 0.02500000000000000139, 0.02638888888888888881, 0.02708333333333333426 ),
 .UNSPECIFIED. ) 
 CURVE ( )  GEOMETRIC_REPRESENTATION_ITEM ( )  RATIONAL_B_SPLINE_CURVE ( ( 0.9330127018922194093, 0.9330127018922195203, 1.000000000000000000, 0.8660254037844387076, 1.000000000000000000, 0.8660254037844387076, 1.000000000000000000, 0.9330127018922191873, 0.9330127018922194093 ) ) 
 REPRESENTATION_ITEM ( '' )  );
#58570=LINE ( 'NONE', #52800, #48289 ) ;
#58572=DIRECTION ( 'NONE',  ( -0.000000000000000000, 1.000000000000000000, -0.000000000000000000 ) ) ;
#58573=ORIENTED_EDGE ( 'NONE', *, *, #22568, .F. ) ;
#58574=CARTESIAN_POINT ( 'NONE',  ( -3.152548672688508926E-16, 18.43750000136559564, -5.148502694627439702 ) ) ;
#58576=CARTESIAN_POINT ( 'NONE',  ( 2.229367062499998831, -6.895833331967741842, -3.861377020970580887 ) ) ;
#58577=CARTESIAN_POINT ( 'NONE',  ( 3.535533905932738197, -169.0000000027312126, -3.535533905932738197 ) ) ;
#58579=CARTESIAN_POINT ( 'NONE',  ( 4.458734125000000326, -166.3750000013655779, -1.846868145590734978 ) ) ;
#58585=( BOUNDED_CURVE ( )  B_SPLINE_CURVE ( 2, ( #10570, #5116, #55294, #44338, #49809, #19900, #39514, #5754, #59152 ),
 .UNSPECIFIED., .F., .F. ) 
 B_SPLINE_CURVE_WITH_KNOTS ( ( 3, 2, 2, 2, 3 ),
 ( 0.7145833333333333481, 0.7152777777777777901, 0.7166666666666666741, 0.7180555555555555580, 0.7187500000000000000 ),
 .UNSPECIFIED. ) 
 CURVE ( )  GEOMETRIC_REPRESENTATION_ITEM ( )  RATIONAL_B_SPLINE_CURVE ( ( 0.9330127018922194093, 0.9330127018922194093, 1.000000000000000000, 0.8660254037844387076, 1.000000000000000000, 0.8660254037844387076, 1.000000000000000000, 0.9330127018922194093, 0.9330127018922194093 ) ) 
 REPRESENTATION_ITEM ( '' )  );
#58588=CARTESIAN_POINT ( 'NONE',  ( -3.152801135295367985, -152.0625000013655779, 3.152801135295367096 ) ) ;
#58592=EDGE_LOOP ( 'NONE', ( #15157, #22884, #22359, #4420 ) ) ;
#58595=CARTESIAN_POINT ( 'NONE',  ( -6.972266317189433020E-16, 12.75000000000000178, -5.000000000000000000 ) ) ;
#58596=CARTESIAN_POINT ( 'NONE',  ( 2.499999999999998668, 4.666666666666666075, -4.330127018922193649 ) ) ;
#58597=CARTESIAN_POINT ( 'NONE',  ( 4.458734125000000326, -62.89583333196774362, 2.574251347313718519 ) ) ;
#58601=CARTESIAN_POINT ( 'NONE',  ( -2.500000000000000444, -4.041666663935479242, -4.330127018922193649 ) ) ;
#58602=CARTESIAN_POINT ( 'NONE',  ( -2.229367062500000163, -31.47916666530107577, -3.861377020970580443 ) ) ;
#58603=ORIENTED_EDGE ( 'NONE', *, *, #61045, .T. ) ;
#58604=CARTESIAN_POINT ( 'NONE',  ( -2.500000000000000444, -42.16666666666667140, -4.330127018922193649 ) ) ;
#58605=CARTESIAN_POINT ( 'NONE',  ( -6.972266317189433020E-16, -42.24999999999998579, -5.000000000000000000 ) ) ;
#58607=CARTESIAN_POINT ( 'NONE',  ( -3.535250795749689387E-16, -43.24999999999999289, -5.773502691896257311 ) ) ;
#58610=CARTESIAN_POINT ( 'NONE',  ( 2.229367062500001939, -67.97916666530106511, 3.861377020970579999 ) ) ;
#58611=CARTESIAN_POINT ( 'NONE',  ( -4.458734124999999437, -144.1875000013656063, -5.460374474430324690E-16 ) ) ;
#58612=CARTESIAN_POINT ( 'NONE',  ( -2.229367062500000163, -75.47916666530106511, -3.861377020970580443 ) ) ;
#58614=ADVANCED_FACE ( 'NONE', ( #8499 ), #32623, .T. ) ;
#58615=CARTESIAN_POINT ( 'NONE',  ( 4.458734124999999437, -30.06249999863440436, -5.460374474430324690E-16 ) ) ;
#58616=CARTESIAN_POINT ( 'NONE',  ( 1.060575238724906964E-15, -68.62499999726881583, 5.773502691896257311 ) ) ;
#58620=EDGE_LOOP ( 'NONE', ( #7385, #32444, #32605, #48335 ) ) ;
#58626=CARTESIAN_POINT ( 'NONE',  ( -4.458734124999999437, -58.64583333196774362, -2.574251347313719407 ) ) ;
#58628=ORIENTED_EDGE ( 'NONE', *, *, #9512, .F. ) ;
#58629=CARTESIAN_POINT ( 'NONE',  ( -5.000000000000000000, -146.5000000000000284, -6.123233995736766282E-16 ) ) ;
#58631=CARTESIAN_POINT ( 'NONE',  ( 4.458734124999998549, 13.27083333469892779, -2.574251347313721627 ) ) ;
#58633=CARTESIAN_POINT ( 'NONE',  ( 2.500000000000002220, -32.66666666666666430, 4.330127018922192761 ) ) ;
#58634=CARTESIAN_POINT ( 'NONE',  ( 2.730187237215162345E-16, -166.1875000013655779, -4.458734124999999437 ) ) ;
#58635=( BOUNDED_CURVE ( )  B_SPLINE_CURVE ( 2, ( #35993, #6724, #40486, #26334, #7045, #45951, #20883, #1916, #60127 ),
 .UNSPECIFIED., .F., .F. ) 
 B_SPLINE_CURVE_WITH_KNOTS ( ( 3, 2, 2, 2, 3 ),
 ( 0.4770833333333333592, 0.4777777777777778012, 0.4791666666666666852, 0.4805555555555555691, 0.4812500000000000111 ),
 .UNSPECIFIED. ) 
 CURVE ( )  GEOMETRIC_REPRESENTATION_ITEM ( )  RATIONAL_B_SPLINE_CURVE ( ( 0.9330127018922194093, 0.9330127018922220739, 1.000000000000000000, 0.8660254037844387076, 1.000000000000000000, 0.8660254037844387076, 1.000000000000000000, 0.9330127018922194093, 0.9330127018922194093 ) ) 
 REPRESENTATION_ITEM ( '' )  );
#58638=CARTESIAN_POINT ( 'NONE',  ( 1.975475456537005874E-15, -16.74999999999999645, 5.000000000000000000 ) ) ;
#58643=LINE ( 'NONE', #48352, #33709 ) ;
#58648=CARTESIAN_POINT ( 'NONE',  ( -4.458734124999997661, 8.520833334698926009, 2.574251347313722516 ) ) ;
#58650=CARTESIAN_POINT ( 'NONE',  ( 2.071067811865476394, -148.3125000027312126, 5.000000000000000000 ) ) ;
#58655=CARTESIAN_POINT ( 'NONE',  ( 5.000000000000000888, -141.9375000000000000, -2.071067811865475505 ) ) ;
#58657=CARTESIAN_POINT ( 'NONE',  ( 3.152801135295366208, -166.8125000013656063, 3.152801135295367985 ) ) ;
#58658=CARTESIAN_POINT ( 'NONE',  ( 4.458734125000000326, -31.89583333196773651, 2.574251347313718519 ) ) ;
#58660=CARTESIAN_POINT ( 'NONE',  ( 2.500000000000002220, -45.54166666393547303, 4.330127018922192761 ) ) ;
#58662=CARTESIAN_POINT ( 'NONE',  ( 1.846868145590735200, -143.2500000013655779, -4.458734125000000326 ) ) ;
#58663=ORIENTED_EDGE ( 'NONE', *, *, #14961, .T. ) ;
#58664=CARTESIAN_POINT ( 'NONE',  ( -2.229367062500000163, 29.27083333469892779, -3.861377020970580443 ) ) ;
#58665=CARTESIAN_POINT ( 'NONE',  ( 2.229367062499998831, -56.89583333196773651, -3.861377020970580887 ) ) ;
#58666=( BOUNDED_CURVE ( )  B_SPLINE_CURVE ( 2, ( #60991, #50371, #11444, #7278, #26889, #2452, #45542, #31063, #6630 ),
 .UNSPECIFIED., .F., .F. ) 
 B_SPLINE_CURVE_WITH_KNOTS ( ( 3, 2, 2, 2, 3 ),
 ( 0.3354166666666666963, 0.3361111111111111382, 0.3375000000000000222, 0.3388888888888889062, 0.3395833333333333481 ),
 .UNSPECIFIED. ) 
 CURVE ( )  GEOMETRIC_REPRESENTATION_ITEM ( )  RATIONAL_B_SPLINE_CURVE ( ( 0.9330127018922194093, 0.9330127018922220739, 1.000000000000000000, 0.8660254037844387076, 1.000000000000000000, 0.8660254037844387076, 1.000000000000000000, 0.9330127018922194093, 0.9330127018922194093 ) ) 
 REPRESENTATION_ITEM ( '' )  );
#58668=CARTESIAN_POINT ( 'NONE',  ( 5.000000000000000888, 17.41666666666666430, 2.886751345948126879 ) ) ;
#58669=CARTESIAN_POINT ( 'NONE',  ( -1.339745962155610925, -88.79465819873851729, 5.000000000000000000 ) ) ;
#58670=CARTESIAN_POINT ( 'NONE',  ( -2.229367062499996610, -4.145833331967739177, 3.861377020970582219 ) ) ;
#58671=CARTESIAN_POINT ( 'NONE',  ( -2.500000000000000444, -23.16666666666666785, -4.330127018922193649 ) ) ;
#58673=CARTESIAN_POINT ( 'NONE',  ( 0.000000000000000000, -170.0000000000000000, 0.000000000000000000 ) ) ;
#58675=LINE ( 'NONE', #63197, #19178 ) ;
#58678=PLANE ( 'NONE',  #8094 ) ;
#58679=CARTESIAN_POINT ( 'NONE',  ( 2.229367062500001939, -52.97916666530107221, 3.861377020970579999 ) ) ;
#58680=CARTESIAN_POINT ( 'NONE',  ( -1.846868145590737420, -158.0000000013655779, 4.458734124999999437 ) ) ;
#58681=CARTESIAN_POINT ( 'NONE',  ( -4.999999999999999112, -49.79166666393547303, 2.886751345948131764 ) ) ;
#58683=CARTESIAN_POINT ( 'NONE',  ( 4.458734125000001214, 3.854166668032260823, 2.574251347313718519 ) ) ;
#58684=ORIENTED_EDGE ( 'NONE', *, *, #39442, .F. ) ;
#58686=DIRECTION ( 'NONE',  ( -0.000000000000000000, 1.000000000000000000, -0.000000000000000000 ) ) ;
#58687=CARTESIAN_POINT ( 'NONE',  ( 1.846868145590735200, -158.2500000013656063, -4.458734125000000326 ) ) ;
#58689=ORIENTED_EDGE ( 'NONE', *, *, #56301, .T. ) ;
#58690=ADVANCED_FACE ( 'NONE', ( #27792 ), #42271, .T. ) ;
#58693=CARTESIAN_POINT ( 'NONE',  ( 4.458734124999999437, -41.06249999863440081, -5.460374474430324690E-16 ) ) ;
#58694=VERTEX_POINT ( 'NONE', #13322 ) ;
#58695=EDGE_CURVE ( 'NONE', #49893, #25625, #23739, .T. ) ;
#58696=CARTESIAN_POINT ( 'NONE',  ( -2.499999999999996447, -45.83333333333333570, 4.330127018922195425 ) ) ;
#58699=VERTEX_POINT ( 'NONE', #12376 ) ;
#58700=CARTESIAN_POINT ( 'NONE',  ( 4.458734124999998549, 27.27083333469892423, -2.574251347313721627 ) ) ;
#58702=CYLINDRICAL_SURFACE ( 'NONE', #48018, 5.000000000000000000 ) ;
#58707=VECTOR ( 'NONE', #56458, 1000.000000000000000 ) ;
#58709=CARTESIAN_POINT ( 'NONE',  ( -5.000000000000000000, -90.00000000000000000, 0.000000000000000000 ) ) ;
#58713=CARTESIAN_POINT ( 'NONE',  ( -5.000000000000000000, -66.95833333060214443, -2.886751345948128211 ) ) ;
#58718=CARTESIAN_POINT ( 'NONE',  ( 5.000000000000000000, -9.291666663935483683, -2.886751345948130876 ) ) ;
#58720=CARTESIAN_POINT ( 'NONE',  ( 2.071067811865476394, -160.3125000027312410, 5.000000000000000000 ) ) ;
#58722=CARTESIAN_POINT ( 'NONE',  ( 5.000000000000000000, -49.37499999726880873, -6.123233995736766282E-16 ) ) ;
#58730=CARTESIAN_POINT ( 'NONE',  ( -4.999999999999998224, -53.91666666666667140, 2.886751345948131764 ) ) ;
#58731=CARTESIAN_POINT ( 'NONE',  ( 4.458734125000000326, -11.89583333196774184, 2.574251347313718519 ) ) ;
#58733=CARTESIAN_POINT ( 'NONE',  ( -9.184850993605147944E-16, -155.2500000000000000, 5.000000000000000000 ) ) ;
#58736=CARTESIAN_POINT ( 'NONE',  ( -4.458734124999997661, -41.47916666530107932, 2.574251347313722516 ) ) ;
#58737=DIRECTION ( 'NONE',  ( 0.000000000000000000, 0.000000000000000000, 1.000000000000000000 ) ) ;
#58739=CARTESIAN_POINT ( 'NONE',  ( -6.972266317189433020E-16, -2.250000000000000000, -5.000000000000000000 ) ) ;
#58742=CARTESIAN_POINT ( 'NONE',  ( 2.229367062499998831, 11.35416666803225993, -3.861377020970580887 ) ) ;
#58744=CARTESIAN_POINT ( 'NONE',  ( 4.458734125000000326, -89.14583333196773651, 2.574251347313718519 ) ) ;
#58745=CARTESIAN_POINT ( 'NONE',  ( 4.458734124999999437, 21.93750000136559208, -5.460374474430324690E-16 ) ) ;
#58747=CARTESIAN_POINT ( 'NONE',  ( -3.535250795749689387E-16, 12.87500000273118417, -5.773502691896257311 ) ) ;
#58749=CARTESIAN_POINT ( 'NONE',  ( -4.999999999999998224, -6.791666663935481019, 2.886751345948131764 ) ) ;
#58751=FACE_OUTER_BOUND ( 'NONE', #58880, .T. ) ;
#58752=CARTESIAN_POINT ( 'NONE',  ( 2.500000000000002220, -34.66666666666666430, 4.330127018922192761 ) ) ;
#58753=CARTESIAN_POINT ( 'NONE',  ( 2.229367062500001939, -38.97916666530107221, 3.861377020970579999 ) ) ;
#58754=( BOUNDED_CURVE ( )  B_SPLINE_CURVE ( 2, ( #22330, #7225, #61254, #51911, #22652, #42562, #60940, #46765, #50961 ),
 .UNSPECIFIED., .F., .F. ) 
 B_SPLINE_CURVE_WITH_KNOTS ( ( 3, 2, 2, 2, 3 ),
 ( 0.3187499999999999778, 0.3194444444444444198, 0.3208333333333333592, 0.3222222222222222432, 0.3229166666666666852 ),
 .UNSPECIFIED. ) 
 CURVE ( )  GEOMETRIC_REPRESENTATION_ITEM ( )  RATIONAL_B_SPLINE_CURVE ( ( 0.9330127018922194093, 0.9330127018922194093, 1.000000000000000000, 0.8660254037844387076, 1.000000000000000000, 0.8660254037844387076, 1.000000000000000000, 0.9330127018922194093, 0.9330127018922194093 ) ) 
 REPRESENTATION_ITEM ( '' )  );
#58755=CARTESIAN_POINT ( 'NONE',  ( -2.500000000000000444, -34.04166666393547303, -4.330127018922193649 ) ) ;
#58756=CARTESIAN_POINT ( 'NONE',  ( 2.229367062499998831, -63.64583333196772941, -3.861377020970580887 ) ) ;
#58757=ORIENTED_EDGE ( 'NONE', *, *, #10205, .F. ) ;
#58759=CARTESIAN_POINT ( 'NONE',  ( 2.229367062499998831, -10.64583333196773829, -3.861377020970580887 ) ) ;
#58760=CARTESIAN_POINT ( 'NONE',  ( 2.229367062499998831, -16.89583333196773651, -3.861377020970580887 ) ) ;
#58762=CARTESIAN_POINT ( 'NONE',  ( -5.000000000000000000, -82.00000000000000000, 0.000000000000000000 ) ) ;
#58765=CARTESIAN_POINT ( 'NONE',  ( -5.000000000000000000, -81.87499999726881583, 0.000000000000000000 ) ) ;
#58769=CARTESIAN_POINT ( 'NONE',  ( 4.458734124999999437, -27.06249999863440081, -5.460374474430324690E-16 ) ) ;
#58770=EDGE_LOOP ( 'NONE', ( #44122, #13676, #52118, #49963 ) ) ;
#58772=CARTESIAN_POINT ( 'NONE',  ( -1.846868145590734756, -165.3750000013656347, -4.458734125000000326 ) ) ;
#58778=CARTESIAN_POINT ( 'NONE',  ( 4.458734124999999437, -144.6875000013656063, 0.000000000000000000 ) ) ;
#58779=CARTESIAN_POINT ( 'NONE',  ( 0.000000000000000000, -170.0000000000000000, 0.000000000000000000 ) ) ;
#58780=CARTESIAN_POINT ( 'NONE',  ( 1.975475456537005874E-15, 0.2500000000000001665, 5.000000000000000000 ) ) ;
#58783=EDGE_LOOP ( 'NONE', ( #13983, #28410, #59879, #37983 ) ) ;
#58784=CARTESIAN_POINT ( 'NONE',  ( 4.458734124999999437, -143.6875000013656063, 0.000000000000000000 ) ) ;
#58789=CARTESIAN_POINT ( 'NONE',  ( 9.457646018065525792E-16, -66.31249999863440792, 5.148502694627439702 ) ) ;
#58790=DIRECTION ( 'NONE',  ( -0.000000000000000000, 1.000000000000000000, -0.000000000000000000 ) ) ;
#58800=CARTESIAN_POINT ( 'NONE',  ( -2.229367062500000163, 22.27083333469892423, -3.861377020970580443 ) ) ;
#58801=CARTESIAN_POINT ( 'NONE',  ( 5.000000000000000888, -18.58333333333333215, 2.886751345948126879 ) ) ;
#58808=CARTESIAN_POINT ( 'NONE',  ( 4.458734124999999437, 4.187500001365595637, -5.460374474430324690E-16 ) ) ;
#58809=ORIENTED_EDGE ( 'NONE', *, *, #52399, .F. ) ;
#58810=CARTESIAN_POINT ( 'NONE',  ( -2.229367062499996610, -24.39583333196773651, 3.861377020970582219 ) ) ;
#58814=CARTESIAN_POINT ( 'NONE',  ( 4.458734124999999437, 25.18750000136559208, -5.460374474430324690E-16 ) ) ;
#58817=CARTESIAN_POINT ( 'NONE',  ( -4.458734124999999437, -70.64583333196773651, -2.574251347313719407 ) ) ;
#58820=CARTESIAN_POINT ( 'NONE',  ( -5.000000000000000000, 28.12500000273118417, 0.000000000000000000 ) ) ;
#58821=ORIENTED_EDGE ( 'NONE', *, *, #62515, .F. ) ;
#58822=CARTESIAN_POINT ( 'NONE',  ( -5.000000000000000000, -140.5000000000000000, -6.123233995736766282E-16 ) ) ;
#58824=CARTESIAN_POINT ( 'NONE',  ( -2.500000000000000444, -20.16666666666666430, -4.330127018922193649 ) ) ;
#58825=CARTESIAN_POINT ( 'NONE',  ( 9.457646018065525792E-16, -22.06249999863440436, 5.148502694627439702 ) ) ;
#58826=CARTESIAN_POINT ( 'NONE',  ( -2.229367062500000163, -80.47916666530106511, -3.861377020970580443 ) ) ;
#58827=CARTESIAN_POINT ( 'NONE',  ( -3.152801135295367096, -167.3125000013656063, -3.152801135295367541 ) ) ;
#58828=CARTESIAN_POINT ( 'NONE',  ( -5.000000000000000000, -15.87499999726881406, 0.000000000000000000 ) ) ;
#58829=CARTESIAN_POINT ( 'NONE',  ( -2.229367062499996610, -48.14583333196772941, 3.861377020970582219 ) ) ;
#58832=CARTESIAN_POINT ( 'NONE',  ( -1.339745962155564296, -28.08034179853029144, -5.000000000000028422 ) ) ;
#58833=CARTESIAN_POINT ( 'NONE',  ( 4.458734125000001214, 1.854166668032262155, 2.574251347313718519 ) ) ;
#58837=CARTESIAN_POINT ( 'NONE',  ( -2.499999999999996447, -66.83333333333332860, 4.330127018922195425 ) ) ;
#58838=CARTESIAN_POINT ( 'NONE',  ( -4.458734124999999437, -157.1875000013655779, -5.460374474430324690E-16 ) ) ;
#58841=CARTESIAN_POINT ( 'NONE',  ( 5.000000000000000888, -162.9375000000000000, -2.071067811865475505 ) ) ;
#58842=CARTESIAN_POINT ( 'NONE',  ( -6.972266317189433020E-16, -30.12499999726880873, -5.000000000000000000 ) ) ;
#58844=CARTESIAN_POINT ( 'NONE',  ( 2.229367062500001939, -10.22916666530106866, 3.861377020970579999 ) ) ;
#58845=CARTESIAN_POINT ( 'NONE',  ( -4.458734124999999437, -44.64583333196773651, -2.574251347313719407 ) ) ;
#58846=CYLINDRICAL_SURFACE ( 'NONE', #48340, 5.000000000000000000 ) ;
#58847=CARTESIAN_POINT ( 'NONE',  ( -3.152801135295367985, -146.8125000013655779, 3.152801135295367096 ) ) ;
#58849=CARTESIAN_POINT ( 'NONE',  ( 1.975475456537005874E-15, 8.249999999999998224, 5.000000000000000000 ) ) ;
#58852=CARTESIAN_POINT ( 'NONE',  ( 1.975475456537005874E-15, -68.62499999726881583, 5.000000000000000000 ) ) ;
#58860=CARTESIAN_POINT ( 'NONE',  ( -6.972266317189433020E-16, -51.25000000000000000, -5.000000000000000000 ) ) ;
#58861=CARTESIAN_POINT ( 'NONE',  ( -3.152548672688508926E-16, -2.562499998634407028, -5.148502694627439702 ) ) ;
#58863=CARTESIAN_POINT ( 'NONE',  ( 4.458734124999999437, -153.4375000013655779, 0.000000000000000000 ) ) ;
#58865=ORIENTED_EDGE ( 'NONE', *, *, #27013, .F. ) ;
#58867=CARTESIAN_POINT ( 'NONE',  ( -5.000000000000000000, -75.00000000000000000, 0.000000000000000000 ) ) ;
#58871=CARTESIAN_POINT ( 'NONE',  ( 1.975475456537005874E-15, -76.62499999726880162, 5.000000000000000000 ) ) ;
#58872=CARTESIAN_POINT ( 'NONE',  ( 6.972266317189433020E-16, 29.74999999999999645, -5.000000000000000000 ) ) ;
#58878=CARTESIAN_POINT ( 'NONE',  ( 4.458734125000000326, 16.10416666803225993, 2.574251347313718519 ) ) ;
#58880=EDGE_LOOP ( 'NONE', ( #7702, #61575, #19057, #44282 ) ) ;
#58881=CARTESIAN_POINT ( 'NONE',  ( -4.458734124999997661, -8.479166665301073991, 2.574251347313722516 ) ) ;
#58882=CARTESIAN_POINT ( 'NONE',  ( 1.975475456537005874E-15, -30.74999999999999645, 5.000000000000000000 ) ) ;
#58884=CARTESIAN_POINT ( 'NONE',  ( -3.152801135295367985, -168.8125000013656063, 3.152801135295367096 ) ) ;
#58890=EDGE_CURVE ( 'NONE', #25930, #27870, #41755, .T. ) ;
#58891=CARTESIAN_POINT ( 'NONE',  ( 2.071067811865392461, -142.3125000027312410, 5.000000000000084377 ) ) ;
#58892=CARTESIAN_POINT ( 'NONE',  ( 1.339745962155615144, -69.70534180126148271, 4.999999999999999112 ) ) ;
#58894=CARTESIAN_POINT ( 'NONE',  ( -3.152801135295367985, -155.0625000013656063, 3.152801135295367096 ) ) ;
#58898=ORIENTED_EDGE ( 'NONE', *, *, #37056, .T. ) ;
#58901=DIRECTION ( 'NONE',  ( 0.000000000000000000, 0.000000000000000000, 1.000000000000000000 ) ) ;
#58902=CARTESIAN_POINT ( 'NONE',  ( 5.000000000000000888, -2.583333333333333481, 2.886751345948126879 ) ) ;
#58903=EDGE_CURVE ( 'NONE', #15666, #7607, #9428, .T. ) ;
#58904=CARTESIAN_POINT ( 'NONE',  ( 9.457646018065525792E-16, -69.06249999863439371, 5.148502694627439702 ) ) ;
#58905=AXIS2_PLACEMENT_3D ( 'NONE', #23756, #42721, #42405 ) ;
#58907=CARTESIAN_POINT ( 'NONE',  ( -5.000000000000000000, 0.04166666939785235169, -2.886751345948128211 ) ) ;
#58908=CARTESIAN_POINT ( 'NONE',  ( 9.457646018065525792E-16, -32.06249999863440792, 5.148502694627439702 ) ) ;
#58911=DIRECTION ( 'NONE',  ( -0.000000000000000000, 1.000000000000000000, -0.000000000000000000 ) ) ;
#58913=CARTESIAN_POINT ( 'NONE',  ( -4.999999999999999112, -45.91666666666665719, 2.886751345948131764 ) ) ;
#58914=DIRECTION ( 'NONE',  ( 0.000000000000000000, 0.000000000000000000, 1.000000000000000000 ) ) ;
#58916=CARTESIAN_POINT ( 'NONE',  ( -9.184850993605147944E-16, -155.2500000000000000, 5.000000000000000000 ) ) ;
#58917=CARTESIAN_POINT ( 'NONE',  ( -2.229367062500000163, -71.47916666530107932, -3.861377020970580443 ) ) ;
#58918=CARTESIAN_POINT ( 'NONE',  ( -4.458734124999999437, -143.1875000013656063, -5.460374474430324690E-16 ) ) ;
#58919=CARTESIAN_POINT ( 'NONE',  ( -2.229367062499996610, -83.14583333196773651, 3.861377020970582219 ) ) ;
#58921=CARTESIAN_POINT ( 'NONE',  ( 2.229367062499998831, -32.89583333196773651, -3.861377020970580887 ) ) ;
#58922=CARTESIAN_POINT ( 'NONE',  ( -2.500000000000000444, -73.04166666393548724, -4.330127018922193649 ) ) ;
#58924=EDGE_CURVE ( 'NONE', #46451, #34949, #13399, .T. ) ;
#58925=LINE ( 'NONE', #14853, #37172 ) ;
#58926=EDGE_LOOP ( 'NONE', ( #35290, #19208, #30337, #38134 ) ) ;
#58930=ORIENTED_EDGE ( 'NONE', *, *, #9512, .T. ) ;
#58931=CARTESIAN_POINT ( 'NONE',  ( -2.499999999999996447, 17.16666666666666430, 4.330127018922195425 ) ) ;
#58933=CARTESIAN_POINT ( 'NONE',  ( -4.458734124999998549, -59.47916666530106511, 2.574251347313722516 ) ) ;
#58936=( BOUNDED_CURVE ( )  B_SPLINE_CURVE ( 2, ( #61884, #46123, #26185, #11697, #46756, #2087, #31317, #26828, #60930 ),
 .UNSPECIFIED., .F., .F. ) 
 B_SPLINE_CURVE_WITH_KNOTS ( ( 3, 2, 2, 2, 3 ),
 ( 0.5020833333333333259, 0.5027777777777777679, 0.5041666666666666519, 0.5055555555555555358, 0.5062499999999999778 ),
 .UNSPECIFIED. ) 
 CURVE ( )  GEOMETRIC_REPRESENTATION_ITEM ( )  RATIONAL_B_SPLINE_CURVE ( ( 0.9330127018922194093, 0.9330127018922194093, 1.000000000000000000, 0.8660254037844387076, 1.000000000000000000, 0.8660254037844387076, 1.000000000000000000, 0.9330127018922194093, 0.9330127018922194093 ) ) 
 REPRESENTATION_ITEM ( '' )  );
#58938=CARTESIAN_POINT ( 'NONE',  ( -4.999999999999998224, -22.79166666393548013, 2.886751345948131764 ) ) ;
#58939=CARTESIAN_POINT ( 'NONE',  ( 4.458734124999999437, 15.18750000136559564, -5.460374474430324690E-16 ) ) ;
#58941=CARTESIAN_POINT ( 'NONE',  ( -1.846868145590737420, -163.7500000013655779, 4.458734124999997661 ) ) ;
#58944=DIRECTION ( 'NONE',  ( -0.000000000000000000, 1.000000000000000000, -0.000000000000000000 ) ) ;
#58946=EDGE_CURVE ( 'NONE', #14245, #50889, #15084, .T. ) ;
#58948=( BOUNDED_CURVE ( )  B_SPLINE_CURVE ( 2, ( #40116, #40751, #15683, #34659, #35302, #24695, #10849, #16326, #30464 ),
 .UNSPECIFIED., .F., .F. ) 
 B_SPLINE_CURVE_WITH_KNOTS ( ( 3, 2, 2, 2, 3 ),
 ( 0.07500000000000005274, 0.07916666666666671848, 0.08333333333333339810, 0.08750000000000007772, 0.09166666666666674346 ),
 .UNSPECIFIED. ) 
 CURVE ( )  GEOMETRIC_REPRESENTATION_ITEM ( )  RATIONAL_B_SPLINE_CURVE ( ( 0.9999999999999990008, 0.9238795325112877377, 1.000000000000000000, 0.9238795325112867385, 1.000000000000000000, 0.9238795325112867385, 1.000000000000000000, 0.9238795325112851842, 1.000000000000001554 ) ) 
 REPRESENTATION_ITEM ( '' )  );
#58954=CARTESIAN_POINT ( 'NONE',  ( 2.500000000000002220, -20.66666666666666785, 4.330127018922192761 ) ) ;
#58956=CYLINDRICAL_SURFACE ( 'NONE', #49022, 5.000000000000000000 ) ;
#58961=CARTESIAN_POINT ( 'NONE',  ( -2.229367062500000163, 6.270833334698928674, -3.861377020970580443 ) ) ;
#58962=CARTESIAN_POINT ( 'NONE',  ( 3.535533905932738197, -146.0000000027311842, -3.535533905932738197 ) ) ;
#58964=CARTESIAN_POINT ( 'NONE',  ( 2.071067811865475505, -150.9375000027311842, -5.000000000000000888 ) ) ;
#58969=CARTESIAN_POINT ( 'NONE',  ( -5.000000000000000888, -143.5625000000000568, -2.071067811865475949 ) ) ;
#58973=CARTESIAN_POINT ( 'NONE',  ( 2.730187237215162345E-16, -164.4375000013655779, -4.458734124999999437 ) ) ;
#58974=CARTESIAN_POINT ( 'NONE',  ( -4.458734124999999437, -34.31249999863440792, 0.000000000000000000 ) ) ;
#58975=CARTESIAN_POINT ( 'NONE',  ( -2.071067811865372921, -160.3125000000000000, 5.000000000000104805 ) ) ;
#58978=CARTESIAN_POINT ( 'NONE',  ( 4.458734124999999437, -145.5000000013655779, 1.846868145590737864 ) ) ;
#58980=CARTESIAN_POINT ( 'NONE',  ( 1.060575238724906964E-15, -89.62499999726881583, 5.773502691896257311 ) ) ;
#58982=CARTESIAN_POINT ( 'NONE',  ( -4.458734124999997661, -62.47916666530106511, 2.574251347313722516 ) ) ;
#58984=CARTESIAN_POINT ( 'NONE',  ( -2.071067811865548780, -162.6874999999999716, -4.999999999999926281 ) ) ;
#58985=CARTESIAN_POINT ( 'NONE',  ( 5.000000000000000888, 15.41666666666666607, 2.886751345948126879 ) ) ;
#58986=CARTESIAN_POINT ( 'NONE',  ( 9.457646018065525792E-16, -51.06249999863440792, 5.148502694627439702 ) ) ;
#58987=CARTESIAN_POINT ( 'NONE',  ( 4.458734124999998549, -3.729166665301070438, -2.574251347313721627 ) ) ;
#58990=LINE ( 'NONE', #29377, #32286 ) ;
#58992=CARTESIAN_POINT ( 'NONE',  ( 5.000000000000000888, 0.4166666666666659080, 2.886751345948126879 ) ) ;
#58995=CARTESIAN_POINT ( 'NONE',  ( -4.458734124999998549, -54.22916666530107221, 2.574251347313722516 ) ) ;
#58996=CARTESIAN_POINT ( 'NONE',  ( 4.458734125000000326, -155.6250000013656063, -1.846868145590734978 ) ) ;
#58997=VECTOR ( 'NONE', #57903, 1000.000000000000000 ) ;
#58998=CARTESIAN_POINT ( 'NONE',  ( -5.000000000000000000, -52.95833333060214443, -2.886751345948128211 ) ) ;
#58999=ORIENTED_EDGE ( 'NONE', *, *, #17029, .F. ) ;
#59000=CARTESIAN_POINT ( 'NONE',  ( 5.000000000000000000, -26.41666666666666430, -2.886751345948130876 ) ) ;
#59001=CARTESIAN_POINT ( 'NONE',  ( -2.229367062500000163, 7.270833334698929562, -3.861377020970580443 ) ) ;
#59002=ORIENTED_EDGE ( 'NONE', *, *, #6002, .T. ) ;
#59003=CARTESIAN_POINT ( 'NONE',  ( 1.339745962155615144, -56.70534180126148271, 4.999999999999999112 ) ) ;
#59005=CARTESIAN_POINT ( 'NONE',  ( 2.730187237215162345E-16, -155.1875000013655779, -4.458734124999999437 ) ) ;
#59009=CARTESIAN_POINT ( 'NONE',  ( -4.999999999999998224, -58.79166666393546592, 2.886751345948131764 ) ) ;
#59010=CARTESIAN_POINT ( 'NONE',  ( 4.458734125000001214, -41.14583333196774362, 2.574251347313718519 ) ) ;
#59012=CARTESIAN_POINT ( 'NONE',  ( 3.061616997868383141E-16, -145.7500000000000284, -5.000000000000000000 ) ) ;
#59015=ORIENTED_EDGE ( 'NONE', *, *, #61739, .F. ) ;
#59016=CARTESIAN_POINT ( 'NONE',  ( 2.229367062499998831, 29.35416666803225993, -3.861377020970580887 ) ) ;
#59020=DIRECTION ( 'NONE',  ( -0.000000000000000000, 1.000000000000000000, -0.000000000000000000 ) ) ;
#59026=EDGE_CURVE ( 'NONE', #62409, #58377, #36887, .T. ) ;
#59029=CARTESIAN_POINT ( 'NONE',  ( 0.000000000000000000, -170.0000000000000000, 0.000000000000000000 ) ) ;
#59032=ADVANCED_FACE ( 'NONE', ( #4350 ), #5627, .T. ) ;
#59037=CARTESIAN_POINT ( 'NONE',  ( -5.000000000000000888, -163.6875000027311842, -2.071067811865475949 ) ) ;
#59039=CARTESIAN_POINT ( 'NONE',  ( -5.000000000000000000, -161.6250000027311842, -6.123233995736766282E-16 ) ) ;
#59041=CARTESIAN_POINT ( 'NONE',  ( -6.972266317189433020E-16, -19.12499999726880873, -5.000000000000000000 ) ) ;
#59046=AXIS2_PLACEMENT_3D ( 'NONE', #12493, #12178, #27597 ) ;
#59053=CARTESIAN_POINT ( 'NONE',  ( 4.458734124999999437, -16.81249999863440436, -5.460374474430324690E-16 ) ) ;
#59054=CARTESIAN_POINT ( 'NONE',  ( 1.339745962155615144, -71.70534180126148271, 4.999999999999999112 ) ) ;
#59055=CARTESIAN_POINT ( 'NONE',  ( 3.535533905932736864, -153.1250000000000000, 3.535533905932738641 ) ) ;
#59057=EDGE_CURVE ( 'NONE', #8105, #62409, #48406, .T. ) ;
#59059=CARTESIAN_POINT ( 'NONE',  ( -3.152548672688508926E-16, -48.81249999863440792, -5.148502694627439702 ) ) ;
#59061=EDGE_CURVE ( 'NONE', #29588, #1043, #35196, .T. ) ;
#59063=EDGE_CURVE ( 'NONE', #60836, #15263, #54916, .T. ) ;
#59067=CARTESIAN_POINT ( 'NONE',  ( 2.229367062500001939, 10.02083333469892779, 3.861377020970579999 ) ) ;
#59069=CARTESIAN_POINT ( 'NONE',  ( 2.500000000000002220, -37.54166666393548013, 4.330127018922192761 ) ) ;
#59070=CARTESIAN_POINT ( 'NONE',  ( -2.229367062500000163, -86.72916666530107932, -3.861377020970580443 ) ) ;
#59071=CARTESIAN_POINT ( 'NONE',  ( 2.229367062499998831, 20.10416666803225993, -3.861377020970580887 ) ) ;
#59073=CARTESIAN_POINT ( 'NONE',  ( 1.060575238724906964E-15, 7.375000002731186832, 5.773502691896257311 ) ) ;
#59076=EDGE_LOOP ( 'NONE', ( #41367, #52697, #9624, #10515 ) ) ;
#59078=CARTESIAN_POINT ( 'NONE',  ( -3.535250795749689387E-16, -35.25000000000000000, -5.773502691896257311 ) ) ;
#59079=CARTESIAN_POINT ( 'NONE',  ( 4.458734124999998549, -39.72916666530107932, -2.574251347313721627 ) ) ;
#59080=CARTESIAN_POINT ( 'NONE',  ( -2.500000000000000444, -32.04166666393548724, -4.330127018922193649 ) ) ;
#59081=CARTESIAN_POINT ( 'NONE',  ( -3.152548672688508926E-16, -66.56249999863440792, -5.148502694627439702 ) ) ;
#59084=CARTESIAN_POINT ( 'NONE',  ( -2.229367062500000163, -10.47916666530106866, -3.861377020970580443 ) ) ;
#59085=CARTESIAN_POINT ( 'NONE',  ( -4.458734124999998549, -16.47916666530107577, 2.574251347313722516 ) ) ;
#59087=CARTESIAN_POINT ( 'NONE',  ( -5.000000000000000000, -83.99999999999998579, 0.000000000000000000 ) ) ;
#59088=CARTESIAN_POINT ( 'NONE',  ( -4.458734125000001214, -167.8750000013656063, 1.846868145590734089 ) ) ;
#59090=CARTESIAN_POINT ( 'NONE',  ( 5.000000000000000000, -82.37499999726881583, -6.123233995736766282E-16 ) ) ;
#59091=CYLINDRICAL_SURFACE ( 'NONE', #13863, 5.000000000000000000 ) ;
#59092=ORIENTED_EDGE ( 'NONE', *, *, #22922, .F. ) ;
#59094=CARTESIAN_POINT ( 'NONE',  ( -4.458734124999999437, -26.64583333196773651, -2.574251347313719407 ) ) ;
#59098=CARTESIAN_POINT ( 'NONE',  ( -4.458734124999999437, -164.1875000013655779, -5.460374474430324690E-16 ) ) ;
#59100=CARTESIAN_POINT ( 'NONE',  ( -5.000000000000000000, -38.95833333060214443, -2.886751345948128211 ) ) ;
#59103=CARTESIAN_POINT ( 'NONE',  ( -2.229367062500000163, -74.72916666530106511, -3.861377020970580443 ) ) ;
#59106=CARTESIAN_POINT ( 'NONE',  ( 4.458734124999999437, -147.6250000013655779, -1.846868145590734978 ) ) ;
#59112=CARTESIAN_POINT ( 'NONE',  ( -1.846868145590734756, -141.3750000013656063, -4.458734125000000326 ) ) ;
#59117=CARTESIAN_POINT ( 'NONE',  ( -2.229367062499996610, -75.39583333196773651, 3.861377020970582219 ) ) ;
#59118=CARTESIAN_POINT ( 'NONE',  ( -3.535533905932738641, -166.3750000000000284, 3.535533905932737309 ) ) ;
#59119=CARTESIAN_POINT ( 'NONE',  ( -5.000000000000000000, -69.99999999999998579, 0.000000000000000000 ) ) ;
#59122=VERTEX_POINT ( 'NONE', #1142 ) ;
#59124=CARTESIAN_POINT ( 'NONE',  ( 1.255007937094098239E-14, 23.87500000273118417, -4.999999999999999112 ) ) ;
#59129=CARTESIAN_POINT ( 'NONE',  ( 4.458734124999999437, 18.93750000136559564, -5.460374474430324690E-16 ) ) ;
#59135=CARTESIAN_POINT ( 'NONE',  ( -2.500000000000000444, -51.04166666393547303, -4.330127018922193649 ) ) ;
#59136=CARTESIAN_POINT ( 'NONE',  ( 2.229367062500001939, 2.020833334698927786, 3.861377020970579999 ) ) ;
#59138=CARTESIAN_POINT ( 'NONE',  ( 9.457646018065525792E-16, -26.31249999863440792, 5.148502694627439702 ) ) ;
#59142=CARTESIAN_POINT ( 'NONE',  ( -4.458734124999999437, 25.60416666803225993, -2.574251347313719407 ) ) ;
#59146=CARTESIAN_POINT ( 'NONE',  ( 2.229367062500001939, -75.22916666530106511, 3.861377020970579999 ) ) ;
#59149=CARTESIAN_POINT ( 'NONE',  ( -4.999999999999999112, 23.20833333606451632, 2.886751345948131764 ) ) ;
#59151=CARTESIAN_POINT ( 'NONE',  ( -6.972266317189433020E-16, 6.750000000000000000, -5.000000000000000000 ) ) ;
#59152=CARTESIAN_POINT ( 'NONE',  ( -6.972266317189433020E-16, -57.12499999726879452, -5.000000000000000000 ) ) ;
#59153=CARTESIAN_POINT ( 'NONE',  ( -2.500000000000000444, -19.16666666666666430, -4.330127018922193649 ) ) ;
#59154=CARTESIAN_POINT ( 'NONE',  ( -4.458734124999998549, -24.22916666530107577, 2.574251347313722516 ) ) ;
#59155=CARTESIAN_POINT ( 'NONE',  ( -2.229367062500000163, -85.47916666530107932, -3.861377020970580443 ) ) ;
#59156=CARTESIAN_POINT ( 'NONE',  ( 1.846868145590736310, -168.8750000013655779, 4.458734124999999437 ) ) ;
#59157=CARTESIAN_POINT ( 'NONE',  ( -2.499999999999996447, -18.70833333060214798, 4.330127018922195425 ) ) ;
#59158=CARTESIAN_POINT ( 'NONE',  ( -4.458734124999999437, -49.31249999863440792, 0.000000000000000000 ) ) ;
#59159=ORIENTED_EDGE ( 'NONE', *, *, #62275, .F. ) ;
#59162=CARTESIAN_POINT ( 'NONE',  ( 2.229367062500001939, 1.770833334698927786, 3.861377020970579999 ) ) ;
#59165=CARTESIAN_POINT ( 'NONE',  ( -5.000000000000000000, -67.08333333333332860, -2.886751345948128211 ) ) ;
#59166=CARTESIAN_POINT ( 'NONE',  ( 2.730187237215162345E-16, -151.4375000013656063, -4.458734124999999437 ) ) ;
#59169=CARTESIAN_POINT ( 'NONE',  ( -3.535533905932737309, -162.6250000000000284, -3.535533905932738197 ) ) ;
#59170=CARTESIAN_POINT ( 'NONE',  ( -2.499999999999996447, 7.291666669397852019, 4.330127018922195425 ) ) ;
#59172=CARTESIAN_POINT ( 'NONE',  ( -3.152548672688508926E-16, -8.812499998634406140, -5.148502694627439702 ) ) ;
#59173=CARTESIAN_POINT ( 'NONE',  ( 2.229367062500001939, -46.22916666530106511, 3.861377020970579999 ) ) ;
#59175=CARTESIAN_POINT ( 'NONE',  ( 4.458734124999999437, -149.4375000013656063, 0.000000000000000000 ) ) ;
#59177=CARTESIAN_POINT ( 'NONE',  ( -6.972266317189433020E-16, 27.74999999999999645, -5.000000000000000000 ) ) ;
#59180=CARTESIAN_POINT ( 'NONE',  ( -4.458734124999999437, 29.35416666803225993, -2.574251347313719407 ) ) ;
#59182=VECTOR ( 'NONE', #41980, 1000.000000000000000 ) ;
#59184=ORIENTED_EDGE ( 'NONE', *, *, #46516, .F. ) ;
#59187=AXIS2_PLACEMENT_3D ( 'NONE', #59029, #44223, #21073 ) ;
#59190=( BOUNDED_CURVE ( )  B_SPLINE_CURVE ( 2, ( #23893, #43495, #29320, #19053, #24523, #38668, #53472, #9403, #29012 ),
 .UNSPECIFIED., .F., .F. ) 
 B_SPLINE_CURVE_WITH_KNOTS ( ( 3, 2, 2, 2, 3 ),
 ( 0.1250000000000001110, 0.1291666666666667906, 0.1333333333333334425, 0.1375000000000001221, 0.1416666666666667740 ),
 .UNSPECIFIED. ) 
 CURVE ( )  GEOMETRIC_REPRESENTATION_ITEM ( )  RATIONAL_B_SPLINE_CURVE ( ( 0.9999999999999980016, 0.9238795325112887369, 1.000000000000000000, 0.9238795325112867385, 1.000000000000000000, 0.9238795325112867385, 1.000000000000000000, 0.9238795325112847401, 1.000000000000001998 ) ) 
 REPRESENTATION_ITEM ( '' )  );
#59191=CARTESIAN_POINT ( 'NONE',  ( -5.000000000000000000, 8.916666666666666075, -2.886751345948128211 ) ) ;
#59192=CARTESIAN_POINT ( 'NONE',  ( 4.458734124999998549, -0.7291666653010709931, -2.574251347313721627 ) ) ;
#59194=CARTESIAN_POINT ( 'NONE',  ( 1.846868145590736310, -150.6250000013655779, 4.458734124999997661 ) ) ;
#59202=CARTESIAN_POINT ( 'NONE',  ( 2.788906526875773208E-15, 27.87500000273118417, -5.000000000000000000 ) ) ;
#59203=CARTESIAN_POINT ( 'NONE',  ( -2.499999999999996447, -12.83333333333333570, 4.330127018922195425 ) ) ;
#59207=FACE_OUTER_BOUND ( 'NONE', #32666, .T. ) ;
#59209=CARTESIAN_POINT ( 'NONE',  ( -2.229367062499996610, 16.85416666803225993, 3.861377020970582219 ) ) ;
#59212=CARTESIAN_POINT ( 'NONE',  ( 2.229367062500001939, -8.229166665301073991, 3.861377020970579999 ) ) ;
#59214=CARTESIAN_POINT ( 'NONE',  ( 3.152801135295367541, -168.3125000013656063, -3.152801135295367541 ) ) ;
#59220=LINE ( 'NONE', #15794, #2869 ) ;
#59221=CARTESIAN_POINT ( 'NONE',  ( 1.846868145590735200, -155.5000000013656063, -4.458734124999999437 ) ) ;
#59223=CARTESIAN_POINT ( 'NONE',  ( -6.972266317189433020E-16, 0.8750000027311866102, -5.000000000000000000 ) ) ;
#59225=VERTEX_POINT ( 'NONE', #22013 ) ;
#59228=CARTESIAN_POINT ( 'NONE',  ( -5.000000000000000000, -3.083333333333333925, -2.886751345948128211 ) ) ;
#59230=CARTESIAN_POINT ( 'NONE',  ( 4.458734124999998549, -68.72916666530107932, -2.574251347313721627 ) ) ;
#59231=CARTESIAN_POINT ( 'NONE',  ( -4.999999999999999112, 0.2083333360645180099, 2.886751345948131764 ) ) ;
#59232=CARTESIAN_POINT ( 'NONE',  ( -3.152548672688508926E-16, -31.56249999863440436, -5.148502694627439702 ) ) ;
#59233=ORIENTED_EDGE ( 'NONE', *, *, #40356, .F. ) ;
#59234=CARTESIAN_POINT ( 'NONE',  ( 5.000000000000000000, -153.1250000027312126, 0.000000000000000000 ) ) ;
#59235=CARTESIAN_POINT ( 'NONE',  ( 1.975475456537005874E-15, -47.62499999726880873, 5.000000000000000000 ) ) ;
#59238=CARTESIAN_POINT ( 'NONE',  ( -5.000000000000000000, -48.00000000000000000, 0.000000000000000000 ) ) ;
#59239=CARTESIAN_POINT ( 'NONE',  ( 1.339745962155615144, -26.58034179853029855, 4.999999999999999112 ) ) ;
#59241=CARTESIAN_POINT ( 'NONE',  ( -5.000000000000000000, -3.999999999999996447, 0.000000000000000000 ) ) ;
#59242=CARTESIAN_POINT ( 'NONE',  ( -2.229367062499996610, -69.14583333196773651, 3.861377020970582219 ) ) ;
#59244=CARTESIAN_POINT ( 'NONE',  ( 4.458734125000000326, -142.6250000013655779, -1.846868145590734978 ) ) ;
#59245=CARTESIAN_POINT ( 'NONE',  ( -3.152548672688508926E-16, -83.56249999863440792, -5.148502694627439702 ) ) ;
#59246=EDGE_CURVE ( 'NONE', #1843, #41941, #17552, .T. ) ;
#59248=CARTESIAN_POINT ( 'NONE',  ( 4.458734124999998549, -27.97916666530107577, -2.574251347313721627 ) ) ;
#59249=CARTESIAN_POINT ( 'NONE',  ( -2.499999999999996447, -72.70833333060214443, 4.330127018922195425 ) ) ;
#59252=ORIENTED_EDGE ( 'NONE', *, *, #25938, .F. ) ;
#59259=CARTESIAN_POINT ( 'NONE',  ( -2.229367062500000163, -57.72916666530107932, -3.861377020970580443 ) ) ;
#59262=CARTESIAN_POINT ( 'NONE',  ( -9.184850993605147944E-16, -146.2500000000000284, 5.000000000000000000 ) ) ;
#59263=FACE_OUTER_BOUND ( 'NONE', #63038, .T. ) ;
#59264=CARTESIAN_POINT ( 'NONE',  ( -4.458734124999999437, 11.68750000136559564, 0.000000000000000000 ) ) ;
#59266=CARTESIAN_POINT ( 'NONE',  ( 2.499999999999998668, -32.33333333333332860, -4.330127018922193649 ) ) ;
#59267=CARTESIAN_POINT ( 'NONE',  ( 4.458734124999999437, -162.4375000013655779, 0.000000000000000000 ) ) ;
#59272=CIRCLE ( 'NONE', #15106, 5.000000000000000000 ) ;
#59274=CARTESIAN_POINT ( 'NONE',  ( -5.000000000000000000, 1.999999999999998224, 0.000000000000000000 ) ) ;
#59277=CARTESIAN_POINT ( 'NONE',  ( -1.339745962155613812, -29.20534180126147916, -5.000000000000000000 ) ) ;
#59283=CARTESIAN_POINT ( 'NONE',  ( -4.458734124999999437, 9.354166668032261711, -2.574251347313719407 ) ) ;
#59284=CARTESIAN_POINT ( 'NONE',  ( -2.499999999999996447, -9.708333330602146205, 4.330127018922195425 ) ) ;
#59286=CARTESIAN_POINT ( 'NONE',  ( 3.535533905932736864, -149.2500000027311842, 3.535533905932738641 ) ) ;
#59291=CARTESIAN_POINT ( 'NONE',  ( 5.000000000000000000, -140.0625000000000000, 2.071067811865478614 ) ) ;
#59292=CARTESIAN_POINT ( 'NONE',  ( 2.071067811865392461, -141.3125000027312410, 5.000000000000084377 ) ) ;
#59294=CARTESIAN_POINT ( 'NONE',  ( -4.458734125000000326, -167.1250000013656063, 1.846868145590734089 ) ) ;
#59295=CARTESIAN_POINT ( 'NONE',  ( -5.000000000000000888, -160.5625000000000284, -2.071067811865475949 ) ) ;
#59296=CARTESIAN_POINT ( 'NONE',  ( 1.975475456537005874E-15, -45.62499999726880873, 5.000000000000000000 ) ) ;
#59298=CARTESIAN_POINT ( 'NONE',  ( -3.152801135295367985, -144.8125000013655779, 3.152801135295367096 ) ) ;
#59299=ORIENTED_EDGE ( 'NONE', *, *, #45025, .T. ) ;
#59300=CARTESIAN_POINT ( 'NONE',  ( -2.229367062500000163, 28.27083333469892779, -3.861377020970580443 ) ) ;
#59302=CARTESIAN_POINT ( 'NONE',  ( -2.229367062500000163, -61.72916666530106511, -3.861377020970580443 ) ) ;
#59304=CARTESIAN_POINT ( 'NONE',  ( 5.000000000000000000, 13.62500000273118417, -6.123233995736766282E-16 ) ) ;
#59305=CARTESIAN_POINT ( 'NONE',  ( -3.535250795749689387E-16, 14.75000000000000000, -5.773502691896257311 ) ) ;
#59306=CARTESIAN_POINT ( 'NONE',  ( -2.229367062500000163, -50.47916666530107221, -3.861377020970580443 ) ) ;
#59307=CARTESIAN_POINT ( 'NONE',  ( 9.457646018065525792E-16, -6.062499998634403475, 5.148502694627439702 ) ) ;
#59310=CARTESIAN_POINT ( 'NONE',  ( 1.975475456537005874E-15, 13.37500000273118417, 5.000000000000000000 ) ) ;
#59312=CARTESIAN_POINT ( 'NONE',  ( -1.339745962155610925, -58.79465819873852439, 5.000000000000000000 ) ) ;
#59316=CARTESIAN_POINT ( 'NONE',  ( 9.457646018065525792E-16, -55.06249999863439371, 5.148502694627439702 ) ) ;
#59317=CARTESIAN_POINT ( 'NONE',  ( 3.152801135295367541, -154.5625000013656063, -3.152801135295367541 ) ) ;
#59320=( BOUNDED_CURVE ( )  B_SPLINE_CURVE ( 2, ( #49827, #25389, #58535, #19605, #39851, #53703, #976, #9635, #59494 ),
 .UNSPECIFIED., .F., .F. ) 
 B_SPLINE_CURVE_WITH_KNOTS ( ( 3, 2, 2, 2, 3 ),
 ( 0.1562500000000000000, 0.1569444444444444420, 0.1583333333333333259, 0.1597222222222222099, 0.1604166666666666796 ),
 .UNSPECIFIED. ) 
 CURVE ( )  GEOMETRIC_REPRESENTATION_ITEM ( )  RATIONAL_B_SPLINE_CURVE ( ( 0.9330127018922194093, 0.9330127018922194093, 1.000000000000000000, 0.8660254037844387076, 1.000000000000000000, 0.8660254037844387076, 1.000000000000000000, 0.9330127018922180770, 0.9330127018922194093 ) ) 
 REPRESENTATION_ITEM ( '' )  );
#59321=CARTESIAN_POINT ( 'NONE',  ( 5.000000000000000000, -55.29166666393548013, -2.886751345948129988 ) ) ;
#59322=ORIENTED_EDGE ( 'NONE', *, *, #6329, .T. ) ;
#59323=CARTESIAN_POINT ( 'NONE',  ( -1.339745962155610925, -48.79465819873850307, 5.000000000000000000 ) ) ;
#59324=CARTESIAN_POINT ( 'NONE',  ( -4.458734124999999437, 4.354166668032260823, -2.574251347313719407 ) ) ;
#59328=CARTESIAN_POINT ( 'NONE',  ( 1.846868145590736310, -155.6250000013656063, 4.458734124999999437 ) ) ;
#59334=CARTESIAN_POINT ( 'NONE',  ( -4.458734124999999437, -43.64583333196774362, -2.574251347313719407 ) ) ;
#59335=ORIENTED_EDGE ( 'NONE', *, *, #46043, .T. ) ;
#59336=( BOUNDED_SURFACE ( )  B_SPLINE_SURFACE ( 1, 2, ( 
 ( #53689, #38570, #9621, #48544, #18954, #23797, #24740, #19591, #43089, #24422, #14128, #30761, #35591, #59156, #24112, #33442, #29229, #53059, #33755, #23487, #9307, #4483, #28609, #34066, #50382, #62730, #53372, #39202, #58201, #48855, #28921, #44343, #57899, #43710, #4798, #39519, #54003, #63354, #58827, #49182, #19270, #14444, #13823, #8999, #48226, #38886, #15089, #58520, #44024, #63671, #14757, #306, #4183, #19904, #43399, #63044, #34375, #9932, #29548, #11765, #25933, #51348, #36537, #2460, #32350, #46517, #6328, #41994, #35912, #60367, #56494, #26576, #36864, #51022, #21114, #16920, #45552, #1834, #7287, #31384, #16607, #11454, #22071, #12092, #61634, #32027, #6966, #46194, #12415, #27209, #21435, #26898, #2155, #31714, #60686, #37185, #2772, #41663, #61315, #17240, #56810, #26248, #46827, #51663, #17567, #55543, #45870, #36225, #1511, #40719, #7603, #12727, #22393, #16291, #21761, #31073, #50697, #6640, #41039, #55849, #41355, #60998, #56169, #3719, #58049, #18186, #19111, #13360, #62582, #27517, #8848, #32663, #62886, #28462, #48077, #13045, #8228, #13979, #32983, #52603, #18799, #9158, #47455, #52911, #8537, #57749, #42626, #38730, #48392, #4032, #23650, #33292, #58368, #27833, #28772, #13673, #23951, #17869, #3407, #62265, #47147, #3095, #43246, #43555, #38423, #51973, #28147, #63201, #33607, #53227, #7912, #52291, #4334, #14296, #22712, #23337, #42310, #37812, #61950, #47764, #18504, #37490, #57130, #23023, #57440, #42940, #38125, #58680, #53848, #9777, #40002, #29383, #34531, #24587, #49017, #40331, #43867, #25222, #4965, #54816, #796, #44193, #59649, #158, #25540, #49980, #4640, #15582, #5932, #20075, #19754, #10747, #24263, #39365, #15252, #45157, #20403, #54164, #49666, #35201, #10105, #24908, #20727, #29075, #1123, #58996, #59973, #14925, #29713, #49344, #5606, #30356, #33915, #53540, #63515, #9466, #5290, #44511, #473, #39681, #48700, #34878, #59317, #30037, #19439, #10424, #39051, #14607, #34222, #54499, #44833, #36154, #46439, #60612, #30686, #26501, #41915, #11377, #16843, #40964, #26179, #21043, #31640, #21685, #51585, #46116, #15894, #27134, #6564, #51275, #30998, #6887, #56091, #1441, #56419, #11062, #50303, #50946, #12342, #40650, #31953, #1758, #2385, #36786, #60289, #21995, #16529, #2079, #35514, #45798, #55774, #12011, #7523, #46749, #36464, #16213, #7208, #55461, #45477, #35839, #11691, #50625, #21360, #41274, #2694, #31310, #60924, #22314, #55135, #61240, #41588, #26819, #17162, #6251, #25861, #38046, #17492, #62814, #18732, #57363, #37113, #43174, #42548, #38357, #57983, #56732, #12963, #12652, #32267, #37418, #13908, #32910, #7837, #18108, #9087, #61878, #33536, #28075, #32588, #47692, #22952, #57052, #17794, #53151, #57678, #51896, #37730, #8158, #52211, #27757, #33222, #62187, #47385, #3336, #42235, #27438, #28696, #13284, #48004, #52533, #42863, #47072, #8467, #3644, #23255, #23883, #61558, #3021, #22637, #23578, #62508, #18425, #13605, #48315, #52841, #4265, #8775, #28385, #3957, #44436, #34151, #10664, #54744, #15507, #44115, #53463, #49275, #9392, #53773, #43486, #29310, #24513, #48628, #9705, #38974, #48942, #15175, #4890, #14531, #79, #24191, #38659, #25143, #19679, #29961, #43798, #24830, #63131, #58611, #63445, #19362, #5854, #19042, #58298, #33844, #5528, #14217, #29003, #4568, #35128, #39291, #30280, #397, #49900, #58918, #19999, #14847, #34459, #54090, #10029, #29641, #5211, #39607, #59244, #34800, #54423, #10352, #49586, #44754, #715, #20325, #39927, #59574, #41201, #20971, #16456, #2002, #10984, #2315, #20656, #40260, #60532, #21918, #50227, #41515, #11300, #56020, #46361, #6175, #31564, #50551, #36075, #51513, #55383, #6495, #21606, #61168, #17091, #46038, #30604, #60845, #1369, #55060, #45403, #21280, #40572, #60213, #31238, #36713, #25792, #16137 ),
 ( #7129, #26106, #56345, #26745, #1050, #35759, #59900, #15821, #30924, #12266, #55704, #35434, #45727, #31879, #1678, #25462, #11618, #40887, #50869, #6814, #26421, #16771, #45084, #36389, #11934, #51197, #13533, #37338, #38286, #32508, #18029, #46676, #27997, #51819, #18350, #47616, #3569, #32189, #27364, #46998, #33153, #2946, #8082, #61797, #22561, #13834, #17417, #62432, #42161, #28308, #37974, #17723, #52767, #56972, #62742, #23499, #41839, #8696, #43102, #57294, #12889, #47924, #61485, #52140, #52461, #18664, #57606, #27685, #23177, #3880, #47311, #62110, #57912, #2621, #33454, #3264, #7450, #22876, #42469, #37651, #42788, #27058, #22239, #37032, #56658, #12575, #13210, #32832, #8396, #7761, #9011, #34389, #19604, #49195, #15429, #29562, #53071, #25068, #18967, #43412, #39531, #9634, #19917, #34079, #4196, #1, #28623, #48556, #54015, #14457, #63368, #58213, #5134, #58841, #44678, #15101, #53702, #29242, #59169, #10276, #4495, #9947, #48867, #14770, #43723, #20248, #49511, #24751, #44356, #319, #39850, #9319, #29882, #34718, #639, #38582, #28933, #19284, #48239, #23809, #54345, #59493, #5450, #63055, #4812, #14141, #33767, #53387, #24123, #38899, #58533, #24435, #44037, #39216, #1924, #49826, #31164, #21529, #30852, #54980, #26341, #5770, #10909, #26032, #41125, #55632, #20893, #40809, #50795, #40495, #55314, #36317, #10585, #60773, #30524, #16698, #50147, #35358, #60136, #60457, #6732, #55942, #45960, #25388, #35050, #16057, #6102, #25716, #1295, #54662, #21203, #45647, #36002, #30197, #45009, #975, #20577, #45327, #35686, #40184, #1605, #59821, #16383, #11228, #11547, #15742, #50482, #6421, #53903, #39105, #33973, #44567, #34592, #856, #54551, #9829, #29440, #59374, #49717, #24317, #29766, #49072, #54223, #19490, #59701, #25275, #49400, #24962, #10161, #15633, #48753, #5662, #5344, #20459, #58424, #4695, #58733, #24007, #43610, #525, #40058, #15308, #28827, #5020, #35249, #10474, #39734, #48448, #53593, #20134, #34930, #44896, #44246, #30087, #14659, #54869, #24639, #39417, #4388, #63252, #9523, #19168, #38785, #14351, #29130, #43924, #63571, #34278, #210, #19808, #59055, #14983, #17215, #20778, #2134, #25912, #31692, #41332, #50360, #36516, #30739, #2439, #46491, #40383, #1178, #60979, #31052, #16900, #55520, #25599, #21416, #36842, #6308, #11743, #35890, #21094, #15947, #26553, #16586, #22048, #56146, #11434, #50675, #12067, #51327, #45530, #31361, #6617, #36206, #1491, #41641, #7265, #51002, #6942, #55828, #61293, #40698, #26877, #46173, #10800, #60024, #60343, #16271, #5994, #45212, #21737, #30412, #50036, #35569, #26230, #55193, #11113, #45850, #1812, #41019, #60662, #31686, #32955, #42600, #60973, #51321, #3381, #3695, #41326, #16893, #13334, #7569, #52580, #61923, #28121, #36510, #42284, #32002, #8511, #47738, #56141, #41964, #7259, #47119, #26872, #51636, #12061, #27182, #22364, #46484, #51946, #2432, #22042, #46798, #57097, #36836, #32315, #17843, #41634, #18154, #61287, #17209, #12702, #37783, #56466, #57414, #2744, #8202, #62237, #12388, #47430, #61606, #7886, #17540, #37159, #56783, #37466, #27489, #3067, #13016, #22684, #32635, #52264, #27805, #22998, #19086, #62862, #58025, #29050, #44165, #28438, #23626, #19727, #42908, #18775, #24239, #43531, #48674, #13954, #54137, #39336, #43843, #19413, #4614, #10076, #43222, #133, #63489, #58969, #52888, #38402, #33580, #18477, #38098, #39028, #14897, #9751, #23308, #23929, #34506, #48991, #34198, #62557, #48052, #53200, #49318, #9134, #57723, #29358, #28740, #29688, #48367, #33890, #13649, #58655, #4004, #53822, #14575, #4938, #4310, #63175, #38705, #24561, #58342, #14271, #53510, #9440, #33269, #8823, #60265, #20376, #26151, #35808, #44806, #30972, #25190, #60580, #21332, #39654, #50597, #40932, #55108, #39977, #45770, #59291, #59622 ) ),
 .UNSPECIFIED., .F., .F., .F. ) 
 B_SPLINE_SURFACE_WITH_KNOTS ( ( 2, 2 ),
 ( 3, 2, 2, 2, 2, 2, 2, 2, 2, 2, 2, 2, 2, 2, 2, 2, 2, 2, 2, 2, 2, 2, 2, 2, 2, 2, 2, 2, 2, 2, 2, 2, 2, 2, 2, 2, 2, 2, 2, 2, 2, 2, 2, 2, 2, 2, 2, 2, 2, 2, 2, 2, 2, 2, 2, 2, 2, 2, 2, 2, 2, 2, 2, 2, 2, 2, 2, 2, 2, 2, 2, 2, 2, 2, 2, 2, 2, 2, 2, 2, 2, 2, 2, 2, 2, 2, 2, 2, 2, 2, 2, 2, 2, 2, 2, 2, 2, 2, 2, 2, 2, 2, 2, 2, 2, 2, 2, 2, 2, 2, 2, 2, 2, 2, 2, 2, 2, 2, 2, 2, 2, 2, 2, 2, 2, 2, 2, 2, 2, 2, 2, 2, 2, 2, 2, 2, 2, 2, 2, 2, 2, 2, 2, 2, 2, 2, 2, 2, 2, 2, 2, 2, 2, 2, 2, 2, 2, 2, 2, 2, 2, 2, 2, 2, 2, 2, 2, 2, 2, 2, 2, 2, 2, 2, 2, 2, 2, 2, 2, 2, 2, 2, 2, 2, 2, 2, 2, 2, 2, 2, 2, 2, 2, 2, 2, 2, 2, 2, 2, 2, 2, 2, 2, 2, 2, 2, 2, 2, 2, 2, 2, 2, 2, 2, 2, 2, 2, 2, 2, 2, 2, 2, 2, 2, 2, 2, 2, 2, 2, 2, 2, 2, 2, 2, 2, 2, 2, 2, 2, 2, 3 ),
 ( 0.000000000000000000, 1.000000000000000000 ),
 ( 0.000000000000000000, 0.004166666666666666609, 0.008333333333333333218, 0.01250000000000000069, 0.01666666666666666644, 0.02083333333333333218, 0.02500000000000000139, 0.02916666666666666713, 0.03333333333333333287, 0.03749999999999999861, 0.04166666666666666435, 0.04583333333333333010, 0.05000000000000000278, 0.05416666666666666852, 0.05833333333333333426, 0.06250000000000000000, 0.06666666666666666574, 0.07083333333333333148, 0.07499999999999999722, 0.07916666666666666297, 0.08333333333333332871, 0.08749999999999999445, 0.09166666666666666019, 0.09583333333333333981, 0.1000000000000000056, 0.1041666666666666713, 0.1083333333333333370, 0.1125000000000000028, 0.1166666666666666685, 0.1208333333333333343, 0.1250000000000000000, 0.1291666666666666796, 0.1333333333333333315, 0.1375000000000000111, 0.1416666666666666630, 0.1458333333333333426, 0.1499999999999999944, 0.1541666666666666741, 0.1583333333333333259, 0.1625000000000000056, 0.1666666666666666574, 0.1708333333333333370, 0.1749999999999999889, 0.1791666666666666685, 0.1833333333333333204, 0.1875000000000000000, 0.1916666666666666796, 0.1958333333333333315, 0.2000000000000000111, 0.2041666666666666630, 0.2083333333333333426, 0.2124999999999999944, 0.2166666666666666741, 0.2208333333333333259, 0.2250000000000000056, 0.2291666666666666574, 0.2333333333333333370, 0.2374999999999999889, 0.2416666666666666685, 0.2458333333333333204, 0.2500000000000000000, 0.2541666666666666519, 0.2583333333333333592, 0.2625000000000000111, 0.2666666666666666630, 0.2708333333333333148, 0.2750000000000000222, 0.2791666666666666741, 0.2833333333333333259, 0.2874999999999999778, 0.2916666666666666852, 0.2958333333333333370, 0.2999999999999999889, 0.3041666666666666408, 0.3083333333333333481, 0.3125000000000000000, 0.3166666666666666519, 0.3208333333333333592, 0.3250000000000000111, 0.3291666666666666630, 0.3333333333333333148, 0.3375000000000000222, 0.3416666666666666741, 0.3458333333333333259, 0.3499999999999999778, 0.3541666666666666852, 0.3583333333333333370, 0.3624999999999999889, 0.3666666666666666408, 0.3708333333333333481, 0.3750000000000000000, 0.3791666666666666519, 0.3833333333333333592, 0.3875000000000000111, 0.3916666666666666630, 0.3958333333333333148, 0.4000000000000000222, 0.4041666666666666741, 0.4083333333333333259, 0.4124999999999999778, 0.4166666666666666852, 0.4208333333333333370, 0.4249999999999999889, 0.4291666666666666408, 0.4333333333333333481, 0.4375000000000000000, 0.4416666666666666519, 0.4458333333333333592, 0.4500000000000000111, 0.4541666666666666630, 0.4583333333333333148, 0.4625000000000000222, 0.4666666666666666741, 0.4708333333333333259, 0.4749999999999999778, 0.4791666666666666852, 0.4833333333333333370, 0.4874999999999999889, 0.4916666666666666408, 0.4958333333333333481, 0.5000000000000000000, 0.5041666666666666519, 0.5083333333333333037, 0.5124999999999999556, 0.5166666666666667185, 0.5208333333333333703, 0.5250000000000000222, 0.5291666666666666741, 0.5333333333333333259, 0.5374999999999999778, 0.5416666666666666297, 0.5458333333333332815, 0.5500000000000000444, 0.5541666666666666963, 0.5583333333333333481, 0.5625000000000000000, 0.5666666666666666519, 0.5708333333333333037, 0.5749999999999999556, 0.5791666666666667185, 0.5833333333333333703, 0.5875000000000000222, 0.5916666666666666741, 0.5958333333333333259, 0.5999999999999999778, 0.6041666666666666297, 0.6083333333333332815, 0.6125000000000000444, 0.6166666666666666963, 0.6208333333333333481, 0.6250000000000000000, 0.6291666666666666519, 0.6333333333333333037, 0.6374999999999999556, 0.6416666666666667185, 0.6458333333333333703, 0.6500000000000000222, 0.6541666666666666741, 0.6583333333333333259, 0.6624999999999999778, 0.6666666666666666297, 0.6708333333333332815, 0.6750000000000000444, 0.6791666666666666963, 0.6833333333333333481, 0.6875000000000000000, 0.6916666666666666519, 0.6958333333333333037, 0.6999999999999999556, 0.7041666666666667185, 0.7083333333333333703, 0.7125000000000000222, 0.7166666666666666741, 0.7208333333333333259, 0.7249999999999999778, 0.7291666666666666297, 0.7333333333333332815, 0.7375000000000000444, 0.7416666666666666963, 0.7458333333333333481, 0.7500000000000000000, 0.7541666666666666519, 0.7583333333333333037, 0.7624999999999999556, 0.7666666666666667185, 0.7708333333333333703, 0.7750000000000000222, 0.7791666666666666741, 0.7833333333333333259, 0.7874999999999999778, 0.7916666666666666297, 0.7958333333333332815, 0.8000000000000000444, 0.8041666666666666963, 0.8083333333333333481, 0.8125000000000000000, 0.8166666666666666519, 0.8208333333333333037, 0.8249999999999999556, 0.8291666666666667185, 0.8333333333333333703, 0.8375000000000000222, 0.8416666666666666741, 0.8458333333333333259, 0.8499999999999999778, 0.8541666666666666297, 0.8583333333333332815, 0.8625000000000000444, 0.8666666666666666963, 0.8708333333333333481, 0.8750000000000000000, 0.8791666666666666519, 0.8833333333333333037, 0.8874999999999999556, 0.8916666666666667185, 0.8958333333333333703, 0.9000000000000000222, 0.9041666666666666741, 0.9083333333333333259, 0.9124999999999999778, 0.9166666666666666297, 0.9208333333333332815, 0.9250000000000000444, 0.9291666666666666963, 0.9333333333333333481, 0.9375000000000000000, 0.9416666666666666519, 0.9458333333333333037, 0.9499999999999999556, 0.9541666666666667185, 0.9583333333333333703, 0.9625000000000000222, 0.9666666666666666741, 0.9708333333333333259, 0.9749999999999999778, 0.9791666666666666297, 0.9833333333333332815, 0.9875000000000000444, 0.9916666666666666963, 0.9958333333333333481, 1.000000000000000000 ),
 .UNSPECIFIED. ) 
 GEOMETRIC_REPRESENTATION_ITEM ( )  RATIONAL_B_SPLINE_SURFACE ( (
 ( 1.000000000000000000, 0.9238795325112867385, 1.000000000000000000, 0.9238795325112867385, 1.000000000000000000, 0.9238795325112867385, 1.000000000000000000, 0.9238795325112867385, 1.000000000000000000, 0.9238795325112867385, 1.000000000000000000, 0.9238795325112867385, 1.000000000000000000, 0.9238795325112867385, 1.000000000000000000, 0.9238795325112867385, 1.000000000000000000, 0.9238795325112867385, 1.000000000000000000, 0.9238795325112867385, 1.000000000000000000, 0.9238795325112867385, 1.000000000000000000, 0.9238795325112867385, 1.000000000000000000, 0.9238795325112867385, 1.000000000000000000, 0.9238795325112867385, 1.000000000000000000, 0.9238795325112867385, 1.000000000000000000, 0.9238795325112867385, 1.000000000000000000, 0.9238795325112867385, 1.000000000000000000, 0.9238795325112867385, 1.000000000000000000, 0.9238795325112867385, 1.000000000000000000, 0.9238795325112867385, 1.000000000000000000, 0.9238795325112867385, 1.000000000000000000, 0.9238795325112867385, 1.000000000000000000, 0.9238795325112867385, 1.000000000000000000, 0.9238795325112867385, 1.000000000000000000, 0.9238795325112867385, 1.000000000000000000, 0.9238795325112867385, 1.000000000000000000, 0.9238795325112867385, 1.000000000000000000, 0.9238795325112867385, 1.000000000000000000, 0.9238795325112867385, 1.000000000000000000, 0.9238795325112867385, 1.000000000000000000, 0.9238795325112867385, 1.000000000000000000, 0.9238795325112867385, 1.000000000000000000, 0.9238795325112867385, 1.000000000000000000, 0.9238795325112867385, 1.000000000000000000, 0.9238795325112867385, 1.000000000000000000, 0.9238795325112867385, 1.000000000000000000, 0.9238795325112867385, 1.000000000000000000, 0.9238795325112867385, 1.000000000000000000, 0.9238795325112867385, 1.000000000000000000, 0.9238795325112867385, 1.000000000000000000, 0.9238795325112867385, 1.000000000000000000, 0.9238795325112867385, 1.000000000000000000, 0.9238795325112867385, 1.000000000000000000, 0.9238795325112867385, 1.000000000000000000, 0.9238795325112867385, 1.000000000000000000, 0.9238795325112867385, 1.000000000000000000, 0.9238795325112867385, 1.000000000000000000, 0.9238795325112867385, 1.000000000000000000, 0.9238795325112867385, 1.000000000000000000, 0.9238795325112867385, 1.000000000000000000, 0.9238795325112867385, 1.000000000000000000, 0.9238795325112867385, 1.000000000000000000, 0.9238795325112867385, 1.000000000000000000, 0.9238795325112867385, 1.000000000000000000, 0.9238795325112867385, 1.000000000000000000, 0.9238795325112867385, 1.000000000000000000, 0.9238795325112867385, 1.000000000000000000, 0.9238795325112867385, 1.000000000000000000, 0.9238795325112867385, 1.000000000000000000, 0.9238795325112867385, 1.000000000000000000, 0.9238795325112867385, 1.000000000000000000, 0.9238795325112867385, 1.000000000000000000, 0.9238795325112867385, 1.000000000000000000, 0.9238795325112867385, 1.000000000000000000, 0.9238795325112867385, 1.000000000000000000, 0.9238795325112867385, 1.000000000000000000, 0.9238795325112867385, 1.000000000000000000, 0.9238795325112867385, 1.000000000000000000, 0.9238795325112867385, 1.000000000000000000, 0.9238795325112867385, 1.000000000000000000, 0.9238795325112867385, 1.000000000000000000, 0.9238795325112867385, 1.000000000000000000, 0.9238795325112867385, 1.000000000000000000, 0.9238795325112867385, 1.000000000000000000, 0.9238795325112867385, 1.000000000000000000, 0.9238795325112867385, 1.000000000000000000, 0.9238795325112867385, 1.000000000000000000, 0.9238795325112867385, 1.000000000000000000, 0.9238795325112867385, 1.000000000000000000, 0.9238795325112867385, 1.000000000000000000, 0.9238795325112867385, 1.000000000000000000, 0.9238795325112867385, 1.000000000000000000, 0.9238795325112867385, 1.000000000000000000, 0.9238795325112867385, 1.000000000000000000, 0.9238795325112867385, 1.000000000000000000, 0.9238795325112867385, 1.000000000000000000, 0.9238795325112867385, 1.000000000000000000, 0.9238795325112867385, 1.000000000000000000, 0.9238795325112867385, 1.000000000000000000, 0.9238795325112867385, 1.000000000000000000, 0.9238795325112867385, 1.000000000000000000, 0.9238795325112867385, 1.000000000000000000, 0.9238795325112867385, 1.000000000000000000, 0.9238795325112867385, 1.000000000000000000, 0.9238795325112867385, 1.000000000000000000, 0.9238795325112867385, 1.000000000000000000, 0.9238795325112867385, 1.000000000000000000, 0.9238795325112867385, 1.000000000000000000, 0.9238795325112867385, 1.000000000000000000, 0.9238795325112867385, 1.000000000000000000, 0.9238795325112867385, 1.000000000000000000, 0.9238795325112867385, 1.000000000000000000, 0.9238795325112867385, 1.000000000000000000, 0.9238795325112867385, 1.000000000000000000, 0.9238795325112867385, 1.000000000000000000, 0.9238795325112867385, 1.000000000000000000, 0.9238795325112867385, 1.000000000000000000, 0.9238795325112867385, 1.000000000000000000, 0.9238795325112867385, 1.000000000000000000, 0.9238795325112867385, 1.000000000000000000, 0.9238795325112867385, 1.000000000000000000, 0.9238795325112867385, 1.000000000000000000, 0.9238795325112867385, 1.000000000000000000, 0.9238795325112867385, 1.000000000000000000, 0.9238795325112867385, 1.000000000000000000, 0.9238795325112867385, 1.000000000000000000, 0.9238795325112867385, 1.000000000000000000, 0.9238795325112867385, 1.000000000000000000, 0.9238795325112867385, 1.000000000000000000, 0.9238795325112867385, 1.000000000000000000, 0.9238795325112867385, 1.000000000000000000, 0.9238795325112867385, 1.000000000000000000, 0.9238795325112867385, 1.000000000000000000, 0.9238795325112867385, 1.000000000000000000, 0.9238795325112867385, 1.000000000000000000, 0.9238795325112867385, 1.000000000000000000, 0.9238795325112867385, 1.000000000000000000, 0.9238795325112867385, 1.000000000000000000, 0.9238795325112867385, 1.000000000000000000, 0.9238795325112867385, 1.000000000000000000, 0.9238795325112867385, 1.000000000000000000, 0.9238795325112867385, 1.000000000000000000, 0.9238795325112867385, 1.000000000000000000, 0.9238795325112867385, 1.000000000000000000, 0.9238795325112867385, 1.000000000000000000, 0.9238795325112867385, 1.000000000000000000, 0.9238795325112867385, 1.000000000000000000, 0.9238795325112867385, 1.000000000000000000, 0.9238795325112867385, 1.000000000000000000, 0.9238795325112867385, 1.000000000000000000, 0.9238795325112867385, 1.000000000000000000, 0.9238795325112867385, 1.000000000000000000, 0.9238795325112867385, 1.000000000000000000, 0.9238795325112867385, 1.000000000000000000, 0.9238795325112867385, 1.000000000000000000, 0.9238795325112867385, 1.000000000000000000, 0.9238795325112867385, 1.000000000000000000, 0.9238795325112867385, 1.000000000000000000, 0.9238795325112867385, 1.000000000000000000, 0.9238795325112867385, 1.000000000000000000, 0.9238795325112867385, 1.000000000000000000, 0.9238795325112867385, 1.000000000000000000, 0.9238795325112867385, 1.000000000000000000, 0.9238795325112867385, 1.000000000000000000, 0.9238795325112867385, 1.000000000000000000, 0.9238795325112867385, 1.000000000000000000, 0.9238795325112867385, 1.000000000000000000, 0.9238795325112867385, 1.000000000000000000, 0.9238795325112867385, 1.000000000000000000, 0.9238795325112867385, 1.000000000000000000, 0.9238795325112867385, 1.000000000000000000, 0.9238795325112867385, 1.000000000000000000, 0.9238795325112867385, 1.000000000000000000, 0.9238795325112867385, 1.000000000000000000, 0.9238795325112867385, 1.000000000000000000, 0.9238795325112867385, 1.000000000000000000, 0.9238795325112867385, 1.000000000000000000, 0.9238795325112867385, 1.000000000000000000, 0.9238795325112867385, 1.000000000000000000, 0.9238795325112867385, 1.000000000000000000, 0.9238795325112867385, 1.000000000000000000, 0.9238795325112867385, 1.000000000000000000, 0.9238795325112867385, 1.000000000000000000, 0.9238795325112867385, 1.000000000000000000, 0.9238795325112867385, 1.000000000000000000, 0.9238795325112867385, 1.000000000000000000, 0.9238795325112867385, 1.000000000000000000, 0.9238795325112867385, 1.000000000000000000, 0.9238795325112867385, 1.000000000000000000, 0.9238795325112867385, 1.000000000000000000, 0.9238795325112867385, 1.000000000000000000, 0.9238795325112867385, 1.000000000000000000, 0.9238795325112867385, 1.000000000000000000, 0.9238795325112867385, 1.000000000000000000, 0.9238795325112867385, 1.000000000000000000, 0.9238795325112867385, 1.000000000000000000, 0.9238795325112867385, 1.000000000000000000, 0.9238795325112867385, 1.000000000000000000, 0.9238795325112867385, 1.000000000000000000, 0.9238795325112867385, 1.000000000000000000, 0.9238795325112867385, 1.000000000000000000, 0.9238795325112867385, 1.000000000000000000, 0.9238795325112867385, 1.000000000000000000, 0.9238795325112867385, 1.000000000000000000, 0.9238795325112867385, 1.000000000000000000, 0.9238795325112867385, 1.000000000000000000, 0.9238795325112867385, 1.000000000000000000, 0.9238795325112867385, 1.000000000000000000, 0.9238795325112867385, 1.000000000000000000, 0.9238795325112867385, 1.000000000000000000, 0.9238795325112867385, 1.000000000000000000, 0.9238795325112867385, 1.000000000000000000, 0.9238795325112867385, 1.000000000000000000, 0.9238795325112867385, 1.000000000000000000, 0.9238795325112867385, 1.000000000000000000, 0.9238795325112867385, 1.000000000000000000, 0.9238795325112867385, 1.000000000000000000, 0.9238795325112867385, 1.000000000000000000, 0.9238795325112867385, 1.000000000000000000, 0.9238795325112867385, 1.000000000000000000, 0.9238795325112867385, 1.000000000000000000, 0.9238795325112867385, 1.000000000000000000, 0.9238795325112867385, 1.000000000000000000, 0.9238795325112867385, 1.000000000000000000, 0.9238795325112867385, 1.000000000000000000, 0.9238795325112867385, 1.000000000000000000, 0.9238795325112867385, 1.000000000000000000, 0.9238795325112867385, 1.000000000000000000, 0.9238795325112867385, 1.000000000000000000, 0.9238795325112867385, 1.000000000000000000, 0.9238795325112867385, 1.000000000000000000, 0.9238795325112867385, 1.000000000000000000, 0.9238795325112867385, 1.000000000000000000, 0.9238795325112867385, 1.000000000000000000, 0.9238795325112867385, 1.000000000000000000, 0.9238795325112867385, 1.000000000000000000, 0.9238795325112867385, 1.000000000000000000, 0.9238795325112867385, 1.000000000000000000, 0.9238795325112867385, 1.000000000000000000, 0.9238795325112867385, 1.000000000000000000, 0.9238795325112867385, 1.000000000000000000, 0.9238795325112867385, 1.000000000000000000, 0.9238795325112867385, 1.000000000000000000, 0.9238795325112867385, 1.000000000000000000, 0.9238795325112867385, 1.000000000000000000, 0.9238795325112867385, 1.000000000000000000, 0.9238795325112867385, 1.000000000000000000, 0.9238795325112867385, 1.000000000000000000, 0.9238795325112867385, 1.000000000000000000, 0.9238795325112867385, 1.000000000000000000),
 ( 1.000000000000000000, 0.9238795325112867385, 1.000000000000000000, 0.9238795325112867385, 1.000000000000000000, 0.9238795325112867385, 1.000000000000000000, 0.9238795325112867385, 1.000000000000000000, 0.9238795325112867385, 1.000000000000000000, 0.9238795325112867385, 1.000000000000000000, 0.9238795325112867385, 1.000000000000000000, 0.9238795325112867385, 1.000000000000000000, 0.9238795325112867385, 1.000000000000000000, 0.9238795325112867385, 1.000000000000000000, 0.9238795325112867385, 1.000000000000000000, 0.9238795325112867385, 1.000000000000000000, 0.9238795325112867385, 1.000000000000000000, 0.9238795325112867385, 1.000000000000000000, 0.9238795325112867385, 1.000000000000000000, 0.9238795325112867385, 1.000000000000000000, 0.9238795325112867385, 1.000000000000000000, 0.9238795325112867385, 1.000000000000000000, 0.9238795325112867385, 1.000000000000000000, 0.9238795325112867385, 1.000000000000000000, 0.9238795325112867385, 1.000000000000000000, 0.9238795325112867385, 1.000000000000000000, 0.9238795325112867385, 1.000000000000000000, 0.9238795325112867385, 1.000000000000000000, 0.9238795325112867385, 1.000000000000000000, 0.9238795325112867385, 1.000000000000000000, 0.9238795325112867385, 1.000000000000000000, 0.9238795325112867385, 1.000000000000000000, 0.9238795325112867385, 1.000000000000000000, 0.9238795325112867385, 1.000000000000000000, 0.9238795325112867385, 1.000000000000000000, 0.9238795325112867385, 1.000000000000000000, 0.9238795325112867385, 1.000000000000000000, 0.9238795325112867385, 1.000000000000000000, 0.9238795325112867385, 1.000000000000000000, 0.9238795325112867385, 1.000000000000000000, 0.9238795325112867385, 1.000000000000000000, 0.9238795325112867385, 1.000000000000000000, 0.9238795325112867385, 1.000000000000000000, 0.9238795325112867385, 1.000000000000000000, 0.9238795325112867385, 1.000000000000000000, 0.9238795325112867385, 1.000000000000000000, 0.9238795325112867385, 1.000000000000000000, 0.9238795325112867385, 1.000000000000000000, 0.9238795325112867385, 1.000000000000000000, 0.9238795325112867385, 1.000000000000000000, 0.9238795325112867385, 1.000000000000000000, 0.9238795325112867385, 1.000000000000000000, 0.9238795325112867385, 1.000000000000000000, 0.9238795325112867385, 1.000000000000000000, 0.9238795325112867385, 1.000000000000000000, 0.9238795325112867385, 1.000000000000000000, 0.9238795325112867385, 1.000000000000000000, 0.9238795325112867385, 1.000000000000000000, 0.9238795325112867385, 1.000000000000000000, 0.9238795325112867385, 1.000000000000000000, 0.9238795325112867385, 1.000000000000000000, 0.9238795325112867385, 1.000000000000000000, 0.9238795325112867385, 1.000000000000000000, 0.9238795325112867385, 1.000000000000000000, 0.9238795325112867385, 1.000000000000000000, 0.9238795325112867385, 1.000000000000000000, 0.9238795325112867385, 1.000000000000000000, 0.9238795325112867385, 1.000000000000000000, 0.9238795325112867385, 1.000000000000000000, 0.9238795325112867385, 1.000000000000000000, 0.9238795325112867385, 1.000000000000000000, 0.9238795325112867385, 1.000000000000000000, 0.9238795325112867385, 1.000000000000000000, 0.9238795325112867385, 1.000000000000000000, 0.9238795325112867385, 1.000000000000000000, 0.9238795325112867385, 1.000000000000000000, 0.9238795325112867385, 1.000000000000000000, 0.9238795325112867385, 1.000000000000000000, 0.9238795325112867385, 1.000000000000000000, 0.9238795325112867385, 1.000000000000000000, 0.9238795325112867385, 1.000000000000000000, 0.9238795325112867385, 1.000000000000000000, 0.9238795325112867385, 1.000000000000000000, 0.9238795325112867385, 1.000000000000000000, 0.9238795325112867385, 1.000000000000000000, 0.9238795325112867385, 1.000000000000000000, 0.9238795325112867385, 1.000000000000000000, 0.9238795325112867385, 1.000000000000000000, 0.9238795325112867385, 1.000000000000000000, 0.9238795325112867385, 1.000000000000000000, 0.9238795325112867385, 1.000000000000000000, 0.9238795325112867385, 1.000000000000000000, 0.9238795325112867385, 1.000000000000000000, 0.9238795325112867385, 1.000000000000000000, 0.9238795325112867385, 1.000000000000000000, 0.9238795325112867385, 1.000000000000000000, 0.9238795325112867385, 1.000000000000000000, 0.9238795325112867385, 1.000000000000000000, 0.9238795325112867385, 1.000000000000000000, 0.9238795325112867385, 1.000000000000000000, 0.9238795325112867385, 1.000000000000000000, 0.9238795325112867385, 1.000000000000000000, 0.9238795325112867385, 1.000000000000000000, 0.9238795325112867385, 1.000000000000000000, 0.9238795325112867385, 1.000000000000000000, 0.9238795325112867385, 1.000000000000000000, 0.9238795325112867385, 1.000000000000000000, 0.9238795325112867385, 1.000000000000000000, 0.9238795325112867385, 1.000000000000000000, 0.9238795325112867385, 1.000000000000000000, 0.9238795325112867385, 1.000000000000000000, 0.9238795325112867385, 1.000000000000000000, 0.9238795325112867385, 1.000000000000000000, 0.9238795325112867385, 1.000000000000000000, 0.9238795325112867385, 1.000000000000000000, 0.9238795325112867385, 1.000000000000000000, 0.9238795325112867385, 1.000000000000000000, 0.9238795325112867385, 1.000000000000000000, 0.9238795325112867385, 1.000000000000000000, 0.9238795325112867385, 1.000000000000000000, 0.9238795325112867385, 1.000000000000000000, 0.9238795325112867385, 1.000000000000000000, 0.9238795325112867385, 1.000000000000000000, 0.9238795325112867385, 1.000000000000000000, 0.9238795325112867385, 1.000000000000000000, 0.9238795325112867385, 1.000000000000000000, 0.9238795325112867385, 1.000000000000000000, 0.9238795325112867385, 1.000000000000000000, 0.9238795325112867385, 1.000000000000000000, 0.9238795325112867385, 1.000000000000000000, 0.9238795325112867385, 1.000000000000000000, 0.9238795325112867385, 1.000000000000000000, 0.9238795325112867385, 1.000000000000000000, 0.9238795325112867385, 1.000000000000000000, 0.9238795325112867385, 1.000000000000000000, 0.9238795325112867385, 1.000000000000000000, 0.9238795325112867385, 1.000000000000000000, 0.9238795325112867385, 1.000000000000000000, 0.9238795325112867385, 1.000000000000000000, 0.9238795325112867385, 1.000000000000000000, 0.9238795325112867385, 1.000000000000000000, 0.9238795325112867385, 1.000000000000000000, 0.9238795325112867385, 1.000000000000000000, 0.9238795325112867385, 1.000000000000000000, 0.9238795325112867385, 1.000000000000000000, 0.9238795325112867385, 1.000000000000000000, 0.9238795325112867385, 1.000000000000000000, 0.9238795325112867385, 1.000000000000000000, 0.9238795325112867385, 1.000000000000000000, 0.9238795325112867385, 1.000000000000000000, 0.9238795325112867385, 1.000000000000000000, 0.9238795325112867385, 1.000000000000000000, 0.9238795325112867385, 1.000000000000000000, 0.9238795325112867385, 1.000000000000000000, 0.9238795325112867385, 1.000000000000000000, 0.9238795325112867385, 1.000000000000000000, 0.9238795325112867385, 1.000000000000000000, 0.9238795325112867385, 1.000000000000000000, 0.9238795325112867385, 1.000000000000000000, 0.9238795325112867385, 1.000000000000000000, 0.9238795325112867385, 1.000000000000000000, 0.9238795325112867385, 1.000000000000000000, 0.9238795325112867385, 1.000000000000000000, 0.9238795325112867385, 1.000000000000000000, 0.9238795325112867385, 1.000000000000000000, 0.9238795325112867385, 1.000000000000000000, 0.9238795325112867385, 1.000000000000000000, 0.9238795325112867385, 1.000000000000000000, 0.9238795325112867385, 1.000000000000000000, 0.9238795325112867385, 1.000000000000000000, 0.9238795325112867385, 1.000000000000000000, 0.9238795325112867385, 1.000000000000000000, 0.9238795325112867385, 1.000000000000000000, 0.9238795325112867385, 1.000000000000000000, 0.9238795325112867385, 1.000000000000000000, 0.9238795325112867385, 1.000000000000000000, 0.9238795325112867385, 1.000000000000000000, 0.9238795325112867385, 1.000000000000000000, 0.9238795325112867385, 1.000000000000000000, 0.9238795325112867385, 1.000000000000000000, 0.9238795325112867385, 1.000000000000000000, 0.9238795325112867385, 1.000000000000000000, 0.9238795325112867385, 1.000000000000000000, 0.9238795325112867385, 1.000000000000000000, 0.9238795325112867385, 1.000000000000000000, 0.9238795325112867385, 1.000000000000000000, 0.9238795325112867385, 1.000000000000000000, 0.9238795325112867385, 1.000000000000000000, 0.9238795325112867385, 1.000000000000000000, 0.9238795325112867385, 1.000000000000000000, 0.9238795325112867385, 1.000000000000000000, 0.9238795325112867385, 1.000000000000000000, 0.9238795325112867385, 1.000000000000000000, 0.9238795325112867385, 1.000000000000000000, 0.9238795325112867385, 1.000000000000000000, 0.9238795325112867385, 1.000000000000000000, 0.9238795325112867385, 1.000000000000000000, 0.9238795325112867385, 1.000000000000000000, 0.9238795325112867385, 1.000000000000000000, 0.9238795325112867385, 1.000000000000000000, 0.9238795325112867385, 1.000000000000000000, 0.9238795325112867385, 1.000000000000000000, 0.9238795325112867385, 1.000000000000000000, 0.9238795325112867385, 1.000000000000000000, 0.9238795325112867385, 1.000000000000000000, 0.9238795325112867385, 1.000000000000000000, 0.9238795325112867385, 1.000000000000000000, 0.9238795325112867385, 1.000000000000000000, 0.9238795325112867385, 1.000000000000000000, 0.9238795325112867385, 1.000000000000000000, 0.9238795325112867385, 1.000000000000000000, 0.9238795325112867385, 1.000000000000000000, 0.9238795325112867385, 1.000000000000000000, 0.9238795325112867385, 1.000000000000000000, 0.9238795325112867385, 1.000000000000000000, 0.9238795325112867385, 1.000000000000000000, 0.9238795325112867385, 1.000000000000000000, 0.9238795325112867385, 1.000000000000000000, 0.9238795325112867385, 1.000000000000000000, 0.9238795325112867385, 1.000000000000000000, 0.9238795325112867385, 1.000000000000000000, 0.9238795325112867385, 1.000000000000000000, 0.9238795325112867385, 1.000000000000000000, 0.9238795325112867385, 1.000000000000000000, 0.9238795325112867385, 1.000000000000000000, 0.9238795325112867385, 1.000000000000000000, 0.9238795325112867385, 1.000000000000000000, 0.9238795325112867385, 1.000000000000000000, 0.9238795325112867385, 1.000000000000000000, 0.9238795325112867385, 1.000000000000000000, 0.9238795325112867385, 1.000000000000000000, 0.9238795325112867385, 1.000000000000000000, 0.9238795325112867385, 1.000000000000000000, 0.9238795325112867385, 1.000000000000000000, 0.9238795325112867385, 1.000000000000000000, 0.9238795325112867385, 1.000000000000000000, 0.9238795325112867385, 1.000000000000000000, 0.9238795325112867385, 1.000000000000000000, 0.9238795325112867385, 1.000000000000000000, 0.9238795325112867385, 1.000000000000000000, 0.9238795325112867385, 1.000000000000000000, 0.9238795325112867385, 1.000000000000000000, 0.9238795325112867385, 1.000000000000000000, 0.9238795325112867385, 1.000000000000000000) ) ) 
 REPRESENTATION_ITEM ( '' )  SURFACE ( )  );
#59341=CARTESIAN_POINT ( 'NONE',  ( 4.458734124999998549, 28.27083333469892779, -2.574251347313721627 ) ) ;
#59349=CARTESIAN_POINT ( 'NONE',  ( 5.000000000000000888, -33.58333333333332860, 2.886751345948126879 ) ) ;
#59354=CARTESIAN_POINT ( 'NONE',  ( -2.499999999999996447, 11.29166666939785202, 4.330127018922195425 ) ) ;
#59357=CARTESIAN_POINT ( 'NONE',  ( -5.000000000000000888, -169.4375000000000284, 2.071067811865474617 ) ) ;
#59359=CARTESIAN_POINT ( 'NONE',  ( -3.535533905932737309, -161.7500000027312126, -3.535533905932738197 ) ) ;
#59363=CARTESIAN_POINT ( 'NONE',  ( 1.339745962155612702, -19.16965819600733312, -5.000000000000000000 ) ) ;
#59371=CYLINDRICAL_SURFACE ( 'NONE', #61365, 5.000000000000000000 ) ;
#59372=CARTESIAN_POINT ( 'NONE',  ( -4.458734124999999437, -21.39583333196774007, -2.574251347313719407 ) ) ;
#59373=FACE_OUTER_BOUND ( 'NONE', #52228, .T. ) ;
#59374=CARTESIAN_POINT ( 'NONE',  ( -5.000000000000000888, -156.4375000000000284, 2.071067811865474617 ) ) ;
#59376=CARTESIAN_POINT ( 'NONE',  ( 3.152801135295367541, -157.3125000013656063, -3.152801135295367541 ) ) ;
#59378=CARTESIAN_POINT ( 'NONE',  ( -3.152548672688508926E-16, -43.81249999863440081, -5.148502694627439702 ) ) ;
#59379=CARTESIAN_POINT ( 'NONE',  ( 1.339745962155612702, -44.16965819600732601, -5.000000000000000000 ) ) ;
#59381=CARTESIAN_POINT ( 'NONE',  ( 9.457646018065525792E-16, -90.06249999863440792, 5.148502694627439702 ) ) ;
#59385=CARTESIAN_POINT ( 'NONE',  ( 4.458734124999998549, 7.270833334698928674, -2.574251347313721627 ) ) ;
#59389=CARTESIAN_POINT ( 'NONE',  ( 2.229367062499998831, 19.10416666803225993, -3.861377020970580887 ) ) ;
#59391=CARTESIAN_POINT ( 'NONE',  ( 5.000000000000000888, 7.541666669397851130, 2.886751345948126879 ) ) ;
#59393=CARTESIAN_POINT ( 'NONE',  ( 3.061616997868383141E-16, -161.8750000027311842, -5.000000000000000000 ) ) ;
#59396=DIRECTION ( 'NONE',  ( 0.000000000000000000, 0.000000000000000000, 1.000000000000000000 ) ) ;
#59397=CARTESIAN_POINT ( 'NONE',  ( -4.458734124999998549, -38.22916666530107932, 2.574251347313722516 ) ) ;
#59398=EDGE_CURVE ( 'NONE', #53636, #1992, #10569, .T. ) ;
#59399=CARTESIAN_POINT ( 'NONE',  ( 5.000000000000000000, -40.29166666393548013, -2.886751345948129988 ) ) ;
#59403=CARTESIAN_POINT ( 'NONE',  ( -4.458734124999998549, -12.22916666530106866, 2.574251347313722516 ) ) ;
#59404=CARTESIAN_POINT ( 'NONE',  ( 9.457646018065525792E-16, -13.31249999863440259, 5.148502694627439702 ) ) ;
#59405=ORIENTED_EDGE ( 'NONE', *, *, #45623, .F. ) ;
#59407=CARTESIAN_POINT ( 'NONE',  ( -2.499999999999996447, -79.83333333333332860, 4.330127018922195425 ) ) ;
#59408=CARTESIAN_POINT ( 'NONE',  ( -1.846868145590737420, -167.7500000013655779, 4.458734124999999437 ) ) ;
#59410=VECTOR ( 'NONE', #49488, 1000.000000000000000 ) ;
#59411=CARTESIAN_POINT ( 'NONE',  ( -2.499999999999996447, -85.70833333060214443, 4.330127018922195425 ) ) ;
#59412=CARTESIAN_POINT ( 'NONE',  ( -2.499999999999996447, -48.70833333060213732, 4.330127018922195425 ) ) ;
#59416=CARTESIAN_POINT ( 'NONE',  ( 4.458734125000001214, -25.14583333196774007, 2.574251347313718519 ) ) ;
#59420=CARTESIAN_POINT ( 'NONE',  ( -4.458734124999999437, -163.1875000013655779, -5.460374474430324690E-16 ) ) ;
#59421=EDGE_CURVE ( 'NONE', #20741, #32024, #18444, .T. ) ;
#59423=CARTESIAN_POINT ( 'NONE',  ( -1.339745962155610925, -38.66965819600732601, 5.000000000000000000 ) ) ;
#59426=CARTESIAN_POINT ( 'NONE',  ( 2.229367062499998831, -76.89583333196773651, -3.861377020970580887 ) ) ;
#59429=CARTESIAN_POINT ( 'NONE',  ( 3.152801135295366208, -146.8125000013655779, 3.152801135295367985 ) ) ;
#59432=LINE ( 'NONE', #34984, #59945 ) ;
#59437=CARTESIAN_POINT ( 'NONE',  ( 3.152801135295366208, -141.8125000013655779, 3.152801135295367985 ) ) ;
#59440=CARTESIAN_POINT ( 'NONE',  ( -2.499999999999996447, -39.70833333060214443, 4.330127018922195425 ) ) ;
#59442=CARTESIAN_POINT ( 'NONE',  ( 2.229367062499998831, -75.89583333196773651, -3.861377020970580887 ) ) ;
#59444=CARTESIAN_POINT ( 'NONE',  ( 5.000000000000000888, 14.54166666939785202, 2.886751345948126879 ) ) ;
#59452=CARTESIAN_POINT ( 'NONE',  ( -2.229367062500000163, 18.27083333469892779, -3.861377020970580443 ) ) ;
#59453=FACE_OUTER_BOUND ( 'NONE', #56740, .T. ) ;
#59459=CARTESIAN_POINT ( 'NONE',  ( 4.458734124999999437, -4.812499998634402587, -5.460374474430324690E-16 ) ) ;
#59460=CARTESIAN_POINT ( 'NONE',  ( 2.229367062500001939, -31.22916666530107221, 3.861377020970579999 ) ) ;
#59461=AXIS2_PLACEMENT_3D ( 'NONE', #22062, #36216, #60357 ) ;
#59466=CARTESIAN_POINT ( 'NONE',  ( 9.457646018065525792E-16, 27.93750000136559208, 5.148502694627439702 ) ) ;
#59469=CARTESIAN_POINT ( 'NONE',  ( 2.229367062499998831, -77.89583333196773651, -3.861377020970580887 ) ) ;
#59472=CARTESIAN_POINT ( 'NONE',  ( 5.000000000000000000, 26.62500000273118772, -6.123233995736766282E-16 ) ) ;
#59476=CARTESIAN_POINT ( 'NONE',  ( 5.000000000000000888, -17.58333333333333215, 2.886751345948126879 ) ) ;
#59477=CARTESIAN_POINT ( 'NONE',  ( -4.458734124999999437, -23.39583333196773296, -2.574251347313719407 ) ) ;
#59478=CARTESIAN_POINT ( 'NONE',  ( 4.458734125000000326, -82.89583333196773651, 2.574251347313718519 ) ) ;
#59481=CARTESIAN_POINT ( 'NONE',  ( 5.000000000000000000, -21.37499999726881228, -6.123233995736766282E-16 ) ) ;
#59482=CARTESIAN_POINT ( 'NONE',  ( -2.229367062500000163, -51.47916666530107221, -3.861377020970580443 ) ) ;
#59486=CARTESIAN_POINT ( 'NONE',  ( 4.458734124999998549, 4.020833334698926009, -2.574251347313721627 ) ) ;
#59489=CARTESIAN_POINT ( 'NONE',  ( -3.535250795749689387E-16, -65.25000000000000000, -5.773502691896257311 ) ) ;
#59490=CARTESIAN_POINT ( 'NONE',  ( -1.846868145590734756, -153.3750000013656347, -4.458734125000000326 ) ) ;
#59492=CARTESIAN_POINT ( 'NONE',  ( 1.975475456537005874E-15, -76.62499999726880162, 5.000000000000000000 ) ) ;
#59493=CARTESIAN_POINT ( 'NONE',  ( 2.071067811865476394, -161.1875000000000284, 5.000000000000000000 ) ) ;
#59494=CARTESIAN_POINT ( 'NONE',  ( 5.275681513340003914E-14, 10.74999999999999645, -5.000000000000000000 ) ) ;
#59496=CARTESIAN_POINT ( 'NONE',  ( 4.458734124999998549, -8.979166665301073991, -2.574251347313721627 ) ) ;
#59497=CARTESIAN_POINT ( 'NONE',  ( -4.458734124999998549, -45.47916666530105800, 2.574251347313722516 ) ) ;
#59498=CARTESIAN_POINT ( 'NONE',  ( -2.500000000000000444, -8.041666663935481907, -4.330127018922193649 ) ) ;
#59499=CARTESIAN_POINT ( 'NONE',  ( -4.458734125000001214, -143.8750000013656063, 1.846868145590734089 ) ) ;
#59501=CARTESIAN_POINT ( 'NONE',  ( -2.499999999999996447, 21.29166666939785202, 4.330127018922195425 ) ) ;
#59505=CARTESIAN_POINT ( 'NONE',  ( 4.458734124999999437, 28.93750000136559208, -5.460374474430324690E-16 ) ) ;
#59508=ADVANCED_FACE ( 'NONE', ( #27153 ), #7540, .T. ) ;
#59509=CARTESIAN_POINT ( 'NONE',  ( 2.500000000000002220, -29.54166666393548013, 4.330127018922192761 ) ) ;
#59510=ORIENTED_EDGE ( 'NONE', *, *, #27609, .T. ) ;
#59514=CARTESIAN_POINT ( 'NONE',  ( 2.500000000000002220, -19.66666666666666430, 4.330127018922192761 ) ) ;
#59516=CARTESIAN_POINT ( 'NONE',  ( -4.458734124999999437, -5.395833331967740953, -2.574251347313719407 ) ) ;
#59518=CARTESIAN_POINT ( 'NONE',  ( 4.458734124999997661, -149.5000000013656063, 1.846868145590737864 ) ) ;
#59520=ORIENTED_EDGE ( 'NONE', *, *, #47653, .F. ) ;
#59522=LINE ( 'NONE', #31192, #30528 ) ;
#59525=CARTESIAN_POINT ( 'NONE',  ( 2.499999999999998668, -25.20833333060214443, -4.330127018922193649 ) ) ;
#59527=( BOUNDED_CURVE ( )  B_SPLINE_CURVE ( 2, ( #21616, #21292, #41209, #46372, #7141, #16781, #56029, #40897, #60543 ),
 .UNSPECIFIED., .F., .F. ) 
 B_SPLINE_CURVE_WITH_KNOTS ( ( 3, 2, 2, 2, 3 ),
 ( 0.2729166666666666963, 0.2736111111111111382, 0.2750000000000000222, 0.2763888888888889062, 0.2770833333333333481 ),
 .UNSPECIFIED. ) 
 CURVE ( )  GEOMETRIC_REPRESENTATION_ITEM ( )  RATIONAL_B_SPLINE_CURVE ( ( 0.9330127018922194093, 0.9330127018922220739, 1.000000000000000000, 0.8660254037844387076, 1.000000000000000000, 0.8660254037844387076, 1.000000000000000000, 0.9330127018922194093, 0.9330127018922194093 ) ) 
 REPRESENTATION_ITEM ( '' )  );
#59530=DIRECTION ( 'NONE',  ( 0.000000000000000000, 0.000000000000000000, 1.000000000000000000 ) ) ;
#59533=CARTESIAN_POINT ( 'NONE',  ( 2.500000000000002220, 9.333333333333332149, 4.330127018922192761 ) ) ;
#59534=CARTESIAN_POINT ( 'NONE',  ( -4.458734124999997661, 17.77083333469892779, 2.574251347313722516 ) ) ;
#59537=CARTESIAN_POINT ( 'NONE',  ( -3.152548672688508926E-16, -11.81249999863440969, -5.148502694627439702 ) ) ;
#59539=CARTESIAN_POINT ( 'NONE',  ( -3.152801135295367985, -162.8125000013656063, 3.152801135295367096 ) ) ;
#59540=CARTESIAN_POINT ( 'NONE',  ( 5.000000000000000000, -63.29166666393547303, -2.886751345948130876 ) ) ;
#59544=CARTESIAN_POINT ( 'NONE',  ( 5.000000000000000000, -38.41666666666667140, -2.886751345948130876 ) ) ;
#59545=CARTESIAN_POINT ( 'NONE',  ( 3.061616997868383141E-16, -141.8750000027312126, -5.000000000000000000 ) ) ;
#59548=CARTESIAN_POINT ( 'NONE',  ( -8.190561711645485556E-16, -154.9375000013655779, 4.458734124999999437 ) ) ;
#59552=ORIENTED_EDGE ( 'NONE', *, *, #33496, .T. ) ;
#59557=CARTESIAN_POINT ( 'NONE',  ( -2.499999999999996447, -4.833333333333335702, 4.330127018922195425 ) ) ;
#59558=VECTOR ( 'NONE', #19256, 1000.000000000000000 ) ;
#59559=CARTESIAN_POINT ( 'NONE',  ( -2.229367062500000163, -65.47916666530106511, -3.861377020970580443 ) ) ;
#59560=EDGE_CURVE ( 'NONE', #11671, #25951, #37131, .T. ) ;
#59562=CARTESIAN_POINT ( 'NONE',  ( 1.060575238724906964E-15, -4.624999997268816720, 5.773502691896257311 ) ) ;
#59563=CARTESIAN_POINT ( 'NONE',  ( -4.458734124999999437, -34.31249999863440792, 0.000000000000000000 ) ) ;
#59564=VERTEX_POINT ( 'NONE', #32288 ) ;
#59567=ORIENTED_EDGE ( 'NONE', *, *, #6282, .F. ) ;
#59569=CARTESIAN_POINT ( 'NONE',  ( 5.000000000000000000, -50.41666666666666430, -2.886751345948129988 ) ) ;
#59570=CARTESIAN_POINT ( 'NONE',  ( 5.000000000000000888, -46.45833333060214443, 2.886751345948126879 ) ) ;
#59572=CARTESIAN_POINT ( 'NONE',  ( -1.339745962155610925, -41.66965819600731891, 5.000000000000000000 ) ) ;
#59573=CARTESIAN_POINT ( 'NONE',  ( -3.152548672688508926E-16, -76.56249999863440792, -5.148502694627439702 ) ) ;
#59574=CARTESIAN_POINT ( 'NONE',  ( -3.152801135295367985, -142.0625000013655779, 3.152801135295367096 ) ) ;
#59575=CARTESIAN_POINT ( 'NONE',  ( -3.152548672688508926E-16, -79.56249999863440792, -5.148502694627439702 ) ) ;
#59577=CARTESIAN_POINT ( 'NONE',  ( -4.458734124999999437, -28.64583333196774007, -2.574251347313719407 ) ) ;
#59578=CARTESIAN_POINT ( 'NONE',  ( -2.499999999999996447, -69.70833333060214443, 4.330127018922195425 ) ) ;
#59580=CARTESIAN_POINT ( 'NONE',  ( 5.000000000000000888, -51.58333333333332149, 2.886751345948126879 ) ) ;
#59583=CARTESIAN_POINT ( 'NONE',  ( 5.000000000000000000, -21.50000000000000000, -6.123233995736766282E-16 ) ) ;
#59584=VERTEX_POINT ( 'NONE', #47090 ) ;
#59585=CARTESIAN_POINT ( 'NONE',  ( 5.000000000000000000, 27.50000000000000000, -6.123233995736766282E-16 ) ) ;
#59586=( BOUNDED_CURVE ( )  B_SPLINE_CURVE ( 2, ( #31781, #13115, #41736, #46262, #22779, #12162, #7355, #36933, #26643 ),
 .UNSPECIFIED., .F., .F. ) 
 B_SPLINE_CURVE_WITH_KNOTS ( ( 3, 2, 2, 2, 3 ),
 ( 0.8437500000000000000, 0.8444444444444444420, 0.8458333333333333259, 0.8472222222222222099, 0.8479166666666666519 ),
 .UNSPECIFIED. ) 
 CURVE ( )  GEOMETRIC_REPRESENTATION_ITEM ( )  RATIONAL_B_SPLINE_CURVE ( ( 0.9330127018922194093, 0.9330127018922194093, 1.000000000000000000, 0.8660254037844387076, 1.000000000000000000, 0.8660254037844387076, 1.000000000000000000, 0.9330127018922194093, 0.9330127018922194093 ) ) 
 REPRESENTATION_ITEM ( '' )  );
#59587=CARTESIAN_POINT ( 'NONE',  ( 1.339745962155661996, -12.29465819873852084, -4.999999999999970690 ) ) ;
#59588=CARTESIAN_POINT ( 'NONE',  ( -4.458734124999999437, -58.56249999863440081, 0.000000000000000000 ) ) ;
#59591=LINE ( 'NONE', #5870, #40898 ) ;
#59593=CARTESIAN_POINT ( 'NONE',  ( 4.458734125000001214, 15.10416666803225993, 2.574251347313718519 ) ) ;
#59596=CARTESIAN_POINT ( 'NONE',  ( -1.846868145590737420, -161.7500000013655779, 4.458734124999997661 ) ) ;
#59597=CARTESIAN_POINT ( 'NONE',  ( 6.123233995736766282E-16, -170.0000000000000000, -5.000000000000000000 ) ) ;
#59608=CARTESIAN_POINT ( 'NONE',  ( -4.999999999999998224, -20.91666666666666785, 2.886751345948131764 ) ) ;
#59613=CARTESIAN_POINT ( 'NONE',  ( 9.457646018065525792E-16, 9.687500001365593860, 5.148502694627439702 ) ) ;
#59614=CARTESIAN_POINT ( 'NONE',  ( 3.061616997868383141E-16, -161.8750000027311842, -5.000000000000000000 ) ) ;
#59616=CARTESIAN_POINT ( 'NONE',  ( 2.071067811865475505, -143.9375000027311842, -5.000000000000000888 ) ) ;
#59617=CARTESIAN_POINT ( 'NONE',  ( 0.000000000000000000, -170.0000000000000000, 0.000000000000000000 ) ) ;
#59622=CARTESIAN_POINT ( 'NONE',  ( 5.000000000000000000, -140.0000000000000000, 0.000000000000000000 ) ) ;
#59623=CARTESIAN_POINT ( 'NONE',  ( 5.000000000000000000, -141.1250000027312126, 0.000000000000000000 ) ) ;
#59625=CARTESIAN_POINT ( 'NONE',  ( 4.458734124999999437, -164.6875000013655779, 0.000000000000000000 ) ) ;
#59626=CARTESIAN_POINT ( 'NONE',  ( -1.339745962155613812, -33.20534180126147561, -5.000000000000000000 ) ) ;
#59628=CARTESIAN_POINT ( 'NONE',  ( 3.152801135295366208, -145.5625000013655779, 3.152801135295367985 ) ) ;
#59630=CARTESIAN_POINT ( 'NONE',  ( -2.229367062500000163, 22.27083333469892423, -3.861377020970580443 ) ) ;
#59632=CARTESIAN_POINT ( 'NONE',  ( -4.458734124999999437, -61.64583333196774362, -2.574251347313719407 ) ) ;
#59635=CARTESIAN_POINT ( 'NONE',  ( 1.975475456537005874E-15, 2.249999999999999556, 5.000000000000000000 ) ) ;
#59636=CARTESIAN_POINT ( 'NONE',  ( -5.000000000000000000, 13.91666666666666785, -2.886751345948128211 ) ) ;
#59637=CARTESIAN_POINT ( 'NONE',  ( -2.229367062500000163, -49.47916666530107221, -3.861377020970580443 ) ) ;
#59638=CARTESIAN_POINT ( 'NONE',  ( 9.457646018065525792E-16, -12.06249999863440081, 5.148502694627439702 ) ) ;
#59639=DIRECTION ( 'NONE',  ( -0.000000000000000000, 1.000000000000000000, -0.000000000000000000 ) ) ;
#59640=CARTESIAN_POINT ( 'NONE',  ( -1.339745962155610925, -63.66965819600734022, 5.000000000000000000 ) ) ;
#59641=DIRECTION ( 'NONE',  ( 0.000000000000000000, 0.000000000000000000, 1.000000000000000000 ) ) ;
#59645=CARTESIAN_POINT ( 'NONE',  ( -2.500000000000000444, -59.16666666666665719, -4.330127018922193649 ) ) ;
#59648=CARTESIAN_POINT ( 'NONE',  ( 4.458734124999999437, -54.81249999863440081, -5.460374474430324690E-16 ) ) ;
#59649=CARTESIAN_POINT ( 'NONE',  ( -3.152801135295367985, -157.0625000013656063, 3.152801135295367096 ) ) ;
#59651=CARTESIAN_POINT ( 'NONE',  ( 5.000000000000000000, -55.37499999726880162, -6.123233995736766282E-16 ) ) ;
#59652=EDGE_LOOP ( 'NONE', ( #31569, #37431, #7292, #63497 ) ) ;
#59654=CARTESIAN_POINT ( 'NONE',  ( 4.458734124999999437, -3.062499998634407472, -5.460374474430324690E-16 ) ) ;
#59658=CARTESIAN_POINT ( 'NONE',  ( -8.190561711645485556E-16, -157.6875000013655779, 4.458734124999999437 ) ) ;
#59659=VERTEX_POINT ( 'NONE', #34168 ) ;
#59660=CARTESIAN_POINT ( 'NONE',  ( 1.339745962155609149, 25.29465819873851729, 5.000000000000003553 ) ) ;
#59662=CARTESIAN_POINT ( 'NONE',  ( 5.000000000000000000, -80.37499999726881583, -6.123233995736766282E-16 ) ) ;
#59663=CARTESIAN_POINT ( 'NONE',  ( -2.229367062499996610, -44.39583333196774362, 3.861377020970582219 ) ) ;
#59664=VERTEX_POINT ( 'NONE', #33551 ) ;
#59667=CARTESIAN_POINT ( 'NONE',  ( 4.458734125000001214, -90.14583333196773651, 2.574251347313718519 ) ) ;
#59675=CARTESIAN_POINT ( 'NONE',  ( -1.339745962155610925, -26.79465819873852084, 5.000000000000000000 ) ) ;
#59679=DIRECTION ( 'NONE',  ( -0.000000000000000000, 1.000000000000000000, -0.000000000000000000 ) ) ;
#59680=CARTESIAN_POINT ( 'NONE',  ( 2.229367062500001939, -89.22916666530106511, 3.861377020970579999 ) ) ;
#59681=DIRECTION ( 'NONE',  ( 0.000000000000000000, 0.000000000000000000, 1.000000000000000000 ) ) ;
#59683=ORIENTED_EDGE ( 'NONE', *, *, #29997, .T. ) ;
#59684=CARTESIAN_POINT ( 'NONE',  ( -5.000000000000000000, -143.6250000027312126, -6.123233995736766282E-16 ) ) ;
#59686=CARTESIAN_POINT ( 'NONE',  ( 2.071067811865476394, -161.3125000027312126, 5.000000000000000000 ) ) ;
#59690=EDGE_CURVE ( 'NONE', #44836, #13136, #24850, .T. ) ;
#59699=CARTESIAN_POINT ( 'NONE',  ( -4.458734124999997661, -22.22916666530107221, 2.574251347313722516 ) ) ;
#59700=DIRECTION ( 'NONE',  ( 0.000000000000000000, -1.000000000000000000, 0.000000000000000000 ) ) ;
#59701=CARTESIAN_POINT ( 'NONE',  ( 5.000000000000000000, -156.0000000000000000, 0.000000000000000000 ) ) ;
#59703=CARTESIAN_POINT ( 'NONE',  ( 1.846868145590736310, -155.6250000013656063, 4.458734124999999437 ) ) ;
#59705=CARTESIAN_POINT ( 'NONE',  ( 4.458734124999999437, -45.06249999863440081, -5.460374474430324690E-16 ) ) ;
#59708=CARTESIAN_POINT ( 'NONE',  ( -4.458734124999999437, -88.31249999863439371, 0.000000000000000000 ) ) ;
#59709=( BOUNDED_CURVE ( )  B_SPLINE_CURVE ( 2, ( #35629, #55257, #44958, #919, #16005, #15689, #59118, #25661, #10855 ),
 .UNSPECIFIED., .F., .F. ) 
 B_SPLINE_CURVE_WITH_KNOTS ( ( 3, 2, 2, 2, 3 ),
 ( 0.1083333333333334203, 0.1125000000000000999, 0.1166666666666667657, 0.1208333333333334314, 0.1250000000000001110 ),
 .UNSPECIFIED. ) 
 CURVE ( )  GEOMETRIC_REPRESENTATION_ITEM ( )  RATIONAL_B_SPLINE_CURVE ( ( 0.9999999999999984457, 0.9238795325112882928, 1.000000000000000000, 0.9238795325112867385, 1.000000000000000000, 0.9238795325112867385, 1.000000000000000000, 0.9238795325112847401, 1.000000000000001998 ) ) 
 REPRESENTATION_ITEM ( '' )  );
#59710=CARTESIAN_POINT ( 'NONE',  ( -2.229367062500000163, 4.520833334698926897, -3.861377020970580443 ) ) ;
#59711=ADVANCED_FACE ( 'NONE', ( #14865 ), #19058, .T. ) ;
#59714=CARTESIAN_POINT ( 'NONE',  ( 5.000000000000000000, 13.58333333333333215, -2.886751345948130876 ) ) ;
#59715=CARTESIAN_POINT ( 'NONE',  ( -9.184850993605147944E-16, -152.3750000027311842, 5.000000000000000000 ) ) ;
#59716=CARTESIAN_POINT ( 'NONE',  ( 4.458734124999998549, 22.02083333469892779, -2.574251347313721627 ) ) ;
#59718=CARTESIAN_POINT ( 'NONE',  ( 2.499999999999998668, 8.791666669397853795, -4.330127018922193649 ) ) ;
#59721=ORIENTED_EDGE ( 'NONE', *, *, #56752, .T. ) ;
#59723=CARTESIAN_POINT ( 'NONE',  ( 4.458734124999998549, -36.72916666530107221, -2.574251347313721627 ) ) ;
#59724=EDGE_CURVE ( 'NONE', #56134, #29294, #28604, .T. ) ;
#59725=CARTESIAN_POINT ( 'NONE',  ( -5.000000000000000000, -38.95833333060214443, -2.886751345948128211 ) ) ;
#59727=CARTESIAN_POINT ( 'NONE',  ( 4.458734125000001214, -12.89583333196774184, 2.574251347313718519 ) ) ;
#59728=CARTESIAN_POINT ( 'NONE',  ( -4.458734124999999437, -21.56249999863440436, 0.000000000000000000 ) ) ;
#59730=CARTESIAN_POINT ( 'NONE',  ( -3.535250795749689387E-16, -80.25000000000000000, -5.773502691896257311 ) ) ;
#59731=CARTESIAN_POINT ( 'NONE',  ( -6.972266317189433020E-16, -46.12499999726880873, -5.000000000000000000 ) ) ;
#59733=CARTESIAN_POINT ( 'NONE',  ( -3.535250795749689387E-16, -86.12499999726880162, -5.773502691896257311 ) ) ;
#59734=CARTESIAN_POINT ( 'NONE',  ( -6.972266317189433020E-16, -32.24999999999999289, -5.000000000000000000 ) ) ;
#59738=CARTESIAN_POINT ( 'NONE',  ( -3.152548672688508926E-16, -25.81249999863440792, -5.148502694627439702 ) ) ;
#59740=ORIENTED_EDGE ( 'NONE', *, *, #62196, .F. ) ;
#59742=CARTESIAN_POINT ( 'NONE',  ( -3.152801135295367985, -163.0625000013656063, 3.152801135295367096 ) ) ;
#59743=EDGE_CURVE ( 'NONE', #28871, #55230, #52483, .T. ) ;
#59745=CARTESIAN_POINT ( 'NONE',  ( 3.535533905932738197, -155.8750000000000000, -3.535533905932738197 ) ) ;
#59748=CARTESIAN_POINT ( 'NONE',  ( 2.229367062499998831, -74.89583333196773651, -3.861377020970580887 ) ) ;
#59751=CARTESIAN_POINT ( 'NONE',  ( 3.152801135295367541, -140.5625000013655779, -3.152801135295367541 ) ) ;
#59754=LINE ( 'NONE', #40431, #60440 ) ;
#59757=CARTESIAN_POINT ( 'NONE',  ( -4.458734124999999437, -140.1875000013656063, -5.460374474430324690E-16 ) ) ;
#59762=CARTESIAN_POINT ( 'NONE',  ( -4.458734124999998549, -74.47916666530106511, 2.574251347313722516 ) ) ;
#59764=CARTESIAN_POINT ( 'NONE',  ( -5.000000000000000888, -139.5625000027312126, 2.071067811865474617 ) ) ;
#59765=CARTESIAN_POINT ( 'NONE',  ( -9.184850993605147944E-16, -165.2500000000000000, 5.000000000000000000 ) ) ;
#59767=ORIENTED_EDGE ( 'NONE', *, *, #4629, .F. ) ;
#59775=CARTESIAN_POINT ( 'NONE',  ( 4.458734124999999437, 15.93750000136559564, -5.460374474430324690E-16 ) ) ;
#59779=EDGE_CURVE ( 'NONE', #57628, #34331, #4283, .T. ) ;
#59784=CARTESIAN_POINT ( 'NONE',  ( 4.458734124999999437, -83.81249999863439371, -5.460374474430324690E-16 ) ) ;
#59785=CARTESIAN_POINT ( 'NONE',  ( -4.458734124999997661, -4.229166665301070438, 2.574251347313722516 ) ) ;
#59787=CARTESIAN_POINT ( 'NONE',  ( -4.458734124999999437, -31.64583333196773651, -2.574251347313719407 ) ) ;
#59793=CARTESIAN_POINT ( 'NONE',  ( 4.458734124999999437, 23.18750000136559564, -5.460374474430324690E-16 ) ) ;
#59796=CARTESIAN_POINT ( 'NONE',  ( 3.061616997868383141E-16, -145.8750000027312126, -5.000000000000000000 ) ) ;
#59797=CARTESIAN_POINT ( 'NONE',  ( -2.229367062500000163, -79.72916666530106511, -3.861377020970580443 ) ) ;
#59800=CARTESIAN_POINT ( 'NONE',  ( -4.999999999999999112, 25.20833333606451987, 2.886751345948131764 ) ) ;
#59801=ORIENTED_EDGE ( 'NONE', *, *, #33149, .T. ) ;
#59802=CARTESIAN_POINT ( 'NONE',  ( 5.000000000000000888, -1.458333330602148870, 2.886751345948126879 ) ) ;
#59803=CYLINDRICAL_SURFACE ( 'NONE', #23743, 5.000000000000000000 ) ;
#59805=CARTESIAN_POINT ( 'NONE',  ( -4.999999999999999112, -16.91666666666666430, 2.886751345948131764 ) ) ;
#59806=CARTESIAN_POINT ( 'NONE',  ( 4.458734125000001214, -23.89583333196774007, 2.574251347313718519 ) ) ;
#59807=CARTESIAN_POINT ( 'NONE',  ( -2.229367062500000163, -84.47916666530107932, -3.861377020970580443 ) ) ;
#59808=CARTESIAN_POINT ( 'NONE',  ( -3.535250795749689387E-16, -25.12499999726881228, -5.773502691896257311 ) ) ;
#59809=CARTESIAN_POINT ( 'NONE',  ( -2.229367062499996610, -52.14583333196773651, 3.861377020970582219 ) ) ;
#59810=VERTEX_POINT ( 'NONE', #40278 ) ;
#59811=CARTESIAN_POINT ( 'NONE',  ( 1.339745962155615144, -65.70534180126148271, 4.999999999999999112 ) ) ;
#59812=CARTESIAN_POINT ( 'NONE',  ( 5.000000000000000000, -74.37499999726880162, -6.123233995736766282E-16 ) ) ;
#59813=CARTESIAN_POINT ( 'NONE',  ( -4.458734124999999437, -4.645833331967739177, -2.574251347313719407 ) ) ;
#59814=ORIENTED_EDGE ( 'NONE', *, *, #50727, .T. ) ;
#59816=CARTESIAN_POINT ( 'NONE',  ( 5.000000000000000888, -67.58333333333332860, 2.886751345948126879 ) ) ;
#59817=CARTESIAN_POINT ( 'NONE',  ( -4.458734124999999437, -151.1875000013656063, -5.460374474430324690E-16 ) ) ;
#59819=CARTESIAN_POINT ( 'NONE',  ( -6.972266317189433020E-16, -79.24999999999998579, -5.000000000000000000 ) ) ;
#59820=( BOUNDED_CURVE ( )  B_SPLINE_CURVE ( 2, ( #271, #63632, #19869, #39483, #59119, #49776, #5403, #28885, #15049 ),
 .UNSPECIFIED., .F., .F. ) 
 B_SPLINE_CURVE_WITH_KNOTS ( ( 3, 2, 2, 2, 3 ),
 ( 0.8312500000000000444, 0.8319444444444444864, 0.8333333333333333703, 0.8347222222222222543, 0.8354166666666666963 ),
 .UNSPECIFIED. ) 
 CURVE ( )  GEOMETRIC_REPRESENTATION_ITEM ( )  RATIONAL_B_SPLINE_CURVE ( ( 0.9330127018922194093, 0.9330127018922194093, 1.000000000000000000, 0.8660254037844387076, 1.000000000000000000, 0.8660254037844387076, 1.000000000000000000, 0.9330127018922194093, 0.9330127018922194093 ) ) 
 REPRESENTATION_ITEM ( '' )  );
#59821=CARTESIAN_POINT ( 'NONE',  ( -5.000000000000000888, -157.4375000000000000, 2.071067811865474617 ) ) ;
#59822=CARTESIAN_POINT ( 'NONE',  ( -2.500000000000000444, 6.958333336064520758, -4.330127018922193649 ) ) ;
#59824=CARTESIAN_POINT ( 'NONE',  ( 4.458734125000001214, -13.14583333196774184, 2.574251347313718519 ) ) ;
#59825=CARTESIAN_POINT ( 'NONE',  ( -3.152548672688508926E-16, -45.81249999863440081, -5.148502694627439702 ) ) ;
#59827=CARTESIAN_POINT ( 'NONE',  ( -1.846868145590734756, -146.1250000013655779, -4.458734125000000326 ) ) ;
#59829=CARTESIAN_POINT ( 'NONE',  ( -5.000000000000000000, 21.04166666939784847, -2.886751345948128211 ) ) ;
#59830=EDGE_LOOP ( 'NONE', ( #58513, #6865, #22075, #35842 ) ) ;
#59832=CARTESIAN_POINT ( 'NONE',  ( -4.458734124999998549, 26.52083333469892779, 2.574251347313722516 ) ) ;
#59835=VERTEX_POINT ( 'NONE', #30942 ) ;
#59840=CARTESIAN_POINT ( 'NONE',  ( 4.458734125000001214, -9.895833331967736513, 2.574251347313718519 ) ) ;
#59841=CARTESIAN_POINT ( 'NONE',  ( 5.000000000000000888, -73.45833333060214443, 2.886751345948126879 ) ) ;
#59842=CARTESIAN_POINT ( 'NONE',  ( -4.458734124999999437, -150.0000000013656063, -1.846868145590735644 ) ) ;
#59844=ORIENTED_EDGE ( 'NONE', *, *, #14545, .T. ) ;
#59845=CARTESIAN_POINT ( 'NONE',  ( 1.975475456537005874E-15, -26.62499999726881228, 5.000000000000000000 ) ) ;
#59848=CARTESIAN_POINT ( 'NONE',  ( 6.123233995736766282E-16, -170.0000000000000000, -5.000000000000000000 ) ) ;
#59849=CYLINDRICAL_SURFACE ( 'NONE', #1682, 5.000000000000000000 ) ;
#59853=CARTESIAN_POINT ( 'NONE',  ( 5.000000000000000000, -74.50000000000000000, -6.123233995736766282E-16 ) ) ;
#59857=CARTESIAN_POINT ( 'NONE',  ( 2.229367062500001939, 14.02083333469892779, 3.861377020970579999 ) ) ;
#59859=ORIENTED_EDGE ( 'NONE', *, *, #10148, .T. ) ;
#59860=CARTESIAN_POINT ( 'NONE',  ( 2.229367062500001939, -12.22916666530107044, 3.861377020970579999 ) ) ;
#59863=CARTESIAN_POINT ( 'NONE',  ( -4.458734125000000326, -164.0000000013656063, -1.846868145590735644 ) ) ;
#59868=EDGE_CURVE ( 'NONE', #38026, #176, #4016, .T. ) ;
#59873=FACE_OUTER_BOUND ( 'NONE', #23035, .T. ) ;
#59874=CARTESIAN_POINT ( 'NONE',  ( -3.152801135295367985, -149.0625000013655779, 3.152801135295367096 ) ) ;
#59877=ADVANCED_FACE ( 'NONE', ( #60549 ), #50244, .T. ) ;
#59879=ORIENTED_EDGE ( 'NONE', *, *, #26837, .F. ) ;
#59884=CARTESIAN_POINT ( 'NONE',  ( 1.060575238724906964E-15, -2.750000000000002220, 5.773502691896257311 ) ) ;
#59885=CARTESIAN_POINT ( 'NONE',  ( 4.458734124999999437, -65.81249999863440792, -5.460374474430324690E-16 ) ) ;
#59887=EDGE_CURVE ( 'NONE', #25786, #10271, #52853, .T. ) ;
#59888=CARTESIAN_POINT ( 'NONE',  ( -4.999999999999999112, -7.791666663935482795, 2.886751345948131764 ) ) ;
#59889=CARTESIAN_POINT ( 'NONE',  ( -3.152548672688508926E-16, -34.56249999863440792, -5.148502694627439702 ) ) ;
#59891=FACE_OUTER_BOUND ( 'NONE', #57539, .T. ) ;
#59893=CARTESIAN_POINT ( 'NONE',  ( 4.458734124999999437, 11.93750000136559564, -5.460374474430324690E-16 ) ) ;
#59896=CARTESIAN_POINT ( 'NONE',  ( -3.535250795749689387E-16, -52.25000000000001421, -5.773502691896257311 ) ) ;
#59899=CARTESIAN_POINT ( 'NONE',  ( 2.229367062500001939, -73.97916666530106511, 3.861377020970579999 ) ) ;
#59900=CARTESIAN_POINT ( 'NONE',  ( -3.535533905932737309, -169.6250000000000284, -3.535533905932738197 ) ) ;
#59901=CARTESIAN_POINT ( 'NONE',  ( -2.229367062500000163, -84.47916666530107932, -3.861377020970580443 ) ) ;
#59903=( BOUNDED_CURVE ( )  B_SPLINE_CURVE ( 2, ( #10055, #58322, #23908, #44463, #422, #33871, #9418, #15202, #34827 ),
 .UNSPECIFIED., .F., .F. ) 
 B_SPLINE_CURVE_WITH_KNOTS ( ( 3, 2, 2, 2, 3 ),
 ( 0.8229166666666666297, 0.8236111111111110716, 0.8249999999999999556, 0.8263888888888888395, 0.8270833333333332815 ),
 .UNSPECIFIED. ) 
 CURVE ( )  GEOMETRIC_REPRESENTATION_ITEM ( )  RATIONAL_B_SPLINE_CURVE ( ( 0.9330127018922194093, 0.9330127018922194093, 1.000000000000000000, 0.8660254037844387076, 1.000000000000000000, 0.8660254037844387076, 1.000000000000000000, 0.9330127018922194093, 0.9330127018922194093 ) ) 
 REPRESENTATION_ITEM ( '' )  );
#59904=CARTESIAN_POINT ( 'NONE',  ( 4.458734124999999437, -28.06249999863440081, -5.460374474430324690E-16 ) ) ;
#59906=CARTESIAN_POINT ( 'NONE',  ( 2.499999999999998668, -51.33333333333332860, -4.330127018922193649 ) ) ;
#59910=ORIENTED_EDGE ( 'NONE', *, *, #53156, .T. ) ;
#59911=DIRECTION ( 'NONE',  ( 0.000000000000000000, 0.000000000000000000, 1.000000000000000000 ) ) ;
#59913=CARTESIAN_POINT ( 'NONE',  ( 4.458734124999999437, -67.06249999863440792, -5.460374474430324690E-16 ) ) ;
#59915=ORIENTED_EDGE ( 'NONE', *, *, #3220, .F. ) ;
#59919=CARTESIAN_POINT ( 'NONE',  ( -4.458734124999998549, 6.770833334698928674, 2.574251347313722516 ) ) ;
#59921=CARTESIAN_POINT ( 'NONE',  ( -4.458734124999999437, -161.0000000013656063, -1.846868145590735644 ) ) ;
#59923=ORIENTED_EDGE ( 'NONE', *, *, #31896, .F. ) ;
#59925=CARTESIAN_POINT ( 'NONE',  ( 3.535533905932738197, -164.0000000027312126, -3.535533905932738197 ) ) ;
#59927=CARTESIAN_POINT ( 'NONE',  ( 0.000000000000000000, -170.0000000000000000, 5.000000000000000000 ) ) ;
#59928=CARTESIAN_POINT ( 'NONE',  ( 2.499999999999998668, 4.791666669397852907, -4.330127018922193649 ) ) ;
#59932=CARTESIAN_POINT ( 'NONE',  ( 1.975475456537005874E-15, -78.62499999726881583, 5.000000000000000000 ) ) ;
#59934=CARTESIAN_POINT ( 'NONE',  ( -4.458734124999997661, 27.77083333469892423, 2.574251347313722516 ) ) ;
#59937=CARTESIAN_POINT ( 'NONE',  ( 4.458734124999999437, 2.937500001365594304, -5.460374474430324690E-16 ) ) ;
#59940=CARTESIAN_POINT ( 'NONE',  ( -3.535533905932738641, -146.5000000027311842, 3.535533905932737309 ) ) ;
#59941=CARTESIAN_POINT ( 'NONE',  ( 3.535533905932738197, -158.8750000000000284, -3.535533905932738197 ) ) ;
#59945=VECTOR ( 'NONE', #50085, 1000.000000000000000 ) ;
#59949=CARTESIAN_POINT ( 'NONE',  ( 1.846868145590735200, -162.5000000013655779, -4.458734124999999437 ) ) ;
#59950=CARTESIAN_POINT ( 'NONE',  ( -9.184850993605147944E-16, -160.2500000000000000, 5.000000000000000000 ) ) ;
#59953=CARTESIAN_POINT ( 'NONE',  ( 3.152801135295366208, -139.5625000013655779, 3.152801135295367985 ) ) ;
#59954=ORIENTED_EDGE ( 'NONE', *, *, #54712, .T. ) ;
#59955=CARTESIAN_POINT ( 'NONE',  ( -4.458734124999999437, 22.35416666803225638, -2.574251347313719407 ) ) ;
#59957=CARTESIAN_POINT ( 'NONE',  ( -4.458734124999997661, -61.47916666530106511, 2.574251347313722516 ) ) ;
#59959=DIRECTION ( 'NONE',  ( -0.000000000000000000, 1.000000000000000000, -0.000000000000000000 ) ) ;
#59960=CARTESIAN_POINT ( 'NONE',  ( -5.000000000000000000, 16.00000000000000000, 0.000000000000000000 ) ) ;
#59961=CARTESIAN_POINT ( 'NONE',  ( -3.152548672688508926E-16, -49.56249999863441502, -5.148502694627439702 ) ) ;
#59962=CARTESIAN_POINT ( 'NONE',  ( -2.229367062500000163, -12.47916666530107044, -3.861377020970580443 ) ) ;
#59964=EDGE_CURVE ( 'NONE', #47465, #47715, #59591, .T. ) ;
#59965=CARTESIAN_POINT ( 'NONE',  ( -1.339745962155610925, 14.20534180126148094, 5.000000000000000000 ) ) ;
#59969=CARTESIAN_POINT ( 'NONE',  ( -6.972266317189433020E-16, -33.24999999999999289, -5.000000000000000000 ) ) ;
#59972=CARTESIAN_POINT ( 'NONE',  ( 4.458734125000001214, -59.89583333196774362, 2.574251347313718519 ) ) ;
#59973=CARTESIAN_POINT ( 'NONE',  ( 3.152801135295367541, -155.5625000013656063, -3.152801135295367541 ) ) ;
#59974=CARTESIAN_POINT ( 'NONE',  ( -2.500000000000000444, -53.04166666393548013, -4.330127018922193649 ) ) ;
#59977=CARTESIAN_POINT ( 'NONE',  ( 2.229367062499998831, 1.104166668032261711, -3.861377020970580887 ) ) ;
#59981=CARTESIAN_POINT ( 'NONE',  ( 3.152801135295366208, -157.5625000013656063, 3.152801135295367985 ) ) ;
#59983=CYLINDRICAL_SURFACE ( 'NONE', #6720, 5.000000000000000000 ) ;
#59986=CARTESIAN_POINT ( 'NONE',  ( 4.458734124999998549, -50.97916666530107221, -2.574251347313721627 ) ) ;
#59990=CARTESIAN_POINT ( 'NONE',  ( 9.457646018065525792E-16, 26.93750000136559564, 5.148502694627439702 ) ) ;
#59992=CARTESIAN_POINT ( 'NONE',  ( 6.123233995736766282E-16, -170.0000000000000000, -5.000000000000000000 ) ) ;
#59997=CARTESIAN_POINT ( 'NONE',  ( 1.975475456537005874E-15, 7.249999999999998224, 5.000000000000000000 ) ) ;
#59998=CARTESIAN_POINT ( 'NONE',  ( 3.061616997868383141E-16, -157.7500000000000000, -5.000000000000000000 ) ) ;
#60003=CARTESIAN_POINT ( 'NONE',  ( 4.458734124999998549, -88.97916666530107932, -2.574251347313721627 ) ) ;
#60004=CARTESIAN_POINT ( 'NONE',  ( 0.000000000000000000, -170.0000000000000000, 5.000000000000000000 ) ) ;
#60006=ORIENTED_EDGE ( 'NONE', *, *, #56503, .T. ) ;
#60007=( BOUNDED_CURVE ( )  B_SPLINE_CURVE ( 2, ( #57871, #13793, #34350, #33415, #49474, #53979, #9907, #48517, #29517 ),
 .UNSPECIFIED., .F., .F. ) 
 B_SPLINE_CURVE_WITH_KNOTS ( ( 3, 2, 2, 2, 3 ),
 ( 0.04791666666666666990, 0.04861111111111111188, 0.05000000000000000278, 0.05138888888888888673, 0.05208333333333333565 ),
 .UNSPECIFIED. ) 
 CURVE ( )  GEOMETRIC_REPRESENTATION_ITEM ( )  RATIONAL_B_SPLINE_CURVE ( ( 0.9330127018922192983, 0.9330127018922196314, 1.000000000000000000, 0.8660254037844387076, 1.000000000000000000, 0.8660254037844387076, 1.000000000000000000, 0.9330127018922189652, 0.9330127018922192983 ) ) 
 REPRESENTATION_ITEM ( '' )  );
#60008=CARTESIAN_POINT ( 'NONE',  ( 2.500000000000002220, -31.66666666666666075, 4.330127018922192761 ) ) ;
#60010=CARTESIAN_POINT ( 'NONE',  ( -3.535533905932737309, -156.7500000027312126, -3.535533905932738197 ) ) ;
#60022=CARTESIAN_POINT ( 'NONE',  ( 4.458734124999998549, -19.72916666530107221, -2.574251347313721627 ) ) ;
#60024=CARTESIAN_POINT ( 'NONE',  ( 5.000000000000000000, -150.0000000000000284, 0.000000000000000000 ) ) ;
#60026=CARTESIAN_POINT ( 'NONE',  ( 4.458734125000000326, -150.3750000013655779, -1.846868145590734978 ) ) ;
#60028=CARTESIAN_POINT ( 'NONE',  ( 4.458734124999999437, -46.06249999863440081, -5.460374474430324690E-16 ) ) ;
#60029=CARTESIAN_POINT ( 'NONE',  ( -6.972266317189433020E-16, -44.12499999726880162, -5.000000000000000000 ) ) ;
#60031=CARTESIAN_POINT ( 'NONE',  ( -2.229367062499996610, -89.14583333196773651, 3.861377020970582219 ) ) ;
#60032=CARTESIAN_POINT ( 'NONE',  ( -2.229367062500000163, 6.520833334698928674, -3.861377020970580443 ) ) ;
#60033=CARTESIAN_POINT ( 'NONE',  ( 1.339745962155615144, -41.58034179853029144, 4.999999999999999112 ) ) ;
#60035=CARTESIAN_POINT ( 'NONE',  ( -2.229367062500000163, 18.27083333469892779, -3.861377020970580443 ) ) ;
#60037=CARTESIAN_POINT ( 'NONE',  ( -3.535250795749689387E-16, 10.87500000273118417, -5.773502691896257311 ) ) ;
#60039=CARTESIAN_POINT ( 'NONE',  ( 5.000000000000000888, -162.0625000027312410, -2.071067811865475505 ) ) ;
#60042=CARTESIAN_POINT ( 'NONE',  ( -2.229367062499996610, -44.14583333196774362, 3.861377020970582219 ) ) ;
#60043=CARTESIAN_POINT ( 'NONE',  ( -2.499999999999996447, -41.70833333060214443, 4.330127018922195425 ) ) ;
#60044=ORIENTED_EDGE ( 'NONE', *, *, #46767, .F. ) ;
#60045=CARTESIAN_POINT ( 'NONE',  ( -2.229367062499996610, -20.14583333196774007, 3.861377020970582219 ) ) ;
#60046=ORIENTED_EDGE ( 'NONE', *, *, #61844, .T. ) ;
#60047=CARTESIAN_POINT ( 'NONE',  ( -4.999999999999999112, -82.91666666666667140, 2.886751345948131764 ) ) ;
#60049=CARTESIAN_POINT ( 'NONE',  ( -3.535250795749689387E-16, -88.12499999726878741, -5.773502691896257311 ) ) ;
#60051=EDGE_LOOP ( 'NONE', ( #4403, #16536, #39349, #9861 ) ) ;
#60054=CARTESIAN_POINT ( 'NONE',  ( 9.457646018065525792E-16, -28.31249999863440081, 5.148502694627439702 ) ) ;
#60055=ORIENTED_EDGE ( 'NONE', *, *, #40513, .F. ) ;
#60057=CARTESIAN_POINT ( 'NONE',  ( 1.846868145590735200, -163.5000000013655779, -4.458734125000000326 ) ) ;
#60060=CARTESIAN_POINT ( 'NONE',  ( 5.000000000000000000, -148.0000000000000284, 0.000000000000000000 ) ) ;
#60064=CARTESIAN_POINT ( 'NONE',  ( -2.229367062499996610, -74.39583333196773651, 3.861377020970582219 ) ) ;
#60067=CARTESIAN_POINT ( 'NONE',  ( 1.846868145590735200, -141.5000000013655779, -4.458734124999999437 ) ) ;
#60068=CARTESIAN_POINT ( 'NONE',  ( 2.499999999999998668, 24.66666666666666785, -4.330127018922193649 ) ) ;
#60070=CARTESIAN_POINT ( 'NONE',  ( 2.229367062499998831, -46.64583333196774362, -3.861377020970580887 ) ) ;
#60074=VECTOR ( 'NONE', #5780, 1000.000000000000227 ) ;
#60075=EDGE_CURVE ( 'NONE', #46520, #859, #1970, .T. ) ;
#60076=CARTESIAN_POINT ( 'NONE',  ( 1.846868145590735200, -141.5000000013655779, -4.458734125000000326 ) ) ;
#60078=EDGE_CURVE ( 'NONE', #31090, #44817, #28014, .T. ) ;
#60080=CARTESIAN_POINT ( 'NONE',  ( -1.339745962155613812, -53.20534180126147561, -5.000000000000000000 ) ) ;
#60082=CARTESIAN_POINT ( 'NONE',  ( -2.229367062500000163, -75.72916666530106511, -3.861377020970580443 ) ) ;
#60087=CARTESIAN_POINT ( 'NONE',  ( 3.061616997868383141E-16, -159.7500000000000000, -5.000000000000000000 ) ) ;
#60093=CARTESIAN_POINT ( 'NONE',  ( 4.458734124999998549, 17.02083333469892779, -2.574251347313721627 ) ) ;
#60095=( BOUNDED_CURVE ( )  B_SPLINE_CURVE ( 2, ( #62374, #14407, #42415, #62058, #3514, #57551, #24072, #38240, #18297 ),
 .UNSPECIFIED., .F., .F. ) 
 B_SPLINE_CURVE_WITH_KNOTS ( ( 3, 2, 2, 2, 3 ),
 ( 0.6104166666666667185, 0.6111111111111111605, 0.6125000000000000444, 0.6138888888888889284, 0.6145833333333333703 ),
 .UNSPECIFIED. ) 
 CURVE ( )  GEOMETRIC_REPRESENTATION_ITEM ( )  RATIONAL_B_SPLINE_CURVE ( ( 0.9330127018922194093, 0.9330127018922194093, 1.000000000000000000, 0.8660254037844387076, 1.000000000000000000, 0.8660254037844387076, 1.000000000000000000, 0.9330127018922194093, 0.9330127018922194093 ) ) 
 REPRESENTATION_ITEM ( '' )  );
#60100=DIRECTION ( 'NONE',  ( 0.000000000000000000, 0.000000000000000000, 1.000000000000000000 ) ) ;
#60101=CARTESIAN_POINT ( 'NONE',  ( -4.458734124999998549, -84.22916666530107932, 2.574251347313722516 ) ) ;
#60102=CARTESIAN_POINT ( 'NONE',  ( -2.229367062499996610, -1.145833331967736957, 3.861377020970582219 ) ) ;
#60105=CARTESIAN_POINT ( 'NONE',  ( 9.457646018065525792E-16, -32.31249999863440792, 5.148502694627439702 ) ) ;
#60109=CARTESIAN_POINT ( 'NONE',  ( 2.229367062500001939, 20.02083333469892779, 3.861377020970579999 ) ) ;
#60111=CARTESIAN_POINT ( 'NONE',  ( 1.062108568985190270E-13, -10.25000000000000355, -4.999999999999999112 ) ) ;
#60112=CARTESIAN_POINT ( 'NONE',  ( 2.229367062499998831, -80.89583333196773651, -3.861377020970580887 ) ) ;
#60114=CYLINDRICAL_SURFACE ( 'NONE', #12077, 5.000000000000000000 ) ;
#60115=CARTESIAN_POINT ( 'NONE',  ( 2.500000000000002220, 24.45833333606451987, 4.330127018922192761 ) ) ;
#60116=ORIENTED_EDGE ( 'NONE', *, *, #37074, .F. ) ;
#60119=CARTESIAN_POINT ( 'NONE',  ( 0.000000000000000000, -170.0000000000000000, 0.000000000000000000 ) ) ;
#60120=CARTESIAN_POINT ( 'NONE',  ( 5.000000000000000888, -21.58333333333332860, 2.886751345948126879 ) ) ;
#60121=CARTESIAN_POINT ( 'NONE',  ( -4.458734124999999437, -27.31249999863440081, 0.000000000000000000 ) ) ;
#60122=CARTESIAN_POINT ( 'NONE',  ( -2.229367062500000163, -88.47916666530106511, -3.861377020970580443 ) ) ;
#60124=CARTESIAN_POINT ( 'NONE',  ( -5.000000000000000000, -21.95833333060214798, -2.886751345948128211 ) ) ;
#60125=CARTESIAN_POINT ( 'NONE',  ( 4.458734124999998549, -57.72916666530107221, -2.574251347313721627 ) ) ;
#60127=CARTESIAN_POINT ( 'NONE',  ( 1.975475456537005874E-15, -27.74999999999999645, 5.000000000000000000 ) ) ;
#60129=CARTESIAN_POINT ( 'NONE',  ( 4.458734125000001214, -6.145833331967741842, 2.574251347313718519 ) ) ;
#60132=CARTESIAN_POINT ( 'NONE',  ( -5.000000000000000000, -67.99999999999998579, 0.000000000000000000 ) ) ;
#60133=CARTESIAN_POINT ( 'NONE',  ( 4.458734125000000326, -150.6250000013655779, -1.846868145590734978 ) ) ;
#60136=CARTESIAN_POINT ( 'NONE',  ( 3.535533905932738197, -158.8750000000000284, -3.535533905932738197 ) ) ;
#60137=CARTESIAN_POINT ( 'NONE',  ( 0.000000000000000000, -170.0000000000000000, 0.000000000000000000 ) ) ;
#60140=CARTESIAN_POINT ( 'NONE',  ( -4.458734124999999437, -8.562499998634406140, 0.000000000000000000 ) ) ;
#60141=CARTESIAN_POINT ( 'NONE',  ( 4.458734124999999437, -51.06249999863440792, -5.460374474430324690E-16 ) ) ;
#60143=CARTESIAN_POINT ( 'NONE',  ( 4.458734124999999437, -143.4375000013656063, 0.000000000000000000 ) ) ;
#60145=CARTESIAN_POINT ( 'NONE',  ( 0.000000000000000000, -170.0000000000000000, 5.000000000000000000 ) ) ;
#60146=( BOUNDED_CURVE ( )  B_SPLINE_CURVE ( 2, ( #42009, #12744, #13061, #4352, #23038, #38439, #18204, #14314, #32680 ),
 .UNSPECIFIED., .F., .F. ) 
 B_SPLINE_CURVE_WITH_KNOTS ( ( 3, 2, 2, 2, 3 ),
 ( 0.7437500000000000222, 0.7444444444444444642, 0.7458333333333333481, 0.7472222222222222321, 0.7479166666666666741 ),
 .UNSPECIFIED. ) 
 CURVE ( )  GEOMETRIC_REPRESENTATION_ITEM ( )  RATIONAL_B_SPLINE_CURVE ( ( 0.9330127018922194093, 0.9330127018922194093, 1.000000000000000000, 0.8660254037844387076, 1.000000000000000000, 0.8660254037844387076, 1.000000000000000000, 0.9330127018922194093, 0.9330127018922194093 ) ) 
 REPRESENTATION_ITEM ( '' )  );
#60147=ORIENTED_EDGE ( 'NONE', *, *, #50340, .F. ) ;
#60148=DIRECTION ( 'NONE',  ( -0.000000000000000000, 1.000000000000000000, -0.000000000000000000 ) ) ;
#60149=CARTESIAN_POINT ( 'NONE',  ( 4.458734124999998549, 25.02083333469892423, -2.574251347313721627 ) ) ;
#60155=CARTESIAN_POINT ( 'NONE',  ( 0.000000000000000000, -170.0000000000000000, 0.000000000000000000 ) ) ;
#60157=EDGE_CURVE ( 'NONE', #14479, #12628, #50794, .T. ) ;
#60159=CARTESIAN_POINT ( 'NONE',  ( 4.458734125000001214, -7.895833331967735624, 2.574251347313718519 ) ) ;
#60162=CARTESIAN_POINT ( 'NONE',  ( -1.846868145590734756, -147.1250000013656063, -4.458734124999999437 ) ) ;
#60164=ORIENTED_EDGE ( 'NONE', *, *, #28411, .T. ) ;
#60165=DIRECTION ( 'NONE',  ( -0.000000000000000000, 1.000000000000000000, -0.000000000000000000 ) ) ;
#60168=CARTESIAN_POINT ( 'NONE',  ( 5.000000000000000888, -85.45833333060213022, 2.886751345948126879 ) ) ;
#60176=CARTESIAN_POINT ( 'NONE',  ( -4.458734124999999437, 13.68750000136559386, 0.000000000000000000 ) ) ;
#60178=CARTESIAN_POINT ( 'NONE',  ( 9.457646018065525792E-16, -16.31249999863440436, 5.148502694627439702 ) ) ;
#60180=CARTESIAN_POINT ( 'NONE',  ( -8.190561711645485556E-16, -164.6875000013655779, 4.458734124999999437 ) ) ;
#60188=CARTESIAN_POINT ( 'NONE',  ( -4.458734124999999437, -35.31249999863440792, 0.000000000000000000 ) ) ;
#60190=CARTESIAN_POINT ( 'NONE',  ( -3.152801135295367096, -150.3125000013655779, -3.152801135295367541 ) ) ;
#60192=CARTESIAN_POINT ( 'NONE',  ( -6.972266317189433020E-16, -58.12499999726880162, -5.000000000000000000 ) ) ;
#60199=CARTESIAN_POINT ( 'NONE',  ( -2.500000000000000444, -9.041666663935483683, -4.330127018922193649 ) ) ;
#60200=CARTESIAN_POINT ( 'NONE',  ( 5.000000000000000000, -0.4166666666666659080, -2.886751345948129988 ) ) ;
#60201=CARTESIAN_POINT ( 'NONE',  ( 2.229367062499998831, -68.64583333196773651, -3.861377020970580887 ) ) ;
#60202=CARTESIAN_POINT ( 'NONE',  ( -5.000000000000000000, -17.00000000000000000, 0.000000000000000000 ) ) ;
#60203=CARTESIAN_POINT ( 'NONE',  ( -2.499999999999996447, -5.708333330602148870, 4.330127018922195425 ) ) ;
#60204=CARTESIAN_POINT ( 'NONE',  ( 4.458734124999998549, -36.72916666530107221, -2.574251347313721627 ) ) ;
#60205=ORIENTED_EDGE ( 'NONE', *, *, #18363, .T. ) ;
#60206=CARTESIAN_POINT ( 'NONE',  ( 4.458734124999999437, 12.93750000136559208, -5.460374474430324690E-16 ) ) ;
#60207=ORIENTED_EDGE ( 'NONE', *, *, #55529, .T. ) ;
#60209=CARTESIAN_POINT ( 'NONE',  ( -2.500000000000000444, -49.16666666666666430, -4.330127018922193649 ) ) ;
#60211=CARTESIAN_POINT ( 'NONE',  ( 1.339745962155565406, -4.705341801261480050, 5.000000000000028422 ) ) ;
#60212=CARTESIAN_POINT ( 'NONE',  ( 9.457646018065525792E-16, -77.06249999863440792, 5.148502694627439702 ) ) ;
#60213=CARTESIAN_POINT ( 'NONE',  ( -8.190561711645485556E-16, -139.9375000013656063, 4.458734124999999437 ) ) ;
#60214=CARTESIAN_POINT ( 'NONE',  ( -4.458734124999998549, -83.22916666530106511, 2.574251347313722516 ) ) ;
#60216=CARTESIAN_POINT ( 'NONE',  ( -4.458734124999999437, -37.56249999863440792, 0.000000000000000000 ) ) ;
#60218=ORIENTED_EDGE ( 'NONE', *, *, #29190, .F. ) ;
#60227=CARTESIAN_POINT ( 'NONE',  ( 3.061616997868383141E-16, -163.8750000027311842, -5.000000000000000000 ) ) ;
#60228=CARTESIAN_POINT ( 'NONE',  ( 4.458734124999999437, -65.06249999863440792, -5.460374474430324690E-16 ) ) ;
#60232=CARTESIAN_POINT ( 'NONE',  ( 5.000000000000000000, 3.625000002731186388, -6.123233995736766282E-16 ) ) ;
#60233=CARTESIAN_POINT ( 'NONE',  ( -1.339745962155610925, 5.330341803992665994, 5.000000000000000000 ) ) ;
#60237=CARTESIAN_POINT ( 'NONE',  ( -3.152548672688508926E-16, 7.437500001365594748, -5.148502694627439702 ) ) ;
#60238=CARTESIAN_POINT ( 'NONE',  ( 5.000000000000000888, -153.9375000000000000, -2.071067811865475505 ) ) ;
#60239=CARTESIAN_POINT ( 'NONE',  ( 4.458734124999999437, -159.4375000013655779, 0.000000000000000000 ) ) ;
#60240=CYLINDRICAL_SURFACE ( 'NONE', #25524, 5.000000000000000000 ) ;
#60241=ORIENTED_EDGE ( 'NONE', *, *, #826, .T. ) ;
#60243=EDGE_CURVE ( 'NONE', #56895, #14032, #59754, .T. ) ;
#60247=CARTESIAN_POINT ( 'NONE',  ( -5.000000000000000000, -68.08333333333332860, -2.886751345948128211 ) ) ;
#60250=CARTESIAN_POINT ( 'NONE',  ( 1.975475456537005874E-15, 12.37500000273118417, 5.000000000000000000 ) ) ;
#60251=CARTESIAN_POINT ( 'NONE',  ( 0.000000000000000000, -170.0000000000000000, 5.000000000000000000 ) ) ;
#60253=CARTESIAN_POINT ( 'NONE',  ( -2.229367062500000163, 26.52083333469892779, -3.861377020970580443 ) ) ;
#60256=CARTESIAN_POINT ( 'NONE',  ( -4.458734124999999437, 3.354166668032260823, -2.574251347313719407 ) ) ;
#60257=VECTOR ( 'NONE', #57587, 1000.000000000000000 ) ;
#60258=CARTESIAN_POINT ( 'NONE',  ( 1.975475456537005874E-15, -0.6249999972688137229, 5.000000000000000000 ) ) ;
#60260=CARTESIAN_POINT ( 'NONE',  ( -5.000000000000000888, -143.5625000027311842, 2.071067811865474617 ) ) ;
#60265=CARTESIAN_POINT ( 'NONE',  ( 5.000000000000000000, -141.0000000000000000, 0.000000000000000000 ) ) ;
#60266=CARTESIAN_POINT ( 'NONE',  ( 2.071067811865517694, -140.9375000027311557, -4.999999999999958256 ) ) ;
#60268=CARTESIAN_POINT ( 'NONE',  ( -4.458734125000000326, -162.1250000013656347, 1.846868145590734089 ) ) ;
#60269=CARTESIAN_POINT ( 'NONE',  ( -5.000000000000000888, -159.6875000027312126, -2.071067811865475949 ) ) ;
#60271=CARTESIAN_POINT ( 'NONE',  ( -2.499999999999996447, -56.83333333333333570, 4.330127018922195425 ) ) ;
#60272=ORIENTED_EDGE ( 'NONE', *, *, #35911, .F. ) ;
#60273=CARTESIAN_POINT ( 'NONE',  ( 2.229367062500001939, 24.77083333469892779, 3.861377020970579999 ) ) ;
#60276=CARTESIAN_POINT ( 'NONE',  ( -3.535250795749689387E-16, 12.75000000000000000, -5.773502691896257311 ) ) ;
#60277=( BOUNDED_CURVE ( )  B_SPLINE_CURVE ( 2, ( #61890, #19294, #32281, #48250, #27452, #61571, #41601, #27147, #38912 ),
 .UNSPECIFIED., .F., .F. ) 
 B_SPLINE_CURVE_WITH_KNOTS ( ( 3, 2, 2, 2, 3 ),
 ( 0.2145833333333333481, 0.2152777777777777901, 0.2166666666666666741, 0.2180555555555555580, 0.2187500000000000000 ),
 .UNSPECIFIED. ) 
 CURVE ( )  GEOMETRIC_REPRESENTATION_ITEM ( )  RATIONAL_B_SPLINE_CURVE ( ( 0.9330127018922194093, 0.9330127018922207416, 1.000000000000000000, 0.8660254037844387076, 1.000000000000000000, 0.8660254037844387076, 1.000000000000000000, 0.9330127018922194093, 0.9330127018922194093 ) ) 
 REPRESENTATION_ITEM ( '' )  );
#60278=CARTESIAN_POINT ( 'NONE',  ( -4.458734124999997661, -50.22916666530107221, 2.574251347313722516 ) ) ;
#60279=CARTESIAN_POINT ( 'NONE',  ( 9.457646018065525792E-16, -13.06249999863440259, 5.148502694627439702 ) ) ;
#60281=CARTESIAN_POINT ( 'NONE',  ( -6.972266317189433020E-16, -64.12499999726880162, -5.000000000000000000 ) ) ;
#60283=CARTESIAN_POINT ( 'NONE',  ( -2.499999999999996447, -32.83333333333332860, 4.330127018922195425 ) ) ;
#60285=CARTESIAN_POINT ( 'NONE',  ( 1.975475456537005874E-15, -55.62499999726880873, 5.000000000000000000 ) ) ;
#60288=CARTESIAN_POINT ( 'NONE',  ( -2.229367062499996610, -58.14583333196773651, 3.861377020970582219 ) ) ;
#60289=CARTESIAN_POINT ( 'NONE',  ( -8.190561711645485556E-16, -151.9375000013655779, 4.458734124999999437 ) ) ;
#60290=CARTESIAN_POINT ( 'NONE',  ( 4.458734124999999437, -66.81249999863440792, -5.460374474430324690E-16 ) ) ;
#60291=( BOUNDED_CURVE ( )  B_SPLINE_CURVE ( 2, ( #39805, #10541, #5727, #44964, #16648, #31755, #27871, #17279, #60726 ),
 .UNSPECIFIED., .F., .F. ) 
 B_SPLINE_CURVE_WITH_KNOTS ( ( 3, 2, 2, 2, 3 ),
 ( 0.3645833333333333148, 0.3652777777777777568, 0.3666666666666666408, 0.3680555555555555802, 0.3687500000000000222 ),
 .UNSPECIFIED. ) 
 CURVE ( )  GEOMETRIC_REPRESENTATION_ITEM ( )  RATIONAL_B_SPLINE_CURVE ( ( 0.9330127018922194093, 0.9330127018922194093, 1.000000000000000000, 0.8660254037844387076, 1.000000000000000000, 0.8660254037844387076, 1.000000000000000000, 0.9330127018922194093, 0.9330127018922194093 ) ) 
 REPRESENTATION_ITEM ( '' )  );
#60292=CARTESIAN_POINT ( 'NONE',  ( 2.499999999999998668, -57.20833333060214443, -4.330127018922193649 ) ) ;
#60293=ORIENTED_EDGE ( 'NONE', *, *, #20924, .T. ) ;
#60298=CARTESIAN_POINT ( 'NONE',  ( -1.846868145590734756, -154.1250000013656063, -4.458734125000000326 ) ) ;
#60302=CARTESIAN_POINT ( 'NONE',  ( 5.000000000000000000, -80.29166666393547303, -2.886751345948130876 ) ) ;
#60303=CARTESIAN_POINT ( 'NONE',  ( -2.229367062499996610, -46.39583333196774362, 3.861377020970582219 ) ) ;
#60304=VECTOR ( 'NONE', #20448, 1000.000000000000000 ) ;
#60306=VECTOR ( 'NONE', #56853, 1000.000000000000000 ) ;
#60310=CARTESIAN_POINT ( 'NONE',  ( -3.152548672688508926E-16, 23.43750000136559564, -5.148502694627439702 ) ) ;
#60320=EDGE_CURVE ( 'NONE', #63065, #62891, #43435, .T. ) ;
#60331=CARTESIAN_POINT ( 'NONE',  ( 2.071067811865476394, -157.3125000027312126, 5.000000000000000000 ) ) ;
#60341=CARTESIAN_POINT ( 'NONE',  ( 2.229367062499998831, -20.64583333196774007, -3.861377020970580887 ) ) ;
#60342=DIRECTION ( 'NONE',  ( 0.000000000000000000, 0.000000000000000000, 1.000000000000000000 ) ) ;
#60343=CARTESIAN_POINT ( 'NONE',  ( 5.000000000000000888, -149.9375000000000000, -2.071067811865475505 ) ) ;
#60345=CARTESIAN_POINT ( 'NONE',  ( -4.458734125000001214, -151.8750000013655779, 1.846868145590734089 ) ) ;
#60346=VERTEX_POINT ( 'NONE', #54275 ) ;
#60347=CARTESIAN_POINT ( 'NONE',  ( 4.458734124999999437, -48.06249999863440792, -5.460374474430324690E-16 ) ) ;
#60351=CARTESIAN_POINT ( 'NONE',  ( -6.972266317189433020E-16, -52.12499999726880873, -5.000000000000000000 ) ) ;
#60352=CARTESIAN_POINT ( 'NONE',  ( 1.060575238724906964E-15, 27.25000000000000000, 5.773502691896257311 ) ) ;
#60354=CARTESIAN_POINT ( 'NONE',  ( -3.152548672688508926E-16, 3.437500001365594748, -5.148502694627439702 ) ) ;
#60356=VECTOR ( 'NONE', #45274, 1000.000000000000000 ) ;
#60357=DIRECTION ( 'NONE',  ( 0.000000000000000000, 0.000000000000000000, 1.000000000000000000 ) ) ;
#60359=CARTESIAN_POINT ( 'NONE',  ( -3.152548672688508926E-16, 13.18750000136559208, -5.148502694627439702 ) ) ;
#60361=CARTESIAN_POINT ( 'NONE',  ( -2.500000000000000444, 7.958333336064518093, -4.330127018922193649 ) ) ;
#60362=ORIENTED_EDGE ( 'NONE', *, *, #32193, .F. ) ;
#60366=CARTESIAN_POINT ( 'NONE',  ( 4.458734125000001214, -44.89583333196774362, 2.574251347313718519 ) ) ;
#60367=CARTESIAN_POINT ( 'NONE',  ( -1.846868145590734756, -165.3750000013656347, -4.458734125000000326 ) ) ;
#60368=EDGE_CURVE ( 'NONE', #27206, #15666, #37265, .T. ) ;
#60369=CARTESIAN_POINT ( 'NONE',  ( -5.000000000000000000, -39.87499999726880162, 0.000000000000000000 ) ) ;
#60370=ORIENTED_EDGE ( 'NONE', *, *, #62495, .F. ) ;
#60371=CARTESIAN_POINT ( 'NONE',  ( 2.229367062499998831, -15.64583333196773651, -3.861377020970580887 ) ) ;
#60372=VERTEX_POINT ( 'NONE', #55571 ) ;
#60373=CARTESIAN_POINT ( 'NONE',  ( -2.499999999999996447, -86.83333333333332860, 4.330127018922195425 ) ) ;
#60374=CARTESIAN_POINT ( 'NONE',  ( 2.730187237215162345E-16, -168.1875000013655779, -4.458734124999999437 ) ) ;
#60375=CARTESIAN_POINT ( 'NONE',  ( 1.060575238724906964E-15, -87.62499999726880162, 5.773502691896257311 ) ) ;
#60377=ORIENTED_EDGE ( 'NONE', *, *, #56635, .T. ) ;
#60379=CARTESIAN_POINT ( 'NONE',  ( 4.458734125000001214, -35.14583333196772941, 2.574251347313718519 ) ) ;
#60380=CARTESIAN_POINT ( 'NONE',  ( 2.499999999999998668, -5.208333330602148870, -4.330127018922193649 ) ) ;
#60386=CARTESIAN_POINT ( 'NONE',  ( 6.123233995736766282E-16, -170.0000000000000000, -5.000000000000000000 ) ) ;
#60388=CARTESIAN_POINT ( 'NONE',  ( -3.152548672688508926E-16, -81.81249999863440792, -5.148502694627439702 ) ) ;
#60391=CARTESIAN_POINT ( 'NONE',  ( 4.458734124999999437, -143.6875000013656063, 0.000000000000000000 ) ) ;
#60392=AXIS2_PLACEMENT_3D ( 'NONE', #43985, #19552, #36822 ) ;
#60393=CARTESIAN_POINT ( 'NONE',  ( -1.339745962155610925, -57.79465819873852439, 5.000000000000000000 ) ) ;
#60395=CARTESIAN_POINT ( 'NONE',  ( 2.229367062500001939, -46.97916666530106511, 3.861377020970579999 ) ) ;
#60397=VECTOR ( 'NONE', #56559, 1000.000000000000000 ) ;
#60405=CARTESIAN_POINT ( 'NONE',  ( 4.458734124999999437, -78.06249999863440792, -5.460374474430324690E-16 ) ) ;
#60408=VERTEX_POINT ( 'NONE', #6361 ) ;
#60415=CARTESIAN_POINT ( 'NONE',  ( 4.458734125000000326, 18.85416666803225993, 2.574251347313718519 ) ) ;
#60416=CYLINDRICAL_SURFACE ( 'NONE', #46936, 5.000000000000000000 ) ;
#60422=CARTESIAN_POINT ( 'NONE',  ( 2.229367062500001939, -86.97916666530107932, 3.861377020970579999 ) ) ;
#60423=CARTESIAN_POINT ( 'NONE',  ( -3.152548672688508926E-16, -1.562499998634406140, -5.148502694627439702 ) ) ;
#60426=CARTESIAN_POINT ( 'NONE',  ( -4.458734124999997661, -31.47916666530107577, 2.574251347313722516 ) ) ;
#60430=EDGE_CURVE ( 'NONE', #35906, #25520, #6836, .T. ) ;
#60431=CARTESIAN_POINT ( 'NONE',  ( 9.457646018065525792E-16, 20.93750000136558853, 5.148502694627439702 ) ) ;
#60432=CARTESIAN_POINT ( 'NONE',  ( 1.339745962155615144, -53.70534180126147561, 4.999999999999999112 ) ) ;
#60433=CARTESIAN_POINT ( 'NONE',  ( 2.499999999999998668, -28.33333333333333570, -4.330127018922193649 ) ) ;
#60434=CARTESIAN_POINT ( 'NONE',  ( -2.229367062499996610, -76.39583333196773651, 3.861377020970582219 ) ) ;
#60436=CARTESIAN_POINT ( 'NONE',  ( -9.184850993605147944E-16, -143.2500000000000284, 5.000000000000000000 ) ) ;
#60437=CARTESIAN_POINT ( 'NONE',  ( 5.000000000000000000, 22.62500000273118772, -6.123233995736766282E-16 ) ) ;
#60438=EDGE_LOOP ( 'NONE', ( #1797, #14966, #36165, #52388 ) ) ;
#60440=VECTOR ( 'NONE', #25649, 1000.000000000000000 ) ;
#60441=CARTESIAN_POINT ( 'NONE',  ( 0.000000000000000000, -170.0000000000000000, 0.000000000000000000 ) ) ;
#60442=CARTESIAN_POINT ( 'NONE',  ( 5.000000000000000000, -0.4166666666666659080, -2.886751345948130876 ) ) ;
#60443=CARTESIAN_POINT ( 'NONE',  ( -3.535250795749689387E-16, -22.24999999999999645, -5.773502691896257311 ) ) ;
#60444=CARTESIAN_POINT ( 'NONE',  ( 4.458734125000001214, -28.89583333196774007, 2.574251347313718519 ) ) ;
#60445=CARTESIAN_POINT ( 'NONE',  ( -2.229367062499996610, -89.14583333196773651, 3.861377020970582219 ) ) ;
#60446=CARTESIAN_POINT ( 'NONE',  ( 5.000000000000000000, -22.37499999726881228, -6.123233995736766282E-16 ) ) ;
#60447=CARTESIAN_POINT ( 'NONE',  ( 4.458734125000001214, -57.89583333196773651, 2.574251347313718519 ) ) ;
#60449=CARTESIAN_POINT ( 'NONE',  ( 2.499999999999998668, -49.33333333333332860, -4.330127018922193649 ) ) ;
#60451=CARTESIAN_POINT ( 'NONE',  ( -2.229367062499996610, -3.395833331967738733, 3.861377020970582219 ) ) ;
#60453=CARTESIAN_POINT ( 'NONE',  ( 1.060575238724906964E-15, -72.74999999999998579, 5.773502691896257311 ) ) ;
#60454=CARTESIAN_POINT ( 'NONE',  ( -8.190561711645485556E-16, -150.9375000013656063, 4.458734124999999437 ) ) ;
#60457=CARTESIAN_POINT ( 'NONE',  ( 2.071067811865475505, -158.8125000000000284, -5.000000000000000888 ) ) ;
#60458=CARTESIAN_POINT ( 'NONE',  ( -1.339745962155610925, -85.79465819873851729, 5.000000000000000000 ) ) ;
#60460=CARTESIAN_POINT ( 'NONE',  ( 4.458734124999998549, -14.97916666530107221, -2.574251347313721627 ) ) ;
#60462=CARTESIAN_POINT ( 'NONE',  ( -2.229367062499996610, -53.39583333196773651, 3.861377020970582219 ) ) ;
#60464=CARTESIAN_POINT ( 'NONE',  ( 2.730187237215162345E-16, -144.1875000013656063, -4.458734124999999437 ) ) ;
#60469=CARTESIAN_POINT ( 'NONE',  ( 2.229367062499998831, 25.10416666803225993, -3.861377020970580887 ) ) ;
#60471=CARTESIAN_POINT ( 'NONE',  ( 5.000000000000000000, -50.50000000000000000, -6.123233995736766282E-16 ) ) ;
#60472=ORIENTED_EDGE ( 'NONE', *, *, #16531, .F. ) ;
#60477=FACE_OUTER_BOUND ( 'NONE', #53610, .T. ) ;
#60478=CARTESIAN_POINT ( 'NONE',  ( 2.229367062499998831, -8.645833331967736513, -3.861377020970580887 ) ) ;
#60479=CARTESIAN_POINT ( 'NONE',  ( 5.000000000000000000, 6.625000002731185944, -6.123233995736766282E-16 ) ) ;
#60480=CARTESIAN_POINT ( 'NONE',  ( -1.846868145590734756, -150.1250000013655779, -4.458734124999999437 ) ) ;
#60485=VECTOR ( 'NONE', #43484, 1000.000000000000000 ) ;
#60489=CARTESIAN_POINT ( 'NONE',  ( 3.535533905932736864, -150.2500000027312126, 3.535533905932738641 ) ) ;
#60493=CARTESIAN_POINT ( 'NONE',  ( 2.229367062500001939, 11.02083333469892956, 3.861377020970579999 ) ) ;
#60495=CARTESIAN_POINT ( 'NONE',  ( 4.458734124999998549, -14.97916666530107399, -2.574251347313721627 ) ) ;
#60497=CARTESIAN_POINT ( 'NONE',  ( 1.846868145590736310, -163.6250000013656063, 4.458734124999999437 ) ) ;
#60505=CARTESIAN_POINT ( 'NONE',  ( 2.229367062500001939, -35.97916666530107221, 3.861377020970579999 ) ) ;
#60506=CARTESIAN_POINT ( 'NONE',  ( 2.499999999999998668, 19.79166666939785202, -4.330127018922193649 ) ) ;
#60510=ORIENTED_EDGE ( 'NONE', *, *, #23403, .F. ) ;
#60514=CARTESIAN_POINT ( 'NONE',  ( 1.060575238724906964E-15, -6.749999999999999112, 5.773502691896257311 ) ) ;
#60515=CARTESIAN_POINT ( 'NONE',  ( -4.458734124999999437, -73.39583333196772230, -2.574251347313719407 ) ) ;
#60516=CARTESIAN_POINT ( 'NONE',  ( 1.975475456537005874E-15, 14.25000000000000000, 5.000000000000000000 ) ) ;
#60518=CARTESIAN_POINT ( 'NONE',  ( 5.000000000000000888, -7.458333330602143540, 2.886751345948126879 ) ) ;
#60519=CARTESIAN_POINT ( 'NONE',  ( -4.458734124999999437, -37.39583333196773651, -2.574251347313719407 ) ) ;
#60523=CARTESIAN_POINT ( 'NONE',  ( -2.229367062499996610, 14.60416666803226171, 3.861377020970582219 ) ) ;
#60524=ORIENTED_EDGE ( 'NONE', *, *, #20143, .F. ) ;
#60525=( BOUNDED_CURVE ( )  B_SPLINE_CURVE ( 2, ( #45571, #59423, #25318, #44290, #35289, #59100, #25638, #30452, #50077 ),
 .UNSPECIFIED., .F., .F. ) 
 B_SPLINE_CURVE_WITH_KNOTS ( ( 3, 2, 2, 2, 3 ),
 ( 0.5645833333333333259, 0.5652777777777777679, 0.5666666666666666519, 0.5680555555555555358, 0.5687499999999999778 ),
 .UNSPECIFIED. ) 
 CURVE ( )  GEOMETRIC_REPRESENTATION_ITEM ( )  RATIONAL_B_SPLINE_CURVE ( ( 0.9330127018922194093, 0.9330127018922194093, 1.000000000000000000, 0.8660254037844387076, 1.000000000000000000, 0.8660254037844387076, 1.000000000000000000, 0.9330127018922194093, 0.9330127018922194093 ) ) 
 REPRESENTATION_ITEM ( '' )  );
#60527=CARTESIAN_POINT ( 'NONE',  ( -5.000000000000000000, -50.08333333333332149, -2.886751345948128211 ) ) ;
#60530=CARTESIAN_POINT ( 'NONE',  ( 1.339745962155612702, -4.294658198738519062, -5.000000000000000000 ) ) ;
#60531=CARTESIAN_POINT ( 'NONE',  ( 4.458734125000001214, -77.89583333196773651, 2.574251347313718519 ) ) ;
#60532=CARTESIAN_POINT ( 'NONE',  ( 1.846868145590735200, -141.5000000013655779, -4.458734125000000326 ) ) ;
#60533=CARTESIAN_POINT ( 'NONE',  ( 4.458734125000001214, -88.89583333196773651, 2.574251347313718519 ) ) ;
#60537=CARTESIAN_POINT ( 'NONE',  ( 2.229367062500001939, -38.22916666530107221, 3.861377020970579999 ) ) ;
#60539=VERTEX_POINT ( 'NONE', #43585 ) ;
#60543=CARTESIAN_POINT ( 'NONE',  ( -6.972266317189433020E-16, -4.124999997268814056, -5.000000000000000000 ) ) ;
#60544=CYLINDRICAL_SURFACE ( 'NONE', #7551, 5.000000000000000000 ) ;
#60545=CARTESIAN_POINT ( 'NONE',  ( 2.229367062500001939, -64.22916666530106511, 3.861377020970579999 ) ) ;
#60547=ORIENTED_EDGE ( 'NONE', *, *, #58924, .F. ) ;
#60549=FACE_OUTER_BOUND ( 'NONE', #18053, .T. ) ;
#60553=CARTESIAN_POINT ( 'NONE',  ( 4.458734124999999437, 7.187500001365594748, -5.460374474430324690E-16 ) ) ;
#60554=CARTESIAN_POINT ( 'NONE',  ( -1.339745962155613812, -33.08034179853029144, -5.000000000000000000 ) ) ;
#60555=CARTESIAN_POINT ( 'NONE',  ( 1.846868145590735200, -162.2500000013656063, -4.458734124999999437 ) ) ;
#60556=CARTESIAN_POINT ( 'NONE',  ( 0.000000000000000000, -170.0000000000000000, 5.000000000000000000 ) ) ;
#60557=ORIENTED_EDGE ( 'NONE', *, *, #63292, .F. ) ;
#60561=CARTESIAN_POINT ( 'NONE',  ( 2.500000000000002220, -71.54166666393547303, 4.330127018922192761 ) ) ;
#60565=CARTESIAN_POINT ( 'NONE',  ( 4.458734124999999437, 28.18750000136559208, -5.460374474430324690E-16 ) ) ;
#60568=CARTESIAN_POINT ( 'NONE',  ( -3.152548672688508926E-16, 0.1875000013655953035, -5.148502694627439702 ) ) ;
#60571=LINE ( 'NONE', #51237, #55562 ) ;
#60573=CARTESIAN_POINT ( 'NONE',  ( -9.184850993605147944E-16, -145.3750000027312126, 5.000000000000000000 ) ) ;
#60574=CARTESIAN_POINT ( 'NONE',  ( 5.000000000000000000, -159.0000000000000000, 0.000000000000000000 ) ) ;
#60580=CARTESIAN_POINT ( 'NONE',  ( -5.000000000000000888, -140.5625000000000000, -2.071067811865475949 ) ) ;
#60581=ADVANCED_FACE ( 'NONE', ( #9492 ), #29984, .T. ) ;
#60583=EDGE_CURVE ( 'NONE', #63065, #1762, #44779, .T. ) ;
#60585=CARTESIAN_POINT ( 'NONE',  ( 4.458734124999999437, -160.6250000013656063, -1.846868145590734978 ) ) ;
#60588=CARTESIAN_POINT ( 'NONE',  ( -3.152801135295367096, -140.0625000013655779, -3.152801135295367541 ) ) ;
#60589=ORIENTED_EDGE ( 'NONE', *, *, #49598, .F. ) ;
#60590=CARTESIAN_POINT ( 'NONE',  ( -4.458734124999999437, 23.35416666803226349, -2.574251347313719407 ) ) ;
#60591=ORIENTED_EDGE ( 'NONE', *, *, #16209, .F. ) ;
#60596=CARTESIAN_POINT ( 'NONE',  ( 2.500000000000002220, 8.333333333333332149, 4.330127018922192761 ) ) ;
#60597=EDGE_CURVE ( 'NONE', #2792, #10271, #39949, .T. ) ;
#60598=CARTESIAN_POINT ( 'NONE',  ( 4.458734124999999437, -56.81249999863440081, -5.460374474430324690E-16 ) ) ;
#60599=CARTESIAN_POINT ( 'NONE',  ( -4.458734124999999437, -9.312499998634406140, 0.000000000000000000 ) ) ;
#60602=CARTESIAN_POINT ( 'NONE',  ( -5.000000000000000000, 13.99999999999999822, 0.000000000000000000 ) ) ;
#60603=CARTESIAN_POINT ( 'NONE',  ( -6.972266317189433020E-16, -64.24999999999998579, -5.000000000000000000 ) ) ;
#60604=ADVANCED_FACE ( 'NONE', ( #15530 ), #47481, .T. ) ;
#60606=CARTESIAN_POINT ( 'NONE',  ( 5.000000000000000000, -36.41666666666666430, -2.886751345948129988 ) ) ;
#60608=CARTESIAN_POINT ( 'NONE',  ( -2.499999999999996447, -33.83333333333332860, 4.330127018922195425 ) ) ;
#60611=CARTESIAN_POINT ( 'NONE',  ( 4.458734125000001214, -61.89583333196773651, 2.574251347313718519 ) ) ;
#60612=CARTESIAN_POINT ( 'NONE',  ( 1.846868145590736310, -153.8750000013655779, 4.458734124999999437 ) ) ;
#60613=CARTESIAN_POINT ( 'NONE',  ( -3.152548672688508926E-16, -71.56249999863440792, -5.148502694627439702 ) ) ;
#60615=CARTESIAN_POINT ( 'NONE',  ( -5.000000000000000000, -60.87499999726880873, 0.000000000000000000 ) ) ;
#60616=ORIENTED_EDGE ( 'NONE', *, *, #19300, .T. ) ;
#60617=CARTESIAN_POINT ( 'NONE',  ( -2.071067811865604735, -150.3125000000000284, 4.999999999999872990 ) ) ;
#60621=CARTESIAN_POINT ( 'NONE',  ( 4.458734124999999437, -153.4375000013655779, 0.000000000000000000 ) ) ;
#60623=CARTESIAN_POINT ( 'NONE',  ( 2.500000000000002220, -54.66666666666667140, 4.330127018922192761 ) ) ;
#60625=CARTESIAN_POINT ( 'NONE',  ( -9.184850993605147944E-16, -161.3750000027311842, 5.000000000000000000 ) ) ;
#60627=CARTESIAN_POINT ( 'NONE',  ( 4.458734124999998549, -47.97916666530107221, -2.574251347313721627 ) ) ;
#60628=ORIENTED_EDGE ( 'NONE', *, *, #54683, .F. ) ;
#60629=CARTESIAN_POINT ( 'NONE',  ( -3.535533905932738641, -145.3750000000000000, 3.535533905932737309 ) ) ;
#60631=CARTESIAN_POINT ( 'NONE',  ( -2.229367062500000163, 22.52083333469892423, -3.861377020970580443 ) ) ;
#60634=CARTESIAN_POINT ( 'NONE',  ( -2.500000000000000444, -36.04166666393547303, -4.330127018922193649 ) ) ;
#60647=CARTESIAN_POINT ( 'NONE',  ( -6.972266317189433020E-16, -5.124999997268812280, -5.000000000000000000 ) ) ;
#60649=CARTESIAN_POINT ( 'NONE',  ( -9.184850993605147944E-16, -158.3750000027311842, 5.000000000000000000 ) ) ;
#60650=ORIENTED_EDGE ( 'NONE', *, *, #49530, .T. ) ;
#60654=( BOUNDED_CURVE ( )  B_SPLINE_CURVE ( 2, ( #1708, #50255, #21314, #30953, #11644, #6204, #50579, #45112, #6522 ),
 .UNSPECIFIED., .F., .F. ) 
 B_SPLINE_CURVE_WITH_KNOTS ( ( 3, 2, 2, 2, 3 ),
 ( 0.02708333333333333426, 0.02777777777777777624, 0.02916666666666666713, 0.03055555555555555455, 0.03125000000000000000 ),
 .UNSPECIFIED. ) 
 CURVE ( )  GEOMETRIC_REPRESENTATION_ITEM ( )  RATIONAL_B_SPLINE_CURVE ( ( 0.9330127018922194093, 0.9330127018922195203, 1.000000000000000000, 0.8660254037844387076, 1.000000000000000000, 0.8660254037844387076, 1.000000000000000000, 0.9330127018922191873, 0.9330127018922194093 ) ) 
 REPRESENTATION_ITEM ( '' )  );
#60657=EDGE_CURVE ( 'NONE', #1513, #50070, #30948, .T. ) ;
#60660=CARTESIAN_POINT ( 'NONE',  ( -4.458734124999997661, -18.22916666530106866, 2.574251347313722516 ) ) ;
#60661=CARTESIAN_POINT ( 'NONE',  ( 5.000000000000000000, -147.0000000000000284, 0.000000000000000000 ) ) ;
#60662=CARTESIAN_POINT ( 'NONE',  ( 5.000000000000000000, -149.0625000000000000, 2.071067811865478614 ) ) ;
#60664=CARTESIAN_POINT ( 'NONE',  ( 4.458734124999999437, -151.5000000013655779, 1.846868145590737864 ) ) ;
#60665=EDGE_LOOP ( 'NONE', ( #60272, #62045, #20966, #51414 ) ) ;
#60667=CARTESIAN_POINT ( 'NONE',  ( 2.229367062500001939, -51.22916666530107221, 3.861377020970579999 ) ) ;
#60668=CARTESIAN_POINT ( 'NONE',  ( 1.339745962155565406, -2.705341801261481383, 5.000000000000028422 ) ) ;
#60670=CARTESIAN_POINT ( 'NONE',  ( -3.535250795749689387E-16, 29.74999999999999645, -5.773502691896257311 ) ) ;
#60673=CARTESIAN_POINT ( 'NONE',  ( -2.229367062499996610, 1.854166668032262377, 3.861377020970582219 ) ) ;
#60674=( BOUNDED_CURVE ( )  B_SPLINE_CURVE ( 2, ( #38040, #21988, #42228, #12336, #51578, #61872, #13598, #12956, #46742 ),
 .UNSPECIFIED., .F., .F. ) 
 B_SPLINE_CURVE_WITH_KNOTS ( ( 3, 2, 2, 2, 3 ),
 ( 0.4479166666666666852, 0.4486111111111111271, 0.4500000000000000111, 0.4513888888888888951, 0.4520833333333333370 ),
 .UNSPECIFIED. ) 
 CURVE ( )  GEOMETRIC_REPRESENTATION_ITEM ( )  RATIONAL_B_SPLINE_CURVE ( ( 0.9330127018922194093, 0.9330127018922194093, 1.000000000000000000, 0.8660254037844387076, 1.000000000000000000, 0.8660254037844387076, 1.000000000000000000, 0.9330127018922194093, 0.9330127018922194093 ) ) 
 REPRESENTATION_ITEM ( '' )  );
#60675=CARTESIAN_POINT ( 'NONE',  ( -6.972266317189433020E-16, -82.12499999726881583, -5.000000000000000000 ) ) ;
#60676=CARTESIAN_POINT ( 'NONE',  ( 2.499999999999998668, -17.33333333333333215, -4.330127018922193649 ) ) ;
#60677=CARTESIAN_POINT ( 'NONE',  ( -3.152548672688508926E-16, 15.18750000136559386, -5.148502694627439702 ) ) ;
#60678=CARTESIAN_POINT ( 'NONE',  ( 1.060575238724906964E-15, 4.375000002731186832, 5.773502691896257311 ) ) ;
#60682=ORIENTED_EDGE ( 'NONE', *, *, #43376, .F. ) ;
#60684=CARTESIAN_POINT ( 'NONE',  ( 9.457646018065525792E-16, -46.06249999863440081, 5.148502694627439702 ) ) ;
#60685=ADVANCED_FACE ( 'NONE', ( #40596 ), #2334, .T. ) ;
#60686=CARTESIAN_POINT ( 'NONE',  ( 3.152801135295366208, -163.8125000013656063, 3.152801135295367985 ) ) ;
#60687=ADVANCED_FACE ( 'NONE', ( #5878 ), #60240, .T. ) ;
#60688=CARTESIAN_POINT ( 'NONE',  ( 5.000000000000000000, -40.37499999726880162, -6.123233995736766282E-16 ) ) ;
#60690=CARTESIAN_POINT ( 'NONE',  ( 2.229367062499998831, -16.64583333196773651, -3.861377020970580887 ) ) ;
#60692=CARTESIAN_POINT ( 'NONE',  ( -3.535250795749689387E-16, -86.25000000000000000, -5.773502691896257311 ) ) ;
#60693=CARTESIAN_POINT ( 'NONE',  ( 4.458734125000000326, -165.3750000013656347, -1.846868145590734978 ) ) ;
#60694=CARTESIAN_POINT ( 'NONE',  ( -2.499999999999996447, -34.70833333060213732, 4.330127018922195425 ) ) ;
#60697=CARTESIAN_POINT ( 'NONE',  ( 4.458734124999998549, -32.97916666530106511, -2.574251347313721627 ) ) ;
#60698=CARTESIAN_POINT ( 'NONE',  ( -1.339745962155610925, -38.79465819873851729, 5.000000000000000000 ) ) ;
#60703=ORIENTED_EDGE ( 'NONE', *, *, #50764, .T. ) ;
#60704=CARTESIAN_POINT ( 'NONE',  ( -3.535533905932737309, -161.6250000000000284, -3.535533905932738197 ) ) ;
#60707=CARTESIAN_POINT ( 'NONE',  ( 4.458734125000001214, -80.14583333196773651, 2.574251347313718519 ) ) ;
#60710=CARTESIAN_POINT ( 'NONE',  ( 4.458734124999997661, -143.7500000013655779, 1.846868145590737864 ) ) ;
#60712=CARTESIAN_POINT ( 'NONE',  ( 2.229367062500001939, -43.97916666530106511, 3.861377020970579999 ) ) ;
#60714=CARTESIAN_POINT ( 'NONE',  ( 1.975475456537005874E-15, -3.750000000000001776, 5.000000000000000000 ) ) ;
#60717=CARTESIAN_POINT ( 'NONE',  ( 1.339745962155612702, 16.83034180399266688, -5.000000000000000000 ) ) ;
#60719=CARTESIAN_POINT ( 'NONE',  ( 2.229367062499998831, -79.89583333196773651, -3.861377020970580887 ) ) ;
#60723=( BOUNDED_CURVE ( )  B_SPLINE_CURVE ( 2, ( #22309, #16839, #51270, #47380, #7832, #26813, #22631, #56414, #7518 ),
 .UNSPECIFIED., .F., .F. ) 
 B_SPLINE_CURVE_WITH_KNOTS ( ( 3, 2, 2, 2, 3 ),
 ( 0.1312500000000000056, 0.1319444444444444475, 0.1333333333333333315, 0.1347222222222222154, 0.1354166666666666574 ),
 .UNSPECIFIED. ) 
 CURVE ( )  GEOMETRIC_REPRESENTATION_ITEM ( )  RATIONAL_B_SPLINE_CURVE ( ( 0.9330127018922194093, 0.9330127018922194093, 1.000000000000000000, 0.8660254037844387076, 1.000000000000000000, 0.8660254037844387076, 1.000000000000000000, 0.9330127018922194093, 0.9330127018922194093 ) ) 
 REPRESENTATION_ITEM ( '' )  );
#60726=CARTESIAN_POINT ( 'NONE',  ( -6.972266317189433020E-16, -15.12499999726881050, -5.000000000000000000 ) ) ;
#60730=CARTESIAN_POINT ( 'NONE',  ( 4.458734125000000326, 11.85416666803225993, 2.574251347313718519 ) ) ;
#60733=EDGE_CURVE ( 'NONE', #14373, #50115, #11959, .T. ) ;
#60737=CARTESIAN_POINT ( 'NONE',  ( -1.339745962155613812, -14.08034179853029144, -5.000000000000000000 ) ) ;
#60738=CARTESIAN_POINT ( 'NONE',  ( -2.229367062499996610, -85.14583333196773651, 3.861377020970582219 ) ) ;
#60739=CARTESIAN_POINT ( 'NONE',  ( 4.458734124999998549, -2.729166665301069550, -2.574251347313721627 ) ) ;
#60740=CARTESIAN_POINT ( 'NONE',  ( -5.000000000000000000, -31.08333333333332860, -2.886751345948128211 ) ) ;
#60741=EDGE_LOOP ( 'NONE', ( #2971, #39419, #9401, #39950 ) ) ;
#60742=CARTESIAN_POINT ( 'NONE',  ( -3.152548672688508926E-16, -32.81249999863440792, -5.148502694627439702 ) ) ;
#60746=CARTESIAN_POINT ( 'NONE',  ( 9.457646018065525792E-16, 19.93750000136559208, 5.148502694627439702 ) ) ;
#60748=CARTESIAN_POINT ( 'NONE',  ( 1.975475456537005874E-15, 1.250000000000000000, 5.000000000000000000 ) ) ;
#60749=CARTESIAN_POINT ( 'NONE',  ( -2.229367062500000163, -78.72916666530106511, -3.861377020970580443 ) ) ;
#60752=CARTESIAN_POINT ( 'NONE',  ( -2.500000000000000444, 17.95833333606451632, -4.330127018922193649 ) ) ;
#60753=ORIENTED_EDGE ( 'NONE', *, *, #62515, .T. ) ;
#60755=( BOUNDED_CURVE ( )  B_SPLINE_CURVE ( 2, ( #48387, #466, #4329, #53841, #49337, #29070, #5281, #24900, #39673 ),
 .UNSPECIFIED., .F., .F. ) 
 B_SPLINE_CURVE_WITH_KNOTS ( ( 3, 2, 2, 2, 3 ),
 ( 0.3229166666666666852, 0.3236111111111111271, 0.3250000000000000111, 0.3263888888888888951, 0.3270833333333333370 ),
 .UNSPECIFIED. ) 
 CURVE ( )  GEOMETRIC_REPRESENTATION_ITEM ( )  RATIONAL_B_SPLINE_CURVE ( ( 0.9330127018922194093, 0.9330127018922194093, 1.000000000000000000, 0.8660254037844387076, 1.000000000000000000, 0.8660254037844387076, 1.000000000000000000, 0.9330127018922194093, 0.9330127018922194093 ) ) 
 REPRESENTATION_ITEM ( '' )  );
#60756=CARTESIAN_POINT ( 'NONE',  ( -5.000000000000000888, -168.6875000027311842, -2.071067811865475949 ) ) ;
#60757=CARTESIAN_POINT ( 'NONE',  ( 1.339745962155615144, -0.7053418012614794952, 4.999999999999999112 ) ) ;
#60758=CARTESIAN_POINT ( 'NONE',  ( -5.000000000000000000, -23.08333333333332860, -2.886751345948128211 ) ) ;
#60759=CARTESIAN_POINT ( 'NONE',  ( -3.152548672688508926E-16, -28.56249999863440436, -5.148502694627439702 ) ) ;
#60761=CARTESIAN_POINT ( 'NONE',  ( 2.229367062500001939, -89.97916666530106511, 3.861377020970579999 ) ) ;
#60762=CARTESIAN_POINT ( 'NONE',  ( 2.500000000000002220, -25.54166666393547658, 4.330127018922192761 ) ) ;
#60763=CARTESIAN_POINT ( 'NONE',  ( -4.458734124999998549, -57.22916666530107932, 2.574251347313722516 ) ) ;
#60765=CARTESIAN_POINT ( 'NONE',  ( 1.339745962155615144, -49.70534180126148271, 4.999999999999999112 ) ) ;
#60766=DIRECTION ( 'NONE',  ( 0.000000000000000000, 0.000000000000000000, 1.000000000000000000 ) ) ;
#60767=CARTESIAN_POINT ( 'NONE',  ( 2.229367062500001939, -4.229166665301070438, 3.861377020970579999 ) ) ;
#60769=CARTESIAN_POINT ( 'NONE',  ( 2.500000000000002220, -71.66666666666667140, 4.330127018922192761 ) ) ;
#60773=CARTESIAN_POINT ( 'NONE',  ( 2.071067811865476394, -159.1875000000000000, 5.000000000000000000 ) ) ;
#60774=CARTESIAN_POINT ( 'NONE',  ( -4.999999999999999112, -71.79166666393547303, 2.886751345948131764 ) ) ;
#60777=CARTESIAN_POINT ( 'NONE',  ( 4.458734124999999437, -17.06249999863440792, -5.460374474430324690E-16 ) ) ;
#60778=CARTESIAN_POINT ( 'NONE',  ( 4.458734125000001214, -54.14583333196773651, 2.574251347313718519 ) ) ;
#60779=CARTESIAN_POINT ( 'NONE',  ( 5.000000000000000000, 10.58333333333333393, -2.886751345948130876 ) ) ;
#60781=CARTESIAN_POINT ( 'NONE',  ( 1.846868145590735200, -143.2500000013655779, -4.458734125000000326 ) ) ;
#60783=CARTESIAN_POINT ( 'NONE',  ( 0.000000000000000000, -170.0000000000000000, 5.000000000000000000 ) ) ;
#60785=CARTESIAN_POINT ( 'NONE',  ( 0.000000000000000000, -170.0000000000000000, 5.000000000000000000 ) ) ;
#60786=CARTESIAN_POINT ( 'NONE',  ( -2.229367062499996610, 24.60416666803225993, 3.861377020970582219 ) ) ;
#60790=CARTESIAN_POINT ( 'NONE',  ( -1.846868145590737420, -149.0000000013656063, 4.458734124999999437 ) ) ;
#60792=CARTESIAN_POINT ( 'NONE',  ( 2.229367062499998831, -62.89583333196774362, -3.861377020970580887 ) ) ;
#60793=CARTESIAN_POINT ( 'NONE',  ( 4.729367062499999719, -139.8437500006828031, 0.000000000000000000 ) ) ;
#60794=CARTESIAN_POINT ( 'NONE',  ( -2.229367062500000163, -8.479166665301073991, -3.861377020970580443 ) ) ;
#60796=CARTESIAN_POINT ( 'NONE',  ( -3.152801135295367985, -143.8125000013655779, 3.152801135295367096 ) ) ;
#60802=CARTESIAN_POINT ( 'NONE',  ( -3.152548672688508926E-16, 27.18750000136559564, -5.148502694627439702 ) ) ;
#60803=CARTESIAN_POINT ( 'NONE',  ( 1.339745962155612702, -88.16965819600733312, -5.000000000000000000 ) ) ;
#60806=CARTESIAN_POINT ( 'NONE',  ( 5.000000000000000000, -150.1250000027312126, 0.000000000000000000 ) ) ;
#60808=FACE_OUTER_BOUND ( 'NONE', #58783, .T. ) ;
#60810=CARTESIAN_POINT ( 'NONE',  ( 1.339745962155612702, -60.16965819600731891, -5.000000000000000000 ) ) ;
#60811=CARTESIAN_POINT ( 'NONE',  ( 9.457646018065525792E-16, 13.93750000136559564, 5.148502694627439702 ) ) ;
#60813=VECTOR ( 'NONE', #722, 1000.000000000000000 ) ;
#60814=CARTESIAN_POINT ( 'NONE',  ( -4.458734124999999437, -12.64583333196774007, -2.574251347313719407 ) ) ;
#60816=CARTESIAN_POINT ( 'NONE',  ( 3.152801135295366208, -164.5625000013656063, 3.152801135295367985 ) ) ;
#60817=CARTESIAN_POINT ( 'NONE',  ( -6.972266317189433020E-16, -41.12499999726880162, -5.000000000000000000 ) ) ;
#60822=CARTESIAN_POINT ( 'NONE',  ( -3.152548672688508926E-16, -35.56249999863440792, -5.148502694627439702 ) ) ;
#60823=LINE ( 'NONE', #51173, #34841 ) ;
#60827=ORIENTED_EDGE ( 'NONE', *, *, #19267, .F. ) ;
#60831=CARTESIAN_POINT ( 'NONE',  ( 5.000000000000000000, -5.499999999999998224, -6.123233995736766282E-16 ) ) ;
#60832=CARTESIAN_POINT ( 'NONE',  ( -4.458734124999997661, -74.22916666530106511, 2.574251347313722516 ) ) ;
#60834=CARTESIAN_POINT ( 'NONE',  ( -4.999999999999999112, -8.791666663935483683, 2.886751345948131764 ) ) ;
#60835=CARTESIAN_POINT ( 'NONE',  ( 4.458734124999999437, -36.81249999863440792, -5.460374474430324690E-16 ) ) ;
#60836=VERTEX_POINT ( 'NONE', #46387 ) ;
#60838=CARTESIAN_POINT ( 'NONE',  ( 2.229367062499998831, 12.10416666803226171, -3.861377020970580887 ) ) ;
#60841=CARTESIAN_POINT ( 'NONE',  ( -3.535250795749689387E-16, -56.25000000000000000, -5.773502691896257311 ) ) ;
#60844=CARTESIAN_POINT ( 'NONE',  ( -4.458734124999999437, -74.31249999863440792, 0.000000000000000000 ) ) ;
#60845=CARTESIAN_POINT ( 'NONE',  ( -3.152801135295367096, -140.3125000013655779, -3.152801135295367541 ) ) ;
#60846=CARTESIAN_POINT ( 'NONE',  ( 4.458734125000001214, -87.89583333196773651, 2.574251347313718519 ) ) ;
#60848=CARTESIAN_POINT ( 'NONE',  ( 4.458734125000001214, -34.14583333196772941, 2.574251347313718519 ) ) ;
#60853=CARTESIAN_POINT ( 'NONE',  ( 1.339745962155612702, -86.29465819873851729, -5.000000000000000000 ) ) ;
#60856=CARTESIAN_POINT ( 'NONE',  ( 3.535533905932736864, -152.1250000000000000, 3.535533905932738641 ) ) ;
#60857=CARTESIAN_POINT ( 'NONE',  ( 2.229367062500001939, -66.22916666530106511, 3.861377020970579999 ) ) ;
#60862=CARTESIAN_POINT ( 'NONE',  ( -2.500000000000000444, 4.958333336064518981, -4.330127018922193649 ) ) ;
#60863=ORIENTED_EDGE ( 'NONE', *, *, #62096, .T. ) ;
#60866=CARTESIAN_POINT ( 'NONE',  ( -4.458734124999998549, 7.770833334698925121, 2.574251347313722516 ) ) ;
#60868=CARTESIAN_POINT ( 'NONE',  ( -1.846868145590734756, -156.1250000013655779, -4.458734124999999437 ) ) ;
#60872=CARTESIAN_POINT ( 'NONE',  ( 2.071067811865412445, -163.9375000027311842, -5.000000000000063949 ) ) ;
#60874=CYLINDRICAL_SURFACE ( 'NONE', #25248, 5.000000000000000000 ) ;
#60875=EDGE_CURVE ( 'NONE', #551, #29321, #2333, .T. ) ;
#60880=CARTESIAN_POINT ( 'NONE',  ( 4.458734124999998549, 29.27083333469893134, -2.574251347313721627 ) ) ;
#60883=CARTESIAN_POINT ( 'NONE',  ( -4.458734124999999437, 3.437500001365594748, 0.000000000000000000 ) ) ;
#60886=CARTESIAN_POINT ( 'NONE',  ( -5.000000000000000000, -146.6250000027312126, -6.123233995736766282E-16 ) ) ;
#60887=CARTESIAN_POINT ( 'NONE',  ( 5.000000000000000000, -33.37499999726880873, -6.123233995736766282E-16 ) ) ;
#60892=LINE ( 'NONE', #36435, #55531 ) ;
#60893=LINE ( 'NONE', #37388, #35731 ) ;
#60895=CARTESIAN_POINT ( 'NONE',  ( -4.458734124999999437, -160.1875000013655779, -5.460374474430324690E-16 ) ) ;
#60897=CARTESIAN_POINT ( 'NONE',  ( 1.975475456537005874E-15, 7.249999999999998224, 5.000000000000000000 ) ) ;
#60899=CARTESIAN_POINT ( 'NONE',  ( -1.846868145590737420, -141.7500000013655779, 4.458734124999999437 ) ) ;
#60900=ORIENTED_EDGE ( 'NONE', *, *, #19682, .F. ) ;
#60901=CARTESIAN_POINT ( 'NONE',  ( -2.229367062499996610, 21.60416666803226349, 3.861377020970582219 ) ) ;
#60907=CARTESIAN_POINT ( 'NONE',  ( 1.339745962155612702, 2.705341801261480050, -5.000000000000000000 ) ) ;
#60908=CARTESIAN_POINT ( 'NONE',  ( 5.000000000000000000, 10.58333333333333393, -2.886751345948129988 ) ) ;
#60909=CARTESIAN_POINT ( 'NONE',  ( -3.152548672688508926E-16, -53.56249999863439371, -5.148502694627439702 ) ) ;
#60910=CARTESIAN_POINT ( 'NONE',  ( 2.229367062500001939, -10.97916666530107044, 3.861377020970579999 ) ) ;
#60913=EDGE_CURVE ( 'NONE', #11078, #33613, #29217, .T. ) ;
#60915=LINE ( 'NONE', #11367, #8138 ) ;
#60918=CARTESIAN_POINT ( 'NONE',  ( 5.000000000000000000, -37.41666666666666430, -2.886751345948129988 ) ) ;
#60923=CARTESIAN_POINT ( 'NONE',  ( -2.229367062500000163, -61.47916666530106511, -3.861377020970580443 ) ) ;
#60924=CARTESIAN_POINT ( 'NONE',  ( 3.152801135295367541, -150.5625000013655779, -3.152801135295367541 ) ) ;
#60925=CARTESIAN_POINT ( 'NONE',  ( 4.458734125000001214, -68.89583333196773651, 2.574251347313718519 ) ) ;
#60927=CARTESIAN_POINT ( 'NONE',  ( 4.458734125000001214, -18.14583333196773651, 2.574251347313718519 ) ) ;
#60928=CARTESIAN_POINT ( 'NONE',  ( -3.535250795749689387E-16, -63.12499999726880873, -5.773502691896257311 ) ) ;
#60930=CARTESIAN_POINT ( 'NONE',  ( 1.975475456537005874E-15, -31.62499999726880873, 5.000000000000000000 ) ) ;
#60936=CARTESIAN_POINT ( 'NONE',  ( -4.458734124999999437, -153.9375000013655779, -5.460374474430324690E-16 ) ) ;
#60937=ORIENTED_EDGE ( 'NONE', *, *, #8743, .F. ) ;
#60938=CARTESIAN_POINT ( 'NONE',  ( 5.000000000000000000, -54.49999999999999289, -6.123233995736766282E-16 ) ) ;
#60940=CARTESIAN_POINT ( 'NONE',  ( 2.500000000000002220, -8.666666666666669627, 4.330127018922192761 ) ) ;
#60941=CARTESIAN_POINT ( 'NONE',  ( -4.458734124999999437, -49.56249999863440792, 0.000000000000000000 ) ) ;
#60944=CARTESIAN_POINT ( 'NONE',  ( 5.000000000000000888, 10.54166666939785202, 2.886751345948126879 ) ) ;
#60946=CARTESIAN_POINT ( 'NONE',  ( -4.458734124999998549, 22.77083333469892423, 2.574251347313722516 ) ) ;
#60949=CYLINDRICAL_SURFACE ( 'NONE', #21176, 5.000000000000000000 ) ;
#60950=( BOUNDED_CURVE ( )  B_SPLINE_CURVE ( 2, ( #1649, #40540, #11270, #18319, #12543, #13502, #51792, #3230, #62081 ),
 .UNSPECIFIED., .F., .F. ) 
 B_SPLINE_CURVE_WITH_KNOTS ( ( 3, 2, 2, 2, 3 ),
 ( 0.05208333333333333565, 0.05277777777777777762, 0.05416666666666666852, 0.05555555555555555247, 0.05625000000000000139 ),
 .UNSPECIFIED. ) 
 CURVE ( )  GEOMETRIC_REPRESENTATION_ITEM ( )  RATIONAL_B_SPLINE_CURVE ( ( 0.9330127018922192983, 0.9330127018922196314, 1.000000000000000000, 0.8660254037844387076, 1.000000000000000000, 0.8660254037844387076, 1.000000000000000000, 0.9330127018922189652, 0.9330127018922192983 ) ) 
 REPRESENTATION_ITEM ( '' )  );
#60955=CARTESIAN_POINT ( 'NONE',  ( 1.339745962155615144, -63.70534180126147561, 4.999999999999999112 ) ) ;
#60960=CARTESIAN_POINT ( 'NONE',  ( 2.499999999999998668, 4.666666666666666075, -4.330127018922193649 ) ) ;
#60962=CARTESIAN_POINT ( 'NONE',  ( 0.000000000000000000, -170.0000000000000000, 0.000000000000000000 ) ) ;
#60964=ORIENTED_EDGE ( 'NONE', *, *, #3572, .T. ) ;
#60967=CARTESIAN_POINT ( 'NONE',  ( 3.535533905932736864, -158.2500000027312126, 3.535533905932738641 ) ) ;
#60973=CARTESIAN_POINT ( 'NONE',  ( 2.071067811865475505, -148.8125000000000284, -5.000000000000000888 ) ) ;
#60977=CARTESIAN_POINT ( 'NONE',  ( 2.229367062500001939, -25.97916666530106866, 3.861377020970579999 ) ) ;
#60979=CARTESIAN_POINT ( 'NONE',  ( 2.071067811865476394, -152.1875000000000000, 5.000000000000000000 ) ) ;
#60981=CARTESIAN_POINT ( 'NONE',  ( -1.846868145590737420, -152.7500000013656063, 4.458734124999999437 ) ) ;
#60982=VERTEX_POINT ( 'NONE', #39508 ) ;
#60983=CARTESIAN_POINT ( 'NONE',  ( 2.229367062500001939, -49.22916666530107221, 3.861377020970579999 ) ) ;
#60986=CARTESIAN_POINT ( 'NONE',  ( -5.000000000000000000, 24.99999999999999645, 0.000000000000000000 ) ) ;
#60989=CARTESIAN_POINT ( 'NONE',  ( -2.229367062500000163, 2.520833334698928230, -3.861377020970580443 ) ) ;
#60990=CARTESIAN_POINT ( 'NONE',  ( -2.499999999999996447, -73.70833333060214443, 4.330127018922195425 ) ) ;
#60991=CARTESIAN_POINT ( 'NONE',  ( 1.062108568985190270E-13, -11.12499999726881761, -4.999999999999999112 ) ) ;
#60992=CARTESIAN_POINT ( 'NONE',  ( 1.975475456537005874E-15, -24.62499999726881583, 5.000000000000000000 ) ) ;
#60993=CARTESIAN_POINT ( 'NONE',  ( 4.458734124999999437, 13.93750000136559386, -5.460374474430324690E-16 ) ) ;
#60994=CARTESIAN_POINT ( 'NONE',  ( 5.000000000000000888, 4.541666669397852019, 2.886751345948126879 ) ) ;
#60995=VERTEX_POINT ( 'NONE', #9920 ) ;
#60997=CARTESIAN_POINT ( 'NONE',  ( -4.458734124999999437, -44.31249999863440081, 0.000000000000000000 ) ) ;
#60998=CARTESIAN_POINT ( 'NONE',  ( -4.458734125000001214, -162.1250000013655779, 1.846868145590734089 ) ) ;
#61000=CARTESIAN_POINT ( 'NONE',  ( 2.499999999999998668, -46.20833333060214443, -4.330127018922193649 ) ) ;
#61002=CARTESIAN_POINT ( 'NONE',  ( -4.458734124999999437, -15.39583333196773474, -2.574251347313719407 ) ) ;
#61003=EDGE_LOOP ( 'NONE', ( #3312, #46463, #57287, #31040 ) ) ;
#61004=CARTESIAN_POINT ( 'NONE',  ( 2.500000000000002220, -89.66666666666665719, 4.330127018922192761 ) ) ;
#61005=CARTESIAN_POINT ( 'NONE',  ( 4.458734124999999437, -163.5000000013655779, 1.846868145590737864 ) ) ;
#61006=CARTESIAN_POINT ( 'NONE',  ( -2.499999999999996447, -60.70833333060214443, 4.330127018922195425 ) ) ;
#61007=ORIENTED_EDGE ( 'NONE', *, *, #22199, .F. ) ;
#61009=CARTESIAN_POINT ( 'NONE',  ( 2.229367062499998831, -33.89583333196772941, -3.861377020970580887 ) ) ;
#61010=CARTESIAN_POINT ( 'NONE',  ( -5.000000000000000000, -38.99999999999999289, 0.000000000000000000 ) ) ;
#61013=ADVANCED_FACE ( 'NONE', ( #15401 ), #40152, .T. ) ;
#61020=CARTESIAN_POINT ( 'NONE',  ( -4.458734124999998549, -81.47916666530106511, 2.574251347313722516 ) ) ;
#61022=FACE_OUTER_BOUND ( 'NONE', #38889, .T. ) ;
#61023=CARTESIAN_POINT ( 'NONE',  ( 3.152801135295367541, -141.5625000013655779, -3.152801135295367541 ) ) ;
#61024=EDGE_CURVE ( 'NONE', #57124, #41833, #8523, .T. ) ;
#61025=CARTESIAN_POINT ( 'NONE',  ( -6.972266317189433020E-16, -84.12499999726880162, -5.000000000000000000 ) ) ;
#61027=CARTESIAN_POINT ( 'NONE',  ( -4.458734124999997661, -47.22916666530105800, 2.574251347313722516 ) ) ;
#61033=FACE_OUTER_BOUND ( 'NONE', #35587, .T. ) ;
#61036=CARTESIAN_POINT ( 'NONE',  ( 5.000000000000000000, 16.62500000273118417, -6.123233995736766282E-16 ) ) ;
#61038=CARTESIAN_POINT ( 'NONE',  ( 2.229367062499998831, -77.89583333196773651, -3.861377020970580887 ) ) ;
#61043=EDGE_LOOP ( 'NONE', ( #3147, #23266, #14451, #10789 ) ) ;
#61045=EDGE_CURVE ( 'NONE', #16689, #53339, #28229, .T. ) ;
#61046=CARTESIAN_POINT ( 'NONE',  ( 1.339745962155615144, -47.70534180126147561, 4.999999999999999112 ) ) ;
#61048=EDGE_CURVE ( 'NONE', #29621, #21623, #57376, .T. ) ;
#61049=CARTESIAN_POINT ( 'NONE',  ( 2.071067811865475505, -168.9375000027311842, -5.000000000000000888 ) ) ;
#61051=CARTESIAN_POINT ( 'NONE',  ( 4.458734124999998549, 14.02083333469892779, -2.574251347313721627 ) ) ;
#61058=CARTESIAN_POINT ( 'NONE',  ( -1.339745962155610925, -13.66965819600733489, 5.000000000000000000 ) ) ;
#61059=CARTESIAN_POINT ( 'NONE',  ( 2.229367062499998831, -87.64583333196773651, -3.861377020970580887 ) ) ;
#61060=CARTESIAN_POINT ( 'NONE',  ( -4.458734124999997661, -11.22916666530107044, 2.574251347313722516 ) ) ;
#61063=CARTESIAN_POINT ( 'NONE',  ( -3.152548672688508926E-16, -37.81249999863440792, -5.148502694627439702 ) ) ;
#61067=CARTESIAN_POINT ( 'NONE',  ( 2.229367062499998831, 19.35416666803225993, -3.861377020970580887 ) ) ;
#61069=CARTESIAN_POINT ( 'NONE',  ( 5.000000000000000000, -66.41666666666667140, -2.886751345948130876 ) ) ;
#61070=CARTESIAN_POINT ( 'NONE',  ( -2.229367062499996610, -84.39583333196773651, 3.861377020970582219 ) ) ;
#61073=CARTESIAN_POINT ( 'NONE',  ( 5.000000000000000888, 19.54166666939785202, 2.886751345948126879 ) ) ;
#61074=VERTEX_POINT ( 'NONE', #6398 ) ;
#61075=CARTESIAN_POINT ( 'NONE',  ( -6.972266317189433020E-16, -81.24999999999998579, -5.000000000000000000 ) ) ;
#61076=CARTESIAN_POINT ( 'NONE',  ( -2.071067811865470620, -168.4375000027311557, 5.000000000000007105 ) ) ;
#61077=DIRECTION ( 'NONE',  ( -0.000000000000000000, 1.000000000000000000, -0.000000000000000000 ) ) ;
#61078=CARTESIAN_POINT ( 'NONE',  ( -5.000000000000000000, -25.00000000000000000, 0.000000000000000000 ) ) ;
#61079=CARTESIAN_POINT ( 'NONE',  ( 4.458734124999998549, -27.72916666530107221, -2.574251347313721627 ) ) ;
#61080=CARTESIAN_POINT ( 'NONE',  ( 4.458734124999999437, -89.81249999863440792, -5.460374474430324690E-16 ) ) ;
#61081=CARTESIAN_POINT ( 'NONE',  ( -3.535250795749689387E-16, -30.12499999726881228, -5.773502691896257311 ) ) ;
#61082=CARTESIAN_POINT ( 'NONE',  ( 9.457646018065525792E-16, -53.06249999863441502, 5.148502694627439702 ) ) ;
#61083=ORIENTED_EDGE ( 'NONE', *, *, #2009, .F. ) ;
#61085=CARTESIAN_POINT ( 'NONE',  ( 4.458734124999999437, -1.062499998634405696, -5.460374474430324690E-16 ) ) ;
#61086=ORIENTED_EDGE ( 'NONE', *, *, #44784, .F. ) ;
#61087=CARTESIAN_POINT ( 'NONE',  ( -4.999999999999999112, -73.91666666666664298, 2.886751345948131764 ) ) ;
#61091=CARTESIAN_POINT ( 'NONE',  ( 5.000000000000000888, -72.45833333060213022, 2.886751345948126879 ) ) ;
#61094=CARTESIAN_POINT ( 'NONE',  ( 9.457646018065525792E-16, -15.31249999863440436, 5.148502694627439702 ) ) ;
#61095=CARTESIAN_POINT ( 'NONE',  ( -4.458734124999999437, -50.64583333196773651, -2.574251347313719407 ) ) ;
#61096=CARTESIAN_POINT ( 'NONE',  ( 1.975475456537005874E-15, -29.62499999726881228, 5.000000000000000000 ) ) ;
#61098=CARTESIAN_POINT ( 'NONE',  ( 4.458734124999999437, -141.5000000013655779, 1.846868145590737864 ) ) ;
#61100=CARTESIAN_POINT ( 'NONE',  ( 2.071067811865349828, -148.3125000027312126, 5.000000000000126121 ) ) ;
#61101=VERTEX_POINT ( 'NONE', #36294 ) ;
#61102=CARTESIAN_POINT ( 'NONE',  ( -4.458734124999998549, 23.52083333469892779, 2.574251347313722516 ) ) ;
#61105=DIRECTION ( 'NONE',  ( 0.000000000000000000, 0.000000000000000000, 1.000000000000000000 ) ) ;
#61108=CARTESIAN_POINT ( 'NONE',  ( -3.152801135295367985, -149.0625000013655779, 3.152801135295367096 ) ) ;
#61112=CARTESIAN_POINT ( 'NONE',  ( 2.229367062499998831, -65.89583333196773651, -3.861377020970580887 ) ) ;
#61113=EDGE_CURVE ( 'NONE', #37331, #57060, #34813, .T. ) ;
#61114=CARTESIAN_POINT ( 'NONE',  ( -3.535533905932738641, -154.5000000027312126, 3.535533905932737309 ) ) ;
#61116=CARTESIAN_POINT ( 'NONE',  ( 4.458734124999999437, -145.4375000013656063, 0.000000000000000000 ) ) ;
#61120=CARTESIAN_POINT ( 'NONE',  ( 0.000000000000000000, -170.0000000000000000, 0.000000000000000000 ) ) ;
#61123=CARTESIAN_POINT ( 'NONE',  ( 9.457646018065525792E-16, 27.68750000136559208, 5.148502694627439702 ) ) ;
#61126=ADVANCED_FACE ( 'NONE', ( #21821 ), #31778, .T. ) ;
#61128=CARTESIAN_POINT ( 'NONE',  ( 3.061616997868383141E-16, -149.8750000027312126, -5.000000000000000000 ) ) ;
#61131=CARTESIAN_POINT ( 'NONE',  ( -6.972266317189433020E-16, -8.124999997268814056, -5.000000000000000000 ) ) ;
#61132=CARTESIAN_POINT ( 'NONE',  ( 2.229367062499998831, 9.354166668032261711, -3.861377020970580887 ) ) ;
#61134=CARTESIAN_POINT ( 'NONE',  ( 4.458734124999999437, -22.06249999863440436, -5.460374474430324690E-16 ) ) ;
#61137=CARTESIAN_POINT ( 'NONE',  ( -1.846868145590737420, -159.7500000013656063, 4.458734124999999437 ) ) ;
#61143=CARTESIAN_POINT ( 'NONE',  ( 4.458734124999999437, -34.81249999863440792, -5.460374474430324690E-16 ) ) ;
#61144=CARTESIAN_POINT ( 'NONE',  ( 2.499999999999998668, -60.33333333333333570, -4.330127018922193649 ) ) ;
#61145=CARTESIAN_POINT ( 'NONE',  ( -3.152548672688508926E-16, -62.81249999863440792, -5.148502694627439702 ) ) ;
#61148=CARTESIAN_POINT ( 'NONE',  ( 3.061616997868383141E-16, -151.8750000027311842, -5.000000000000000000 ) ) ;
#61152=FACE_OUTER_BOUND ( 'NONE', #56323, .T. ) ;
#61153=CARTESIAN_POINT ( 'NONE',  ( 5.000000000000000000, -6.499999999999999112, -6.123233995736766282E-16 ) ) ;
#61154=CARTESIAN_POINT ( 'NONE',  ( -4.458734124999999437, -74.31249999863440792, 0.000000000000000000 ) ) ;
#61156=CARTESIAN_POINT ( 'NONE',  ( 2.500000000000002220, -13.54166666393548013, 4.330127018922192761 ) ) ;
#61157=CARTESIAN_POINT ( 'NONE',  ( -4.458734124999999437, -39.39583333196773651, -2.574251347313719407 ) ) ;
#61158=VERTEX_POINT ( 'NONE', #60111 ) ;
#61160=CARTESIAN_POINT ( 'NONE',  ( 4.458734125000001214, 14.85416666803225993, 2.574251347313718519 ) ) ;
#61161=EDGE_LOOP ( 'NONE', ( #47916, #50451, #33920, #61646 ) ) ;
#61162=CARTESIAN_POINT ( 'NONE',  ( 5.000000000000000000, -81.41666666666667140, -2.886751345948130876 ) ) ;
#61163=CARTESIAN_POINT ( 'NONE',  ( -2.500000000000000444, -56.16666666666667140, -4.330127018922193649 ) ) ;
#61164=CARTESIAN_POINT ( 'NONE',  ( -3.152801135295367096, -159.3125000013656063, -3.152801135295367541 ) ) ;
#61167=CARTESIAN_POINT ( 'NONE',  ( -2.229367062500000163, -81.47916666530106511, -3.861377020970580443 ) ) ;
#61168=CARTESIAN_POINT ( 'NONE',  ( 3.152801135295367541, -140.5625000013655779, -3.152801135295367541 ) ) ;
#61169=CARTESIAN_POINT ( 'NONE',  ( -2.229367062500000163, -86.47916666530107932, -3.861377020970580443 ) ) ;
#61171=CARTESIAN_POINT ( 'NONE',  ( -4.458734124999999437, -2.562499998634407028, 0.000000000000000000 ) ) ;
#61172=CARTESIAN_POINT ( 'NONE',  ( 4.458734124999999437, -36.06249999863440792, -5.460374474430324690E-16 ) ) ;
#61173=CARTESIAN_POINT ( 'NONE',  ( 1.339745962155612702, -16.16965819600733667, -5.000000000000000000 ) ) ;
#61176=ORIENTED_EDGE ( 'NONE', *, *, #19239, .T. ) ;
#61178=CARTESIAN_POINT ( 'NONE',  ( 0.000000000000000000, -170.0000000000000000, 0.000000000000000000 ) ) ;
#61179=CARTESIAN_POINT ( 'NONE',  ( 2.229367062499998831, -66.89583333196773651, -3.861377020970580887 ) ) ;
#61182=AXIS2_PLACEMENT_3D ( 'NONE', #3011, #51574, #61231 ) ;
#61183=CARTESIAN_POINT ( 'NONE',  ( 5.000000000000000000, -5.499999999999998224, -6.123233995736766282E-16 ) ) ;
#61187=CARTESIAN_POINT ( 'NONE',  ( 2.229367062499998831, 7.354166668032259935, -3.861377020970580887 ) ) ;
#61188=CARTESIAN_POINT ( 'NONE',  ( 0.000000000000000000, -170.0000000000000000, 5.000000000000000000 ) ) ;
#61189=CARTESIAN_POINT ( 'NONE',  ( -1.846868145590737420, -155.7500000013656063, 4.458734124999997661 ) ) ;
#61191=ORIENTED_EDGE ( 'NONE', *, *, #16566, .T. ) ;
#61195=CARTESIAN_POINT ( 'NONE',  ( 1.975475456537005874E-15, -75.74999999999998579, 5.000000000000000000 ) ) ;
#61200=CARTESIAN_POINT ( 'NONE',  ( -2.229367062500000163, 27.52083333469892779, -3.861377020970580443 ) ) ;
#61203=CARTESIAN_POINT ( 'NONE',  ( -4.458734124999999437, -0.5624999986344053626, 0.000000000000000000 ) ) ;
#61204=CARTESIAN_POINT ( 'NONE',  ( 3.061616997868383141E-16, -159.8750000027311842, -5.000000000000000000 ) ) ;
#61206=CARTESIAN_POINT ( 'NONE',  ( -5.000000000000000000, -140.6250000027312126, -6.123233995736766282E-16 ) ) ;
#61207=DIRECTION ( 'NONE',  ( -0.000000000000000000, 1.000000000000000000, -0.000000000000000000 ) ) ;
#61212=DIRECTION ( 'NONE',  ( -0.000000000000000000, 1.000000000000000000, -0.000000000000000000 ) ) ;
#61214=CARTESIAN_POINT ( 'NONE',  ( -3.152801135295367985, -160.0625000013656063, 3.152801135295367096 ) ) ;
#61217=CARTESIAN_POINT ( 'NONE',  ( 1.975475456537005874E-15, -56.75000000000000000, 5.000000000000000000 ) ) ;
#61218=EDGE_LOOP ( 'NONE', ( #56009, #52153, #14643, #24945, #48894, #14863, #42949, #9256, #40318, #58663, #4486, #41644, #60046, #54321, #10684, #32355, #12666, #723, #58371, #28647, #18573, #48493, #43650, #51956, #36470, #54480, #56175, #48795, #13525, #41568, #47395, #30124, #60616, #34378, #22465, #38670, #26694, #38028, #2471, #56253, #7842, #5584, #36245, #3100, #48591, #21600, #42244, #10829, #56044, #14510, #1306, #35353, #22644, #6373, #36866, #32064, #49093, #51630, #62839, #45368, #9214, #62721, #38268, #16447 ) ) ;
#61220=CARTESIAN_POINT ( 'NONE',  ( -3.152548672688508926E-16, 16.18750000136559564, -5.148502694627439702 ) ) ;
#61226=CARTESIAN_POINT ( 'NONE',  ( 1.060575238724906964E-15, 6.249999999999998224, 5.773502691896257311 ) ) ;
#61227=EDGE_CURVE ( 'NONE', #42031, #49174, #33133, .T. ) ;
#61228=CARTESIAN_POINT ( 'NONE',  ( 4.458734124999998549, -54.72916666530107221, -2.574251347313721627 ) ) ;
#61231=DIRECTION ( 'NONE',  ( 0.000000000000000000, 0.000000000000000000, 1.000000000000000000 ) ) ;
#61232=CARTESIAN_POINT ( 'NONE',  ( 1.339745962155612702, 7.830341803992665106, -5.000000000000000000 ) ) ;
#61233=CARTESIAN_POINT ( 'NONE',  ( 0.000000000000000000, -170.0000000000000000, 0.000000000000000000 ) ) ;
#61234=CARTESIAN_POINT ( 'NONE',  ( -5.000000000000000000, -39.08333333333332860, -2.886751345948128211 ) ) ;
#61235=CYLINDRICAL_SURFACE ( 'NONE', #44849, 5.000000000000000000 ) ;
#61238=CARTESIAN_POINT ( 'NONE',  ( -9.184850993605147944E-16, -143.2500000000000284, 5.000000000000000000 ) ) ;
#61239=CARTESIAN_POINT ( 'NONE',  ( 9.457646018065525792E-16, -67.06249999863440792, 5.148502694627439702 ) ) ;
#61240=CARTESIAN_POINT ( 'NONE',  ( -1.846868145590734756, -150.3750000013655779, -4.458734125000000326 ) ) ;
#61241=CARTESIAN_POINT ( 'NONE',  ( -2.229367062500000163, -73.47916666530106511, -3.861377020970580443 ) ) ;
#61243=CARTESIAN_POINT ( 'NONE',  ( 9.457646018065525792E-16, -22.31249999863440792, 5.148502694627439702 ) ) ;
#61244=CARTESIAN_POINT ( 'NONE',  ( 5.000000000000000888, -61.45833333060214443, 2.886751345948126879 ) ) ;
#61246=DIRECTION ( 'NONE',  ( -0.000000000000000000, 1.000000000000000000, -0.000000000000000000 ) ) ;
#61247=EDGE_LOOP ( 'NONE', ( #8075, #46950, #5359, #40270 ) ) ;
#61250=CARTESIAN_POINT ( 'NONE',  ( -1.846868145590734756, -152.1250000013655779, -4.458734125000000326 ) ) ;
#61251=ORIENTED_EDGE ( 'NONE', *, *, #47312, .T. ) ;
#61252=CARTESIAN_POINT ( 'NONE',  ( -9.184850993605147944E-16, -155.3750000027311842, 5.000000000000000000 ) ) ;
#61254=CARTESIAN_POINT ( 'NONE',  ( 2.499999999999998668, -8.333333333333332149, -4.330127018922193649 ) ) ;
#61255=CARTESIAN_POINT ( 'NONE',  ( -4.458734124999998549, -49.47916666530106511, 2.574251347313722516 ) ) ;
#61259=CARTESIAN_POINT ( 'NONE',  ( -2.229367062499996610, 21.85416666803226349, 3.861377020970582219 ) ) ;
#61268=VECTOR ( 'NONE', #47274, 1000.000000000000000 ) ;
#61275=CARTESIAN_POINT ( 'NONE',  ( -5.000000000000000000, 19.00000000000000000, 0.000000000000000000 ) ) ;
#61278=VERTEX_POINT ( 'NONE', #61699 ) ;
#61281=CARTESIAN_POINT ( 'NONE',  ( 2.071067811865476394, -158.3125000027312410, 5.000000000000000000 ) ) ;
#61287=CARTESIAN_POINT ( 'NONE',  ( -5.000000000000000888, -146.5625000000000284, -2.071067811865475949 ) ) ;
#61291=CARTESIAN_POINT ( 'NONE',  ( -4.458734124999999437, -24.31249999863440436, 0.000000000000000000 ) ) ;
#61292=CARTESIAN_POINT ( 'NONE',  ( 2.500000000000002220, 14.33333333333333393, 4.330127018922192761 ) ) ;
#61293=CARTESIAN_POINT ( 'NONE',  ( -2.071067811865478170, -150.3125000000000284, 5.000000000000000000 ) ) ;
#61295=CARTESIAN_POINT ( 'NONE',  ( 4.458734124999999437, -152.4375000013655779, 0.000000000000000000 ) ) ;
#61298=CARTESIAN_POINT ( 'NONE',  ( -3.152548672688508926E-16, -52.81249999863440792, -5.148502694627439702 ) ) ;
#61300=CARTESIAN_POINT ( 'NONE',  ( -2.500000000000000444, 24.83333333333333215, -4.330127018922193649 ) ) ;
#61302=LINE ( 'NONE', #7589, #59182 ) ;
#61303=CARTESIAN_POINT ( 'NONE',  ( 2.229367062499998831, 0.3541666680322609340, -3.861377020970580887 ) ) ;
#61304=CARTESIAN_POINT ( 'NONE',  ( -5.000000000000000888, -142.4375000000000000, 2.071067811865474617 ) ) ;
#61305=CARTESIAN_POINT ( 'NONE',  ( -6.972266317189433020E-16, -52.25000000000000711, -5.000000000000000000 ) ) ;
#61307=CARTESIAN_POINT ( 'NONE',  ( -2.229367062500000163, 17.27083333469892779, -3.861377020970580443 ) ) ;
#61309=CARTESIAN_POINT ( 'NONE',  ( 5.000000000000000000, 0.7083333360645184262, -2.886751345948129988 ) ) ;
#61310=ORIENTED_EDGE ( 'NONE', *, *, #35011, .F. ) ;
#61311=CARTESIAN_POINT ( 'NONE',  ( 1.339745962155612258, 26.29465819873852084, 5.000000000000000888 ) ) ;
#61313=CARTESIAN_POINT ( 'NONE',  ( 5.000000000000000000, 27.70833333606451987, -2.886751345948130876 ) ) ;
#61314=CARTESIAN_POINT ( 'NONE',  ( 2.229367062500001939, -41.97916666530107932, 3.861377020970579999 ) ) ;
#61315=CARTESIAN_POINT ( 'NONE',  ( 3.152801135295367541, -163.5625000013656063, -3.152801135295367541 ) ) ;
#61316=ADVANCED_FACE ( 'NONE', ( #8294 ), #27897, .T. ) ;
#61317=CARTESIAN_POINT ( 'NONE',  ( 2.499999999999998668, -45.20833333060214443, -4.330127018922193649 ) ) ;
#61319=CARTESIAN_POINT ( 'NONE',  ( 2.229367062500001939, -18.97916666530106866, 3.861377020970579999 ) ) ;
#61322=CARTESIAN_POINT ( 'NONE',  ( -5.000000000000000000, -88.00000000000000000, 0.000000000000000000 ) ) ;
#61323=CARTESIAN_POINT ( 'NONE',  ( -1.846868145590737420, -165.7500000013655495, 4.458734124999999437 ) ) ;
#61324=( BOUNDED_CURVE ( )  B_SPLINE_CURVE ( 2, ( #6520, #6201, #35788, #2028, #41225, #45429, #59925, #60872, #40599 ),
 .UNSPECIFIED., .F., .F. ) 
 B_SPLINE_CURVE_WITH_KNOTS ( ( 3, 2, 2, 2, 3 ),
 ( 0.1583333333333334925, 0.1625000000000001721, 0.1666666666666668239, 0.1708333333333335036, 0.1750000000000001554 ),
 .UNSPECIFIED. ) 
 CURVE ( )  GEOMETRIC_REPRESENTATION_ITEM ( )  RATIONAL_B_SPLINE_CURVE ( ( 0.9999999999999970024, 0.9238795325112897361, 1.000000000000000000, 0.9238795325112867385, 1.000000000000000000, 0.9238795325112867385, 1.000000000000000000, 0.9238795325112837409, 1.000000000000003109 ) ) 
 REPRESENTATION_ITEM ( '' )  );
#61326=VERTEX_POINT ( 'NONE', #56872 ) ;
#61328=CARTESIAN_POINT ( 'NONE',  ( 4.458734124999998549, -29.97916666530107577, -2.574251347313721627 ) ) ;
#61337=CARTESIAN_POINT ( 'NONE',  ( -3.152548672688508926E-16, -79.81249999863440792, -5.148502694627439702 ) ) ;
#61339=CARTESIAN_POINT ( 'NONE',  ( 1.339745962155602488, 22.29465819873851729, 5.000000000000007105 ) ) ;
#61341=CARTESIAN_POINT ( 'NONE',  ( 5.000000000000000000, 24.58333333333333215, -2.886751345948130876 ) ) ;
#61343=CARTESIAN_POINT ( 'NONE',  ( -3.152548672688508926E-16, -47.56249999863442213, -5.148502694627439702 ) ) ;
#61345=CARTESIAN_POINT ( 'NONE',  ( -2.499999999999996447, 4.166666666666666075, 4.330127018922195425 ) ) ;
#61347=EDGE_CURVE ( 'NONE', #57375, #23803, #30293, .T. ) ;
#61349=FACE_OUTER_BOUND ( 'NONE', #45865, .T. ) ;
#61351=CARTESIAN_POINT ( 'NONE',  ( -4.458734124999998549, -79.47916666530106511, 2.574251347313722516 ) ) ;
#61352=FACE_OUTER_BOUND ( 'NONE', #39683, .T. ) ;
#61361=CARTESIAN_POINT ( 'NONE',  ( -2.229367062500000163, 13.27083333469892779, -3.861377020970580443 ) ) ;
#61362=CARTESIAN_POINT ( 'NONE',  ( 6.123233995736766282E-16, -170.0000000000000000, -5.000000000000000000 ) ) ;
#61365=AXIS2_PLACEMENT_3D ( 'NONE', #49070, #10471, #24636 ) ;
#61370=CARTESIAN_POINT ( 'NONE',  ( 2.229367062499998831, -7.645833331967735624, -3.861377020970580887 ) ) ;
#61372=VERTEX_POINT ( 'NONE', #22776 ) ;
#61373=CARTESIAN_POINT ( 'NONE',  ( -4.458734124999999437, -36.56249999863440792, 0.000000000000000000 ) ) ;
#61375=CARTESIAN_POINT ( 'NONE',  ( 3.061616997868383141E-16, -155.8750000027311842, -5.000000000000000000 ) ) ;
#61378=CARTESIAN_POINT ( 'NONE',  ( 4.458734124999999437, -150.6875000013656063, 0.000000000000000000 ) ) ;
#61379=CARTESIAN_POINT ( 'NONE',  ( -4.458734124999999437, 20.68750000136559208, 0.000000000000000000 ) ) ;
#61380=ADVANCED_FACE ( 'NONE', ( #42685 ), #12790, .T. ) ;
#61383=CARTESIAN_POINT ( 'NONE',  ( 1.339745962155612702, -66.29465819873851729, -5.000000000000000000 ) ) ;
#61384=CARTESIAN_POINT ( 'NONE',  ( 9.457646018065525792E-16, -85.31249999863439371, 5.148502694627439702 ) ) ;
#61386=CARTESIAN_POINT ( 'NONE',  ( -4.999999999999999112, 20.20833333606451987, 2.886751345948131764 ) ) ;
#61391=CARTESIAN_POINT ( 'NONE',  ( -3.535250795749689387E-16, -24.24999999999999645, -5.773502691896257311 ) ) ;
#61392=CARTESIAN_POINT ( 'NONE',  ( -4.458734124999999437, -29.31249999863440436, 0.000000000000000000 ) ) ;
#61393=CARTESIAN_POINT ( 'NONE',  ( -4.458734124999999437, -86.39583333196772230, -2.574251347313719407 ) ) ;
#61394=EDGE_CURVE ( 'NONE', #34762, #35874, #47949, .T. ) ;
#61395=CARTESIAN_POINT ( 'NONE',  ( 2.500000000000002220, -31.54166666393548724, 4.330127018922192761 ) ) ;
#61396=CARTESIAN_POINT ( 'NONE',  ( -4.458734124999999437, -56.39583333196773651, -2.574251347313719407 ) ) ;
#61400=CARTESIAN_POINT ( 'NONE',  ( 4.458734124999999437, -10.06249999863440614, -5.460374474430324690E-16 ) ) ;
#61401=EDGE_LOOP ( 'NONE', ( #39617, #18618, #10815, #45198 ) ) ;
#61402=CARTESIAN_POINT ( 'NONE',  ( 2.499999999999998668, -70.33333333333332860, -4.330127018922193649 ) ) ;
#61405=VECTOR ( 'NONE', #56682, 1000.000000000000000 ) ;
#61406=CARTESIAN_POINT ( 'NONE',  ( -3.535250795749689387E-16, -75.12499999726880162, -5.773502691896257311 ) ) ;
#61407=CARTESIAN_POINT ( 'NONE',  ( 1.975475456537005874E-15, -85.75000000000000000, 5.000000000000000000 ) ) ;
#61411=CARTESIAN_POINT ( 'NONE',  ( -4.458734124999998549, -16.47916666530107577, 2.574251347313722516 ) ) ;
#61412=CARTESIAN_POINT ( 'NONE',  ( 4.458734125000001214, -51.14583333196772941, 2.574251347313718519 ) ) ;
#61415=CARTESIAN_POINT ( 'NONE',  ( 1.846868145590736310, -139.6250000013656347, 4.458734124999999437 ) ) ;
#61421=CARTESIAN_POINT ( 'NONE',  ( 5.000000000000000000, 18.50000000000000000, -6.123233995736766282E-16 ) ) ;
#61425=CARTESIAN_POINT ( 'NONE',  ( 1.846868145590735200, -149.5000000013655779, -4.458734125000000326 ) ) ;
#61427=LINE ( 'NONE', #36974, #35542 ) ;
#61429=CARTESIAN_POINT ( 'NONE',  ( -4.458734124999999437, -61.64583333196773651, -2.574251347313719407 ) ) ;
#61430=CARTESIAN_POINT ( 'NONE',  ( -5.000000000000000000, -83.95833333060214443, -2.886751345948128211 ) ) ;
#61431=CARTESIAN_POINT ( 'NONE',  ( 3.152801135295367541, -143.3125000013655779, -3.152801135295367541 ) ) ;
#61433=ORIENTED_EDGE ( 'NONE', *, *, #8743, .T. ) ;
#61440=FACE_OUTER_BOUND ( 'NONE', #16855, .T. ) ;
#61448=CARTESIAN_POINT ( 'NONE',  ( 2.229367062499998831, 5.354166668032261711, -3.861377020970580887 ) ) ;
#61450=CARTESIAN_POINT ( 'NONE',  ( -3.152548672688508926E-16, -17.81249999863440792, -5.148502694627439702 ) ) ;
#61451=AXIS2_PLACEMENT_3D ( 'NONE', #50984, #6924, #59681 ) ;
#61453=CARTESIAN_POINT ( 'NONE',  ( 1.846868145590735200, -159.2500000013656063, -4.458734125000000326 ) ) ;
#61458=CARTESIAN_POINT ( 'NONE',  ( -2.229367062499996610, -40.14583333196773651, 3.861377020970582219 ) ) ;
#61460=CARTESIAN_POINT ( 'NONE',  ( 1.339745962155615144, -60.70534180126147561, 4.999999999999999112 ) ) ;
#61461=CARTESIAN_POINT ( 'NONE',  ( -3.152548672688508926E-16, -67.81249999863440792, -5.148502694627439702 ) ) ;
#61464=CARTESIAN_POINT ( 'NONE',  ( 1.975475456537005874E-15, -68.62499999726881583, 5.000000000000000000 ) ) ;
#61465=ORIENTED_EDGE ( 'NONE', *, *, #39441, .T. ) ;
#61468=CARTESIAN_POINT ( 'NONE',  ( -5.000000000000000000, -6.083333333333336590, -2.886751345948128211 ) ) ;
#61469=CARTESIAN_POINT ( 'NONE',  ( -3.152548672688508926E-16, -72.56249999863439371, -5.148502694627439702 ) ) ;
#61471=CARTESIAN_POINT ( 'NONE',  ( 2.500000000000002220, -12.54166666393548013, 4.330127018922192761 ) ) ;
#61472=CARTESIAN_POINT ( 'NONE',  ( -4.458734124999999437, -41.39583333196773651, -2.574251347313719407 ) ) ;
#61474=CYLINDRICAL_SURFACE ( 'NONE', #3556, 5.000000000000000000 ) ;
#61475=CARTESIAN_POINT ( 'NONE',  ( -3.152548672688508926E-16, 7.187500001365594748, -5.148502694627439702 ) ) ;
#61476=ORIENTED_EDGE ( 'NONE', *, *, #14861, .F. ) ;
#61477=CARTESIAN_POINT ( 'NONE',  ( -5.000000000000000888, -151.5625000000001137, -2.071067811865475949 ) ) ;
#61478=CARTESIAN_POINT ( 'NONE',  ( -2.500000000000000444, -57.16666666666667140, -4.330127018922193649 ) ) ;
#61480=CARTESIAN_POINT ( 'NONE',  ( -3.152801135295367985, -161.0625000013656063, 3.152801135295367096 ) ) ;
#61483=CARTESIAN_POINT ( 'NONE',  ( 4.458734124999998549, -81.72916666530106511, -2.574251347313721627 ) ) ;
#61485=CARTESIAN_POINT ( 'NONE',  ( 3.535533905932736864, -166.1250000000000284, 3.535533905932738641 ) ) ;
#61486=EDGE_CURVE ( 'NONE', #34014, #11394, #8884, .T. ) ;
#61487=CARTESIAN_POINT ( 'NONE',  ( -2.229367062499996610, -89.14583333196773651, 3.861377020970582219 ) ) ;
#61489=CARTESIAN_POINT ( 'NONE',  ( 4.458734124999998549, 0.02083333469892617584, -2.574251347313721627 ) ) ;
#61490=CARTESIAN_POINT ( 'NONE',  ( -2.229367062499996610, -34.39583333196772941, 3.861377020970582219 ) ) ;
#61491=EDGE_CURVE ( 'NONE', #27115, #3560, #15472, .T. ) ;
#61492=CARTESIAN_POINT ( 'NONE',  ( 5.000000000000000000, -16.29166666393548368, -2.886751345948130876 ) ) ;
#61494=CARTESIAN_POINT ( 'NONE',  ( -5.000000000000000000, 16.04166666939785202, -2.886751345948128211 ) ) ;
#61496=CARTESIAN_POINT ( 'NONE',  ( -3.535533905932737309, -148.7500000027311842, -3.535533905932738197 ) ) ;
#61497=FACE_OUTER_BOUND ( 'NONE', #35182, .T. ) ;
#61498=CARTESIAN_POINT ( 'NONE',  ( 4.458734125000001214, -72.14583333196773651, 2.574251347313718519 ) ) ;
#61502=CARTESIAN_POINT ( 'NONE',  ( 5.000000000000000000, -164.0000000000000000, 0.000000000000000000 ) ) ;
#61506=CARTESIAN_POINT ( 'NONE',  ( -4.458734124999999437, 2.604166668032263043, -2.574251347313719407 ) ) ;
#61508=CARTESIAN_POINT ( 'NONE',  ( 4.458734124999999437, -157.3750000013655779, -1.846868145590734978 ) ) ;
#61515=DIRECTION ( 'NONE',  ( 0.000000000000000000, 0.000000000000000000, 1.000000000000000000 ) ) ;
#61517=DIRECTION ( 'NONE',  ( 0.000000000000000000, 0.000000000000000000, 1.000000000000000000 ) ) ;
#61519=CARTESIAN_POINT ( 'NONE',  ( 6.123233995736766282E-16, -170.0000000000000000, -5.000000000000000000 ) ) ;
#61522=CARTESIAN_POINT ( 'NONE',  ( -4.458734124999997661, 21.77083333469892779, 2.574251347313722516 ) ) ;
#61524=CARTESIAN_POINT ( 'NONE',  ( -2.229367062499996610, -2.395833331967737845, 3.861377020970582219 ) ) ;
#61526=CARTESIAN_POINT ( 'NONE',  ( 5.000000000000000888, -142.0625000027311842, -2.071067811865475505 ) ) ;
#61531=LINE ( 'NONE', #17463, #4181 ) ;
#61533=CARTESIAN_POINT ( 'NONE',  ( 1.975475456537005874E-15, 6.249999999999998224, 5.000000000000000000 ) ) ;
#61535=CARTESIAN_POINT ( 'NONE',  ( 1.846868145590735200, -157.5000000013656063, -4.458734124999999437 ) ) ;
#61537=VERTEX_POINT ( 'NONE', #14045 ) ;
#61538=CARTESIAN_POINT ( 'NONE',  ( -4.458734124999998549, 15.52083333469892779, 2.574251347313722516 ) ) ;
#61539=ORIENTED_EDGE ( 'NONE', *, *, #37842, .F. ) ;
#61542=AXIS2_PLACEMENT_3D ( 'NONE', #58673, #30676, #25852 ) ;
#61544=CARTESIAN_POINT ( 'NONE',  ( 1.975475456537005874E-15, -10.75000000000000000, 5.000000000000000000 ) ) ;
#61545=CARTESIAN_POINT ( 'NONE',  ( 5.000000000000000000, 6.499999999999999112, -6.123233995736766282E-16 ) ) ;
#61547=CARTESIAN_POINT ( 'NONE',  ( 2.229367062499998831, -56.64583333196773651, -3.861377020970580887 ) ) ;
#61551=LINE ( 'NONE', #17154, #4987 ) ;
#61553=CARTESIAN_POINT ( 'NONE',  ( 5.000000000000000000, -39.41666666666666430, -2.886751345948129988 ) ) ;
#61555=CARTESIAN_POINT ( 'NONE',  ( -1.339745962155610925, -47.79465819873851729, 5.000000000000000000 ) ) ;
#61557=CARTESIAN_POINT ( 'NONE',  ( 2.229367062499998831, -62.64583333196774362, -3.861377020970580887 ) ) ;
#61558=CARTESIAN_POINT ( 'NONE',  ( 3.152801135295366208, -146.8125000013655779, 3.152801135295367985 ) ) ;
#61559=CARTESIAN_POINT ( 'NONE',  ( -4.458734124999998549, -73.22916666530106511, 2.574251347313722516 ) ) ;
#61561=CARTESIAN_POINT ( 'NONE',  ( -2.229367062499996610, -19.39583333196774007, 3.861377020970582219 ) ) ;
#61562=CARTESIAN_POINT ( 'NONE',  ( 1.060575238724906964E-15, -62.62499999726880873, 5.773502691896257311 ) ) ;
#61564=CYLINDRICAL_SURFACE ( 'NONE', #28190, 5.000000000000000000 ) ;
#61565=VERTEX_POINT ( 'NONE', #34944 ) ;
#61567=CARTESIAN_POINT ( 'NONE',  ( 5.000000000000000000, -21.37499999726881228, -6.123233995736766282E-16 ) ) ;
#61568=DIRECTION ( 'NONE',  ( -0.000000000000000000, 1.000000000000000000, -0.000000000000000000 ) ) ;
#61569=CARTESIAN_POINT ( 'NONE',  ( -4.458734124999999437, -152.9375000013655779, -5.460374474430324690E-16 ) ) ;
#61570=ORIENTED_EDGE ( 'NONE', *, *, #46256, .F. ) ;
#61571=CARTESIAN_POINT ( 'NONE',  ( -5.000000000000000000, 3.041666669397851130, -2.886751345948128211 ) ) ;
#61574=CARTESIAN_POINT ( 'NONE',  ( -3.152548672688508926E-16, -52.81249999863440792, -5.148502694627439702 ) ) ;
#61575=ORIENTED_EDGE ( 'NONE', *, *, #58903, .T. ) ;
#61578=CARTESIAN_POINT ( 'NONE',  ( 4.458734124999999437, 21.18750000136559208, -5.460374474430324690E-16 ) ) ;
#61581=CARTESIAN_POINT ( 'NONE',  ( 3.152801135295367541, -169.3125000013656063, -3.152801135295367541 ) ) ;
#61587=EDGE_CURVE ( 'NONE', #23020, #31090, #1209, .T. ) ;
#61591=DIRECTION ( 'NONE',  ( 0.000000000000000000, 0.000000000000000000, -1.000000000000000000 ) ) ;
#61592=CARTESIAN_POINT ( 'NONE',  ( -9.184850993605147944E-16, -161.2500000000000000, 5.000000000000000000 ) ) ;
#61597=ORIENTED_EDGE ( 'NONE', *, *, #17302, .F. ) ;
#61599=CARTESIAN_POINT ( 'NONE',  ( 5.000000000000000000, -154.1250000027312126, 0.000000000000000000 ) ) ;
#61605=( BOUNDED_CURVE ( )  B_SPLINE_CURVE ( 2, ( #22573, #47323, #61496, #38298, #42170, #57616, #3891, #28321, #46684 ),
 .UNSPECIFIED., .F., .F. ) 
 B_SPLINE_CURVE_WITH_KNOTS ( ( 3, 2, 2, 2, 3 ),
 ( 0.6749999999999996003, 0.6791666666666662522, 0.6833333333333329040, 0.6874999999999996669, 0.6916666666666663188 ),
 .UNSPECIFIED. ) 
 CURVE ( )  GEOMETRIC_REPRESENTATION_ITEM ( )  RATIONAL_B_SPLINE_CURVE ( ( 1.000000000000008216, 0.9238795325112786339, 1.000000000000000000, 0.9238795325112867385, 1.000000000000000000, 0.9238795325112867385, 1.000000000000000000, 0.9238795325112928447, 0.9999999999999938938 ) ) 
 REPRESENTATION_ITEM ( '' )  );
#61606=CARTESIAN_POINT ( 'NONE',  ( 3.535533905932738197, -145.8750000000000000, -3.535533905932738197 ) ) ;
#61609=CARTESIAN_POINT ( 'NONE',  ( 1.975475456537005874E-15, -74.75000000000000000, 5.000000000000000000 ) ) ;
#61610=CARTESIAN_POINT ( 'NONE',  ( 2.229367062499998831, -23.64583333196773651, -3.861377020970580887 ) ) ;
#61612=CARTESIAN_POINT ( 'NONE',  ( -5.000000000000000000, 9.125000002731184168, 0.000000000000000000 ) ) ;
#61614=CARTESIAN_POINT ( 'NONE',  ( 4.458734125000000326, -148.3750000013655779, -1.846868145590734978 ) ) ;
#61615=ORIENTED_EDGE ( 'NONE', *, *, #22697, .T. ) ;
#61617=CARTESIAN_POINT ( 'NONE',  ( -2.229367062499996610, -53.39583333196773651, 3.861377020970582219 ) ) ;
#61618=CARTESIAN_POINT ( 'NONE',  ( 5.000000000000000000, -2.416666666666663410, -2.886751345948130876 ) ) ;
#61620=CARTESIAN_POINT ( 'NONE',  ( 5.000000000000000000, 24.58333333333333215, -2.886751345948129988 ) ) ;
#61622=CARTESIAN_POINT ( 'NONE',  ( -4.458734124999999437, -1.395833331967737179, -2.574251347313719407 ) ) ;
#61626=CARTESIAN_POINT ( 'NONE',  ( -4.458734124999998549, 8.520833334698926009, 2.574251347313722516 ) ) ;
#61627=CARTESIAN_POINT ( 'NONE',  ( -5.000000000000000000, 4.041666669397852019, -2.886751345948128211 ) ) ;
#61630=ORIENTED_EDGE ( 'NONE', *, *, #18363, .F. ) ;
#61631=( GEOMETRIC_REPRESENTATION_CONTEXT ( 3 ) GLOBAL_UNCERTAINTY_ASSIGNED_CONTEXT ( ( #58378 ) ) GLOBAL_UNIT_ASSIGNED_CONTEXT ( ( #17021, #17337, #56587 ) ) REPRESENTATION_CONTEXT ( 'NONE', 'WORKASPACE' ) );
#61633=CARTESIAN_POINT ( 'NONE',  ( -2.229367062499996610, -49.14583333196772941, 3.861377020970582219 ) ) ;
#61634=CARTESIAN_POINT ( 'NONE',  ( 2.730187237215162345E-16, -164.4375000013655779, -4.458734124999999437 ) ) ;
#61635=AXIS2_PLACEMENT_3D ( 'NONE', #52522, #3632, #42853 ) ;
#61636=CARTESIAN_POINT ( 'NONE',  ( 5.000000000000000000, -42.29166666393548724, -2.886751345948129988 ) ) ;
#61637=EDGE_LOOP ( 'NONE', ( #37424, #15022, #60164, #3188 ) ) ;
#61638=CARTESIAN_POINT ( 'NONE',  ( 2.229367062499998831, -23.64583333196773651, -3.861377020970580887 ) ) ;
#61640=CARTESIAN_POINT ( 'NONE',  ( 2.500000000000002220, -88.66666666666665719, 4.330127018922192761 ) ) ;
#61641=CARTESIAN_POINT ( 'NONE',  ( 3.152801135295366208, -162.5625000013656063, 3.152801135295367985 ) ) ;
#61644=CARTESIAN_POINT ( 'NONE',  ( -2.229367062499996610, -36.39583333196773651, 3.861377020970582219 ) ) ;
#61645=CARTESIAN_POINT ( 'NONE',  ( -5.000000000000000000, 20.04166666939785202, -2.886751345948128211 ) ) ;
#61646=ORIENTED_EDGE ( 'NONE', *, *, #44001, .T. ) ;
#61649=CARTESIAN_POINT ( 'NONE',  ( -6.972266317189433020E-16, 24.87500000273118417, -5.000000000000000000 ) ) ;
#61651=DIRECTION ( 'NONE',  ( 0.000000000000000000, 0.000000000000000000, 1.000000000000000000 ) ) ;
#61653=CARTESIAN_POINT ( 'NONE',  ( 4.458734124999998549, -78.97916666530106511, -2.574251347313721627 ) ) ;
#61658=CARTESIAN_POINT ( 'NONE',  ( -2.500000000000000444, -47.04166666393547303, -4.330127018922193649 ) ) ;
#61667=CARTESIAN_POINT ( 'NONE',  ( 0.000000000000000000, -170.0000000000000000, 0.000000000000000000 ) ) ;
#61669=CARTESIAN_POINT ( 'NONE',  ( -2.229367062499996610, -80.39583333196773651, 3.861377020970582219 ) ) ;
#61672=ORIENTED_EDGE ( 'NONE', *, *, #62612, .T. ) ;
#61673=CARTESIAN_POINT ( 'NONE',  ( 0.000000000000000000, -170.0000000000000000, 5.000000000000000000 ) ) ;
#61675=CARTESIAN_POINT ( 'NONE',  ( -9.184850993605147944E-16, -165.3750000027312126, 5.000000000000000000 ) ) ;
#61677=CARTESIAN_POINT ( 'NONE',  ( -3.152548672688508926E-16, 12.18750000136559564, -5.148502694627439702 ) ) ;
#61680=ADVANCED_FACE ( 'NONE', ( #14361 ), #33984, .T. ) ;
#61683=EDGE_CURVE ( 'NONE', #46689, #25400, #5692, .T. ) ;
#61685=CARTESIAN_POINT ( 'NONE',  ( 1.339745962155615144, -38.58034179853029144, 4.999999999999999112 ) ) ;
#61686=CARTESIAN_POINT ( 'NONE',  ( -5.000000000000000000, -21.87499999726881228, 0.000000000000000000 ) ) ;
#61687=CARTESIAN_POINT ( 'NONE',  ( 4.458734124999998549, -8.729166665301073991, -2.574251347313721627 ) ) ;
#61688=CYLINDRICAL_SURFACE ( 'NONE', #31903, 5.000000000000000000 ) ;
#61690=CARTESIAN_POINT ( 'NONE',  ( 9.457646018065525792E-16, -35.31249999863440792, 5.148502694627439702 ) ) ;
#61696=CARTESIAN_POINT ( 'NONE',  ( 2.730187237215162345E-16, -150.4375000013656063, -4.458734124999999437 ) ) ;
#61697=CARTESIAN_POINT ( 'NONE',  ( -4.458734124999999437, 16.68750000136559564, 0.000000000000000000 ) ) ;
#61698=CARTESIAN_POINT ( 'NONE',  ( -1.339745962155610925, -43.66965819600732601, 5.000000000000000000 ) ) ;
#61699=CARTESIAN_POINT ( 'NONE',  ( -9.184850993605147944E-16, -155.2500000000000000, 5.000000000000000000 ) ) ;
#61700=CARTESIAN_POINT ( 'NONE',  ( -4.458734124999999437, -85.56249999863439371, 0.000000000000000000 ) ) ;
#61703=CARTESIAN_POINT ( 'NONE',  ( -5.000000000000000000, 20.12500000273118772, 0.000000000000000000 ) ) ;
#61704=ORIENTED_EDGE ( 'NONE', *, *, #411, .F. ) ;
#61705=CARTESIAN_POINT ( 'NONE',  ( 1.975475456537005874E-15, -35.75000000000000711, 5.000000000000000000 ) ) ;
#61706=( BOUNDED_CURVE ( )  B_SPLINE_CURVE ( 2, ( #7519, #61555, #46745, #2690, #17488, #8154, #27753, #47381, #3332 ),
 .UNSPECIFIED., .F., .F. ) 
 B_SPLINE_CURVE_WITH_KNOTS ( ( 3, 2, 2, 2, 3 ),
 ( 0.6479166666666666963, 0.6486111111111111382, 0.6500000000000000222, 0.6513888888888889062, 0.6520833333333333481 ),
 .UNSPECIFIED. ) 
 CURVE ( )  GEOMETRIC_REPRESENTATION_ITEM ( )  RATIONAL_B_SPLINE_CURVE ( ( 0.9330127018922194093, 0.9330127018922194093, 1.000000000000000000, 0.8660254037844387076, 1.000000000000000000, 0.8660254037844387076, 1.000000000000000000, 0.9330127018922194093, 0.9330127018922194093 ) ) 
 REPRESENTATION_ITEM ( '' )  );
#61707=CARTESIAN_POINT ( 'NONE',  ( -5.000000000000000000, -30.00000000000000000, 0.000000000000000000 ) ) ;
#61708=CARTESIAN_POINT ( 'NONE',  ( -4.458734124999999437, -33.31249999863440792, 0.000000000000000000 ) ) ;
#61710=CARTESIAN_POINT ( 'NONE',  ( 5.000000000000000000, -26.37499999726881583, -6.123233995736766282E-16 ) ) ;
#61711=ADVANCED_FACE ( 'NONE', ( #55534 ), #20790, .T. ) ;
#61712=CARTESIAN_POINT ( 'NONE',  ( 4.458734124999999437, -61.81249999863440081, -5.460374474430324690E-16 ) ) ;
#61713=ORIENTED_EDGE ( 'NONE', *, *, #53716, .T. ) ;
#61715=CARTESIAN_POINT ( 'NONE',  ( 2.229367062499998831, -7.895833331967735624, -3.861377020970580887 ) ) ;
#61717=CARTESIAN_POINT ( 'NONE',  ( -4.999999999999999112, -70.91666666666667140, 2.886751345948131764 ) ) ;
#61721=CARTESIAN_POINT ( 'NONE',  ( -2.500000000000000444, -77.04166666393547303, -4.330127018922193649 ) ) ;
#61726=CARTESIAN_POINT ( 'NONE',  ( -4.458734124999998549, -17.47916666530106866, 2.574251347313722516 ) ) ;
#61727=CARTESIAN_POINT ( 'NONE',  ( -4.458734124999998549, -58.47916666530106511, 2.574251347313722516 ) ) ;
#61728=CARTESIAN_POINT ( 'NONE',  ( -5.000000000000000000, -24.00000000000000000, 0.000000000000000000 ) ) ;
#61729=CARTESIAN_POINT ( 'NONE',  ( -8.190561711645485556E-16, -140.6875000013656063, 4.458734124999999437 ) ) ;
#61732=EDGE_LOOP ( 'NONE', ( #57693, #42481, #8489, #34556 ) ) ;
#61735=CARTESIAN_POINT ( 'NONE',  ( -2.500000000000000444, -13.04166666393548013, -4.330127018922193649 ) ) ;
#61736=EDGE_CURVE ( 'NONE', #14373, #51592, #36498, .T. ) ;
#61739=EDGE_CURVE ( 'NONE', #52296, #34949, #41029, .T. ) ;
#61741=CARTESIAN_POINT ( 'NONE',  ( -3.152801135295367985, -147.0625000013655779, 3.152801135295367096 ) ) ;
#61745=CARTESIAN_POINT ( 'NONE',  ( 4.458734124999999437, -61.06249999863440081, -5.460374474430324690E-16 ) ) ;
#61748=CARTESIAN_POINT ( 'NONE',  ( -1.846868145590737420, -146.7500000013656063, 4.458734124999997661 ) ) ;
#61750=ORIENTED_EDGE ( 'NONE', *, *, #19636, .F. ) ;
#61751=CARTESIAN_POINT ( 'NONE',  ( -2.071067811865517250, -164.8125000027312126, -4.999999999999958256 ) ) ;
#61752=FACE_OUTER_BOUND ( 'NONE', #55378, .T. ) ;
#61755=DIRECTION ( 'NONE',  ( -0.000000000000000000, 1.000000000000000000, -0.000000000000000000 ) ) ;
#61757=CARTESIAN_POINT ( 'NONE',  ( -4.458734124999999437, 27.43750000136559208, 0.000000000000000000 ) ) ;
#61760=CARTESIAN_POINT ( 'NONE',  ( 0.000000000000000000, -170.0000000000000000, 0.000000000000000000 ) ) ;
#61761=EDGE_CURVE ( 'NONE', #18747, #57597, #25609, .T. ) ;
#61763=CARTESIAN_POINT ( 'NONE',  ( 2.229367062499998831, 6.354166668032262599, -3.861377020970580887 ) ) ;
#61765=CARTESIAN_POINT ( 'NONE',  ( 9.457646018065525792E-16, -20.31249999863439726, 5.148502694627439702 ) ) ;
#61767=CARTESIAN_POINT ( 'NONE',  ( 2.730187237215162345E-16, -158.1875000013655779, -4.458734124999999437 ) ) ;
#61768=CARTESIAN_POINT ( 'NONE',  ( 0.000000000000000000, -170.0000000000000000, 5.000000000000000000 ) ) ;
#61769=VECTOR ( 'NONE', #18535, 1000.000000000000000 ) ;
#61773=CARTESIAN_POINT ( 'NONE',  ( -3.152548672688508926E-16, -41.56249999863440081, -5.148502694627439702 ) ) ;
#61775=CARTESIAN_POINT ( 'NONE',  ( -4.458734124999997661, -67.47916666530106511, 2.574251347313722516 ) ) ;
#61777=CARTESIAN_POINT ( 'NONE',  ( 1.975475456537005874E-15, -10.62499999726881228, 5.000000000000000000 ) ) ;
#61778=EDGE_LOOP ( 'NONE', ( #15587, #42957, #12764, #42169, #56649, #23058, #35417, #27347 ) ) ;
#61779=CARTESIAN_POINT ( 'NONE',  ( 1.975475456537005874E-15, -89.74999999999998579, 5.000000000000000000 ) ) ;
#61781=CARTESIAN_POINT ( 'NONE',  ( 5.000000000000000000, -8.500000000000000000, -6.123233995736766282E-16 ) ) ;
#61782=CARTESIAN_POINT ( 'NONE',  ( 4.458734124999998549, -77.72916666530106511, -2.574251347313721627 ) ) ;
#61785=CARTESIAN_POINT ( 'NONE',  ( -5.000000000000000000, -10.87499999726881583, 0.000000000000000000 ) ) ;
#61786=CARTESIAN_POINT ( 'NONE',  ( -2.229367062500000163, -42.47916666530107932, -3.861377020970580443 ) ) ;
#61787=ORIENTED_EDGE ( 'NONE', *, *, #56397, .F. ) ;
#61788=CARTESIAN_POINT ( 'NONE',  ( 2.071067811865392461, -144.1875000000000284, 5.000000000000084377 ) ) ;
#61789=CARTESIAN_POINT ( 'NONE',  ( 4.458734125000001214, 4.854166668032262599, 2.574251347313718519 ) ) ;
#61790=VERTEX_POINT ( 'NONE', #45859 ) ;
#61792=CARTESIAN_POINT ( 'NONE',  ( 1.060575238724906964E-15, -57.75000000000000000, 5.773502691896257311 ) ) ;
#61793=CARTESIAN_POINT ( 'NONE',  ( 1.846868145590736310, -158.8750000013655779, 4.458734124999999437 ) ) ;
#61796=CARTESIAN_POINT ( 'NONE',  ( 4.458734125000001214, -81.89583333196773651, 2.574251347313718519 ) ) ;
#61797=CARTESIAN_POINT ( 'NONE',  ( -2.071067811865478170, -167.3125000000000000, 5.000000000000000000 ) ) ;
#61798=CARTESIAN_POINT ( 'NONE',  ( 4.458734124999999437, -89.81249999863440792, -5.460374474430324690E-16 ) ) ;
#61800=CARTESIAN_POINT ( 'NONE',  ( -3.152548672688508926E-16, 0.1875000013655953035, -5.148502694627439702 ) ) ;
#61801=CARTESIAN_POINT ( 'NONE',  ( -4.458734124999998549, -39.47916666530107932, 2.574251347313722516 ) ) ;
#61805=ORIENTED_EDGE ( 'NONE', *, *, #33469, .T. ) ;
#61806=DIRECTION ( 'NONE',  ( -0.000000000000000000, 1.000000000000000000, -0.000000000000000000 ) ) ;
#61807=CARTESIAN_POINT ( 'NONE',  ( 5.000000000000000000, -152.0625000000000284, 2.071067811865478614 ) ) ;
#61809=CARTESIAN_POINT ( 'NONE',  ( 4.458734125000001214, -70.14583333196773651, 2.574251347313718519 ) ) ;
#61812=EDGE_LOOP ( 'NONE', ( #34299, #17706, #50542, #21908 ) ) ;
#61815=EDGE_CURVE ( 'NONE', #60408, #21932, #23364, .T. ) ;
#61818=EDGE_CURVE ( 'NONE', #15531, #18022, #58666, .T. ) ;
#61820=CARTESIAN_POINT ( 'NONE',  ( 2.229367062500001939, 4.020833334698926009, 3.861377020970579999 ) ) ;
#61821=CARTESIAN_POINT ( 'NONE',  ( 1.339745962155615144, -30.58034179853029499, 4.999999999999999112 ) ) ;
#61822=CARTESIAN_POINT ( 'NONE',  ( 4.458734124999999437, -157.4375000013655779, 0.000000000000000000 ) ) ;
#61823=EDGE_CURVE ( 'NONE', #37557, #8687, #32372, .T. ) ;
#61827=CARTESIAN_POINT ( 'NONE',  ( -2.500000000000000444, -25.16666666666666430, -4.330127018922193649 ) ) ;
#61830=CARTESIAN_POINT ( 'NONE',  ( 0.000000000000000000, -170.0000000000000000, 5.000000000000000000 ) ) ;
#61832=CARTESIAN_POINT ( 'NONE',  ( 5.000000000000000000, -23.37499999726881228, -6.123233995736766282E-16 ) ) ;
#61833=CARTESIAN_POINT ( 'NONE',  ( 1.339745962155615144, -67.70534180126149693, 4.999999999999999112 ) ) ;
#61835=CARTESIAN_POINT ( 'NONE',  ( 5.000000000000000888, -78.58333333333334281, 2.886751345948126879 ) ) ;
#61837=CARTESIAN_POINT ( 'NONE',  ( 1.339745962155615144, -10.70534180126147916, 4.999999999999999112 ) ) ;
#61838=CARTESIAN_POINT ( 'NONE',  ( 2.229367062500001939, 24.02083333469892779, 3.861377020970579999 ) ) ;
#61841=CARTESIAN_POINT ( 'NONE',  ( -4.458734124999999437, -4.562499998634401699, 0.000000000000000000 ) ) ;
#61844=EDGE_CURVE ( 'NONE', #30447, #56964, #16782, .T. ) ;
#61845=CARTESIAN_POINT ( 'NONE',  ( 5.000000000000000000, -141.1250000027312126, 0.000000000000000000 ) ) ;
#61846=CARTESIAN_POINT ( 'NONE',  ( -5.000000000000000000, -52.08333333333332860, -2.886751345948128211 ) ) ;
#61851=ADVANCED_FACE ( 'NONE', ( #52596 ), #8530, .T. ) ;
#61852=CARTESIAN_POINT ( 'NONE',  ( -2.500000000000000444, -88.16666666666665719, -4.330127018922193649 ) ) ;
#61854=CARTESIAN_POINT ( 'NONE',  ( 1.846868145590735200, -159.5000000013656063, -4.458734124999999437 ) ) ;
#61856=( NAMED_UNIT ( * ) PLANE_ANGLE_UNIT ( ) SI_UNIT ( $, .RADIAN. ) );
#61857=ORIENTED_EDGE ( 'NONE', *, *, #40609, .F. ) ;
#61858=CARTESIAN_POINT ( 'NONE',  ( 4.458734124999998549, 19.02083333469892779, -2.574251347313721627 ) ) ;
#61859=ORIENTED_EDGE ( 'NONE', *, *, #33768, .T. ) ;
#61863=( BOUNDED_CURVE ( )  B_SPLINE_CURVE ( 2, ( #21884, #60810, #16736, #48208, #29209, #19249, #18633, #57876, #4162 ),
 .UNSPECIFIED., .F., .F. ) 
 B_SPLINE_CURVE_WITH_KNOTS ( ( 3, 2, 2, 2, 3 ),
 ( 0.7437500000000000222, 0.7444444444444444642, 0.7458333333333333481, 0.7472222222222222321, 0.7479166666666666741 ),
 .UNSPECIFIED. ) 
 CURVE ( )  GEOMETRIC_REPRESENTATION_ITEM ( )  RATIONAL_B_SPLINE_CURVE ( ( 0.9330127018922194093, 0.9330127018922194093, 1.000000000000000000, 0.8660254037844387076, 1.000000000000000000, 0.8660254037844387076, 1.000000000000000000, 0.9330127018922194093, 0.9330127018922194093 ) ) 
 REPRESENTATION_ITEM ( '' )  );
#61865=CARTESIAN_POINT ( 'NONE',  ( 2.499999999999998668, 5.666666666666666963, -4.330127018922193649 ) ) ;
#61866=CARTESIAN_POINT ( 'NONE',  ( -4.458734124999997661, -54.22916666530107221, 2.574251347313722516 ) ) ;
#61870=CARTESIAN_POINT ( 'NONE',  ( 2.499999999999998668, 7.791666669397852019, -4.330127018922193649 ) ) ;
#61872=CARTESIAN_POINT ( 'NONE',  ( -5.000000000000000000, -24.95833333060214443, -2.886751345948128211 ) ) ;
#61873=CARTESIAN_POINT ( 'NONE',  ( 2.499999999999998668, -40.33333333333332860, -4.330127018922193649 ) ) ;
#61876=DIRECTION ( 'NONE',  ( -0.000000000000000000, 1.000000000000000000, -0.000000000000000000 ) ) ;
#61877=CARTESIAN_POINT ( 'NONE',  ( -2.229367062499996610, -65.14583333196773651, 3.861377020970582219 ) ) ;
#61878=CARTESIAN_POINT ( 'NONE',  ( 4.458734124999999437, -148.7500000013656063, 1.846868145590737864 ) ) ;
#61879=CARTESIAN_POINT ( 'NONE',  ( 2.229367062499998831, -70.64583333196773651, -3.861377020970580887 ) ) ;
#61881=CARTESIAN_POINT ( 'NONE',  ( -4.458734124999999437, -22.56249999863440436, 0.000000000000000000 ) ) ;
#61882=CARTESIAN_POINT ( 'NONE',  ( 5.000000000000000000, -59.37499999726880873, -6.123233995736766282E-16 ) ) ;
#61883=ORIENTED_EDGE ( 'NONE', *, *, #27518, .T. ) ;
#61884=CARTESIAN_POINT ( 'NONE',  ( -6.972266317189433020E-16, -31.12499999726880873, -5.000000000000000000 ) ) ;
#61890=CARTESIAN_POINT ( 'NONE',  ( -5.147856630858197489E-14, 3.375000002731183280, 5.000000000000000000 ) ) ;
#61893=CARTESIAN_POINT ( 'NONE',  ( 9.457646018065525792E-16, -54.31249999863440081, 5.148502694627439702 ) ) ;
#61897=CARTESIAN_POINT ( 'NONE',  ( 2.229367062500001939, 19.02083333469892779, 3.861377020970579999 ) ) ;
#61900=CARTESIAN_POINT ( 'NONE',  ( -3.152801135295367096, -169.0625000013656063, -3.152801135295367541 ) ) ;
#61903=CARTESIAN_POINT ( 'NONE',  ( -5.000000000000000000, -40.08333333333332860, -2.886751345948128211 ) ) ;
#61911=CARTESIAN_POINT ( 'NONE',  ( -4.999999999999998224, 19.08333333333333570, 2.886751345948131764 ) ) ;
#61914=ORIENTED_EDGE ( 'NONE', *, *, #42909, .T. ) ;
#61915=CARTESIAN_POINT ( 'NONE',  ( -6.972266317189433020E-16, 19.87500000273118417, -5.000000000000000000 ) ) ;
#61917=CARTESIAN_POINT ( 'NONE',  ( 2.071067811865475505, -152.9375000027312126, -5.000000000000000888 ) ) ;
#61923=CARTESIAN_POINT ( 'NONE',  ( -9.184850993605147944E-16, -148.2500000000000284, 5.000000000000000000 ) ) ;
#61927=CARTESIAN_POINT ( 'NONE',  ( -3.152801135295367096, -169.3125000013656063, -3.152801135295367541 ) ) ;
#61928=CARTESIAN_POINT ( 'NONE',  ( -2.229367062500000163, -24.47916666530106866, -3.861377020970580443 ) ) ;
#61932=CARTESIAN_POINT ( 'NONE',  ( -8.190561711645485556E-16, -149.6875000013656063, 4.458734124999999437 ) ) ;
#61933=VERTEX_POINT ( 'NONE', #13667 ) ;
#61934=LINE ( 'NONE', #38110, #17356 ) ;
#61935=CARTESIAN_POINT ( 'NONE',  ( -4.458734124999999437, -52.56249999863440792, 0.000000000000000000 ) ) ;
#61938=CARTESIAN_POINT ( 'NONE',  ( 5.000000000000000888, 26.41666666666666430, 2.886751345948126879 ) ) ;
#61939=CYLINDRICAL_SURFACE ( 'NONE', #6813, 5.000000000000000000 ) ;
#61940=CARTESIAN_POINT ( 'NONE',  ( 2.229367062500001939, -0.9791666653010712151, 3.861377020970579999 ) ) ;
#61944=CARTESIAN_POINT ( 'NONE',  ( 2.229367062499998831, 11.10416666803225993, -3.861377020970580887 ) ) ;
#61949=CARTESIAN_POINT ( 'NONE',  ( 9.457646018065525792E-16, -47.06249999863440792, 5.148502694627439702 ) ) ;
#61950=CARTESIAN_POINT ( 'NONE',  ( 3.152801135295367541, -158.5625000013656063, -3.152801135295367541 ) ) ;
#61951=CARTESIAN_POINT ( 'NONE',  ( 5.000000000000000888, -46.45833333060214443, 2.886751345948126879 ) ) ;
#61953=CARTESIAN_POINT ( 'NONE',  ( 4.458734124999999437, -25.81249999863440792, -5.460374474430324690E-16 ) ) ;
#61954=ORIENTED_EDGE ( 'NONE', *, *, #34737, .F. ) ;
#61955=CARTESIAN_POINT ( 'NONE',  ( 3.061616997868383141E-16, -169.7500000000000000, -5.000000000000000000 ) ) ;
#61956=CARTESIAN_POINT ( 'NONE',  ( 4.458734124999999437, -165.5000000013655779, 1.846868145590737864 ) ) ;
#61959=CARTESIAN_POINT ( 'NONE',  ( -4.458734124999999437, -35.64583333196772941, -2.574251347313719407 ) ) ;
#61960=CARTESIAN_POINT ( 'NONE',  ( -2.499999999999996447, 20.29166666939784847, 4.330127018922195425 ) ) ;
#61962=( BOUNDED_CURVE ( )  B_SPLINE_CURVE ( 2, ( #8038, #22196, #37610, #56929, #42427, #23136, #46634, #56292, #47271 ),
 .UNSPECIFIED., .F., .F. ) 
 B_SPLINE_CURVE_WITH_KNOTS ( ( 3, 2, 2, 2, 3 ),
 ( 0.3895833333333333370, 0.3902777777777777790, 0.3916666666666666630, 0.3930555555555555469, 0.3937499999999999889 ),
 .UNSPECIFIED. ) 
 CURVE ( )  GEOMETRIC_REPRESENTATION_ITEM ( )  RATIONAL_B_SPLINE_CURVE ( ( 0.9330127018922194093, 0.9330127018922194093, 1.000000000000000000, 0.8660254037844387076, 1.000000000000000000, 0.8660254037844387076, 1.000000000000000000, 0.9330127018922194093, 0.9330127018922194093 ) ) 
 REPRESENTATION_ITEM ( '' )  );
#61966=ORIENTED_EDGE ( 'NONE', *, *, #39709, .F. ) ;
#61967=CARTESIAN_POINT ( 'NONE',  ( -5.000000000000000000, -22.87499999726881228, 0.000000000000000000 ) ) ;
#61969=CARTESIAN_POINT ( 'NONE',  ( -2.229367062500000163, -83.72916666530106511, -3.861377020970580443 ) ) ;
#61971=DIRECTION ( 'NONE',  ( -0.000000000000000000, 1.000000000000000000, -0.000000000000000000 ) ) ;
#61972=DIRECTION ( 'NONE',  ( -0.000000000000000000, 1.000000000000000000, -0.000000000000000000 ) ) ;
#61973=CARTESIAN_POINT ( 'NONE',  ( -6.972266317189433020E-16, -47.12499999726880873, -5.000000000000000000 ) ) ;
#61978=CARTESIAN_POINT ( 'NONE',  ( 2.500000000000002220, -3.666666666666665186, 4.330127018922192761 ) ) ;
#61981=CARTESIAN_POINT ( 'NONE',  ( -3.535533905932738641, -153.5000000027312126, 3.535533905932737309 ) ) ;
#61983=CARTESIAN_POINT ( 'NONE',  ( -3.152548672688508926E-16, -84.81249999863439371, -5.148502694627439702 ) ) ;
#61986=VERTEX_POINT ( 'NONE', #48071 ) ;
#61989=CARTESIAN_POINT ( 'NONE',  ( 5.000000000000000888, -165.0625000027312126, -2.071067811865475505 ) ) ;
#61992=CARTESIAN_POINT ( 'NONE',  ( 2.229367062500001939, 14.77083333469892779, 3.861377020970579999 ) ) ;
#61999=CARTESIAN_POINT ( 'NONE',  ( -6.972266317189433020E-16, -22.12499999726881228, -5.000000000000000000 ) ) ;
#62000=CARTESIAN_POINT ( 'NONE',  ( -4.458734124999999437, -7.312499998634404363, 0.000000000000000000 ) ) ;
#62003=CARTESIAN_POINT ( 'NONE',  ( -2.229367062500000163, -36.72916666530107221, -3.861377020970580443 ) ) ;
#62008=AXIS2_PLACEMENT_3D ( 'NONE', #51761, #26681, #17665 ) ;
#62009=CARTESIAN_POINT ( 'NONE',  ( 2.229367062499998831, 15.35416666803225993, -3.861377020970580887 ) ) ;
#62011=CARTESIAN_POINT ( 'NONE',  ( 2.229367062500001939, -81.22916666530106511, 3.861377020970579999 ) ) ;
#62014=CARTESIAN_POINT ( 'NONE',  ( 2.500000000000002220, 16.45833333606451987, 4.330127018922192761 ) ) ;
#62015=ORIENTED_EDGE ( 'NONE', *, *, #19513, .F. ) ;
#62016=CARTESIAN_POINT ( 'NONE',  ( 2.071067811865349828, -147.3125000027311842, 5.000000000000126121 ) ) ;
#62019=CARTESIAN_POINT ( 'NONE',  ( -2.500000000000000444, -28.16666666666666785, -4.330127018922193649 ) ) ;
#62020=CARTESIAN_POINT ( 'NONE',  ( -4.458734124999999437, -32.39583333196773651, -2.574251347313719407 ) ) ;
#62023=CARTESIAN_POINT ( 'NONE',  ( -4.999999999999999112, -26.79166666393548013, 2.886751345948131764 ) ) ;
#62024=CARTESIAN_POINT ( 'NONE',  ( -4.458734124999998549, -59.22916666530106511, 2.574251347313722516 ) ) ;
#62027=CARTESIAN_POINT ( 'NONE',  ( 9.457646018065525792E-16, -11.31249999863440792, 5.148502694627439702 ) ) ;
#62029=CARTESIAN_POINT ( 'NONE',  ( 5.000000000000000000, -79.50000000000000000, -6.123233995736766282E-16 ) ) ;
#62033=CARTESIAN_POINT ( 'NONE',  ( 2.500000000000002220, -79.54166666393547303, 4.330127018922192761 ) ) ;
#62034=CARTESIAN_POINT ( 'NONE',  ( 2.499999999999998668, -65.20833333060213022, -4.330127018922193649 ) ) ;
#62037=CARTESIAN_POINT ( 'NONE',  ( -3.152548672688508926E-16, -21.81249999863440436, -5.148502694627439702 ) ) ;
#62038=CARTESIAN_POINT ( 'NONE',  ( 9.457646018065525792E-16, -59.31249999863440081, 5.148502694627439702 ) ) ;
#62042=CARTESIAN_POINT ( 'NONE',  ( 1.846868145590736310, -168.8750000013655779, 4.458734124999999437 ) ) ;
#62044=CARTESIAN_POINT ( 'NONE',  ( -6.972266317189433020E-16, -8.124999997268814056, -5.000000000000000000 ) ) ;
#62045=ORIENTED_EDGE ( 'NONE', *, *, #16924, .T. ) ;
#62051=AXIS2_PLACEMENT_3D ( 'NONE', #31901, #7467, #8100 ) ;
#62052=CARTESIAN_POINT ( 'NONE',  ( -4.458734125000000326, -150.2500000013656063, -1.846868145590735644 ) ) ;
#62057=CARTESIAN_POINT ( 'NONE',  ( 9.457646018065525792E-16, -63.31249999863440081, 5.148502694627439702 ) ) ;
#62058=CARTESIAN_POINT ( 'NONE',  ( 5.000000000000000000, -43.41666666666666430, -2.886751345948130876 ) ) ;
#62060=CARTESIAN_POINT ( 'NONE',  ( 3.152801135295367541, -144.3125000013655779, -3.152801135295367541 ) ) ;
#62062=EDGE_LOOP ( 'NONE', ( #54148, #18512, #23275, #35766 ) ) ;
#62063=CARTESIAN_POINT ( 'NONE',  ( 1.975475456537005874E-15, 19.25000000000000000, 5.000000000000000000 ) ) ;
#62067=CARTESIAN_POINT ( 'NONE',  ( 5.000000000000000000, -14.29166666393548013, -2.886751345948130876 ) ) ;
#62070=CARTESIAN_POINT ( 'NONE',  ( 1.339745962155612702, -76.16965819600731891, -5.000000000000000000 ) ) ;
#62073=DIRECTION ( 'NONE',  ( 0.000000000000000000, 0.000000000000000000, 1.000000000000000000 ) ) ;
#62075=CARTESIAN_POINT ( 'NONE',  ( 2.229367062500001939, 5.020833334698926897, 3.861377020970579999 ) ) ;
#62077=CARTESIAN_POINT ( 'NONE',  ( -2.229367062500000163, -18.72916666530106866, -3.861377020970580443 ) ) ;
#62080=CARTESIAN_POINT ( 'NONE',  ( -3.152801135295367985, -159.8125000013656063, 3.152801135295367096 ) ) ;
#62081=CARTESIAN_POINT ( 'NONE',  ( -1.127183054612291972E-14, 23.25000000000000000, 4.999999999999999112 ) ) ;
#62085=CARTESIAN_POINT ( 'NONE',  ( -2.229367062500000163, -42.47916666530107932, -3.861377020970580443 ) ) ;
#62087=CARTESIAN_POINT ( 'NONE',  ( 2.229367062499998831, -66.89583333196773651, -3.861377020970580887 ) ) ;
#62089=CARTESIAN_POINT ( 'NONE',  ( 1.975475456537005874E-15, -40.74999999999999289, 5.000000000000000000 ) ) ;
#62090=CARTESIAN_POINT ( 'NONE',  ( 1.339745962155615144, -68.58034179853028434, 4.999999999999999112 ) ) ;
#62091=VERTEX_POINT ( 'NONE', #61305 ) ;
#62092=CARTESIAN_POINT ( 'NONE',  ( -2.499999999999996447, 15.29166666939785202, 4.330127018922195425 ) ) ;
#62094=CARTESIAN_POINT ( 'NONE',  ( -2.500000000000000444, -13.16666666666666607, -4.330127018922193649 ) ) ;
#62095=CARTESIAN_POINT ( 'NONE',  ( 4.458734124999999437, -18.81249999863440792, -5.460374474430324690E-16 ) ) ;
#62096=EDGE_CURVE ( 'NONE', #11394, #40265, #40633, .T. ) ;
#62097=CARTESIAN_POINT ( 'NONE',  ( -4.458734124999997661, -79.22916666530106511, 2.574251347313722516 ) ) ;
#62099=CARTESIAN_POINT ( 'NONE',  ( -2.499999999999996447, -14.70833333060214976, 4.330127018922195425 ) ) ;
#62100=CARTESIAN_POINT ( 'NONE',  ( 2.229367062500001939, -42.97916666530107932, 3.861377020970579999 ) ) ;
#62101=ORIENTED_EDGE ( 'NONE', *, *, #50975, .T. ) ;
#62102=CARTESIAN_POINT ( 'NONE',  ( -6.972266317189433020E-16, -41.24999999999998579, -5.000000000000000000 ) ) ;
#62103=CARTESIAN_POINT ( 'NONE',  ( -4.458734124999999437, 6.354166668032259047, -2.574251347313719407 ) ) ;
#62105=CARTESIAN_POINT ( 'NONE',  ( 2.499999999999998668, -61.33333333333333570, -4.330127018922193649 ) ) ;
#62106=CARTESIAN_POINT ( 'NONE',  ( -4.458734125000000326, -159.2500000013656063, -1.846868145590735644 ) ) ;
#62108=CARTESIAN_POINT ( 'NONE',  ( 2.071067811865560326, -144.8124999999999716, -4.999999999999914735 ) ) ;
#62109=CARTESIAN_POINT ( 'NONE',  ( 4.458734124999998549, -78.72916666530106511, -2.574251347313721627 ) ) ;
#62110=CARTESIAN_POINT ( 'NONE',  ( -5.000000000000000888, -165.5625000000000568, -2.071067811865475949 ) ) ;
#62114=CARTESIAN_POINT ( 'NONE',  ( -2.229367062499996610, -3.395833331967738733, 3.861377020970582219 ) ) ;
#62115=CARTESIAN_POINT ( 'NONE',  ( -4.458734124999999437, -41.64583333196773651, -2.574251347313719407 ) ) ;
#62116=CARTESIAN_POINT ( 'NONE',  ( 3.535533905932736864, -151.2500000027312126, 3.535533905932738641 ) ) ;
#62117=EDGE_CURVE ( 'NONE', #3560, #59122, #33909, .T. ) ;
#62119=CARTESIAN_POINT ( 'NONE',  ( 5.000000000000000888, -86.58333333333332860, 2.886751345948126879 ) ) ;
#62122=CARTESIAN_POINT ( 'NONE',  ( 2.500000000000002220, -2.541666663935477466, 4.330127018922192761 ) ) ;
#62123=CARTESIAN_POINT ( 'NONE',  ( -2.229367062499996610, -71.39583333196773651, 3.861377020970582219 ) ) ;
#62124=CARTESIAN_POINT ( 'NONE',  ( 1.846868145590736310, -145.8750000013656063, 4.458734124999997661 ) ) ;
#62126=CARTESIAN_POINT ( 'NONE',  ( 0.000000000000000000, -170.0000000000000000, 5.000000000000000000 ) ) ;
#62129=CARTESIAN_POINT ( 'NONE',  ( -2.499999999999996447, 3.166666666666664742, 4.330127018922195425 ) ) ;
#62130=CARTESIAN_POINT ( 'NONE',  ( -4.458734124999999437, 4.604166668032261711, -2.574251347313719407 ) ) ;
#62131=CARTESIAN_POINT ( 'NONE',  ( -6.972266317189433020E-16, -30.12499999726880873, -5.000000000000000000 ) ) ;
#62132=CARTESIAN_POINT ( 'NONE',  ( -4.458734124999999437, -155.9375000013655779, -5.460374474430324690E-16 ) ) ;
#62139=CYLINDRICAL_SURFACE ( 'NONE', #13911, 5.000000000000000000 ) ;
#62146=EDGE_CURVE ( 'NONE', #2325, #54415, #60755, .T. ) ;
#62147=CARTESIAN_POINT ( 'NONE',  ( 2.229367062499998831, 20.35416666803225993, -3.861377020970580887 ) ) ;
#62149=CARTESIAN_POINT ( 'NONE',  ( -3.152548672688508926E-16, -1.812499998634406584, -5.148502694627439702 ) ) ;
#62152=CARTESIAN_POINT ( 'NONE',  ( 3.535533905932738197, -140.0000000027311842, -3.535533905932738197 ) ) ;
#62153=CARTESIAN_POINT ( 'NONE',  ( 1.339745962155615144, -75.58034179853029855, 4.999999999999999112 ) ) ;
#62157=( BOUNDED_CURVE ( )  B_SPLINE_CURVE ( 2, ( #20827, #60393, #6358, #45579, #1535, #21140, #31102, #35939, #55880 ),
 .UNSPECIFIED., .F., .F. ) 
 B_SPLINE_CURVE_WITH_KNOTS ( ( 3, 2, 2, 2, 3 ),
 ( 0.7312499999999999556, 0.7319444444444443976, 0.7333333333333332815, 0.7347222222222222765, 0.7354166666666667185 ),
 .UNSPECIFIED. ) 
 CURVE ( )  GEOMETRIC_REPRESENTATION_ITEM ( )  RATIONAL_B_SPLINE_CURVE ( ( 0.9330127018922194093, 0.9330127018922194093, 1.000000000000000000, 0.8660254037844387076, 1.000000000000000000, 0.8660254037844387076, 1.000000000000000000, 0.9330127018922194093, 0.9330127018922194093 ) ) 
 REPRESENTATION_ITEM ( '' )  );
#62158=CARTESIAN_POINT ( 'NONE',  ( -2.500000000000000444, -87.16666666666667140, -4.330127018922193649 ) ) ;
#62159=FACE_OUTER_BOUND ( 'NONE', #9761, .T. ) ;
#62161=CARTESIAN_POINT ( 'NONE',  ( -8.190561711645485556E-16, -156.9375000013655779, 4.458734124999999437 ) ) ;
#62163=CARTESIAN_POINT ( 'NONE',  ( -3.535533905932738641, -147.3750000000000000, 3.535533905932737309 ) ) ;
#62165=CARTESIAN_POINT ( 'NONE',  ( 2.229367062500001939, 19.77083333469892779, 3.861377020970579999 ) ) ;
#62166=ORIENTED_EDGE ( 'NONE', *, *, #42115, .T. ) ;
#62170=CARTESIAN_POINT ( 'NONE',  ( 2.500000000000002220, 2.333333333333333037, 4.330127018922192761 ) ) ;
#62171=CARTESIAN_POINT ( 'NONE',  ( -3.152548672688508926E-16, -59.56249999863440081, -5.148502694627439702 ) ) ;
#62175=ADVANCED_FACE ( 'NONE', ( #9769 ), #4958, .T. ) ;
#62176=CARTESIAN_POINT ( 'NONE',  ( -2.229367062499996610, -26.14583333196773651, 3.861377020970582219 ) ) ;
#62180=CARTESIAN_POINT ( 'NONE',  ( -3.535533905932737309, -151.7500000027312126, -3.535533905932738197 ) ) ;
#62181=CARTESIAN_POINT ( 'NONE',  ( 5.000000000000000000, -38.49999999999999289, -6.123233995736766282E-16 ) ) ;
#62186=CARTESIAN_POINT ( 'NONE',  ( -2.229367062500000163, -63.47916666530106511, -3.861377020970580443 ) ) ;
#62187=CARTESIAN_POINT ( 'NONE',  ( 4.458734124999999437, -147.7500000013655779, 1.846868145590737864 ) ) ;
#62188=CARTESIAN_POINT ( 'NONE',  ( -4.458734124999999437, -74.39583333196775072, -2.574251347313719407 ) ) ;
#62190=ADVANCED_FACE ( 'NONE', ( #18792 ), #43861, .T. ) ;
#62192=CARTESIAN_POINT ( 'NONE',  ( -4.458734124999999437, -24.56249999863440436, 0.000000000000000000 ) ) ;
#62193=CARTESIAN_POINT ( 'NONE',  ( -2.500000000000000444, -68.04166666393547303, -4.330127018922193649 ) ) ;
#62196=EDGE_CURVE ( 'NONE', #20174, #14373, #36135, .T. ) ;
#62200=CARTESIAN_POINT ( 'NONE',  ( 0.000000000000000000, 0.000000000000000000, 0.000000000000000000 ) ) ;
#62201=EDGE_CURVE ( 'NONE', #10085, #13039, #53768, .T. ) ;
#62205=CARTESIAN_POINT ( 'NONE',  ( -1.339745962155610925, -74.66965819600731891, 5.000000000000000000 ) ) ;
#62206=CARTESIAN_POINT ( 'NONE',  ( 4.458734124999998549, -54.97916666530107221, -2.574251347313721627 ) ) ;
#62210=CARTESIAN_POINT ( 'NONE',  ( -2.229367062500000163, 16.52083333469892779, -3.861377020970580443 ) ) ;
#62212=CARTESIAN_POINT ( 'NONE',  ( -2.499999999999996447, -1.833333333333332593, 4.330127018922195425 ) ) ;
#62213=CARTESIAN_POINT ( 'NONE',  ( 4.458734124999999437, -169.4375000013656063, 0.000000000000000000 ) ) ;
#62218=LINE ( 'NONE', #18136, #797 ) ;
#62223=DIRECTION ( 'NONE',  ( -0.000000000000000000, 1.000000000000000000, -0.000000000000000000 ) ) ;
#62230=CARTESIAN_POINT ( 'NONE',  ( -2.071067811865478170, -154.4375000027312126, 5.000000000000000000 ) ) ;
#62235=AXIS2_PLACEMENT_3D ( 'NONE', #36988, #32145, #46957 ) ;
#62237=CARTESIAN_POINT ( 'NONE',  ( 5.000000000000000000, -146.0625000000000000, 2.071067811865478614 ) ) ;
#62240=CARTESIAN_POINT ( 'NONE',  ( -4.458734124999999437, -168.1875000013655779, -5.460374474430324690E-16 ) ) ;
#62242=CARTESIAN_POINT ( 'NONE',  ( 2.229367062499998831, -32.64583333196773651, -3.861377020970580887 ) ) ;
#62243=LINE ( 'NONE', #4314, #12238 ) ;
#62246=CARTESIAN_POINT ( 'NONE',  ( 4.458734125000000326, -146.3750000013655779, -1.846868145590734978 ) ) ;
#62247=ORIENTED_EDGE ( 'NONE', *, *, #56159, .T. ) ;
#62249=CARTESIAN_POINT ( 'NONE',  ( 2.229367062500001939, -58.22916666530107932, 3.861377020970579999 ) ) ;
#62252=CARTESIAN_POINT ( 'NONE',  ( -5.000000000000000000, 26.91666666666666075, -2.886751345948128211 ) ) ;
#62253=CARTESIAN_POINT ( 'NONE',  ( 0.000000000000000000, -170.0000000000000000, 0.000000000000000000 ) ) ;
#62254=CARTESIAN_POINT ( 'NONE',  ( 4.458734125000001214, 0.1041666680322607674, 2.574251347313718519 ) ) ;
#62255=CARTESIAN_POINT ( 'NONE',  ( 1.339745962155612702, -48.29465819873851729, -5.000000000000000000 ) ) ;
#62256=ADVANCED_FACE ( 'NONE', ( #44825 ), #49971, .T. ) ;
#62258=CARTESIAN_POINT ( 'NONE',  ( 4.458734125000001214, 8.854166668032261711, 2.574251347313718519 ) ) ;
#62262=( BOUNDED_CURVE ( )  B_SPLINE_CURVE ( 2, ( #9726, #42011, #32366, #14550, #37827, #53792, #51990, #13063, #32683 ),
 .UNSPECIFIED., .F., .F. ) 
 B_SPLINE_CURVE_WITH_KNOTS ( ( 3, 2, 2, 2, 3 ),
 ( 0.7395833333333333703, 0.7402777777777778123, 0.7416666666666666963, 0.7430555555555555802, 0.7437500000000000222 ),
 .UNSPECIFIED. ) 
 CURVE ( )  GEOMETRIC_REPRESENTATION_ITEM ( )  RATIONAL_B_SPLINE_CURVE ( ( 0.9330127018922194093, 0.9330127018922194093, 1.000000000000000000, 0.8660254037844387076, 1.000000000000000000, 0.8660254037844387076, 1.000000000000000000, 0.9330127018922194093, 0.9330127018922194093 ) ) 
 REPRESENTATION_ITEM ( '' )  );
#62263=CARTESIAN_POINT ( 'NONE',  ( 1.975475456537005874E-15, -83.62499999726878741, 5.000000000000000000 ) ) ;
#62264=CARTESIAN_POINT ( 'NONE',  ( -4.458734124999998549, -48.22916666530106511, 2.574251347313722516 ) ) ;
#62265=CARTESIAN_POINT ( 'NONE',  ( 4.458734124999999437, -159.7500000013656063, 1.846868145590737864 ) ) ;
#62266=CARTESIAN_POINT ( 'NONE',  ( 1.060575238724906964E-15, -49.62499999726880873, 5.773502691896257311 ) ) ;
#62268=CARTESIAN_POINT ( 'NONE',  ( 2.229367062500001939, -23.97916666530107577, 3.861377020970579999 ) ) ;
#62272=CARTESIAN_POINT ( 'NONE',  ( -8.190561711645485556E-16, -159.6875000013655779, 4.458734124999999437 ) ) ;
#62275=EDGE_CURVE ( 'NONE', #55065, #12482, #60915, .T. ) ;
#62278=CARTESIAN_POINT ( 'NONE',  ( 4.458734124999998549, -35.97916666530107221, -2.574251347313721627 ) ) ;
#62280=ADVANCED_FACE ( 'NONE', ( #30990 ), #40954, .T. ) ;
#62286=CARTESIAN_POINT ( 'NONE',  ( 4.458734124999998549, -84.97916666530106511, -2.574251347313721627 ) ) ;
#62289=CARTESIAN_POINT ( 'NONE',  ( 1.339745962155615144, -9.705341801261479162, 4.999999999999999112 ) ) ;
#62290=CARTESIAN_POINT ( 'NONE',  ( 1.339745962155612702, -57.29465819873851729, -5.000000000000000000 ) ) ;
#62292=CARTESIAN_POINT ( 'NONE',  ( -6.972266317189433020E-16, -37.25000000000000000, -5.000000000000000000 ) ) ;
#62294=LINE ( 'NONE', #57160, #42236 ) ;
#62299=CARTESIAN_POINT ( 'NONE',  ( 4.458734124999998549, -82.97916666530107932, -2.574251347313721627 ) ) ;
#62302=ORIENTED_EDGE ( 'NONE', *, *, #54619, .F. ) ;
#62303=CARTESIAN_POINT ( 'NONE',  ( -1.339745962155613812, 17.91965820146970856, -5.000000000000000000 ) ) ;
#62305=CARTESIAN_POINT ( 'NONE',  ( -5.000000000000000888, -166.5625000027312126, 2.071067811865474617 ) ) ;
#62312=CARTESIAN_POINT ( 'NONE',  ( -1.339745962155613812, -20.20534180126147916, -5.000000000000000000 ) ) ;
#62313=CARTESIAN_POINT ( 'NONE',  ( 1.339745962155612702, 17.70534180126147916, -5.000000000000000000 ) ) ;
#62314=CARTESIAN_POINT ( 'NONE',  ( 4.458734124999999437, -10.81249999863440792, -5.460374474430324690E-16 ) ) ;
#62317=CARTESIAN_POINT ( 'NONE',  ( 2.229367062499998831, -37.89583333196773651, -3.861377020970580887 ) ) ;
#62318=VECTOR ( 'NONE', #14509, 1000.000000000000000 ) ;
#62321=CARTESIAN_POINT ( 'NONE',  ( 1.975475456537005874E-15, 10.24999999999999822, 5.000000000000000000 ) ) ;
#62324=VECTOR ( 'NONE', #40077, 1000.000000000000000 ) ;
#62326=CARTESIAN_POINT ( 'NONE',  ( 4.458734124999998549, 16.27083333469892779, -2.574251347313721627 ) ) ;
#62330=CARTESIAN_POINT ( 'NONE',  ( -4.458734124999999437, -84.56249999863439371, 0.000000000000000000 ) ) ;
#62332=CARTESIAN_POINT ( 'NONE',  ( 1.060575238724906964E-15, 11.37500000273118594, 5.773502691896257311 ) ) ;
#62333=ORIENTED_EDGE ( 'NONE', *, *, #61739, .T. ) ;
#62334=CARTESIAN_POINT ( 'NONE',  ( -6.972266317189433020E-16, -35.25000000000000000, -5.000000000000000000 ) ) ;
#62336=CARTESIAN_POINT ( 'NONE',  ( 5.000000000000000000, -52.50000000000000711, -6.123233995736766282E-16 ) ) ;
#62337=CARTESIAN_POINT ( 'NONE',  ( 5.000000000000000000, -31.50000000000000000, -6.123233995736766282E-16 ) ) ;
#62338=CARTESIAN_POINT ( 'NONE',  ( -4.458734124999999437, -32.31249999863440792, 0.000000000000000000 ) ) ;
#62340=( BOUNDED_CURVE ( )  B_SPLINE_CURVE ( 2, ( #13475, #34026, #13778, #48187, #28881, #43665, #43357, #4140, #63306 ),
 .UNSPECIFIED., .F., .F. ) 
 B_SPLINE_CURVE_WITH_KNOTS ( ( 3, 2, 2, 2, 3 ),
 ( 0.8354166666666666963, 0.8361111111111111382, 0.8375000000000000222, 0.8388888888888889062, 0.8395833333333333481 ),
 .UNSPECIFIED. ) 
 CURVE ( )  GEOMETRIC_REPRESENTATION_ITEM ( )  RATIONAL_B_SPLINE_CURVE ( ( 0.9330127018922194093, 0.9330127018922194093, 1.000000000000000000, 0.8660254037844387076, 1.000000000000000000, 0.8660254037844387076, 1.000000000000000000, 0.9330127018922194093, 0.9330127018922194093 ) ) 
 REPRESENTATION_ITEM ( '' )  );
#62341=CARTESIAN_POINT ( 'NONE',  ( 2.500000000000002220, -28.54166666393548013, 4.330127018922192761 ) ) ;
#62342=CARTESIAN_POINT ( 'NONE',  ( -4.458734124999999437, -60.39583333196773651, -2.574251347313719407 ) ) ;
#62345=CARTESIAN_POINT ( 'NONE',  ( 4.458734124999998549, -6.979166665301073103, -2.574251347313721627 ) ) ;
#62347=CARTESIAN_POINT ( 'NONE',  ( 5.000000000000000888, -75.58333333333334281, 2.886751345948126879 ) ) ;
#62350=CARTESIAN_POINT ( 'NONE',  ( -2.499999999999996447, -74.70833333060214443, 4.330127018922195425 ) ) ;
#62353=CARTESIAN_POINT ( 'NONE',  ( 9.457646018065525792E-16, -22.31249999863440792, 5.148502694627439702 ) ) ;
#62354=CARTESIAN_POINT ( 'NONE',  ( -4.458734124999999437, -59.64583333196773651, -2.574251347313719407 ) ) ;
#62356=( BOUNDED_CURVE ( )  B_SPLINE_CURVE ( 2, ( #30396, #20761, #24946, #20118, #40367, #39720, #60008, #15931, #35554 ),
 .UNSPECIFIED., .F., .F. ) 
 B_SPLINE_CURVE_WITH_KNOTS ( ( 3, 2, 2, 2, 3 ),
 ( 0.5104166666666666297, 0.5111111111111110716, 0.5124999999999999556, 0.5138888888888888395, 0.5145833333333332815 ),
 .UNSPECIFIED. ) 
 CURVE ( )  GEOMETRIC_REPRESENTATION_ITEM ( )  RATIONAL_B_SPLINE_CURVE ( ( 0.9330127018922194093, 0.9330127018922194093, 1.000000000000000000, 0.8660254037844387076, 1.000000000000000000, 0.8660254037844387076, 1.000000000000000000, 0.9330127018922194093, 0.9330127018922194093 ) ) 
 REPRESENTATION_ITEM ( '' )  );
#62358=CARTESIAN_POINT ( 'NONE',  ( 1.846868145590735200, -142.2500000013656063, -4.458734125000000326 ) ) ;
#62368=CARTESIAN_POINT ( 'NONE',  ( 2.730187237215162345E-16, -143.4375000013656063, -4.458734124999999437 ) ) ;
#62371=CYLINDRICAL_SURFACE ( 'NONE', #11890, 5.000000000000000000 ) ;
#62373=CARTESIAN_POINT ( 'NONE',  ( -2.229367062500000163, -67.72916666530106511, -3.861377020970580443 ) ) ;
#62374=CARTESIAN_POINT ( 'NONE',  ( -6.972266317189433020E-16, -43.25000000000000000, -5.000000000000000000 ) ) ;
#62376=CARTESIAN_POINT ( 'NONE',  ( 4.458734124999999437, -142.4375000013656063, 0.000000000000000000 ) ) ;
#62378=ORIENTED_EDGE ( 'NONE', *, *, #53865, .F. ) ;
#62386=CARTESIAN_POINT ( 'NONE',  ( 2.229367062500001939, 24.77083333469892779, 3.861377020970579999 ) ) ;
#62387=CARTESIAN_POINT ( 'NONE',  ( 5.000000000000000000, -76.29166666393547303, -2.886751345948130876 ) ) ;
#62393=CARTESIAN_POINT ( 'NONE',  ( -2.229367062500000163, 6.520833334698928674, -3.861377020970580443 ) ) ;
#62395=CARTESIAN_POINT ( 'NONE',  ( -2.229367062499996610, -17.39583333196773651, 3.861377020970582219 ) ) ;
#62397=CARTESIAN_POINT ( 'NONE',  ( 4.458734124999999437, -161.4375000013655779, 0.000000000000000000 ) ) ;
#62398=CARTESIAN_POINT ( 'NONE',  ( -3.535533905932737309, -158.6250000000000284, -3.535533905932738197 ) ) ;
#62401=DIRECTION ( 'NONE',  ( 0.000000000000000000, 0.000000000000000000, 1.000000000000000000 ) ) ;
#62402=CARTESIAN_POINT ( 'NONE',  ( 2.229367062499998831, -42.64583333196773651, -3.861377020970580887 ) ) ;
#62403=CARTESIAN_POINT ( 'NONE',  ( 1.975475456537005874E-15, -83.74999999999998579, 5.000000000000000000 ) ) ;
#62405=CARTESIAN_POINT ( 'NONE',  ( 9.457646018065525792E-16, -68.31249999863440792, 5.148502694627439702 ) ) ;
#62407=CARTESIAN_POINT ( 'NONE',  ( -5.000000000000000000, -41.08333333333333570, -2.886751345948128211 ) ) ;
#62409=VERTEX_POINT ( 'NONE', #31945 ) ;
#62411=( BOUNDED_CURVE ( )  B_SPLINE_CURVE ( 2, ( #22219, #27975, #17704, #37318, #18006, #52746, #42765, #37629, #57270 ),
 .UNSPECIFIED., .F., .F. ) 
 B_SPLINE_CURVE_WITH_KNOTS ( ( 3, 2, 2, 2, 3 ),
 ( 0.7187500000000000000, 0.7194444444444444420, 0.7208333333333333259, 0.7222222222222222099, 0.7229166666666666519 ),
 .UNSPECIFIED. ) 
 CURVE ( )  GEOMETRIC_REPRESENTATION_ITEM ( )  RATIONAL_B_SPLINE_CURVE ( ( 0.9330127018922194093, 0.9330127018922194093, 1.000000000000000000, 0.8660254037844387076, 1.000000000000000000, 0.8660254037844387076, 1.000000000000000000, 0.9330127018922194093, 0.9330127018922194093 ) ) 
 REPRESENTATION_ITEM ( '' )  );
#62412=VECTOR ( 'NONE', #19779, 1000.000000000000000 ) ;
#62414=CARTESIAN_POINT ( 'NONE',  ( 5.000000000000000000, -11.49999999999999645, -6.123233995736766282E-16 ) ) ;
#62415=CARTESIAN_POINT ( 'NONE',  ( -3.152548672688508926E-16, -18.56249999863440792, -5.148502694627439702 ) ) ;
#62416=VECTOR ( 'NONE', #8128, 1000.000000000000000 ) ;
#62417=CARTESIAN_POINT ( 'NONE',  ( 4.458734125000000326, -77.89583333196773651, 2.574251347313718519 ) ) ;
#62420=CARTESIAN_POINT ( 'NONE',  ( 1.060575238724906964E-15, -10.62499999726881583, 5.773502691896257311 ) ) ;
#62421=CARTESIAN_POINT ( 'NONE',  ( -4.458734124999999437, -46.31249999863440792, 0.000000000000000000 ) ) ;
#62423=AXIS2_PLACEMENT_3D ( 'NONE', #54287, #15691, #54931 ) ;
#62424=CARTESIAN_POINT ( 'NONE',  ( 5.000000000000000000, -144.0000000000000284, 0.000000000000000000 ) ) ;
#62425=CARTESIAN_POINT ( 'NONE',  ( 2.229367062500001939, 7.770833334698926009, 3.861377020970579999 ) ) ;
#62426=EDGE_LOOP ( 'NONE', ( #44514, #3651, #55178, #12880 ) ) ;
#62427=FACE_OUTER_BOUND ( 'NONE', #30979, .T. ) ;
#62428=CARTESIAN_POINT ( 'NONE',  ( -5.000000000000000000, -61.08333333333333570, -2.886751345948128211 ) ) ;
#62429=CARTESIAN_POINT ( 'NONE',  ( -4.458734124999999437, -159.1875000013655779, -5.460374474430324690E-16 ) ) ;
#62432=CARTESIAN_POINT ( 'NONE',  ( 5.000000000000000000, -167.0624999999999716, 2.071067811865478614 ) ) ;
#62433=CARTESIAN_POINT ( 'NONE',  ( 1.339745962155615144, -11.70534180126147739, 4.999999999999999112 ) ) ;
#62435=CARTESIAN_POINT ( 'NONE',  ( -4.458734124999998549, -7.479166665301073991, 2.574251347313722516 ) ) ;
#62436=CARTESIAN_POINT ( 'NONE',  ( -3.152548672688508926E-16, -38.81249999863440081, -5.148502694627439702 ) ) ;
#62437=CARTESIAN_POINT ( 'NONE',  ( 5.000000000000000000, -67.37499999726881583, -6.123233995736766282E-16 ) ) ;
#62441=CARTESIAN_POINT ( 'NONE',  ( 1.975475456537005874E-15, -9.624999997268814056, 5.000000000000000000 ) ) ;
#62443=CARTESIAN_POINT ( 'NONE',  ( 1.339745962155612702, -2.169658196007333562, -5.000000000000000000 ) ) ;
#62444=CARTESIAN_POINT ( 'NONE',  ( 4.458734124999999437, -68.06249999863440792, -5.460374474430324690E-16 ) ) ;
#62445=CARTESIAN_POINT ( 'NONE',  ( 4.458734124999997661, -147.7500000013656063, 1.846868145590737864 ) ) ;
#62446=ORIENTED_EDGE ( 'NONE', *, *, #6282, .T. ) ;
#62448=CARTESIAN_POINT ( 'NONE',  ( -6.972266317189433020E-16, -79.12499999726881583, -5.000000000000000000 ) ) ;
#62449=CARTESIAN_POINT ( 'NONE',  ( -2.229367062500000163, 1.520833334698927564, -3.861377020970580443 ) ) ;
#62451=CARTESIAN_POINT ( 'NONE',  ( 1.846868145590736310, -152.6250000013655495, 4.458734124999997661 ) ) ;
#62452=VECTOR ( 'NONE', #3368, 1000.000000000000000 ) ;
#62453=( BOUNDED_CURVE ( )  B_SPLINE_CURVE ( 2, ( #10531, #15369, #49772, #40119, #34992, #5399, #30467, #60080, #25657 ),
 .UNSPECIFIED., .F., .F. ) 
 B_SPLINE_CURVE_WITH_KNOTS ( ( 3, 2, 2, 2, 3 ),
 ( 0.6895833333333333259, 0.6902777777777777679, 0.6916666666666666519, 0.6930555555555555358, 0.6937499999999999778 ),
 .UNSPECIFIED. ) 
 CURVE ( )  GEOMETRIC_REPRESENTATION_ITEM ( )  RATIONAL_B_SPLINE_CURVE ( ( 0.9330127018922194093, 0.9330127018922194093, 1.000000000000000000, 0.8660254037844387076, 1.000000000000000000, 0.8660254037844387076, 1.000000000000000000, 0.9330127018922194093, 0.9330127018922194093 ) ) 
 REPRESENTATION_ITEM ( '' )  );
#62455=ORIENTED_EDGE ( 'NONE', *, *, #1642, .T. ) ;
#62460=EDGE_CURVE ( 'NONE', #25400, #33613, #18467, .T. ) ;
#62462=CARTESIAN_POINT ( 'NONE',  ( 0.000000000000000000, -170.0000000000000000, 0.000000000000000000 ) ) ;
#62463=CARTESIAN_POINT ( 'NONE',  ( -6.972266317189433020E-16, 8.875000002731184168, -5.000000000000000000 ) ) ;
#62466=CARTESIAN_POINT ( 'NONE',  ( 5.000000000000000888, -64.45833333060213022, 2.886751345948126879 ) ) ;
#62469=CARTESIAN_POINT ( 'NONE',  ( 9.457646018065525792E-16, 22.93750000136559919, 5.148502694627439702 ) ) ;
#62471=CARTESIAN_POINT ( 'NONE',  ( -4.458734124999999437, -2.645833331967738289, -2.574251347313719407 ) ) ;
#62472=FACE_OUTER_BOUND ( 'NONE', #16938, .T. ) ;
#62474=CARTESIAN_POINT ( 'NONE',  ( -5.000000000000000000, -139.6250000027312126, -6.123233995736766282E-16 ) ) ;
#62481=DIRECTION ( 'NONE',  ( -0.000000000000000000, 1.000000000000000000, -0.000000000000000000 ) ) ;
#62482=EDGE_CURVE ( 'NONE', #53339, #25310, #61551, .T. ) ;
#62484=CARTESIAN_POINT ( 'NONE',  ( -3.152801135295367985, -156.0625000013656063, 3.152801135295367096 ) ) ;
#62488=CARTESIAN_POINT ( 'NONE',  ( 4.458734124999998549, 17.02083333469892423, -2.574251347313721627 ) ) ;
#62493=CARTESIAN_POINT ( 'NONE',  ( -1.339745962155610925, -87.66965819600731891, 5.000000000000000000 ) ) ;
#62494=CARTESIAN_POINT ( 'NONE',  ( -2.499999999999996447, 3.166666666666664742, 4.330127018922195425 ) ) ;
#62495=EDGE_CURVE ( 'NONE', #30540, #32917, #29907, .T. ) ;
#62496=CARTESIAN_POINT ( 'NONE',  ( -4.458734124999997661, -63.22916666530106511, 2.574251347313722516 ) ) ;
#62497=FACE_OUTER_BOUND ( 'NONE', #63384, .T. ) ;
#62498=CARTESIAN_POINT ( 'NONE',  ( -4.458734124999998549, -29.22916666530107221, 2.574251347313722516 ) ) ;
#62502=CARTESIAN_POINT ( 'NONE',  ( 1.060575238724906964E-15, -42.75000000000000000, 5.773502691896257311 ) ) ;
#62506=CARTESIAN_POINT ( 'NONE',  ( 3.535533905932738197, -154.8750000000000000, -3.535533905932738197 ) ) ;
#62507=CARTESIAN_POINT ( 'NONE',  ( 9.457646018065525792E-16, -65.06249999863440792, 5.148502694627439702 ) ) ;
#62508=CARTESIAN_POINT ( 'NONE',  ( 3.152801135295367541, -146.5625000013655779, -3.152801135295367541 ) ) ;
#62509=CARTESIAN_POINT ( 'NONE',  ( 4.458734124999999437, -77.81249999863440792, -5.460374474430324690E-16 ) ) ;
#62510=VECTOR ( 'NONE', #25765, 1000.000000000000114 ) ;
#62512=CARTESIAN_POINT ( 'NONE',  ( 4.458734125000001214, -25.14583333196774007, 2.574251347313718519 ) ) ;
#62513=CARTESIAN_POINT ( 'NONE',  ( -2.499999999999996447, -63.70833333060215153, 4.330127018922195425 ) ) ;
#62515=EDGE_CURVE ( 'NONE', #63378, #6056, #56410, .T. ) ;
#62516=CARTESIAN_POINT ( 'NONE',  ( -2.500000000000000444, -22.16666666666666785, -4.330127018922193649 ) ) ;
#62521=CYLINDRICAL_SURFACE ( 'NONE', #3466, 5.000000000000000000 ) ;
#62522=CARTESIAN_POINT ( 'NONE',  ( 4.458734124999999437, -54.06249999863440081, -5.460374474430324690E-16 ) ) ;
#62527=CARTESIAN_POINT ( 'NONE',  ( 2.229367062499998831, 16.35416666803225993, -3.861377020970580887 ) ) ;
#62529=CARTESIAN_POINT ( 'NONE',  ( -6.972266317189433020E-16, -42.12499999726880873, -5.000000000000000000 ) ) ;
#62530=CARTESIAN_POINT ( 'NONE',  ( -3.152801135295367985, -166.8125000013656063, 3.152801135295367096 ) ) ;
#62531=VERTEX_POINT ( 'NONE', #3634 ) ;
#62535=( BOUNDED_CURVE ( )  B_SPLINE_CURVE ( 2, ( #29248, #54667, #9, #30205, #44362, #19609, #59498, #14776, #324 ),
 .UNSPECIFIED., .F., .F. ) 
 B_SPLINE_CURVE_WITH_KNOTS ( ( 3, 2, 2, 2, 3 ),
 ( 0.3062500000000000222, 0.3069444444444444642, 0.3083333333333333481, 0.3097222222222222321, 0.3104166666666666741 ),
 .UNSPECIFIED. ) 
 CURVE ( )  GEOMETRIC_REPRESENTATION_ITEM ( )  RATIONAL_B_SPLINE_CURVE ( ( 0.9330127018922194093, 0.9330127018922194093, 1.000000000000000000, 0.8660254037844387076, 1.000000000000000000, 0.8660254037844387076, 1.000000000000000000, 0.9330127018922194093, 0.9330127018922194093 ) ) 
 REPRESENTATION_ITEM ( '' )  );
#62538=EDGE_CURVE ( 'NONE', #36403, #25339, #8153, .T. ) ;
#62542=LINE ( 'NONE', #13320, #57314 ) ;
#62544=CARTESIAN_POINT ( 'NONE',  ( 5.000000000000000000, -18.29166666393547658, -2.886751345948130876 ) ) ;
#62551=CARTESIAN_POINT ( 'NONE',  ( 5.000000000000000000, -152.1250000027312126, 0.000000000000000000 ) ) ;
#62555=EDGE_CURVE ( 'NONE', #39254, #39875, #51733, .T. ) ;
#62557=CARTESIAN_POINT ( 'NONE',  ( -2.071067811865475061, -142.6875000000000568, -5.000000000000000888 ) ) ;
#62561=CARTESIAN_POINT ( 'NONE',  ( -8.190561711645485556E-16, -168.9375000013656063, 4.458734124999999437 ) ) ;
#62562=CARTESIAN_POINT ( 'NONE',  ( -2.229367062499996610, -32.14583333196773651, 3.861377020970582219 ) ) ;
#62564=CARTESIAN_POINT ( 'NONE',  ( 0.000000000000000000, -170.0000000000000000, 5.000000000000000000 ) ) ;
#62566=CARTESIAN_POINT ( 'NONE',  ( 4.458734124999999437, -146.5000000013656347, 1.846868145590737864 ) ) ;
#62567=VERTEX_POINT ( 'NONE', #14208 ) ;
#62569=CARTESIAN_POINT ( 'NONE',  ( 4.458734124999998549, -55.97916666530107932, -2.574251347313721627 ) ) ;
#62572=CARTESIAN_POINT ( 'NONE',  ( 1.060575238724906964E-15, 20.24999999999999645, 5.773502691896257311 ) ) ;
#62573=AXIS2_PLACEMENT_3D ( 'NONE', #38104, #43535, #23631 ) ;
#62575=CARTESIAN_POINT ( 'NONE',  ( -4.458734124999999437, -2.395833331967737845, -2.574251347313719407 ) ) ;
#62576=CARTESIAN_POINT ( 'NONE',  ( 2.071067811865392461, -141.1875000000000284, 5.000000000000084377 ) ) ;
#62577=CARTESIAN_POINT ( 'NONE',  ( 9.457646018065525792E-16, 10.68750000136559386, 5.148502694627439702 ) ) ;
#62579=ORIENTED_EDGE ( 'NONE', *, *, #37160, .F. ) ;
#62580=CARTESIAN_POINT ( 'NONE',  ( 3.535533905932738197, -168.0000000027312126, -3.535533905932738197 ) ) ;
#62581=CARTESIAN_POINT ( 'NONE',  ( 9.457646018065525792E-16, -48.06249999863440081, 5.148502694627439702 ) ) ;
#62582=CARTESIAN_POINT ( 'NONE',  ( 4.458734124999999437, -161.6875000013655779, 0.000000000000000000 ) ) ;
#62583=CARTESIAN_POINT ( 'NONE',  ( 5.000000000000000888, -48.45833333060215153, 2.886751345948126879 ) ) ;
#62584=ORIENTED_EDGE ( 'NONE', *, *, #60320, .T. ) ;
#62585=CARTESIAN_POINT ( 'NONE',  ( 4.458734124999998549, -20.72916666530106866, -2.574251347313721627 ) ) ;
#62590=CARTESIAN_POINT ( 'NONE',  ( 4.458734124999999437, -161.4375000013655779, 0.000000000000000000 ) ) ;
#62591=ORIENTED_EDGE ( 'NONE', *, *, #43698, .F. ) ;
#62593=CARTESIAN_POINT ( 'NONE',  ( 1.975475456537005874E-15, -43.62499999726880873, 5.000000000000000000 ) ) ;
#62595=CARTESIAN_POINT ( 'NONE',  ( 4.458734125000001214, -36.14583333196773651, 2.574251347313718519 ) ) ;
#62596=ORIENTED_EDGE ( 'NONE', *, *, #58233, .F. ) ;
#62602=CARTESIAN_POINT ( 'NONE',  ( -4.458734124999999437, -85.64583333196773651, -2.574251347313719407 ) ) ;
#62605=CARTESIAN_POINT ( 'NONE',  ( 1.339745962155612702, -9.294658198738520838, -5.000000000000000000 ) ) ;
#62606=CARTESIAN_POINT ( 'NONE',  ( -5.000000000000000000, -46.95833333060214443, -2.886751345948128211 ) ) ;
#62608=CARTESIAN_POINT ( 'NONE',  ( -4.999999999999998224, -84.79166666393547303, 2.886751345948131764 ) ) ;
#62612=EDGE_CURVE ( 'NONE', #27799, #53636, #34049, .T. ) ;
#62617=CARTESIAN_POINT ( 'NONE',  ( 4.458734124999999437, -83.06249999863440792, -5.460374474430324690E-16 ) ) ;
#62622=CARTESIAN_POINT ( 'NONE',  ( -2.499999999999996447, 18.29166666939785202, 4.330127018922195425 ) ) ;
#62624=CARTESIAN_POINT ( 'NONE',  ( -2.071067811865478170, -166.4375000027311842, 5.000000000000000000 ) ) ;
#62627=ADVANCED_FACE ( 'NONE', ( #10021 ), #5203, .T. ) ;
#62635=CARTESIAN_POINT ( 'NONE',  ( -2.229367062499996610, -15.14583333196773474, 3.861377020970582219 ) ) ;
#62636=LINE ( 'NONE', #53592, #42181 ) ;
#62639=CARTESIAN_POINT ( 'NONE',  ( -4.458734124999999437, -41.64583333196773651, -2.574251347313719407 ) ) ;
#62640=( BOUNDED_CURVE ( )  B_SPLINE_CURVE ( 2, ( #44959, #4444, #920, #40123, #24073, #43669, #19232, #9586, #29192 ),
 .UNSPECIFIED., .F., .F. ) 
 B_SPLINE_CURVE_WITH_KNOTS ( ( 3, 2, 2, 2, 3 ),
 ( 0.2479166666666666741, 0.2486111111111111160, 0.2500000000000000000, 0.2513888888888888840, 0.2520833333333333259 ),
 .UNSPECIFIED. ) 
 CURVE ( )  GEOMETRIC_REPRESENTATION_ITEM ( )  RATIONAL_B_SPLINE_CURVE ( ( 0.9330127018922194093, 0.9330127018922194093, 1.000000000000000000, 0.8660254037844387076, 1.000000000000000000, 0.8660254037844387076, 1.000000000000000000, 0.9330127018922194093, 0.9330127018922194093 ) ) 
 REPRESENTATION_ITEM ( '' )  );
#62643=CARTESIAN_POINT ( 'NONE',  ( 2.499999999999998668, 0.7916666693978530178, -4.330127018922193649 ) ) ;
#62647=CARTESIAN_POINT ( 'NONE',  ( -4.458734124999999437, 14.60416666803226171, -2.574251347313719407 ) ) ;
#62650=DIRECTION ( 'NONE',  ( 0.000000000000000000, 0.000000000000000000, 1.000000000000000000 ) ) ;
#62651=CARTESIAN_POINT ( 'NONE',  ( 2.229367062500001939, -90.22916666530106511, 3.861377020970579999 ) ) ;
#62653=CARTESIAN_POINT ( 'NONE',  ( 5.000000000000000888, 11.54166666939785202, 2.886751345948126879 ) ) ;
#62655=CYLINDRICAL_SURFACE ( 'NONE', #28369, 5.000000000000000000 ) ;
#62657=CARTESIAN_POINT ( 'NONE',  ( -5.000000000000000000, -26.99999999999999645, 0.000000000000000000 ) ) ;
#62658=CARTESIAN_POINT ( 'NONE',  ( -4.458734124999998549, -35.22916666530107221, 2.574251347313722516 ) ) ;
#62659=CARTESIAN_POINT ( 'NONE',  ( 2.500000000000002220, -35.54166666393547303, 4.330127018922192761 ) ) ;
#62660=CARTESIAN_POINT ( 'NONE',  ( 4.458734124999998549, -60.72916666530106511, -2.574251347313721627 ) ) ;
#62661=ORIENTED_EDGE ( 'NONE', *, *, #36943, .F. ) ;
#62663=CARTESIAN_POINT ( 'NONE',  ( 9.457646018065525792E-16, -9.312499998634406140, 5.148502694627439702 ) ) ;
#62664=ORIENTED_EDGE ( 'NONE', *, *, #16065, .F. ) ;
#62665=CARTESIAN_POINT ( 'NONE',  ( -4.999999999999999112, -75.91666666666667140, 2.886751345948131764 ) ) ;
#62668=CARTESIAN_POINT ( 'NONE',  ( 2.499999999999998668, -75.20833333060214443, -4.330127018922193649 ) ) ;
#62670=ORIENTED_EDGE ( 'NONE', *, *, #18867, .T. ) ;
#62672=CARTESIAN_POINT ( 'NONE',  ( 4.458734124999999437, -20.06249999863440081, -5.460374474430324690E-16 ) ) ;
#62673=CARTESIAN_POINT ( 'NONE',  ( 9.457646018065525792E-16, -56.31249999863440081, 5.148502694627439702 ) ) ;
#62676=CARTESIAN_POINT ( 'NONE',  ( 4.458734124999999437, -165.7500000013655495, 1.846868145590737864 ) ) ;
#62678=CARTESIAN_POINT ( 'NONE',  ( 2.500000000000002220, -50.54166666393547303, 4.330127018922192761 ) ) ;
#62683=VECTOR ( 'NONE', #19502, 1000.000000000000000 ) ;
#62686=CARTESIAN_POINT ( 'NONE',  ( -3.152801135295367096, -144.3125000013655779, -3.152801135295367541 ) ) ;
#62690=CARTESIAN_POINT ( 'NONE',  ( 2.229367062500001939, -69.22916666530107932, 3.861377020970579999 ) ) ;
#62691=DIRECTION ( 'NONE',  ( 0.000000000000000000, 0.000000000000000000, 1.000000000000000000 ) ) ;
#62692=CARTESIAN_POINT ( 'NONE',  ( 1.339745962155612702, -68.29465819873851729, -5.000000000000000000 ) ) ;
#62701=CARTESIAN_POINT ( 'NONE',  ( -4.458734124999997661, 24.52083333469892779, 2.574251347313722516 ) ) ;
#62707=CARTESIAN_POINT ( 'NONE',  ( 1.339745962155612702, -80.29465819873850307, -5.000000000000000000 ) ) ;
#62708=CARTESIAN_POINT ( 'NONE',  ( -4.458734124999997661, 2.770833334698928674, 2.574251347313722516 ) ) ;
#62709=CARTESIAN_POINT ( 'NONE',  ( -4.458734124999999437, -22.64583333196773651, -2.574251347313719407 ) ) ;
#62710=CARTESIAN_POINT ( 'NONE',  ( 2.730187237215162345E-16, -154.1875000013656063, -4.458734124999999437 ) ) ;
#62713=( BOUNDED_CURVE ( )  B_SPLINE_CURVE ( 2, ( #24274, #63210, #9171, #168, #40015, #53551, #14935, #20086, #49676 ),
 .UNSPECIFIED., .F., .F. ) 
 B_SPLINE_CURVE_WITH_KNOTS ( ( 3, 2, 2, 2, 3 ),
 ( 0.9687500000000000000, 0.9694444444444444420, 0.9708333333333333259, 0.9722222222222222099, 0.9729166666666666519 ),
 .UNSPECIFIED. ) 
 CURVE ( )  GEOMETRIC_REPRESENTATION_ITEM ( )  RATIONAL_B_SPLINE_CURVE ( ( 0.9330127018922194093, 0.9330127018922194093, 1.000000000000000000, 0.8660254037844387076, 1.000000000000000000, 0.8660254037844387076, 1.000000000000000000, 0.9330127018922194093, 0.9330127018922194093 ) ) 
 REPRESENTATION_ITEM ( '' )  );
#62714=CARTESIAN_POINT ( 'NONE',  ( -2.498395430326213474E-14, 15.25000000000000000, 5.000000000000000000 ) ) ;
#62717=CARTESIAN_POINT ( 'NONE',  ( 2.229367062500001939, -66.22916666530106511, 3.861377020970579999 ) ) ;
#62719=CARTESIAN_POINT ( 'NONE',  ( -4.999999999999998224, -65.79166666393547303, 2.886751345948131764 ) ) ;
#62720=CARTESIAN_POINT ( 'NONE',  ( 1.060575238724906964E-15, 27.37500000273118062, 5.773502691896257311 ) ) ;
#62721=ORIENTED_EDGE ( 'NONE', *, *, #43698, .T. ) ;
#62725=CARTESIAN_POINT ( 'NONE',  ( 1.060575238724906964E-15, -11.74999999999999467, 5.773502691896257311 ) ) ;
#62726=CARTESIAN_POINT ( 'NONE',  ( -2.229367062499996610, -15.14583333196773474, 3.861377020970582219 ) ) ;
#62727=AXIS2_PLACEMENT_3D ( 'NONE', #25605, #15953, #21744 ) ;
#62728=CARTESIAN_POINT ( 'NONE',  ( -2.229367062499996610, -80.14583333196773651, 3.861377020970582219 ) ) ;
#62729=( BOUNDED_CURVE ( )  B_SPLINE_CURVE ( 2, ( #57288, #7444, #2309, #61162, #17085, #13204, #36705, #42155, #27052 ),
 .UNSPECIFIED., .F., .F. ) 
 B_SPLINE_CURVE_WITH_KNOTS ( ( 3, 2, 2, 2, 3 ),
 ( 0.9270833333333333703, 0.9277777777777778123, 0.9291666666666666963, 0.9305555555555555802, 0.9312500000000000222 ),
 .UNSPECIFIED. ) 
 CURVE ( )  GEOMETRIC_REPRESENTATION_ITEM ( )  RATIONAL_B_SPLINE_CURVE ( ( 0.9330127018922194093, 0.9330127018922194093, 1.000000000000000000, 0.8660254037844387076, 1.000000000000000000, 0.8660254037844387076, 1.000000000000000000, 0.9330127018922194093, 0.9330127018922194093 ) ) 
 REPRESENTATION_ITEM ( '' )  );
#62730=CARTESIAN_POINT ( 'NONE',  ( -4.458734125000001214, -168.1250000013656063, 1.846868145590734089 ) ) ;
#62731=CARTESIAN_POINT ( 'NONE',  ( -5.000000000000000000, -17.87499999726881583, 0.000000000000000000 ) ) ;
#62732=CARTESIAN_POINT ( 'NONE',  ( -3.152548672688508926E-16, -44.56249999863440081, -5.148502694627439702 ) ) ;
#62735=CARTESIAN_POINT ( 'NONE',  ( 4.458734124999999437, 6.937500001365594748, -5.460374474430324690E-16 ) ) ;
#62736=ORIENTED_EDGE ( 'NONE', *, *, #21575, .T. ) ;
#62738=CARTESIAN_POINT ( 'NONE',  ( 5.000000000000000000, -58.50000000000000000, -6.123233995736766282E-16 ) ) ;
#62739=CARTESIAN_POINT ( 'NONE',  ( 1.846868145590735200, -155.5000000013655779, -4.458734125000000326 ) ) ;
#62742=CARTESIAN_POINT ( 'NONE',  ( -3.535533905932737309, -166.6250000000000284, -3.535533905932738197 ) ) ;
#62744=CARTESIAN_POINT ( 'NONE',  ( -2.229367062499996610, -90.14583333196773651, 3.861377020970582219 ) ) ;
#62746=CARTESIAN_POINT ( 'NONE',  ( 2.229367062499998831, -4.895833331967740065, -3.861377020970580887 ) ) ;
#62747=CARTESIAN_POINT ( 'NONE',  ( 9.457646018065525792E-16, -39.31249999863439371, 5.148502694627439702 ) ) ;
#62749=CARTESIAN_POINT ( 'NONE',  ( -4.458734125000001214, -149.8750000013655779, 1.846868145590734089 ) ) ;
#62754=CARTESIAN_POINT ( 'NONE',  ( 0.000000000000000000, -170.0000000000000000, 0.000000000000000000 ) ) ;
#62755=CARTESIAN_POINT ( 'NONE',  ( 4.458734124999999437, -73.06249999863439371, -5.460374474430324690E-16 ) ) ;
#62756=ORIENTED_EDGE ( 'NONE', *, *, #60430, .T. ) ;
#62759=CARTESIAN_POINT ( 'NONE',  ( 5.000000000000000888, -79.45833333060213022, 2.886751345948126879 ) ) ;
#62760=CARTESIAN_POINT ( 'NONE',  ( 2.229367062499998831, 2.354166668032262599, -3.861377020970580887 ) ) ;
#62762=CARTESIAN_POINT ( 'NONE',  ( 4.458734124999999437, -151.3750000013656063, -1.846868145590734978 ) ) ;
#62769=DIRECTION ( 'NONE',  ( -0.000000000000000000, 1.000000000000000000, -0.000000000000000000 ) ) ;
#62775=CARTESIAN_POINT ( 'NONE',  ( 5.000000000000000000, -44.50000000000000000, -6.123233995736766282E-16 ) ) ;
#62776=CARTESIAN_POINT ( 'NONE',  ( -4.458734124999999437, 22.60416666803225993, -2.574251347313719407 ) ) ;
#62778=CARTESIAN_POINT ( 'NONE',  ( 2.229367062500001939, -11.22916666530107044, 3.861377020970579999 ) ) ;
#62779=( BOUNDED_CURVE ( )  B_SPLINE_CURVE ( 2, ( #3474, #8604, #51415, #27279, #43010, #23087, #46586, #42690, #2529 ),
 .UNSPECIFIED., .F., .F. ) 
 B_SPLINE_CURVE_WITH_KNOTS ( ( 3, 2, 2, 2, 3 ),
 ( 0.4604166666666666963, 0.4611111111111111382, 0.4625000000000000222, 0.4638888888888889062, 0.4645833333333333481 ),
 .UNSPECIFIED. ) 
 CURVE ( )  GEOMETRIC_REPRESENTATION_ITEM ( )  RATIONAL_B_SPLINE_CURVE ( ( 0.9330127018922194093, 0.9330127018922220739, 1.000000000000000000, 0.8660254037844387076, 1.000000000000000000, 0.8660254037844387076, 1.000000000000000000, 0.9330127018922194093, 0.9330127018922194093 ) ) 
 REPRESENTATION_ITEM ( '' )  );
#62780=CARTESIAN_POINT ( 'NONE',  ( -9.184850993605147944E-16, -149.3750000027312126, 5.000000000000000000 ) ) ;
#62782=CARTESIAN_POINT ( 'NONE',  ( 4.458734124999999437, -166.5000000013655779, 1.846868145590737864 ) ) ;
#62790=CARTESIAN_POINT ( 'NONE',  ( -4.458734125000000326, -157.1250000013656063, 1.846868145590734089 ) ) ;
#62792=FACE_OUTER_BOUND ( 'NONE', #49432, .T. ) ;
#62794=CARTESIAN_POINT ( 'NONE',  ( 3.061616997868383141E-16, -162.7500000000000000, -5.000000000000000000 ) ) ;
#62795=ORIENTED_EDGE ( 'NONE', *, *, #812, .T. ) ;
#62799=CARTESIAN_POINT ( 'NONE',  ( 2.500000000000002220, 12.33333333333333215, 4.330127018922192761 ) ) ;
#62800=CARTESIAN_POINT ( 'NONE',  ( 1.060575238724906964E-15, 1.250000000000001110, 5.773502691896257311 ) ) ;
#62801=CARTESIAN_POINT ( 'NONE',  ( 9.457646018065525792E-16, -64.06249999863440792, 5.148502694627439702 ) ) ;
#62802=CARTESIAN_POINT ( 'NONE',  ( -5.000000000000000000, -8.000000000000000000, 0.000000000000000000 ) ) ;
#62803=CARTESIAN_POINT ( 'NONE',  ( 2.500000000000002220, 1.458333336064519203, 4.330127018922192761 ) ) ;
#62804=CARTESIAN_POINT ( 'NONE',  ( 2.229367062499998831, -29.64583333196773296, -3.861377020970580887 ) ) ;
#62806=CARTESIAN_POINT ( 'NONE',  ( 6.042630808230842148E-15, 25.87500000273118062, -4.999999999999999112 ) ) ;
#62808=CARTESIAN_POINT ( 'NONE',  ( 5.000000000000000000, -45.50000000000000000, -6.123233995736766282E-16 ) ) ;
#62809=( BOUNDED_CURVE ( )  B_SPLINE_CURVE ( 2, ( #12550, #2922, #60506, #51487, #27034, #46651, #32162, #22216, #30903 ),
 .UNSPECIFIED., .F., .F. ) 
 B_SPLINE_CURVE_WITH_KNOTS ( ( 3, 2, 2, 2, 3 ),
 ( 0.07708333333333333703, 0.07777777777777777901, 0.07916666666666666297, 0.08055555555555556080, 0.08125000000000000278 ),
 .UNSPECIFIED. ) 
 CURVE ( )  GEOMETRIC_REPRESENTATION_ITEM ( )  RATIONAL_B_SPLINE_CURVE ( ( 0.9330127018922194093, 0.9330127018922194093, 1.000000000000000000, 0.8660254037844387076, 1.000000000000000000, 0.8660254037844387076, 1.000000000000000000, 0.9330127018922194093, 0.9330127018922194093 ) ) 
 REPRESENTATION_ITEM ( '' )  );
#62810=CARTESIAN_POINT ( 'NONE',  ( -1.339745962155613812, -45.20534180126146850, -5.000000000000000000 ) ) ;
#62812=CARTESIAN_POINT ( 'NONE',  ( 0.000000000000000000, -170.0000000000000000, 5.000000000000000000 ) ) ;
#62813=CARTESIAN_POINT ( 'NONE',  ( -2.229367062500000163, -68.47916666530107932, -3.861377020970580443 ) ) ;
#62814=CARTESIAN_POINT ( 'NONE',  ( 1.846868145590736310, -149.8750000013655779, 4.458734124999999437 ) ) ;
#62816=CARTESIAN_POINT ( 'NONE',  ( 4.458734125000001214, -77.89583333196773651, 2.574251347313718519 ) ) ;
#62819=CARTESIAN_POINT ( 'NONE',  ( -2.229367062499996610, -22.39583333196773651, 3.861377020970582219 ) ) ;
#62820=CARTESIAN_POINT ( 'NONE',  ( -2.500000000000000444, -65.04166666393547303, -4.330127018922193649 ) ) ;
#62821=ORIENTED_EDGE ( 'NONE', *, *, #380, .T. ) ;
#62822=CARTESIAN_POINT ( 'NONE',  ( 2.500000000000002220, -1.666666666666663410, 4.330127018922192761 ) ) ;
#62827=ORIENTED_EDGE ( 'NONE', *, *, #38843, .F. ) ;
#62829=CARTESIAN_POINT ( 'NONE',  ( -2.229367062500000163, -53.72916666530107221, -3.861377020970580443 ) ) ;
#62831=VERTEX_POINT ( 'NONE', #34791 ) ;
#62834=EDGE_CURVE ( 'NONE', #18181, #56895, #58293, .T. ) ;
#62835=CARTESIAN_POINT ( 'NONE',  ( 4.458734125000001214, 19.10416666803225638, 2.574251347313718519 ) ) ;
#62837=CARTESIAN_POINT ( 'NONE',  ( 0.000000000000000000, -170.0000000000000000, 5.000000000000000000 ) ) ;
#62838=CARTESIAN_POINT ( 'NONE',  ( -3.152801135295367985, -165.8125000013656063, 3.152801135295367096 ) ) ;
#62839=ORIENTED_EDGE ( 'NONE', *, *, #30819, .T. ) ;
#62843=ADVANCED_FACE ( 'NONE', ( #30595 ), #40251, .T. ) ;
#62844=CARTESIAN_POINT ( 'NONE',  ( -2.500000000000000444, 1.833333333333332593, -4.330127018922193649 ) ) ;
#62849=DIRECTION ( 'NONE',  ( 0.000000000000000000, 0.000000000000000000, 1.000000000000000000 ) ) ;
#62854=CARTESIAN_POINT ( 'NONE',  ( 1.339745962155637349, 11.70534180126147739, -4.999999999999985789 ) ) ;
#62856=CARTESIAN_POINT ( 'NONE',  ( -5.000000000000000888, -154.6875000027312126, -2.071067811865475949 ) ) ;
#62857=ORIENTED_EDGE ( 'NONE', *, *, #8739, .T. ) ;
#62862=CARTESIAN_POINT ( 'NONE',  ( 5.000000000000000888, -144.9375000000000000, -2.071067811865475505 ) ) ;
#62863=ADVANCED_FACE ( 'NONE', ( #59891 ), #29952, .T. ) ;
#62865=CARTESIAN_POINT ( 'NONE',  ( -1.846868145590734756, -169.3750000013656347, -4.458734124999999437 ) ) ;
#62866=CARTESIAN_POINT ( 'NONE',  ( 9.457646018065525792E-16, -32.06249999863440792, 5.148502694627439702 ) ) ;
#62870=CARTESIAN_POINT ( 'NONE',  ( -3.152801135295367985, -149.8125000013655779, 3.152801135295367096 ) ) ;
#62871=EDGE_LOOP ( 'NONE', ( #5228, #43654, #11696, #47051 ) ) ;
#62873=CARTESIAN_POINT ( 'NONE',  ( -4.458734124999999437, -59.56249999863440081, 0.000000000000000000 ) ) ;
#62875=CARTESIAN_POINT ( 'NONE',  ( 5.000000000000000888, 13.54166666939785202, 2.886751345948126879 ) ) ;
#62876=CARTESIAN_POINT ( 'NONE',  ( -4.999999999999999112, 17.08333333333333215, 2.886751345948131764 ) ) ;
#62878=CARTESIAN_POINT ( 'NONE',  ( -3.152548672688508926E-16, -4.562499998634401699, -5.148502694627439702 ) ) ;
#62881=CARTESIAN_POINT ( 'NONE',  ( 2.229367062500001939, 9.770833334698927786, 3.861377020970579999 ) ) ;
#62882=CARTESIAN_POINT ( 'NONE',  ( 5.000000000000000000, -53.29166666393548013, -2.886751345948130876 ) ) ;
#62883=VERTEX_POINT ( 'NONE', #50216 ) ;
#62885=CARTESIAN_POINT ( 'NONE',  ( -4.458734124999999437, -49.39583333196773651, -2.574251347313719407 ) ) ;
#62886=CARTESIAN_POINT ( 'NONE',  ( 2.730187237215162345E-16, -161.4375000013655779, -4.458734124999999437 ) ) ;
#62888=CARTESIAN_POINT ( 'NONE',  ( -5.000000000000000000, -51.87499999726881583, 0.000000000000000000 ) ) ;
#62890=CARTESIAN_POINT ( 'NONE',  ( -4.458734124999999437, -22.39583333196773651, -2.574251347313719407 ) ) ;
#62891=VERTEX_POINT ( 'NONE', #57424 ) ;
#62894=CARTESIAN_POINT ( 'NONE',  ( 2.730187237215162345E-16, -159.1875000013655779, -4.458734124999999437 ) ) ;
#62898=CARTESIAN_POINT ( 'NONE',  ( -1.339745962155610925, -58.66965819600732601, 5.000000000000000000 ) ) ;
#62899=CARTESIAN_POINT ( 'NONE',  ( -4.458734124999998549, -37.47916666530107221, 2.574251347313722516 ) ) ;
#62908=EDGE_CURVE ( 'NONE', #53313, #34331, #45512, .T. ) ;
#62909=CARTESIAN_POINT ( 'NONE',  ( -4.458734124999999437, -84.64583333196773651, -2.574251347313719407 ) ) ;
#62921=CARTESIAN_POINT ( 'NONE',  ( -5.000000000000000000, -45.95833333060214443, -2.886751345948128211 ) ) ;
#62922=CARTESIAN_POINT ( 'NONE',  ( -4.458734124999998549, -83.47916666530107932, 2.574251347313722516 ) ) ;
#62926=CARTESIAN_POINT ( 'NONE',  ( -4.999999999999998224, -80.91666666666667140, 2.886751345948131764 ) ) ;
#62928=CARTESIAN_POINT ( 'NONE',  ( -3.535533905932738641, -164.5000000027312126, 3.535533905932737309 ) ) ;
#62930=EDGE_CURVE ( 'NONE', #2867, #33297, #61934, .T. ) ;
#62932=CARTESIAN_POINT ( 'NONE',  ( -6.972266317189433020E-16, -39.12499999726880162, -5.000000000000000000 ) ) ;
#62938=CARTESIAN_POINT ( 'NONE',  ( 2.499999999999998668, -86.20833333060214443, -4.330127018922193649 ) ) ;
#62940=CARTESIAN_POINT ( 'NONE',  ( -2.229367062499996610, -14.14583333196774184, 3.861377020970582219 ) ) ;
#62942=VERTEX_POINT ( 'NONE', #32012 ) ;
#62943=CARTESIAN_POINT ( 'NONE',  ( 9.457646018065525792E-16, -43.31249999863440792, 5.148502694627439702 ) ) ;
#62949=CARTESIAN_POINT ( 'NONE',  ( -2.229367062500000163, 16.52083333469892779, -3.861377020970580443 ) ) ;
#62950=CARTESIAN_POINT ( 'NONE',  ( -2.499999999999996447, -81.70833333060213022, 4.330127018922195425 ) ) ;
#62951=CARTESIAN_POINT ( 'NONE',  ( 0.000000000000000000, -170.0000000000000000, 0.000000000000000000 ) ) ;
#62952=CARTESIAN_POINT ( 'NONE',  ( -4.458734124999999437, -88.56249999863439371, 0.000000000000000000 ) ) ;
#62955=CARTESIAN_POINT ( 'NONE',  ( -3.535250795749689387E-16, 13.87500000273118417, -5.773502691896257311 ) ) ;
#62956=ORIENTED_EDGE ( 'NONE', *, *, #15431, .F. ) ;
#62962=CARTESIAN_POINT ( 'NONE',  ( 5.000000000000000000, -30.50000000000000000, -6.123233995736766282E-16 ) ) ;
#62963=CARTESIAN_POINT ( 'NONE',  ( -4.458734124999999437, -33.39583333196772941, -2.574251347313719407 ) ) ;
#62965=CARTESIAN_POINT ( 'NONE',  ( 5.000000000000000000, -33.37499999726880873, -6.123233995736766282E-16 ) ) ;
#62967=CARTESIAN_POINT ( 'NONE',  ( -4.458734124999999437, -63.31249999863440792, 0.000000000000000000 ) ) ;
#62970=CARTESIAN_POINT ( 'NONE',  ( -4.458734124999999437, -14.56249999863440436, 0.000000000000000000 ) ) ;
#62973=CARTESIAN_POINT ( 'NONE',  ( 2.499999999999998668, -79.33333333333332860, -4.330127018922193649 ) ) ;
#62974=CARTESIAN_POINT ( 'NONE',  ( 2.500000000000002220, 28.45833333606451987, 4.330127018922192761 ) ) ;
#62977=CARTESIAN_POINT ( 'NONE',  ( -5.000000000000000000, -83.95833333060214443, -2.886751345948128211 ) ) ;
#62979=ORIENTED_EDGE ( 'NONE', *, *, #49457, .F. ) ;
#62982=CARTESIAN_POINT ( 'NONE',  ( 9.457646018065525792E-16, -23.31249999863440436, 5.148502694627439702 ) ) ;
#62983=EDGE_CURVE ( 'NONE', #40265, #30447, #3705, .T. ) ;
#62984=CARTESIAN_POINT ( 'NONE',  ( -3.152548672688508926E-16, -59.81249999863440792, -5.148502694627439702 ) ) ;
#62987=CARTESIAN_POINT ( 'NONE',  ( 2.730187237215162345E-16, -166.4375000013655779, -4.458734124999999437 ) ) ;
#62988=ADVANCED_FACE ( 'NONE', ( #52589 ), #26881, .T. ) ;
#62990=CARTESIAN_POINT ( 'NONE',  ( -5.000000000000000000, 17.91666666666666430, -2.886751345948128211 ) ) ;
#62991=( BOUNDED_CURVE ( )  B_SPLINE_CURVE ( 2, ( #55121, #11045, #16515, #31294, #30670, #55445, #50289, #16194, #6237 ),
 .UNSPECIFIED., .F., .F. ) 
 B_SPLINE_CURVE_WITH_KNOTS ( ( 3, 2, 2, 2, 3 ),
 ( 0.2645833333333333370, 0.2652777777777777790, 0.2666666666666666630, 0.2680555555555555469, 0.2687499999999999889 ),
 .UNSPECIFIED. ) 
 CURVE ( )  GEOMETRIC_REPRESENTATION_ITEM ( )  RATIONAL_B_SPLINE_CURVE ( ( 0.9330127018922194093, 0.9330127018922194093, 1.000000000000000000, 0.8660254037844387076, 1.000000000000000000, 0.8660254037844387076, 1.000000000000000000, 0.9330127018922194093, 0.9330127018922194093 ) ) 
 REPRESENTATION_ITEM ( '' )  );
#63002=CARTESIAN_POINT ( 'NONE',  ( -4.458734124999999437, -143.1875000013656063, -5.460374474430324690E-16 ) ) ;
#63006=CARTESIAN_POINT ( 'NONE',  ( -2.229367062500000163, -70.72916666530107932, -3.861377020970580443 ) ) ;
#63008=CARTESIAN_POINT ( 'NONE',  ( -5.000000000000000000, -42.95833333060214443, -2.886751345948128211 ) ) ;
#63009=CARTESIAN_POINT ( 'NONE',  ( -8.190561711645485556E-16, -140.6875000013656063, 4.458734124999999437 ) ) ;
#63010=( BOUNDED_CURVE ( )  B_SPLINE_CURVE ( 2, ( #23220, #18395, #51862, #7805, #48913, #24479, #43455, #34430, #9996 ),
 .UNSPECIFIED., .F., .F. ) 
 B_SPLINE_CURVE_WITH_KNOTS ( ( 3, 2, 2, 2, 3 ),
 ( 0.4145833333333333592, 0.4152777777777778012, 0.4166666666666666852, 0.4180555555555555691, 0.4187500000000000111 ),
 .UNSPECIFIED. ) 
 CURVE ( )  GEOMETRIC_REPRESENTATION_ITEM ( )  RATIONAL_B_SPLINE_CURVE ( ( 0.9330127018922194093, 0.9330127018922220739, 1.000000000000000000, 0.8660254037844387076, 1.000000000000000000, 0.8660254037844387076, 1.000000000000000000, 0.9330127018922194093, 0.9330127018922194093 ) ) 
 REPRESENTATION_ITEM ( '' )  );
#63013=LINE ( 'NONE', #48822, #19223 ) ;
#63014=CARTESIAN_POINT ( 'NONE',  ( -9.184850993605147944E-16, -160.2500000000000000, 5.000000000000000000 ) ) ;
#63019=CARTESIAN_POINT ( 'NONE',  ( 2.229367062499998831, 25.10416666803225993, -3.861377020970580887 ) ) ;
#63020=AXIS2_PLACEMENT_3D ( 'NONE', #7388, #36015, #61105 ) ;
#63026=CARTESIAN_POINT ( 'NONE',  ( -4.458734124999999437, 0.6875000013655957476, 0.000000000000000000 ) ) ;
#63027=CARTESIAN_POINT ( 'NONE',  ( -4.458734124999999437, -26.64583333196774007, -2.574251347313719407 ) ) ;
#63028=CARTESIAN_POINT ( 'NONE',  ( -1.846868145590737420, -155.7500000013655779, 4.458734124999999437 ) ) ;
#63034=CARTESIAN_POINT ( 'NONE',  ( 4.458734124999998549, -71.97916666530107932, -2.574251347313721627 ) ) ;
#63037=CARTESIAN_POINT ( 'NONE',  ( -3.535250795749689387E-16, 28.87500000273118417, -5.773502691896257311 ) ) ;
#63038=EDGE_LOOP ( 'NONE', ( #50895, #3704, #26992, #54482 ) ) ;
#63039=CARTESIAN_POINT ( 'NONE',  ( -9.184850993605147944E-16, -140.2500000000000000, 5.000000000000000000 ) ) ;
#63041=CARTESIAN_POINT ( 'NONE',  ( -3.535250795749689387E-16, -12.24999999999999645, -5.773502691896257311 ) ) ;
#63042=CARTESIAN_POINT ( 'NONE',  ( -2.229367062499996610, -16.14583333196773651, 3.861377020970582219 ) ) ;
#63043=CARTESIAN_POINT ( 'NONE',  ( -2.229367062499996610, -77.14583333196773651, 3.861377020970582219 ) ) ;
#63044=CARTESIAN_POINT ( 'NONE',  ( -4.458734125000000326, -166.2500000013656347, -1.846868145590735644 ) ) ;
#63045=CARTESIAN_POINT ( 'NONE',  ( -4.999999999999999112, -17.79166666393547658, 2.886751345948131764 ) ) ;
#63046=CARTESIAN_POINT ( 'NONE',  ( 4.458734124999998549, -42.72916666530107221, -2.574251347313721627 ) ) ;
#63047=EDGE_LOOP ( 'NONE', ( #41434, #10342, #57890, #19351 ) ) ;
#63049=CARTESIAN_POINT ( 'NONE',  ( 9.457646018065525792E-16, 3.687500001365594748, 5.148502694627439702 ) ) ;
#63050=ORIENTED_EDGE ( 'NONE', *, *, #47318, .F. ) ;
#63052=CARTESIAN_POINT ( 'NONE',  ( -4.999999999999999112, -61.91666666666665719, 2.886751345948131764 ) ) ;
#63053=CARTESIAN_POINT ( 'NONE',  ( 4.458734124999999437, -154.6875000013656063, 0.000000000000000000 ) ) ;
#63055=CARTESIAN_POINT ( 'NONE',  ( 5.000000000000000000, -161.0624999999999716, 2.071067811865478614 ) ) ;
#63056=CARTESIAN_POINT ( 'NONE',  ( 3.535533905932736864, -168.1250000000000284, 3.535533905932738641 ) ) ;
#63058=CARTESIAN_POINT ( 'NONE',  ( -3.152548672688508926E-16, -7.812499998634405252, -5.148502694627439702 ) ) ;
#63059=CARTESIAN_POINT ( 'NONE',  ( 2.229367062500001939, -42.22916666530107932, 3.861377020970579999 ) ) ;
#63060=VECTOR ( 'NONE', #56834, 1000.000000000000000 ) ;
#63062=CARTESIAN_POINT ( 'NONE',  ( -4.458734124999999437, -149.9375000013656063, -5.460374474430324690E-16 ) ) ;
#63065=VERTEX_POINT ( 'NONE', #48684 ) ;
#63070=CARTESIAN_POINT ( 'NONE',  ( 2.229367062500001939, -73.22916666530107932, 3.861377020970579999 ) ) ;
#63073=DIRECTION ( 'NONE',  ( 0.000000000000000000, 0.000000000000000000, 1.000000000000000000 ) ) ;
#63077=CARTESIAN_POINT ( 'NONE',  ( 4.458734124999999437, -1.812499998634406584, -5.460374474430324690E-16 ) ) ;
#63078=CARTESIAN_POINT ( 'NONE',  ( -2.500000000000000444, -43.16666666666665719, -4.330127018922193649 ) ) ;
#63079=CARTESIAN_POINT ( 'NONE',  ( -4.458734125000000326, -152.8750000013655779, 1.846868145590734089 ) ) ;
#63088=( BOUNDED_CURVE ( )  B_SPLINE_CURVE ( 2, ( #50308, #44515, #19758, #59000, #14928, #20079, #16220, #1129, #39684 ),
 .UNSPECIFIED., .F., .F. ) 
 B_SPLINE_CURVE_WITH_KNOTS ( ( 3, 2, 2, 2, 3 ),
 ( 0.4687500000000000000, 0.4694444444444444420, 0.4708333333333333259, 0.4722222222222222099, 0.4729166666666666519 ),
 .UNSPECIFIED. ) 
 CURVE ( )  GEOMETRIC_REPRESENTATION_ITEM ( )  RATIONAL_B_SPLINE_CURVE ( ( 0.9330127018922194093, 0.9330127018922194093, 1.000000000000000000, 0.8660254037844387076, 1.000000000000000000, 0.8660254037844387076, 1.000000000000000000, 0.9330127018922194093, 0.9330127018922194093 ) ) 
 REPRESENTATION_ITEM ( '' )  );
#63093=VERTEX_POINT ( 'NONE', #40236 ) ;
#63094=CARTESIAN_POINT ( 'NONE',  ( -4.458734124999997661, 15.77083333469892601, 2.574251347313722516 ) ) ;
#63096=CARTESIAN_POINT ( 'NONE',  ( 4.458734124999999437, -8.062499998634404363, -5.460374474430324690E-16 ) ) ;
#63099=CARTESIAN_POINT ( 'NONE',  ( -3.152801135295367096, -167.0625000013656063, -3.152801135295367541 ) ) ;
#63108=CARTESIAN_POINT ( 'NONE',  ( 4.458734124999999437, -155.6250000013655779, -1.846868145590734978 ) ) ;
#63111=DIRECTION ( 'NONE',  ( -0.000000000000000000, 1.000000000000000000, -0.000000000000000000 ) ) ;
#63112=ORIENTED_EDGE ( 'NONE', *, *, #56989, .T. ) ;
#63117=CARTESIAN_POINT ( 'NONE',  ( 5.000000000000000000, 0.5000000000000004441, -6.123233995736766282E-16 ) ) ;
#63118=CARTESIAN_POINT ( 'NONE',  ( -2.229367062499996610, -59.14583333196773651, 3.861377020970582219 ) ) ;
#63119=ADVANCED_FACE ( 'NONE', ( #59873 ), #10639, .T. ) ;
#63121=CARTESIAN_POINT ( 'NONE',  ( 2.499999999999998668, -3.208333330602147093, -4.330127018922193649 ) ) ;
#63122=CARTESIAN_POINT ( 'NONE',  ( 2.229367062500001939, -30.97916666530107221, 3.861377020970579999 ) ) ;
#63126=CARTESIAN_POINT ( 'NONE',  ( -5.000000000000000000, -45.08333333333333570, -2.886751345948128211 ) ) ;
#63129=CARTESIAN_POINT ( 'NONE',  ( -6.972266317189433020E-16, 24.87500000273118417, -5.000000000000000000 ) ) ;
#63130=CARTESIAN_POINT ( 'NONE',  ( -4.458734124999999437, -71.31249999863439371, 0.000000000000000000 ) ) ;
#63131=CARTESIAN_POINT ( 'NONE',  ( -4.458734125000000326, -144.2500000013656063, -1.846868145590735644 ) ) ;
#63132=CARTESIAN_POINT ( 'NONE',  ( 4.458734124999999437, -76.81249999863440792, -5.460374474430324690E-16 ) ) ;
#63134=CARTESIAN_POINT ( 'NONE',  ( 4.458734124999999437, -23.06249999863440436, -5.460374474430324690E-16 ) ) ;
#63135=CARTESIAN_POINT ( 'NONE',  ( -4.999999999999999112, -66.79166666393548724, 2.886751345948131764 ) ) ;
#63137=CARTESIAN_POINT ( 'NONE',  ( -3.535533905932737309, -152.7500000027312126, -3.535533905932738197 ) ) ;
#63140=CARTESIAN_POINT ( 'NONE',  ( 5.000000000000000888, 28.41666666666666430, 2.886751345948126879 ) ) ;
#63141=ORIENTED_EDGE ( 'NONE', *, *, #48881, .F. ) ;
#63142=CARTESIAN_POINT ( 'NONE',  ( 0.000000000000000000, -170.0000000000000000, 0.000000000000000000 ) ) ;
#63143=CARTESIAN_POINT ( 'NONE',  ( 4.458734124999998549, -60.97916666530106511, -2.574251347313721627 ) ) ;
#63146=AXIS2_PLACEMENT_3D ( 'NONE', #55696, #50217, #30917 ) ;
#63148=CARTESIAN_POINT ( 'NONE',  ( -4.458734124999998549, 17.77083333469892779, 2.574251347313722516 ) ) ;
#63151=CARTESIAN_POINT ( 'NONE',  ( 1.846868145590735200, -163.2500000013656063, -4.458734124999999437 ) ) ;
#63152=( BOUNDED_CURVE ( )  B_SPLINE_CURVE ( 2, ( #51474, #37303, #31515, #36352, #32472, #17054, #12227, #52101, #51158 ),
 .UNSPECIFIED., .F., .F. ) 
 B_SPLINE_CURVE_WITH_KNOTS ( ( 3, 2, 2, 2, 3 ),
 ( 0.7104166666666666963, 0.7111111111111111382, 0.7125000000000000222, 0.7138888888888889062, 0.7145833333333333481 ),
 .UNSPECIFIED. ) 
 CURVE ( )  GEOMETRIC_REPRESENTATION_ITEM ( )  RATIONAL_B_SPLINE_CURVE ( ( 0.9330127018922194093, 0.9330127018922194093, 1.000000000000000000, 0.8660254037844387076, 1.000000000000000000, 0.8660254037844387076, 1.000000000000000000, 0.9330127018922194093, 0.9330127018922194093 ) ) 
 REPRESENTATION_ITEM ( '' )  );
#63155=CARTESIAN_POINT ( 'NONE',  ( 3.061616997868383141E-16, -153.7500000000000000, -5.000000000000000000 ) ) ;
#63157=CARTESIAN_POINT ( 'NONE',  ( -6.972266317189433020E-16, 4.875000002731184168, -5.000000000000000000 ) ) ;
#63166=CARTESIAN_POINT ( 'NONE',  ( -4.458734124999999437, 9.437500001365593860, 0.000000000000000000 ) ) ;
#63169=CARTESIAN_POINT ( 'NONE',  ( -5.000000000000000888, -147.6875000027312126, -2.071067811865475949 ) ) ;
#63175=CARTESIAN_POINT ( 'NONE',  ( -5.000000000000000888, -141.5625000000000568, -2.071067811865475949 ) ) ;
#63177=CARTESIAN_POINT ( 'NONE',  ( -1.339745962155613812, -55.20534180126147561, -5.000000000000000000 ) ) ;
#63178=CARTESIAN_POINT ( 'NONE',  ( -2.229367062499996610, -31.14583333196773651, 3.861377020970582219 ) ) ;
#63180=DIRECTION ( 'NONE',  ( -0.000000000000000000, 1.000000000000000000, -0.000000000000000000 ) ) ;
#63182=CARTESIAN_POINT ( 'NONE',  ( -3.152801135295367096, -143.0625000013655779, -3.152801135295367541 ) ) ;
#63184=CARTESIAN_POINT ( 'NONE',  ( -2.229367062499996610, 26.60416666803225993, 3.861377020970582219 ) ) ;
#63186=CARTESIAN_POINT ( 'NONE',  ( 4.458734125000000326, -56.14583333196773651, 2.574251347313718519 ) ) ;
#63189=CARTESIAN_POINT ( 'NONE',  ( 1.339745962155615144, 13.41965820146970501, 4.999999999999999112 ) ) ;
#63190=CARTESIAN_POINT ( 'NONE',  ( -5.000000000000000000, 19.91666666666666785, -2.886751345948128211 ) ) ;
#63191=CARTESIAN_POINT ( 'NONE',  ( -5.000000000000000000, -36.95833333060213022, -2.886751345948128211 ) ) ;
#63193=CARTESIAN_POINT ( 'NONE',  ( -4.458734124999999437, -8.312499998634406140, 0.000000000000000000 ) ) ;
#63194=CARTESIAN_POINT ( 'NONE',  ( -5.000000000000000888, -168.4375000000001137, 2.071067811865474617 ) ) ;
#63195=CARTESIAN_POINT ( 'NONE',  ( 2.071067811865433317, -164.9375000027311842, -5.000000000000041744 ) ) ;
#63197=CARTESIAN_POINT ( 'NONE',  ( 6.123233995736766282E-16, -170.0000000000000000, -5.000000000000000000 ) ) ;
#63200=CARTESIAN_POINT ( 'NONE',  ( -2.229367062499996610, -54.14583333196773651, 3.861377020970582219 ) ) ;
#63201=CARTESIAN_POINT ( 'NONE',  ( -4.458734125000000326, -159.2500000013656063, -1.846868145590735644 ) ) ;
#63202=CARTESIAN_POINT ( 'NONE',  ( -2.500000000000000444, -48.04166666393547303, -4.330127018922193649 ) ) ;
#63204=CARTESIAN_POINT ( 'NONE',  ( -4.458734124999999437, 6.354166668032259047, -2.574251347313719407 ) ) ;
#63205=ORIENTED_EDGE ( 'NONE', *, *, #56159, .F. ) ;
#63208=CARTESIAN_POINT ( 'NONE',  ( 1.846868145590736310, -159.6250000013656063, 4.458734124999999437 ) ) ;
#63210=CARTESIAN_POINT ( 'NONE',  ( 1.339745962155612702, -87.16965819600731891, -5.000000000000000000 ) ) ;
#63212=CARTESIAN_POINT ( 'NONE',  ( -1.339745962155613812, -59.08034179853028434, -5.000000000000000000 ) ) ;
#63213=CARTESIAN_POINT ( 'NONE',  ( 2.229367062499998831, -41.89583333196773651, -3.861377020970580887 ) ) ;
#63214=ORIENTED_EDGE ( 'NONE', *, *, #29103, .F. ) ;
#63215=CARTESIAN_POINT ( 'NONE',  ( 3.061616997868383141E-16, -142.8750000027312126, -5.000000000000000000 ) ) ;
#63217=DIRECTION ( 'NONE',  ( -0.000000000000000000, 1.000000000000000000, -0.000000000000000000 ) ) ;
#63219=CARTESIAN_POINT ( 'NONE',  ( -4.458734124999999437, -87.56249999863439371, 0.000000000000000000 ) ) ;
#63223=CARTESIAN_POINT ( 'NONE',  ( 1.339745962155615144, -52.58034179853029144, 4.999999999999999112 ) ) ;
#63229=CARTESIAN_POINT ( 'NONE',  ( -1.339745962155613812, -82.20534180126146850, -5.000000000000000000 ) ) ;
#63232=CARTESIAN_POINT ( 'NONE',  ( -6.972266317189433020E-16, -6.249999999999999112, -5.000000000000000000 ) ) ;
#63234=CARTESIAN_POINT ( 'NONE',  ( 4.458734125000001214, -83.14583333196773651, 2.574251347313718519 ) ) ;
#63238=CARTESIAN_POINT ( 'NONE',  ( -4.999999999999998224, -16.79166666393548368, 2.886751345948131764 ) ) ;
#63240=CARTESIAN_POINT ( 'NONE',  ( 5.000000000000000000, -160.1250000027311842, 0.000000000000000000 ) ) ;
#63244=DIRECTION ( 'NONE',  ( 0.000000000000000000, 0.000000000000000000, 1.000000000000000000 ) ) ;
#63250=CARTESIAN_POINT ( 'NONE',  ( 4.458734125000000326, -15.89583333196773651, 2.574251347313718519 ) ) ;
#63251=DIRECTION ( 'NONE',  ( -0.000000000000000000, 1.000000000000000000, -0.000000000000000000 ) ) ;
#63252=CARTESIAN_POINT ( 'NONE',  ( 2.071067811865475505, -153.8125000000000000, -5.000000000000000888 ) ) ;
#63254=CARTESIAN_POINT ( 'NONE',  ( 2.229367062499998831, -42.89583333196773651, -3.861377020970580887 ) ) ;
#63255=CARTESIAN_POINT ( 'NONE',  ( 2.499999999999998668, -83.20833333060214443, -4.330127018922193649 ) ) ;
#63261=CARTESIAN_POINT ( 'NONE',  ( -3.152548672688508926E-16, 11.43750000136559386, -5.148502694627439702 ) ) ;
#63263=EDGE_CURVE ( 'NONE', #43626, #18601, #37007, .T. ) ;
#63265=CARTESIAN_POINT ( 'NONE',  ( 2.229367062499998831, -87.89583333196773651, -3.861377020970580887 ) ) ;
#63267=CARTESIAN_POINT ( 'NONE',  ( 2.499999999999998668, 14.79166666939785202, -4.330127018922193649 ) ) ;
#63271=CARTESIAN_POINT ( 'NONE',  ( 1.339745962155615144, -85.70534180126146850, 4.999999999999999112 ) ) ;
#63272=CARTESIAN_POINT ( 'NONE',  ( -3.535250795749689387E-16, -36.25000000000000711, -5.773502691896257311 ) ) ;
#63273=CARTESIAN_POINT ( 'NONE',  ( 4.458734124999999437, -35.81249999863440792, -5.460374474430324690E-16 ) ) ;
#63276=CARTESIAN_POINT ( 'NONE',  ( 1.060575238724906964E-15, -36.62499999726880873, 5.773502691896257311 ) ) ;
#63277=CARTESIAN_POINT ( 'NONE',  ( -4.458734124999999437, -67.39583333196773651, -2.574251347313719407 ) ) ;
#63280=CARTESIAN_POINT ( 'NONE',  ( 4.458734124999999437, -13.81249999863440259, -5.460374474430324690E-16 ) ) ;
#63281=CARTESIAN_POINT ( 'NONE',  ( 9.457646018065525792E-16, -14.31249999863440259, 5.148502694627439702 ) ) ;
#63282=EDGE_LOOP ( 'NONE', ( #48682, #3346, #10510, #10612 ) ) ;
#63283=CARTESIAN_POINT ( 'NONE',  ( -2.499999999999996447, -75.83333333333334281, 4.330127018922195425 ) ) ;
#63286=CARTESIAN_POINT ( 'NONE',  ( -2.500000000000000444, -80.04166666393547303, -4.330127018922193649 ) ) ;
#63289=CARTESIAN_POINT ( 'NONE',  ( 4.458734124999999437, -24.06249999863440436, -5.460374474430324690E-16 ) ) ;
#63290=ORIENTED_EDGE ( 'NONE', *, *, #10316, .T. ) ;
#63291=CARTESIAN_POINT ( 'NONE',  ( -3.152801135295367985, -168.0625000013656063, 3.152801135295367096 ) ) ;
#63292=EDGE_CURVE ( 'NONE', #13678, #16051, #1586, .T. ) ;
#63295=ORIENTED_EDGE ( 'NONE', *, *, #32351, .T. ) ;
#63300=CARTESIAN_POINT ( 'NONE',  ( -2.071067811865562991, -146.4375000027311842, 4.999999999999913847 ) ) ;
#63303=ORIENTED_EDGE ( 'NONE', *, *, #4642, .T. ) ;
#63304=CARTESIAN_POINT ( 'NONE',  ( 3.152801135295366208, -145.8125000013655779, 3.152801135295367985 ) ) ;
#63306=CARTESIAN_POINT ( 'NONE',  ( 1.975475456537005874E-15, -70.75000000000000000, 5.000000000000000000 ) ) ;
#63308=CARTESIAN_POINT ( 'NONE',  ( -4.458734124999999437, -69.56249999863439371, 0.000000000000000000 ) ) ;
#63311=CARTESIAN_POINT ( 'NONE',  ( -4.458734125000000326, -142.8750000013656063, 1.846868145590734089 ) ) ;
#63313=ORIENTED_EDGE ( 'NONE', *, *, #16922, .F. ) ;
#63322=CARTESIAN_POINT ( 'NONE',  ( 4.458734124999998549, 24.02083333469892423, -2.574251347313721627 ) ) ;
#63326=ADVANCED_FACE ( 'NONE', ( #17066 ), #21895, .T. ) ;
#63327=EDGE_CURVE ( 'NONE', #36403, #25000, #60823, .T. ) ;
#63333=CARTESIAN_POINT ( 'NONE',  ( -4.458734124999999437, 2.604166668032263043, -2.574251347313719407 ) ) ;
#63334=CARTESIAN_POINT ( 'NONE',  ( -4.458734124999997661, -24.47916666530107577, 2.574251347313722516 ) ) ;
#63335=( BOUNDED_CURVE ( )  B_SPLINE_CURVE ( 2, ( #52601, #32981, #12725, #27207, #32347, #8535, #13043, #32661, #46825 ),
 .UNSPECIFIED., .F., .F. ) 
 B_SPLINE_CURVE_WITH_KNOTS ( ( 3, 2, 2, 2, 3 ),
 ( 0.3020833333333333148, 0.3027777777777777568, 0.3041666666666666408, 0.3055555555555555802, 0.3062500000000000222 ),
 .UNSPECIFIED. ) 
 CURVE ( )  GEOMETRIC_REPRESENTATION_ITEM ( )  RATIONAL_B_SPLINE_CURVE ( ( 0.9330127018922194093, 0.9330127018922194093, 1.000000000000000000, 0.8660254037844387076, 1.000000000000000000, 0.8660254037844387076, 1.000000000000000000, 0.9330127018922194093, 0.9330127018922194093 ) ) 
 REPRESENTATION_ITEM ( '' )  );
#63336=CARTESIAN_POINT ( 'NONE',  ( 3.152801135295366208, -156.5625000013656063, 3.152801135295367985 ) ) ;
#63339=EDGE_CURVE ( 'NONE', #5467, #41613, #6085, .T. ) ;
#63340=CARTESIAN_POINT ( 'NONE',  ( 9.457646018065525792E-16, 26.93750000136559564, 5.148502694627439702 ) ) ;
#63342=EDGE_CURVE ( 'NONE', #27835, #551, #62809, .T. ) ;
#63344=CARTESIAN_POINT ( 'NONE',  ( -4.458734124999999437, -71.56249999863439371, 0.000000000000000000 ) ) ;
#63346=CARTESIAN_POINT ( 'NONE',  ( 5.000000000000000888, -73.58333333333332860, 2.886751345948126879 ) ) ;
#63347=CARTESIAN_POINT ( 'NONE',  ( 5.000000000000000000, -156.1875000027312126, 2.071067811865478614 ) ) ;
#63348=ORIENTED_EDGE ( 'NONE', *, *, #26313, .T. ) ;
#63351=CARTESIAN_POINT ( 'NONE',  ( -5.000000000000000000, -11.99999999999999645, 0.000000000000000000 ) ) ;
#63352=CARTESIAN_POINT ( 'NONE',  ( -4.458734124999999437, -18.31249999863440792, 0.000000000000000000 ) ) ;
#63353=CARTESIAN_POINT ( 'NONE',  ( 2.229367062500001939, -81.97916666530106511, 3.861377020970579999 ) ) ;
#63354=CARTESIAN_POINT ( 'NONE',  ( -1.846868145590734756, -167.3750000013656347, -4.458734125000000326 ) ) ;
#63355=CARTESIAN_POINT ( 'NONE',  ( 5.000000000000000000, -17.37499999726881583, -6.123233995736766282E-16 ) ) ;
#63356=CARTESIAN_POINT ( 'NONE',  ( 2.229367062500001939, -49.97916666530107221, 3.861377020970579999 ) ) ;
#63360=CARTESIAN_POINT ( 'NONE',  ( 9.457646018065525792E-16, 1.687500001365593194, 5.148502694627439702 ) ) ;
#63361=ORIENTED_EDGE ( 'NONE', *, *, #13438, .F. ) ;
#63362=( BOUNDED_CURVE ( )  B_SPLINE_CURVE ( 2, ( #63507, #49008, #9459, #14916, #43549, #15573, #58671, #20068, #19431 ),
 .UNSPECIFIED., .F., .F. ) 
 B_SPLINE_CURVE_WITH_KNOTS ( ( 3, 2, 2, 2, 3 ),
 ( 0.4395833333333333259, 0.4402777777777777679, 0.4416666666666666519, 0.4430555555555555358, 0.4437499999999999778 ),
 .UNSPECIFIED. ) 
 CURVE ( )  GEOMETRIC_REPRESENTATION_ITEM ( )  RATIONAL_B_SPLINE_CURVE ( ( 0.9330127018922194093, 0.9330127018922194093, 1.000000000000000000, 0.8660254037844387076, 1.000000000000000000, 0.8660254037844387076, 1.000000000000000000, 0.9330127018922194093, 0.9330127018922194093 ) ) 
 REPRESENTATION_ITEM ( '' )  );
#63364=CARTESIAN_POINT ( 'NONE',  ( 2.499999999999998668, -62.33333333333333570, -4.330127018922193649 ) ) ;
#63365=CARTESIAN_POINT ( 'NONE',  ( -3.152801135295367096, -156.3125000013656063, -3.152801135295367541 ) ) ;
#63368=CARTESIAN_POINT ( 'NONE',  ( 3.535533905932736864, -163.1250000000000284, 3.535533905932738641 ) ) ;
#63371=VECTOR ( 'NONE', #55769, 1000.000000000000000 ) ;
#63372=CARTESIAN_POINT ( 'NONE',  ( -4.458734124999999437, -3.562499998634407916, 0.000000000000000000 ) ) ;
#63374=CARTESIAN_POINT ( 'NONE',  ( 4.458734125000001214, -46.14583333196773651, 2.574251347313718519 ) ) ;
#63375=CARTESIAN_POINT ( 'NONE',  ( -4.458734125000000326, -148.0000000013655779, -1.846868145590735644 ) ) ;
#63378=VERTEX_POINT ( 'NONE', #26081 ) ;
#63380=CARTESIAN_POINT ( 'NONE',  ( -4.458734124999999437, 29.43750000136559208, 0.000000000000000000 ) ) ;
#63384=EDGE_LOOP ( 'NONE', ( #414, #57759, #53229, #5915 ) ) ;
#63388=CARTESIAN_POINT ( 'NONE',  ( -4.458734124999999437, -0.3958333319677397322, -2.574251347313719407 ) ) ;
#63389=CARTESIAN_POINT ( 'NONE',  ( 1.339745962155615144, -73.58034179853028434, 4.999999999999999112 ) ) ;
#63390=CARTESIAN_POINT ( 'NONE',  ( -3.152801135295367096, -153.0625000013656063, -3.152801135295367541 ) ) ;
#63394=LINE ( 'NONE', #9038, #20253 ) ;
#63395=CARTESIAN_POINT ( 'NONE',  ( -6.972266317189433020E-16, -12.12499999726881406, -5.000000000000000000 ) ) ;
#63402=LINE ( 'NONE', #34110, #17379 ) ;
#63404=CARTESIAN_POINT ( 'NONE',  ( -1.339745962155610925, -71.79465819873850307, 5.000000000000000000 ) ) ;
#63406=CARTESIAN_POINT ( 'NONE',  ( -4.458734124999997661, 19.77083333469893134, 2.574251347313722516 ) ) ;
#63408=CARTESIAN_POINT ( 'NONE',  ( -4.458734124999999437, -9.645833331967738289, -2.574251347313719407 ) ) ;
#63412=CARTESIAN_POINT ( 'NONE',  ( -4.458734124999999437, -166.9375000013655779, -5.460374474430324690E-16 ) ) ;
#63420=CARTESIAN_POINT ( 'NONE',  ( -1.846868145590737420, -154.0000000013656063, 4.458734124999997661 ) ) ;
#63424=CARTESIAN_POINT ( 'NONE',  ( -9.184850993605147944E-16, -167.3750000027312126, 5.000000000000000000 ) ) ;
#63425=VERTEX_POINT ( 'NONE', #48015 ) ;
#63430=CARTESIAN_POINT ( 'NONE',  ( -3.535250795749689387E-16, 0.7500000000000007772, -5.773502691896257311 ) ) ;
#63431=CARTESIAN_POINT ( 'NONE',  ( -2.229367062500000163, -61.47916666530106511, -3.861377020970580443 ) ) ;
#63432=CARTESIAN_POINT ( 'NONE',  ( 0.000000000000000000, -170.0000000000000000, 0.000000000000000000 ) ) ;
#63434=CARTESIAN_POINT ( 'NONE',  ( -5.000000000000000000, -2.958333330602146649, -2.886751345948128211 ) ) ;
#63435=CARTESIAN_POINT ( 'NONE',  ( -4.458734124999999437, -28.39583333196774007, -2.574251347313719407 ) ) ;
#63436=ORIENTED_EDGE ( 'NONE', *, *, #54318, .T. ) ;
#63440=CARTESIAN_POINT ( 'NONE',  ( -3.535250795749689387E-16, -47.25000000000000000, -5.773502691896257311 ) ) ;
#63441=LINE ( 'NONE', #38970, #36595 ) ;
#63443=CARTESIAN_POINT ( 'NONE',  ( -6.972266317189433020E-16, -79.12499999726881583, -5.000000000000000000 ) ) ;
#63444=CARTESIAN_POINT ( 'NONE',  ( -4.458734124999999437, -72.31249999863439371, 0.000000000000000000 ) ) ;
#63445=CARTESIAN_POINT ( 'NONE',  ( -4.458734125000001214, -144.1250000013655779, 1.846868145590734089 ) ) ;
#63446=CARTESIAN_POINT ( 'NONE',  ( -2.229367062499996610, -79.14583333196773651, 3.861377020970582219 ) ) ;
#63448=CARTESIAN_POINT ( 'NONE',  ( 4.458734125000001214, -29.14583333196774362, 2.574251347313718519 ) ) ;
#63449=CARTESIAN_POINT ( 'NONE',  ( -5.000000000000000000, -67.87499999726881583, 0.000000000000000000 ) ) ;
#63454=CARTESIAN_POINT ( 'NONE',  ( -1.339745962155617365, 22.33034180399266688, 4.999999999999998224 ) ) ;
#63456=CARTESIAN_POINT ( 'NONE',  ( 1.339745962155612258, 27.29465819873851729, 5.000000000000000888 ) ) ;
#63457=CARTESIAN_POINT ( 'NONE',  ( -1.049326080737009628E-13, -2.750000000000003109, 5.000000000000000000 ) ) ;
#63458=CARTESIAN_POINT ( 'NONE',  ( 4.458734124999999437, -61.06249999863440081, -5.460374474430324690E-16 ) ) ;
#63464=CARTESIAN_POINT ( 'NONE',  ( -2.229367062500000163, 10.52083333469892779, -3.861377020970580443 ) ) ;
#63467=CARTESIAN_POINT ( 'NONE',  ( 1.846868145590735200, -165.2500000013655779, -4.458734124999999437 ) ) ;
#63470=CARTESIAN_POINT ( 'NONE',  ( -2.500000000000000444, -52.04166666393547303, -4.330127018922193649 ) ) ;
#63472=( BOUNDED_CURVE ( )  B_SPLINE_CURVE ( 2, ( #26326, #45943, #41109, #60756, #16680, #36301, #41427, #61076, #27280 ),
 .UNSPECIFIED., .F., .F. ) 
 B_SPLINE_CURVE_WITH_KNOTS ( ( 3, 2, 2, 2, 3 ),
 ( 0.008333333333333340157, 0.01250000000000001110, 0.01666666666666668031, 0.02083333333333334952, 0.02500000000000002220 ),
 .UNSPECIFIED. ) 
 CURVE ( )  GEOMETRIC_REPRESENTATION_ITEM ( )  RATIONAL_B_SPLINE_CURVE ( ( 0.9999999999999998890, 0.9238795325112868495, 1.000000000000000000, 0.9238795325112867385, 1.000000000000000000, 0.9238795325112867385, 1.000000000000000000, 0.9238795325112864054, 1.000000000000000444 ) ) 
 REPRESENTATION_ITEM ( '' )  );
#63477=CARTESIAN_POINT ( 'NONE',  ( -1.339745962155610925, -82.66965819600731891, 5.000000000000000000 ) ) ;
#63478=CARTESIAN_POINT ( 'NONE',  ( 5.000000000000000000, -58.50000000000000000, -6.123233995736766282E-16 ) ) ;
#63481=CARTESIAN_POINT ( 'NONE',  ( -4.458734124999999437, 5.437500001365592972, 0.000000000000000000 ) ) ;
#63484=CARTESIAN_POINT ( 'NONE',  ( 5.000000000000000000, -149.1250000027312126, 0.000000000000000000 ) ) ;
#63489=CARTESIAN_POINT ( 'NONE',  ( -3.535533905932737309, -143.6250000000000000, -3.535533905932738197 ) ) ;
#63491=CARTESIAN_POINT ( 'NONE',  ( -1.846868145590734756, -164.3750000013656063, -4.458734124999999437 ) ) ;
#63492=CARTESIAN_POINT ( 'NONE',  ( 4.458734124999998549, -28.72916666530107221, -2.574251347313721627 ) ) ;
#63496=CARTESIAN_POINT ( 'NONE',  ( 1.846868145590736310, -145.6250000013655779, 4.458734124999999437 ) ) ;
#63497=ORIENTED_EDGE ( 'NONE', *, *, #3872, .F. ) ;
#63498=CARTESIAN_POINT ( 'NONE',  ( 4.458734124999998549, 26.02083333469892779, -2.574251347313721627 ) ) ;
#63499=CARTESIAN_POINT ( 'NONE',  ( 0.000000000000000000, -170.0000000000000000, 0.000000000000000000 ) ) ;
#63500=CARTESIAN_POINT ( 'NONE',  ( -2.229367062500000163, -57.72916666530107932, -3.861377020970580443 ) ) ;
#63501=AXIS2_PLACEMENT_3D ( 'NONE', #35144, #1065, #40589 ) ;
#63503=CARTESIAN_POINT ( 'NONE',  ( 2.499999999999998668, -90.20833333060214443, -4.330127018922193649 ) ) ;
#63504=CARTESIAN_POINT ( 'NONE',  ( -2.500000000000000444, 17.83333333333333215, -4.330127018922193649 ) ) ;
#63506=CARTESIAN_POINT ( 'NONE',  ( 2.229367062500001939, -5.979166665301072214, 3.861377020970579999 ) ) ;
#63507=CARTESIAN_POINT ( 'NONE',  ( 1.975475456537005874E-15, -22.74999999999999645, 5.000000000000000000 ) ) ;
#63508=CARTESIAN_POINT ( 'NONE',  ( 2.071067811865518582, -165.3125000027312126, 4.999999999999957367 ) ) ;
#63513=FACE_OUTER_BOUND ( 'NONE', #21171, .T. ) ;
#63514=CARTESIAN_POINT ( 'NONE',  ( 4.458734125000001214, -51.89583333196773651, 2.574251347313718519 ) ) ;
#63515=CARTESIAN_POINT ( 'NONE',  ( -3.152801135295367985, -155.0625000013656063, 3.152801135295367096 ) ) ;
#63516=CARTESIAN_POINT ( 'NONE',  ( 5.000000000000000000, -51.29166666393547303, -2.886751345948129988 ) ) ;
#63517=ORIENTED_EDGE ( 'NONE', *, *, #61587, .F. ) ;
#63518=CARTESIAN_POINT ( 'NONE',  ( -4.458734124999998549, 4.520833334698926009, 2.574251347313722516 ) ) ;
#63522=CARTESIAN_POINT ( 'NONE',  ( 3.152801135295366208, -159.5625000013656063, 3.152801135295367985 ) ) ;
#63528=CARTESIAN_POINT ( 'NONE',  ( -1.339745962155613812, -30.08034179853029144, -5.000000000000000000 ) ) ;
#63529=CARTESIAN_POINT ( 'NONE',  ( 4.458734124999998549, -41.97916666530107932, -2.574251347313721627 ) ) ;
#63530=ORIENTED_EDGE ( 'NONE', *, *, #37716, .T. ) ;
#63531=CARTESIAN_POINT ( 'NONE',  ( -5.000000000000000000, -46.00000000000000000, 0.000000000000000000 ) ) ;
#63533=CARTESIAN_POINT ( 'NONE',  ( -6.972266317189433020E-16, -66.24999999999998579, -5.000000000000000000 ) ) ;
#63535=CARTESIAN_POINT ( 'NONE',  ( -4.458734124999999437, 28.68750000136559208, 0.000000000000000000 ) ) ;
#63537=FACE_OUTER_BOUND ( 'NONE', #13049, .T. ) ;
#63540=CARTESIAN_POINT ( 'NONE',  ( 3.061616997868383141E-16, -168.7500000000000000, -5.000000000000000000 ) ) ;
#63549=CARTESIAN_POINT ( 'NONE',  ( -2.499999999999996447, -19.70833333060214798, 4.330127018922195425 ) ) ;
#63552=EDGE_CURVE ( 'NONE', #19516, #50575, #57063, .T. ) ;
#63556=CARTESIAN_POINT ( 'NONE',  ( -1.339745962155613812, -81.20534180126146850, -5.000000000000000000 ) ) ;
#63558=CARTESIAN_POINT ( 'NONE',  ( -2.071067811865475061, -160.8125000027311842, -5.000000000000000888 ) ) ;
#63568=CARTESIAN_POINT ( 'NONE',  ( -2.500000000000000444, -54.16666666666667140, -4.330127018922193649 ) ) ;
#63569=CARTESIAN_POINT ( 'NONE',  ( 2.229367062499998831, -16.64583333196773651, -3.861377020970580887 ) ) ;
#63571=CARTESIAN_POINT ( 'NONE',  ( -3.535533905932738641, -153.3750000000000000, 3.535533905932737309 ) ) ;
#63573=ORIENTED_EDGE ( 'NONE', *, *, #4033, .F. ) ;
#63574=CARTESIAN_POINT ( 'NONE',  ( 4.458734124999999437, -41.06249999863440081, -5.460374474430324690E-16 ) ) ;
#63575=CARTESIAN_POINT ( 'NONE',  ( 3.061616997868383141E-16, -150.7500000000000284, -5.000000000000000000 ) ) ;
#63580=CARTESIAN_POINT ( 'NONE',  ( -4.458734124999998549, 9.770833334698927786, 2.574251347313722516 ) ) ;
#63582=DIRECTION ( 'NONE',  ( -0.000000000000000000, 1.000000000000000000, -0.000000000000000000 ) ) ;
#63583=CARTESIAN_POINT ( 'NONE',  ( -3.152548672688508926E-16, -86.81249999863439371, -5.148502694627439702 ) ) ;
#63584=CARTESIAN_POINT ( 'NONE',  ( -2.229367062500000163, 22.27083333469892423, -3.861377020970580443 ) ) ;
#63586=CARTESIAN_POINT ( 'NONE',  ( -3.535250795749689387E-16, 11.87500000273118594, -5.773502691896257311 ) ) ;
#63588=CARTESIAN_POINT ( 'NONE',  ( 5.000000000000000000, -79.41666666666665719, -2.886751345948130876 ) ) ;
#63589=ORIENTED_EDGE ( 'NONE', *, *, #63263, .F. ) ;
#63590=CARTESIAN_POINT ( 'NONE',  ( 1.975475456537005874E-15, -85.75000000000000000, 5.000000000000000000 ) ) ;
#63591=CARTESIAN_POINT ( 'NONE',  ( -2.499999999999996447, -33.83333333333332860, 4.330127018922195425 ) ) ;
#63592=CARTESIAN_POINT ( 'NONE',  ( -4.458734124999999437, -38.31249999863439371, 0.000000000000000000 ) ) ;
#63593=VECTOR ( 'NONE', #13226, 1000.000000000000000 ) ;
#63594=CARTESIAN_POINT ( 'NONE',  ( 5.000000000000000888, -32.45833333060215153, 2.886751345948126879 ) ) ;
#63595=CARTESIAN_POINT ( 'NONE',  ( -2.229367062499996610, -68.14583333196773651, 3.861377020970582219 ) ) ;
#63598=CARTESIAN_POINT ( 'NONE',  ( -4.458734124999999437, -12.31249999863440259, 0.000000000000000000 ) ) ;
#63599=CARTESIAN_POINT ( 'NONE',  ( -2.229367062500000163, -12.72916666530107044, -3.861377020970580443 ) ) ;
#63601=CARTESIAN_POINT ( 'NONE',  ( 1.060575238724906964E-15, -81.75000000000000000, 5.773502691896257311 ) ) ;
#63604=CARTESIAN_POINT ( 'NONE',  ( -5.000000000000000000, -84.87499999726880162, 0.000000000000000000 ) ) ;
#63609=CARTESIAN_POINT ( 'NONE',  ( -2.229367062500000163, -28.72916666530107221, -3.861377020970580443 ) ) ;
#63611=CARTESIAN_POINT ( 'NONE',  ( 4.458734125000000326, -167.6250000013655779, -1.846868145590734978 ) ) ;
#63613=CARTESIAN_POINT ( 'NONE',  ( 5.000000000000000000, -8.374999997268814056, -6.123233995736766282E-16 ) ) ;
#63618=CARTESIAN_POINT ( 'NONE',  ( -1.846868145590734756, -146.3750000013655779, -4.458734124999999437 ) ) ;
#63619=CARTESIAN_POINT ( 'NONE',  ( -6.972266317189433020E-16, 22.74999999999999645, -5.000000000000000000 ) ) ;
#63625=CARTESIAN_POINT ( 'NONE',  ( 4.458734124999999437, -144.6875000013656063, 0.000000000000000000 ) ) ;
#63630=CARTESIAN_POINT ( 'NONE',  ( 4.458734125000001214, -69.14583333196773651, 2.574251347313718519 ) ) ;
#63632=CARTESIAN_POINT ( 'NONE',  ( -1.339745962155610925, -69.79465819873850307, 5.000000000000000000 ) ) ;
#63634=MECHANICAL_DESIGN_GEOMETRIC_PRESENTATION_REPRESENTATION('',(#55424),#61631);
#63643=CARTESIAN_POINT ( 'NONE',  ( -2.229367062499996610, 23.60416666803225993, 3.861377020970582219 ) ) ;
#63645=ADVANCED_FACE ( 'NONE', ( #32597 ), #52543, .T. ) ;
#63651=CARTESIAN_POINT ( 'NONE',  ( -2.229367062499996610, 3.854166668032260823, 3.861377020970582219 ) ) ;
#63653=CARTESIAN_POINT ( 'NONE',  ( -4.458734124999999437, -22.56249999863440436, 0.000000000000000000 ) ) ;
#63656=( BOUNDED_CURVE ( )  B_SPLINE_CURVE ( 2, ( #45116, #10384, #15540, #34489, #35159, #54774, #10706, #5889, #31596 ),
 .UNSPECIFIED., .F., .F. ) 
 B_SPLINE_CURVE_WITH_KNOTS ( ( 3, 2, 2, 2, 3 ),
 ( 0.8479166666666666519, 0.8486111111111110938, 0.8499999999999999778, 0.8513888888888888618, 0.8520833333333333037 ),
 .UNSPECIFIED. ) 
 CURVE ( )  GEOMETRIC_REPRESENTATION_ITEM ( )  RATIONAL_B_SPLINE_CURVE ( ( 0.9330127018922194093, 0.9330127018922194093, 1.000000000000000000, 0.8660254037844387076, 1.000000000000000000, 0.8660254037844387076, 1.000000000000000000, 0.9330127018922194093, 0.9330127018922194093 ) ) 
 REPRESENTATION_ITEM ( '' )  );
#63657=CARTESIAN_POINT ( 'NONE',  ( 2.229367062499998831, 26.35416666803225993, -3.861377020970580887 ) ) ;
#63661=CARTESIAN_POINT ( 'NONE',  ( -3.152548672688508926E-16, -74.81249999863439371, -5.148502694627439702 ) ) ;
#63667=CARTESIAN_POINT ( 'NONE',  ( 5.000000000000000000, -6.291666663935481019, -2.886751345948130876 ) ) ;
#63668=CARTESIAN_POINT ( 'NONE',  ( -2.499999999999996447, -18.83333333333333215, 4.330127018922195425 ) ) ;
#63669=CARTESIAN_POINT ( 'NONE',  ( 4.458734124999999437, -22.81249999863440436, -5.460374474430324690E-16 ) ) ;
#63670=CARTESIAN_POINT ( 'NONE',  ( 4.458734125000000326, -81.89583333196773651, 2.574251347313718519 ) ) ;
#63671=CARTESIAN_POINT ( 'NONE',  ( 4.458734125000000326, -166.6250000013656063, -1.846868145590734978 ) ) ;
#63672=CARTESIAN_POINT ( 'NONE',  ( 2.499999999999998668, -18.20833333060214798, -4.330127018922193649 ) ) ;
#63673=CARTESIAN_POINT ( 'NONE',  ( 9.457646018065525792E-16, -49.06249999863440792, 5.148502694627439702 ) ) ;
#63674=CARTESIAN_POINT ( 'NONE',  ( -4.999999999999998224, -64.91666666666665719, 2.886751345948131764 ) ) ;
#63692=COLOUR_RGB('Light Blue',0.38,0.62,0.78);
#63693=FILL_AREA_STYLE_COLOUR('',#63692);
#63694=FILL_AREA_STYLE('',(#63693));
#63695=SURFACE_STYLE_FILL_AREA(#63694);
#63696=SURFACE_SIDE_STYLE('',(#63695));
#63697=SURFACE_STYLE_USAGE(.BOTH.,#63696);
#63698=PRESENTATION_STYLE_ASSIGNMENT((#63697));
ENDSEC;
END-ISO-10303-21;
